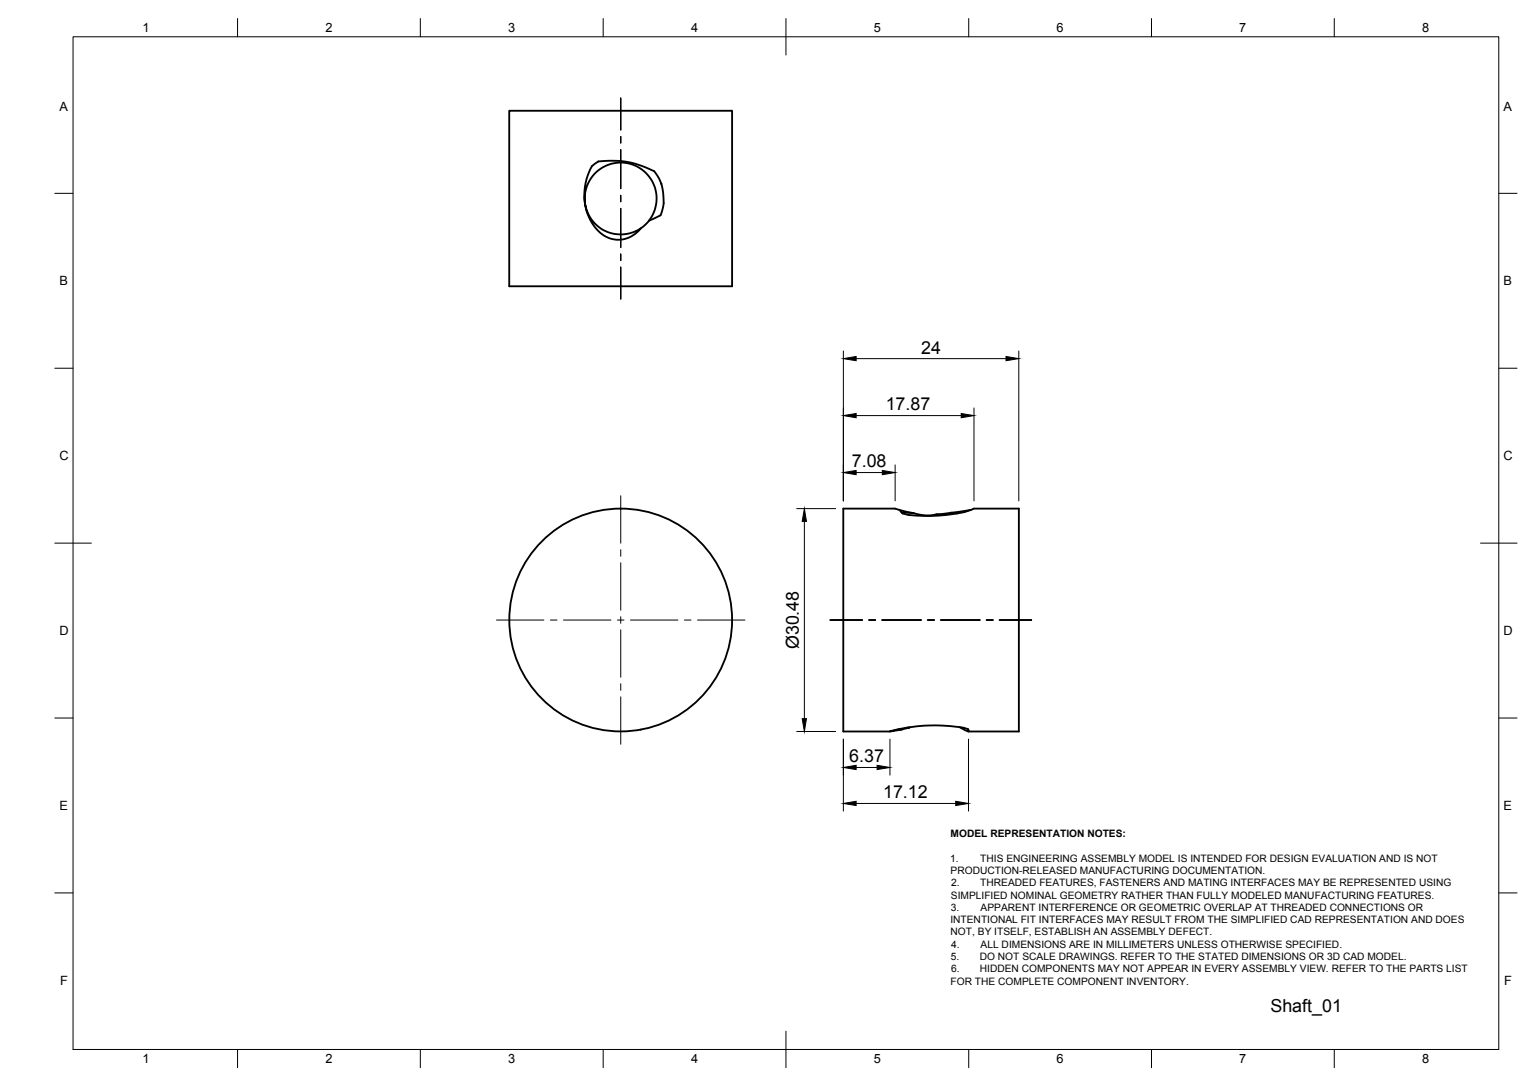
ISO-10303-21;
HEADER;
/* Generated by software containing ST-Developer
 * from STEP Tools, Inc. (www.steptools.com) 
 */

FILE_DESCRIPTION(
/* description */ (''),
/* implementation_level */ '2;1');

FILE_NAME(
/* name */ 'Shaft_01.step',
/* time_stamp */ '2026-10-06T13:41:14-07:00',
/* author */ (''),
/* organization */ (''),
/* preprocessor_version */ 'ST-DEVELOPER v20.2',
/* originating_system */ 'Autodesk Translation Framework v15.15.0.0',
/* authorisation */ '');

FILE_SCHEMA (('AUTOMOTIVE_DESIGN { 1 0 10303 214 3 1 1 }'));
ENDSEC;

DATA;
#10=MECHANICAL_DESIGN_GEOMETRIC_PRESENTATION_REPRESENTATION('',(#1963),#279266);
#49=B_SPLINE_SURFACE_WITH_KNOTS('',3,3,((#209501,#209502,#209503,#209504,
#209505,#209506,#209507,#209508,#209509,#209510,#209511,#209512,#209513,
#209514,#209515,#209516,#209517,#209518,#209519,#209520,#209521,#209522,
#209523,#209524,#209525,#209526,#209527,#209528,#209529,#209530,#209531,
#209532,#209533,#209534,#209535,#209536,#209537,#209538,#209539,#209540,
#209541,#209542,#209543,#209544,#209545,#209546,#209547,#209548,#209549,
#209550,#209551,#209552,#209553,#209554,#209555,#209556,#209557,#209558,
#209559,#209560,#209561,#209562,#209563,#209564,#209565,#209566,#209567,
#209568,#209569,#209570,#209571,#209572,#209573,#209574,#209575,#209576,
#209577,#209578,#209579,#209580,#209581,#209582,#209583,#209584,#209585,
#209586,#209587,#209588,#209589,#209590,#209591,#209592,#209593,#209594,
#209595,#209596,#209597,#209598,#209599,#209600,#209601,#209602,#209603,
#209604,#209605,#209606,#209607,#209608,#209609,#209610,#209611,#209612,
#209613,#209614,#209615,#209616,#209617,#209618,#209619,#209620,#209621,
#209622,#209623,#209624,#209625,#209626,#209627,#209628,#209629,#209630,
#209631,#209632,#209633,#209634,#209635,#209636,#209637,#209638,#209639,
#209640,#209641,#209642,#209643,#209644,#209645,#209646,#209647,#209648,
#209649,#209650,#209651,#209652,#209653,#209654,#209655,#209656,#209657,
#209658,#209659,#209660,#209661,#209662,#209663,#209664,#209665,#209666,
#209667,#209668,#209669,#209670,#209671,#209672,#209673,#209674,#209675,
#209676,#209677,#209678,#209679,#209680,#209681,#209682,#209683,#209684,
#209685,#209686,#209687,#209688,#209689,#209690,#209691,#209692,#209693,
#209694,#209695,#209696,#209697,#209698,#209699,#209700,#209701,#209702,
#209703,#209704,#209705,#209706,#209707,#209708,#209709,#209710,#209711,
#209712,#209713,#209714,#209715,#209716,#209717,#209718,#209719,#209720,
#209721,#209722,#209723,#209724,#209725,#209726,#209727,#209728,#209729,
#209730,#209731,#209732,#209733,#209734,#209735,#209736,#209737,#209738,
#209739,#209740,#209741,#209742,#209743,#209744,#209745,#209746,#209747,
#209748,#209749,#209750,#209751,#209752,#209753,#209754,#209755,#209756,
#209757,#209758,#209759,#209760,#209761,#209762,#209763,#209764,#209765,
#209766,#209767,#209768,#209769,#209770,#209771,#209772,#209773,#209774,
#209775,#209776,#209777,#209778,#209779,#209780,#209781,#209782,#209783,
#209784,#209785,#209786,#209787,#209788,#209789,#209790,#209791,#209792,
#209793,#209794,#209795,#209796,#209797,#209798,#209799,#209800,#209801,
#209802,#209803,#209804,#209805,#209806,#209807,#209808,#209809,#209810,
#209811,#209812,#209813,#209814,#209815,#209816,#209817,#209818,#209819,
#209820,#209821,#209822,#209823,#209824,#209825,#209826,#209827,#209828,
#209829,#209830,#209831,#209832,#209833,#209834,#209835,#209836,#209837,
#209838,#209839,#209840,#209841,#209842,#209843,#209844,#209845,#209846,
#209847,#209848,#209849,#209850,#209851,#209852,#209853,#209854,#209855,
#209856,#209857,#209858,#209859,#209860,#209861,#209862,#209863,#209864,
#209865,#209866,#209867,#209868,#209869,#209870,#209871,#209872,#209873,
#209874,#209875,#209876,#209877,#209878,#209879,#209880,#209881,#209882,
#209883,#209884,#209885,#209886,#209887,#209888,#209889,#209890,#209891,
#209892,#209893,#209894,#209895,#209896,#209897,#209898,#209899,#209900,
#209901,#209902,#209903,#209904,#209905,#209906,#209907,#209908,#209909,
#209910,#209911,#209912,#209913,#209914,#209915,#209916,#209917,#209918,
#209919,#209920,#209921,#209922,#209923,#209924,#209925,#209926,#209927,
#209928,#209929,#209930,#209931,#209932,#209933,#209934,#209935,#209936,
#209937,#209938,#209939,#209940,#209941,#209942,#209943,#209944,#209945,
#209946,#209947,#209948,#209949,#209950,#209951,#209952,#209953,#209954,
#209955,#209956,#209957,#209958,#209959,#209960,#209961,#209962,#209963,
#209964,#209965,#209966,#209967,#209968,#209969,#209970,#209971,#209972,
#209973,#209974,#209975,#209976,#209977,#209978,#209979,#209980,#209981,
#209982,#209983,#209984,#209985,#209986,#209987,#209988,#209989,#209990,
#209991,#209992,#209993,#209994,#209995,#209996,#209997,#209998,#209999,
#210000,#210001,#210002,#210003,#210004,#210005,#210006,#210007,#210008,
#210009,#210010,#210011,#210012,#210013,#210014,#210015,#210016,#210017,
#210018,#210019,#210020,#210021,#210022,#210023,#210024,#210025,#210026,
#210027,#210028,#210029,#210030,#210031,#210032,#210033,#210034,#210035,
#210036,#210037,#210038,#210039,#210040,#210041,#210042,#210043,#210044,
#210045,#210046,#210047,#210048,#210049,#210050,#210051,#210052,#210053,
#210054,#210055,#210056,#210057,#210058,#210059,#210060,#210061,#210062,
#210063,#210064,#210065,#210066,#210067,#210068,#210069,#210070,#210071,
#210072,#210073,#210074,#210075,#210076,#210077,#210078,#210079,#210080,
#210081,#210082,#210083,#210084,#210085,#210086,#210087,#210088,#210089,
#210090,#210091,#210092,#210093,#210094,#210095,#210096,#210097,#210098,
#210099,#210100,#210101,#210102,#210103,#210104,#210105,#210106,#210107,
#210108,#210109,#210110,#210111,#210112,#210113,#210114,#210115,#210116,
#210117,#210118,#210119,#210120,#210121,#210122,#210123,#210124,#210125,
#210126,#210127,#210128,#210129,#210130,#210131,#210132,#210133,#210134,
#210135,#210136,#210137,#210138,#210139,#210140,#210141,#210142,#210143,
#210144,#210145,#210146,#210147,#210148,#210149,#210150,#210151,#210152,
#210153,#210154,#210155,#210156,#210157,#210158,#210159,#210160,#210161,
#210162,#210163,#210164,#210165,#210166,#210167,#210168,#210169,#210170,
#210171,#210172,#210173,#210174,#210175,#210176,#210177,#210178,#210179,
#210180,#210181,#210182,#210183,#210184,#210185,#210186,#210187,#210188,
#210189,#210190,#210191,#210192,#210193,#210194,#210195,#210196,#210197,
#210198,#210199,#210200,#210201,#210202,#210203,#210204,#210205,#210206,
#210207,#210208,#210209,#210210,#210211,#210212,#210213,#210214,#210215,
#210216,#210217,#210218,#210219,#210220,#210221,#210222,#210223,#210224,
#210225,#210226,#210227,#210228,#210229,#210230,#210231,#210232,#210233,
#210234,#210235,#210236,#210237,#210238,#210239,#210240,#210241,#210242,
#210243,#210244,#210245,#210246,#210247,#210248,#210249,#210250,#210251,
#210252,#210253,#210254,#210255,#210256,#210257,#210258,#210259,#210260,
#210261,#210262,#210263,#210264,#210265,#210266,#210267,#210268,#210269,
#210270,#210271,#210272,#210273,#210274,#210275,#210276,#210277,#210278,
#210279,#210280,#210281,#210282,#210283,#210284,#210285,#210286,#210287,
#210288,#210289,#210290,#210291,#210292,#210293,#210294,#210295,#210296,
#210297,#210298,#210299,#210300,#210301,#210302,#210303,#210304,#210305,
#210306,#210307,#210308,#210309,#210310,#210311,#210312,#210313,#210314,
#210315,#210316,#210317,#210318,#210319,#210320,#210321,#210322,#210323,
#210324,#210325,#210326,#210327,#210328,#210329,#210330,#210331,#210332,
#210333,#210334,#210335,#210336,#210337,#210338,#210339,#210340,#210341,
#210342,#210343,#210344,#210345,#210346,#210347,#210348,#210349,#210350,
#210351,#210352,#210353,#210354,#210355,#210356,#210357,#210358,#210359,
#210360,#210361,#210362,#210363,#210364,#210365,#210366,#210367,#210368,
#210369,#210370,#210371,#210372,#210373,#210374,#210375,#210376,#210377,
#210378,#210379,#210380,#210381,#210382,#210383,#210384,#210385,#210386,
#210387,#210388,#210389,#210390,#210391,#210392,#210393,#210394,#210395,
#210396,#210397,#210398,#210399,#210400,#210401,#210402,#210403,#210404,
#210405,#210406,#210407,#210408,#210409,#210410,#210411,#210412,#210413,
#210414,#210415,#210416,#210417,#210418,#210419,#210420,#210421,#210422,
#210423,#210424,#210425,#210426,#210427,#210428,#210429,#210430,#210431,
#210432,#210433,#210434,#210435,#210436,#210437,#210438,#210439,#210440,
#210441,#210442,#210443,#210444,#210445,#210446,#210447,#210448,#210449,
#210450,#210451,#210452,#210453,#210454,#210455,#210456,#210457,#210458,
#210459,#210460,#210461,#210462,#210463,#210464,#210465,#210466,#210467,
#210468,#210469,#210470,#210471,#210472,#210473,#210474,#210475,#210476,
#210477,#210478,#210479,#210480,#210481,#210482,#210483,#210484,#210485,
#210486,#210487,#210488,#210489,#210490,#210491,#210492,#210493,#210494,
#210495,#210496,#210497,#210498,#210499,#210500,#210501,#210502,#210503,
#210504,#210505,#210506,#210507,#210508,#210509,#210510,#210511,#210512,
#210513,#210514,#210515,#210516,#210517,#210518,#210519,#210520,#210521,
#210522,#210523,#210524,#210525,#210526,#210527,#210528,#210529,#210530,
#210531,#210532,#210533,#210534,#210535,#210536,#210537,#210538,#210539,
#210540,#210541,#210542,#210543,#210544,#210545,#210546,#210547,#210548,
#210549,#210550,#210551,#210552,#210553,#210554,#210555,#210556,#210557,
#210558,#210559,#210560,#210561,#210562,#210563,#210564,#210565,#210566,
#210567,#210568,#210569,#210570,#210571,#210572,#210573,#210574,#210575,
#210576,#210577,#210578,#210579,#210580,#210581,#210582,#210583,#210584,
#210585,#210586,#210587,#210588,#210589,#210590,#210591,#210592,#210593,
#210594,#210595,#210596,#210597,#210598,#210599,#210600,#210601,#210602,
#210603,#210604,#210605,#210606,#210607,#210608,#210609,#210610,#210611,
#210612,#210613,#210614,#210615,#210616,#210617,#210618,#210619,#210620,
#210621,#210622,#210623,#210624,#210625,#210626,#210627,#210628,#210629,
#210630,#210631,#210632,#210633,#210634,#210635,#210636,#210637,#210638,
#210639,#210640,#210641,#210642,#210643,#210644,#210645,#210646,#210647,
#210648,#210649,#210650,#210651,#210652,#210653,#210654,#210655,#210656,
#210657,#210658,#210659,#210660,#210661,#210662,#210663,#210664,#210665,
#210666,#210667,#210668,#210669,#210670,#210671,#210672,#210673,#210674,
#210675,#210676,#210677,#210678,#210679,#210680,#210681,#210682,#210683,
#210684,#210685,#210686,#210687,#210688,#210689,#210690,#210691,#210692,
#210693,#210694,#210695,#210696,#210697,#210698,#210699,#210700,#210701,
#210702,#210703,#210704,#210705,#210706,#210707,#210708,#210709,#210710,
#210711,#210712,#210713,#210714,#210715,#210716,#210717,#210718,#210719,
#210720,#210721,#210722,#210723,#210724,#210725,#210726,#210727,#210728,
#210729,#210730,#210731,#210732,#210733,#210734,#210735,#210736,#210737,
#210738,#210739,#210740,#210741,#210742,#210743,#210744,#210745,#210746,
#210747,#210748,#210749,#210750,#210751,#210752,#210753,#210754,#210755,
#210756,#210757,#210758,#210759,#210760,#210761,#210762,#210763,#210764,
#210765,#210766,#210767,#210768,#210769,#210770,#210771,#210772,#210773,
#210774,#210775,#210776,#210777,#210778,#210779,#210780,#210781,#210782,
#210783,#210784,#210785,#210786,#210787,#210788,#210789,#210790,#210791,
#210792,#210793,#210794,#210795,#210796,#210797,#210798,#210799,#210800,
#210801,#210802,#210803,#210804,#210805,#210806,#210807,#210808,#210809,
#210810,#210811,#210812,#210813,#210814,#210815,#210816,#210817,#210818,
#210819,#210820,#210821,#210822,#210823,#210824,#210825,#210826,#210827,
#210828,#210829,#210830,#210831,#210832,#210833,#210834,#210835,#210836,
#210837,#210838,#210839,#210840,#210841,#210842,#210843,#210844,#210845,
#210846,#210847,#210848,#210849,#210850,#210851,#210852,#210853,#210854,
#210855,#210856,#210857,#210858,#210859,#210860,#210861,#210862,#210863,
#210864,#210865,#210866,#210867,#210868,#210869,#210870,#210871,#210872,
#210873,#210874,#210875,#210876,#210877,#210878,#210879,#210880,#210881,
#210882,#210883,#210884,#210885,#210886,#210887,#210888,#210889,#210890,
#210891,#210892,#210893,#210894,#210895,#210896,#210897,#210898,#210899,
#210900,#210901,#210902,#210903,#210904,#210905,#210906,#210907,#210908,
#210909,#210910,#210911,#210912,#210913,#210914,#210915,#210916,#210917,
#210918,#210919,#210920,#210921,#210922,#210923,#210924,#210925,#210926,
#210927,#210928,#210929,#210930,#210931,#210932,#210933,#210934,#210935,
#210936,#210937,#210938,#210939,#210940,#210941,#210942,#210943,#210944,
#210945,#210946,#210947,#210948,#210949,#210950,#210951,#210952,#210953,
#210954,#210955,#210956,#210957,#210958,#210959,#210960,#210961,#210962,
#210963,#210964,#210965,#210966,#210967,#210968,#210969,#210970,#210971,
#210972,#210973,#210974,#210975,#210976,#210977,#210978,#210979,#210980,
#210981,#210982,#210983,#210984,#210985,#210986,#210987,#210988,#210989,
#210990,#210991,#210992,#210993,#210994,#210995,#210996,#210997,#210998,
#210999,#211000,#211001,#211002,#211003,#211004,#211005,#211006,#211007,
#211008,#211009,#211010,#211011,#211012,#211013,#211014,#211015,#211016,
#211017,#211018,#211019,#211020,#211021,#211022,#211023,#211024,#211025,
#211026,#211027,#211028,#211029,#211030,#211031,#211032,#211033,#211034,
#211035,#211036,#211037,#211038,#211039,#211040,#211041,#211042,#211043,
#211044,#211045,#211046,#211047,#211048,#211049,#211050,#211051,#211052,
#211053,#211054,#211055,#211056,#211057,#211058,#211059,#211060,#211061,
#211062,#211063,#211064,#211065,#211066,#211067,#211068,#211069,#211070,
#211071,#211072,#211073,#211074,#211075,#211076,#211077,#211078,#211079,
#211080,#211081,#211082,#211083,#211084,#211085,#211086,#211087,#211088,
#211089,#211090,#211091,#211092,#211093,#211094,#211095,#211096,#211097,
#211098,#211099,#211100,#211101,#211102,#211103,#211104,#211105,#211106,
#211107,#211108,#211109,#211110,#211111,#211112,#211113,#211114,#211115,
#211116,#211117,#211118,#211119,#211120,#211121,#211122,#211123,#211124,
#211125,#211126,#211127,#211128,#211129,#211130,#211131,#211132,#211133,
#211134,#211135,#211136,#211137,#211138,#211139,#211140,#211141,#211142,
#211143,#211144,#211145,#211146,#211147,#211148,#211149,#211150,#211151,
#211152,#211153,#211154,#211155,#211156,#211157,#211158,#211159,#211160,
#211161,#211162,#211163,#211164,#211165,#211166,#211167,#211168,#211169,
#211170,#211171,#211172,#211173,#211174,#211175,#211176,#211177,#211178,
#211179,#211180,#211181,#211182,#211183,#211184,#211185,#211186,#211187,
#211188,#211189,#211190,#211191,#211192,#211193,#211194,#211195),(#211196,
#211197,#211198,#211199,#211200,#211201,#211202,#211203,#211204,#211205,
#211206,#211207,#211208,#211209,#211210,#211211,#211212,#211213,#211214,
#211215,#211216,#211217,#211218,#211219,#211220,#211221,#211222,#211223,
#211224,#211225,#211226,#211227,#211228,#211229,#211230,#211231,#211232,
#211233,#211234,#211235,#211236,#211237,#211238,#211239,#211240,#211241,
#211242,#211243,#211244,#211245,#211246,#211247,#211248,#211249,#211250,
#211251,#211252,#211253,#211254,#211255,#211256,#211257,#211258,#211259,
#211260,#211261,#211262,#211263,#211264,#211265,#211266,#211267,#211268,
#211269,#211270,#211271,#211272,#211273,#211274,#211275,#211276,#211277,
#211278,#211279,#211280,#211281,#211282,#211283,#211284,#211285,#211286,
#211287,#211288,#211289,#211290,#211291,#211292,#211293,#211294,#211295,
#211296,#211297,#211298,#211299,#211300,#211301,#211302,#211303,#211304,
#211305,#211306,#211307,#211308,#211309,#211310,#211311,#211312,#211313,
#211314,#211315,#211316,#211317,#211318,#211319,#211320,#211321,#211322,
#211323,#211324,#211325,#211326,#211327,#211328,#211329,#211330,#211331,
#211332,#211333,#211334,#211335,#211336,#211337,#211338,#211339,#211340,
#211341,#211342,#211343,#211344,#211345,#211346,#211347,#211348,#211349,
#211350,#211351,#211352,#211353,#211354,#211355,#211356,#211357,#211358,
#211359,#211360,#211361,#211362,#211363,#211364,#211365,#211366,#211367,
#211368,#211369,#211370,#211371,#211372,#211373,#211374,#211375,#211376,
#211377,#211378,#211379,#211380,#211381,#211382,#211383,#211384,#211385,
#211386,#211387,#211388,#211389,#211390,#211391,#211392,#211393,#211394,
#211395,#211396,#211397,#211398,#211399,#211400,#211401,#211402,#211403,
#211404,#211405,#211406,#211407,#211408,#211409,#211410,#211411,#211412,
#211413,#211414,#211415,#211416,#211417,#211418,#211419,#211420,#211421,
#211422,#211423,#211424,#211425,#211426,#211427,#211428,#211429,#211430,
#211431,#211432,#211433,#211434,#211435,#211436,#211437,#211438,#211439,
#211440,#211441,#211442,#211443,#211444,#211445,#211446,#211447,#211448,
#211449,#211450,#211451,#211452,#211453,#211454,#211455,#211456,#211457,
#211458,#211459,#211460,#211461,#211462,#211463,#211464,#211465,#211466,
#211467,#211468,#211469,#211470,#211471,#211472,#211473,#211474,#211475,
#211476,#211477,#211478,#211479,#211480,#211481,#211482,#211483,#211484,
#211485,#211486,#211487,#211488,#211489,#211490,#211491,#211492,#211493,
#211494,#211495,#211496,#211497,#211498,#211499,#211500,#211501,#211502,
#211503,#211504,#211505,#211506,#211507,#211508,#211509,#211510,#211511,
#211512,#211513,#211514,#211515,#211516,#211517,#211518,#211519,#211520,
#211521,#211522,#211523,#211524,#211525,#211526,#211527,#211528,#211529,
#211530,#211531,#211532,#211533,#211534,#211535,#211536,#211537,#211538,
#211539,#211540,#211541,#211542,#211543,#211544,#211545,#211546,#211547,
#211548,#211549,#211550,#211551,#211552,#211553,#211554,#211555,#211556,
#211557,#211558,#211559,#211560,#211561,#211562,#211563,#211564,#211565,
#211566,#211567,#211568,#211569,#211570,#211571,#211572,#211573,#211574,
#211575,#211576,#211577,#211578,#211579,#211580,#211581,#211582,#211583,
#211584,#211585,#211586,#211587,#211588,#211589,#211590,#211591,#211592,
#211593,#211594,#211595,#211596,#211597,#211598,#211599,#211600,#211601,
#211602,#211603,#211604,#211605,#211606,#211607,#211608,#211609,#211610,
#211611,#211612,#211613,#211614,#211615,#211616,#211617,#211618,#211619,
#211620,#211621,#211622,#211623,#211624,#211625,#211626,#211627,#211628,
#211629,#211630,#211631,#211632,#211633,#211634,#211635,#211636,#211637,
#211638,#211639,#211640,#211641,#211642,#211643,#211644,#211645,#211646,
#211647,#211648,#211649,#211650,#211651,#211652,#211653,#211654,#211655,
#211656,#211657,#211658,#211659,#211660,#211661,#211662,#211663,#211664,
#211665,#211666,#211667,#211668,#211669,#211670,#211671,#211672,#211673,
#211674,#211675,#211676,#211677,#211678,#211679,#211680,#211681,#211682,
#211683,#211684,#211685,#211686,#211687,#211688,#211689,#211690,#211691,
#211692,#211693,#211694,#211695,#211696,#211697,#211698,#211699,#211700,
#211701,#211702,#211703,#211704,#211705,#211706,#211707,#211708,#211709,
#211710,#211711,#211712,#211713,#211714,#211715,#211716,#211717,#211718,
#211719,#211720,#211721,#211722,#211723,#211724,#211725,#211726,#211727,
#211728,#211729,#211730,#211731,#211732,#211733,#211734,#211735,#211736,
#211737,#211738,#211739,#211740,#211741,#211742,#211743,#211744,#211745,
#211746,#211747,#211748,#211749,#211750,#211751,#211752,#211753,#211754,
#211755,#211756,#211757,#211758,#211759,#211760,#211761,#211762,#211763,
#211764,#211765,#211766,#211767,#211768,#211769,#211770,#211771,#211772,
#211773,#211774,#211775,#211776,#211777,#211778,#211779,#211780,#211781,
#211782,#211783,#211784,#211785,#211786,#211787,#211788,#211789,#211790,
#211791,#211792,#211793,#211794,#211795,#211796,#211797,#211798,#211799,
#211800,#211801,#211802,#211803,#211804,#211805,#211806,#211807,#211808,
#211809,#211810,#211811,#211812,#211813,#211814,#211815,#211816,#211817,
#211818,#211819,#211820,#211821,#211822,#211823,#211824,#211825,#211826,
#211827,#211828,#211829,#211830,#211831,#211832,#211833,#211834,#211835,
#211836,#211837,#211838,#211839,#211840,#211841,#211842,#211843,#211844,
#211845,#211846,#211847,#211848,#211849,#211850,#211851,#211852,#211853,
#211854,#211855,#211856,#211857,#211858,#211859,#211860,#211861,#211862,
#211863,#211864,#211865,#211866,#211867,#211868,#211869,#211870,#211871,
#211872,#211873,#211874,#211875,#211876,#211877,#211878,#211879,#211880,
#211881,#211882,#211883,#211884,#211885,#211886,#211887,#211888,#211889,
#211890,#211891,#211892,#211893,#211894,#211895,#211896,#211897,#211898,
#211899,#211900,#211901,#211902,#211903,#211904,#211905,#211906,#211907,
#211908,#211909,#211910,#211911,#211912,#211913,#211914,#211915,#211916,
#211917,#211918,#211919,#211920,#211921,#211922,#211923,#211924,#211925,
#211926,#211927,#211928,#211929,#211930,#211931,#211932,#211933,#211934,
#211935,#211936,#211937,#211938,#211939,#211940,#211941,#211942,#211943,
#211944,#211945,#211946,#211947,#211948,#211949,#211950,#211951,#211952,
#211953,#211954,#211955,#211956,#211957,#211958,#211959,#211960,#211961,
#211962,#211963,#211964,#211965,#211966,#211967,#211968,#211969,#211970,
#211971,#211972,#211973,#211974,#211975,#211976,#211977,#211978,#211979,
#211980,#211981,#211982,#211983,#211984,#211985,#211986,#211987,#211988,
#211989,#211990,#211991,#211992,#211993,#211994,#211995,#211996,#211997,
#211998,#211999,#212000,#212001,#212002,#212003,#212004,#212005,#212006,
#212007,#212008,#212009,#212010,#212011,#212012,#212013,#212014,#212015,
#212016,#212017,#212018,#212019,#212020,#212021,#212022,#212023,#212024,
#212025,#212026,#212027,#212028,#212029,#212030,#212031,#212032,#212033,
#212034,#212035,#212036,#212037,#212038,#212039,#212040,#212041,#212042,
#212043,#212044,#212045,#212046,#212047,#212048,#212049,#212050,#212051,
#212052,#212053,#212054,#212055,#212056,#212057,#212058,#212059,#212060,
#212061,#212062,#212063,#212064,#212065,#212066,#212067,#212068,#212069,
#212070,#212071,#212072,#212073,#212074,#212075,#212076,#212077,#212078,
#212079,#212080,#212081,#212082,#212083,#212084,#212085,#212086,#212087,
#212088,#212089,#212090,#212091,#212092,#212093,#212094,#212095,#212096,
#212097,#212098,#212099,#212100,#212101,#212102,#212103,#212104,#212105,
#212106,#212107,#212108,#212109,#212110,#212111,#212112,#212113,#212114,
#212115,#212116,#212117,#212118,#212119,#212120,#212121,#212122,#212123,
#212124,#212125,#212126,#212127,#212128,#212129,#212130,#212131,#212132,
#212133,#212134,#212135,#212136,#212137,#212138,#212139,#212140,#212141,
#212142,#212143,#212144,#212145,#212146,#212147,#212148,#212149,#212150,
#212151,#212152,#212153,#212154,#212155,#212156,#212157,#212158,#212159,
#212160,#212161,#212162,#212163,#212164,#212165,#212166,#212167,#212168,
#212169,#212170,#212171,#212172,#212173,#212174,#212175,#212176,#212177,
#212178,#212179,#212180,#212181,#212182,#212183,#212184,#212185,#212186,
#212187,#212188,#212189,#212190,#212191,#212192,#212193,#212194,#212195,
#212196,#212197,#212198,#212199,#212200,#212201,#212202,#212203,#212204,
#212205,#212206,#212207,#212208,#212209,#212210,#212211,#212212,#212213,
#212214,#212215,#212216,#212217,#212218,#212219,#212220,#212221,#212222,
#212223,#212224,#212225,#212226,#212227,#212228,#212229,#212230,#212231,
#212232,#212233,#212234,#212235,#212236,#212237,#212238,#212239,#212240,
#212241,#212242,#212243,#212244,#212245,#212246,#212247,#212248,#212249,
#212250,#212251,#212252,#212253,#212254,#212255,#212256,#212257,#212258,
#212259,#212260,#212261,#212262,#212263,#212264,#212265,#212266,#212267,
#212268,#212269,#212270,#212271,#212272,#212273,#212274,#212275,#212276,
#212277,#212278,#212279,#212280,#212281,#212282,#212283,#212284,#212285,
#212286,#212287,#212288,#212289,#212290,#212291,#212292,#212293,#212294,
#212295,#212296,#212297,#212298,#212299,#212300,#212301,#212302,#212303,
#212304,#212305,#212306,#212307,#212308,#212309,#212310,#212311,#212312,
#212313,#212314,#212315,#212316,#212317,#212318,#212319,#212320,#212321,
#212322,#212323,#212324,#212325,#212326,#212327,#212328,#212329,#212330,
#212331,#212332,#212333,#212334,#212335,#212336,#212337,#212338,#212339,
#212340,#212341,#212342,#212343,#212344,#212345,#212346,#212347,#212348,
#212349,#212350,#212351,#212352,#212353,#212354,#212355,#212356,#212357,
#212358,#212359,#212360,#212361,#212362,#212363,#212364,#212365,#212366,
#212367,#212368,#212369,#212370,#212371,#212372,#212373,#212374,#212375,
#212376,#212377,#212378,#212379,#212380,#212381,#212382,#212383,#212384,
#212385,#212386,#212387,#212388,#212389,#212390,#212391,#212392,#212393,
#212394,#212395,#212396,#212397,#212398,#212399,#212400,#212401,#212402,
#212403,#212404,#212405,#212406,#212407,#212408,#212409,#212410,#212411,
#212412,#212413,#212414,#212415,#212416,#212417,#212418,#212419,#212420,
#212421,#212422,#212423,#212424,#212425,#212426,#212427,#212428,#212429,
#212430,#212431,#212432,#212433,#212434,#212435,#212436,#212437,#212438,
#212439,#212440,#212441,#212442,#212443,#212444,#212445,#212446,#212447,
#212448,#212449,#212450,#212451,#212452,#212453,#212454,#212455,#212456,
#212457,#212458,#212459,#212460,#212461,#212462,#212463,#212464,#212465,
#212466,#212467,#212468,#212469,#212470,#212471,#212472,#212473,#212474,
#212475,#212476,#212477,#212478,#212479,#212480,#212481,#212482,#212483,
#212484,#212485,#212486,#212487,#212488,#212489,#212490,#212491,#212492,
#212493,#212494,#212495,#212496,#212497,#212498,#212499,#212500,#212501,
#212502,#212503,#212504,#212505,#212506,#212507,#212508,#212509,#212510,
#212511,#212512,#212513,#212514,#212515,#212516,#212517,#212518,#212519,
#212520,#212521,#212522,#212523,#212524,#212525,#212526,#212527,#212528,
#212529,#212530,#212531,#212532,#212533,#212534,#212535,#212536,#212537,
#212538,#212539,#212540,#212541,#212542,#212543,#212544,#212545,#212546,
#212547,#212548,#212549,#212550,#212551,#212552,#212553,#212554,#212555,
#212556,#212557,#212558,#212559,#212560,#212561,#212562,#212563,#212564,
#212565,#212566,#212567,#212568,#212569,#212570,#212571,#212572,#212573,
#212574,#212575,#212576,#212577,#212578,#212579,#212580,#212581,#212582,
#212583,#212584,#212585,#212586,#212587,#212588,#212589,#212590,#212591,
#212592,#212593,#212594,#212595,#212596,#212597,#212598,#212599,#212600,
#212601,#212602,#212603,#212604,#212605,#212606,#212607,#212608,#212609,
#212610,#212611,#212612,#212613,#212614,#212615,#212616,#212617,#212618,
#212619,#212620,#212621,#212622,#212623,#212624,#212625,#212626,#212627,
#212628,#212629,#212630,#212631,#212632,#212633,#212634,#212635,#212636,
#212637,#212638,#212639,#212640,#212641,#212642,#212643,#212644,#212645,
#212646,#212647,#212648,#212649,#212650,#212651,#212652,#212653,#212654,
#212655,#212656,#212657,#212658,#212659,#212660,#212661,#212662,#212663,
#212664,#212665,#212666,#212667,#212668,#212669,#212670,#212671,#212672,
#212673,#212674,#212675,#212676,#212677,#212678,#212679,#212680,#212681,
#212682,#212683,#212684,#212685,#212686,#212687,#212688,#212689,#212690,
#212691,#212692,#212693,#212694,#212695,#212696,#212697,#212698,#212699,
#212700,#212701,#212702,#212703,#212704,#212705,#212706,#212707,#212708,
#212709,#212710,#212711,#212712,#212713,#212714,#212715,#212716,#212717,
#212718,#212719,#212720,#212721,#212722,#212723,#212724,#212725,#212726,
#212727,#212728,#212729,#212730,#212731,#212732,#212733,#212734,#212735,
#212736,#212737,#212738,#212739,#212740,#212741,#212742,#212743,#212744,
#212745,#212746,#212747,#212748,#212749,#212750,#212751,#212752,#212753,
#212754,#212755,#212756,#212757,#212758,#212759,#212760,#212761,#212762,
#212763,#212764,#212765,#212766,#212767,#212768,#212769,#212770,#212771,
#212772,#212773,#212774,#212775,#212776,#212777,#212778,#212779,#212780,
#212781,#212782,#212783,#212784,#212785,#212786,#212787,#212788,#212789,
#212790,#212791,#212792,#212793,#212794,#212795,#212796,#212797,#212798,
#212799,#212800,#212801,#212802,#212803,#212804,#212805,#212806,#212807,
#212808,#212809,#212810,#212811,#212812,#212813,#212814,#212815,#212816,
#212817,#212818,#212819,#212820,#212821,#212822,#212823,#212824,#212825,
#212826,#212827,#212828,#212829,#212830,#212831,#212832,#212833,#212834,
#212835,#212836,#212837,#212838,#212839,#212840,#212841,#212842,#212843,
#212844,#212845,#212846,#212847,#212848,#212849,#212850,#212851,#212852,
#212853,#212854,#212855,#212856,#212857,#212858,#212859,#212860,#212861,
#212862,#212863,#212864,#212865,#212866,#212867,#212868,#212869,#212870,
#212871,#212872,#212873,#212874,#212875,#212876,#212877,#212878,#212879,
#212880,#212881,#212882,#212883,#212884,#212885,#212886,#212887,#212888,
#212889,#212890),(#212891,#212892,#212893,#212894,#212895,#212896,#212897,
#212898,#212899,#212900,#212901,#212902,#212903,#212904,#212905,#212906,
#212907,#212908,#212909,#212910,#212911,#212912,#212913,#212914,#212915,
#212916,#212917,#212918,#212919,#212920,#212921,#212922,#212923,#212924,
#212925,#212926,#212927,#212928,#212929,#212930,#212931,#212932,#212933,
#212934,#212935,#212936,#212937,#212938,#212939,#212940,#212941,#212942,
#212943,#212944,#212945,#212946,#212947,#212948,#212949,#212950,#212951,
#212952,#212953,#212954,#212955,#212956,#212957,#212958,#212959,#212960,
#212961,#212962,#212963,#212964,#212965,#212966,#212967,#212968,#212969,
#212970,#212971,#212972,#212973,#212974,#212975,#212976,#212977,#212978,
#212979,#212980,#212981,#212982,#212983,#212984,#212985,#212986,#212987,
#212988,#212989,#212990,#212991,#212992,#212993,#212994,#212995,#212996,
#212997,#212998,#212999,#213000,#213001,#213002,#213003,#213004,#213005,
#213006,#213007,#213008,#213009,#213010,#213011,#213012,#213013,#213014,
#213015,#213016,#213017,#213018,#213019,#213020,#213021,#213022,#213023,
#213024,#213025,#213026,#213027,#213028,#213029,#213030,#213031,#213032,
#213033,#213034,#213035,#213036,#213037,#213038,#213039,#213040,#213041,
#213042,#213043,#213044,#213045,#213046,#213047,#213048,#213049,#213050,
#213051,#213052,#213053,#213054,#213055,#213056,#213057,#213058,#213059,
#213060,#213061,#213062,#213063,#213064,#213065,#213066,#213067,#213068,
#213069,#213070,#213071,#213072,#213073,#213074,#213075,#213076,#213077,
#213078,#213079,#213080,#213081,#213082,#213083,#213084,#213085,#213086,
#213087,#213088,#213089,#213090,#213091,#213092,#213093,#213094,#213095,
#213096,#213097,#213098,#213099,#213100,#213101,#213102,#213103,#213104,
#213105,#213106,#213107,#213108,#213109,#213110,#213111,#213112,#213113,
#213114,#213115,#213116,#213117,#213118,#213119,#213120,#213121,#213122,
#213123,#213124,#213125,#213126,#213127,#213128,#213129,#213130,#213131,
#213132,#213133,#213134,#213135,#213136,#213137,#213138,#213139,#213140,
#213141,#213142,#213143,#213144,#213145,#213146,#213147,#213148,#213149,
#213150,#213151,#213152,#213153,#213154,#213155,#213156,#213157,#213158,
#213159,#213160,#213161,#213162,#213163,#213164,#213165,#213166,#213167,
#213168,#213169,#213170,#213171,#213172,#213173,#213174,#213175,#213176,
#213177,#213178,#213179,#213180,#213181,#213182,#213183,#213184,#213185,
#213186,#213187,#213188,#213189,#213190,#213191,#213192,#213193,#213194,
#213195,#213196,#213197,#213198,#213199,#213200,#213201,#213202,#213203,
#213204,#213205,#213206,#213207,#213208,#213209,#213210,#213211,#213212,
#213213,#213214,#213215,#213216,#213217,#213218,#213219,#213220,#213221,
#213222,#213223,#213224,#213225,#213226,#213227,#213228,#213229,#213230,
#213231,#213232,#213233,#213234,#213235,#213236,#213237,#213238,#213239,
#213240,#213241,#213242,#213243,#213244,#213245,#213246,#213247,#213248,
#213249,#213250,#213251,#213252,#213253,#213254,#213255,#213256,#213257,
#213258,#213259,#213260,#213261,#213262,#213263,#213264,#213265,#213266,
#213267,#213268,#213269,#213270,#213271,#213272,#213273,#213274,#213275,
#213276,#213277,#213278,#213279,#213280,#213281,#213282,#213283,#213284,
#213285,#213286,#213287,#213288,#213289,#213290,#213291,#213292,#213293,
#213294,#213295,#213296,#213297,#213298,#213299,#213300,#213301,#213302,
#213303,#213304,#213305,#213306,#213307,#213308,#213309,#213310,#213311,
#213312,#213313,#213314,#213315,#213316,#213317,#213318,#213319,#213320,
#213321,#213322,#213323,#213324,#213325,#213326,#213327,#213328,#213329,
#213330,#213331,#213332,#213333,#213334,#213335,#213336,#213337,#213338,
#213339,#213340,#213341,#213342,#213343,#213344,#213345,#213346,#213347,
#213348,#213349,#213350,#213351,#213352,#213353,#213354,#213355,#213356,
#213357,#213358,#213359,#213360,#213361,#213362,#213363,#213364,#213365,
#213366,#213367,#213368,#213369,#213370,#213371,#213372,#213373,#213374,
#213375,#213376,#213377,#213378,#213379,#213380,#213381,#213382,#213383,
#213384,#213385,#213386,#213387,#213388,#213389,#213390,#213391,#213392,
#213393,#213394,#213395,#213396,#213397,#213398,#213399,#213400,#213401,
#213402,#213403,#213404,#213405,#213406,#213407,#213408,#213409,#213410,
#213411,#213412,#213413,#213414,#213415,#213416,#213417,#213418,#213419,
#213420,#213421,#213422,#213423,#213424,#213425,#213426,#213427,#213428,
#213429,#213430,#213431,#213432,#213433,#213434,#213435,#213436,#213437,
#213438,#213439,#213440,#213441,#213442,#213443,#213444,#213445,#213446,
#213447,#213448,#213449,#213450,#213451,#213452,#213453,#213454,#213455,
#213456,#213457,#213458,#213459,#213460,#213461,#213462,#213463,#213464,
#213465,#213466,#213467,#213468,#213469,#213470,#213471,#213472,#213473,
#213474,#213475,#213476,#213477,#213478,#213479,#213480,#213481,#213482,
#213483,#213484,#213485,#213486,#213487,#213488,#213489,#213490,#213491,
#213492,#213493,#213494,#213495,#213496,#213497,#213498,#213499,#213500,
#213501,#213502,#213503,#213504,#213505,#213506,#213507,#213508,#213509,
#213510,#213511,#213512,#213513,#213514,#213515,#213516,#213517,#213518,
#213519,#213520,#213521,#213522,#213523,#213524,#213525,#213526,#213527,
#213528,#213529,#213530,#213531,#213532,#213533,#213534,#213535,#213536,
#213537,#213538,#213539,#213540,#213541,#213542,#213543,#213544,#213545,
#213546,#213547,#213548,#213549,#213550,#213551,#213552,#213553,#213554,
#213555,#213556,#213557,#213558,#213559,#213560,#213561,#213562,#213563,
#213564,#213565,#213566,#213567,#213568,#213569,#213570,#213571,#213572,
#213573,#213574,#213575,#213576,#213577,#213578,#213579,#213580,#213581,
#213582,#213583,#213584,#213585,#213586,#213587,#213588,#213589,#213590,
#213591,#213592,#213593,#213594,#213595,#213596,#213597,#213598,#213599,
#213600,#213601,#213602,#213603,#213604,#213605,#213606,#213607,#213608,
#213609,#213610,#213611,#213612,#213613,#213614,#213615,#213616,#213617,
#213618,#213619,#213620,#213621,#213622,#213623,#213624,#213625,#213626,
#213627,#213628,#213629,#213630,#213631,#213632,#213633,#213634,#213635,
#213636,#213637,#213638,#213639,#213640,#213641,#213642,#213643,#213644,
#213645,#213646,#213647,#213648,#213649,#213650,#213651,#213652,#213653,
#213654,#213655,#213656,#213657,#213658,#213659,#213660,#213661,#213662,
#213663,#213664,#213665,#213666,#213667,#213668,#213669,#213670,#213671,
#213672,#213673,#213674,#213675,#213676,#213677,#213678,#213679,#213680,
#213681,#213682,#213683,#213684,#213685,#213686,#213687,#213688,#213689,
#213690,#213691,#213692,#213693,#213694,#213695,#213696,#213697,#213698,
#213699,#213700,#213701,#213702,#213703,#213704,#213705,#213706,#213707,
#213708,#213709,#213710,#213711,#213712,#213713,#213714,#213715,#213716,
#213717,#213718,#213719,#213720,#213721,#213722,#213723,#213724,#213725,
#213726,#213727,#213728,#213729,#213730,#213731,#213732,#213733,#213734,
#213735,#213736,#213737,#213738,#213739,#213740,#213741,#213742,#213743,
#213744,#213745,#213746,#213747,#213748,#213749,#213750,#213751,#213752,
#213753,#213754,#213755,#213756,#213757,#213758,#213759,#213760,#213761,
#213762,#213763,#213764,#213765,#213766,#213767,#213768,#213769,#213770,
#213771,#213772,#213773,#213774,#213775,#213776,#213777,#213778,#213779,
#213780,#213781,#213782,#213783,#213784,#213785,#213786,#213787,#213788,
#213789,#213790,#213791,#213792,#213793,#213794,#213795,#213796,#213797,
#213798,#213799,#213800,#213801,#213802,#213803,#213804,#213805,#213806,
#213807,#213808,#213809,#213810,#213811,#213812,#213813,#213814,#213815,
#213816,#213817,#213818,#213819,#213820,#213821,#213822,#213823,#213824,
#213825,#213826,#213827,#213828,#213829,#213830,#213831,#213832,#213833,
#213834,#213835,#213836,#213837,#213838,#213839,#213840,#213841,#213842,
#213843,#213844,#213845,#213846,#213847,#213848,#213849,#213850,#213851,
#213852,#213853,#213854,#213855,#213856,#213857,#213858,#213859,#213860,
#213861,#213862,#213863,#213864,#213865,#213866,#213867,#213868,#213869,
#213870,#213871,#213872,#213873,#213874,#213875,#213876,#213877,#213878,
#213879,#213880,#213881,#213882,#213883,#213884,#213885,#213886,#213887,
#213888,#213889,#213890,#213891,#213892,#213893,#213894,#213895,#213896,
#213897,#213898,#213899,#213900,#213901,#213902,#213903,#213904,#213905,
#213906,#213907,#213908,#213909,#213910,#213911,#213912,#213913,#213914,
#213915,#213916,#213917,#213918,#213919,#213920,#213921,#213922,#213923,
#213924,#213925,#213926,#213927,#213928,#213929,#213930,#213931,#213932,
#213933,#213934,#213935,#213936,#213937,#213938,#213939,#213940,#213941,
#213942,#213943,#213944,#213945,#213946,#213947,#213948,#213949,#213950,
#213951,#213952,#213953,#213954,#213955,#213956,#213957,#213958,#213959,
#213960,#213961,#213962,#213963,#213964,#213965,#213966,#213967,#213968,
#213969,#213970,#213971,#213972,#213973,#213974,#213975,#213976,#213977,
#213978,#213979,#213980,#213981,#213982,#213983,#213984,#213985,#213986,
#213987,#213988,#213989,#213990,#213991,#213992,#213993,#213994,#213995,
#213996,#213997,#213998,#213999,#214000,#214001,#214002,#214003,#214004,
#214005,#214006,#214007,#214008,#214009,#214010,#214011,#214012,#214013,
#214014,#214015,#214016,#214017,#214018,#214019,#214020,#214021,#214022,
#214023,#214024,#214025,#214026,#214027,#214028,#214029,#214030,#214031,
#214032,#214033,#214034,#214035,#214036,#214037,#214038,#214039,#214040,
#214041,#214042,#214043,#214044,#214045,#214046,#214047,#214048,#214049,
#214050,#214051,#214052,#214053,#214054,#214055,#214056,#214057,#214058,
#214059,#214060,#214061,#214062,#214063,#214064,#214065,#214066,#214067,
#214068,#214069,#214070,#214071,#214072,#214073,#214074,#214075,#214076,
#214077,#214078,#214079,#214080,#214081,#214082,#214083,#214084,#214085,
#214086,#214087,#214088,#214089,#214090,#214091,#214092,#214093,#214094,
#214095,#214096,#214097,#214098,#214099,#214100,#214101,#214102,#214103,
#214104,#214105,#214106,#214107,#214108,#214109,#214110,#214111,#214112,
#214113,#214114,#214115,#214116,#214117,#214118,#214119,#214120,#214121,
#214122,#214123,#214124,#214125,#214126,#214127,#214128,#214129,#214130,
#214131,#214132,#214133,#214134,#214135,#214136,#214137,#214138,#214139,
#214140,#214141,#214142,#214143,#214144,#214145,#214146,#214147,#214148,
#214149,#214150,#214151,#214152,#214153,#214154,#214155,#214156,#214157,
#214158,#214159,#214160,#214161,#214162,#214163,#214164,#214165,#214166,
#214167,#214168,#214169,#214170,#214171,#214172,#214173,#214174,#214175,
#214176,#214177,#214178,#214179,#214180,#214181,#214182,#214183,#214184,
#214185,#214186,#214187,#214188,#214189,#214190,#214191,#214192,#214193,
#214194,#214195,#214196,#214197,#214198,#214199,#214200,#214201,#214202,
#214203,#214204,#214205,#214206,#214207,#214208,#214209,#214210,#214211,
#214212,#214213,#214214,#214215,#214216,#214217,#214218,#214219,#214220,
#214221,#214222,#214223,#214224,#214225,#214226,#214227,#214228,#214229,
#214230,#214231,#214232,#214233,#214234,#214235,#214236,#214237,#214238,
#214239,#214240,#214241,#214242,#214243,#214244,#214245,#214246,#214247,
#214248,#214249,#214250,#214251,#214252,#214253,#214254,#214255,#214256,
#214257,#214258,#214259,#214260,#214261,#214262,#214263,#214264,#214265,
#214266,#214267,#214268,#214269,#214270,#214271,#214272,#214273,#214274,
#214275,#214276,#214277,#214278,#214279,#214280,#214281,#214282,#214283,
#214284,#214285,#214286,#214287,#214288,#214289,#214290,#214291,#214292,
#214293,#214294,#214295,#214296,#214297,#214298,#214299,#214300,#214301,
#214302,#214303,#214304,#214305,#214306,#214307,#214308,#214309,#214310,
#214311,#214312,#214313,#214314,#214315,#214316,#214317,#214318,#214319,
#214320,#214321,#214322,#214323,#214324,#214325,#214326,#214327,#214328,
#214329,#214330,#214331,#214332,#214333,#214334,#214335,#214336,#214337,
#214338,#214339,#214340,#214341,#214342,#214343,#214344,#214345,#214346,
#214347,#214348,#214349,#214350,#214351,#214352,#214353,#214354,#214355,
#214356,#214357,#214358,#214359,#214360,#214361,#214362,#214363,#214364,
#214365,#214366,#214367,#214368,#214369,#214370,#214371,#214372,#214373,
#214374,#214375,#214376,#214377,#214378,#214379,#214380,#214381,#214382,
#214383,#214384,#214385,#214386,#214387,#214388,#214389,#214390,#214391,
#214392,#214393,#214394,#214395,#214396,#214397,#214398,#214399,#214400,
#214401,#214402,#214403,#214404,#214405,#214406,#214407,#214408,#214409,
#214410,#214411,#214412,#214413,#214414,#214415,#214416,#214417,#214418,
#214419,#214420,#214421,#214422,#214423,#214424,#214425,#214426,#214427,
#214428,#214429,#214430,#214431,#214432,#214433,#214434,#214435,#214436,
#214437,#214438,#214439,#214440,#214441,#214442,#214443,#214444,#214445,
#214446,#214447,#214448,#214449,#214450,#214451,#214452,#214453,#214454,
#214455,#214456,#214457,#214458,#214459,#214460,#214461,#214462,#214463,
#214464,#214465,#214466,#214467,#214468,#214469,#214470,#214471,#214472,
#214473,#214474,#214475,#214476,#214477,#214478,#214479,#214480,#214481,
#214482,#214483,#214484,#214485,#214486,#214487,#214488,#214489,#214490,
#214491,#214492,#214493,#214494,#214495,#214496,#214497,#214498,#214499,
#214500,#214501,#214502,#214503,#214504,#214505,#214506,#214507,#214508,
#214509,#214510,#214511,#214512,#214513,#214514,#214515,#214516,#214517,
#214518,#214519,#214520,#214521,#214522,#214523,#214524,#214525,#214526,
#214527,#214528,#214529,#214530,#214531,#214532,#214533,#214534,#214535,
#214536,#214537,#214538,#214539,#214540,#214541,#214542,#214543,#214544,
#214545,#214546,#214547,#214548,#214549,#214550,#214551,#214552,#214553,
#214554,#214555,#214556,#214557,#214558,#214559,#214560,#214561,#214562,
#214563,#214564,#214565,#214566,#214567,#214568,#214569,#214570,#214571,
#214572,#214573,#214574,#214575,#214576,#214577,#214578,#214579,#214580,
#214581,#214582,#214583,#214584,#214585),(#214586,#214587,#214588,#214589,
#214590,#214591,#214592,#214593,#214594,#214595,#214596,#214597,#214598,
#214599,#214600,#214601,#214602,#214603,#214604,#214605,#214606,#214607,
#214608,#214609,#214610,#214611,#214612,#214613,#214614,#214615,#214616,
#214617,#214618,#214619,#214620,#214621,#214622,#214623,#214624,#214625,
#214626,#214627,#214628,#214629,#214630,#214631,#214632,#214633,#214634,
#214635,#214636,#214637,#214638,#214639,#214640,#214641,#214642,#214643,
#214644,#214645,#214646,#214647,#214648,#214649,#214650,#214651,#214652,
#214653,#214654,#214655,#214656,#214657,#214658,#214659,#214660,#214661,
#214662,#214663,#214664,#214665,#214666,#214667,#214668,#214669,#214670,
#214671,#214672,#214673,#214674,#214675,#214676,#214677,#214678,#214679,
#214680,#214681,#214682,#214683,#214684,#214685,#214686,#214687,#214688,
#214689,#214690,#214691,#214692,#214693,#214694,#214695,#214696,#214697,
#214698,#214699,#214700,#214701,#214702,#214703,#214704,#214705,#214706,
#214707,#214708,#214709,#214710,#214711,#214712,#214713,#214714,#214715,
#214716,#214717,#214718,#214719,#214720,#214721,#214722,#214723,#214724,
#214725,#214726,#214727,#214728,#214729,#214730,#214731,#214732,#214733,
#214734,#214735,#214736,#214737,#214738,#214739,#214740,#214741,#214742,
#214743,#214744,#214745,#214746,#214747,#214748,#214749,#214750,#214751,
#214752,#214753,#214754,#214755,#214756,#214757,#214758,#214759,#214760,
#214761,#214762,#214763,#214764,#214765,#214766,#214767,#214768,#214769,
#214770,#214771,#214772,#214773,#214774,#214775,#214776,#214777,#214778,
#214779,#214780,#214781,#214782,#214783,#214784,#214785,#214786,#214787,
#214788,#214789,#214790,#214791,#214792,#214793,#214794,#214795,#214796,
#214797,#214798,#214799,#214800,#214801,#214802,#214803,#214804,#214805,
#214806,#214807,#214808,#214809,#214810,#214811,#214812,#214813,#214814,
#214815,#214816,#214817,#214818,#214819,#214820,#214821,#214822,#214823,
#214824,#214825,#214826,#214827,#214828,#214829,#214830,#214831,#214832,
#214833,#214834,#214835,#214836,#214837,#214838,#214839,#214840,#214841,
#214842,#214843,#214844,#214845,#214846,#214847,#214848,#214849,#214850,
#214851,#214852,#214853,#214854,#214855,#214856,#214857,#214858,#214859,
#214860,#214861,#214862,#214863,#214864,#214865,#214866,#214867,#214868,
#214869,#214870,#214871,#214872,#214873,#214874,#214875,#214876,#214877,
#214878,#214879,#214880,#214881,#214882,#214883,#214884,#214885,#214886,
#214887,#214888,#214889,#214890,#214891,#214892,#214893,#214894,#214895,
#214896,#214897,#214898,#214899,#214900,#214901,#214902,#214903,#214904,
#214905,#214906,#214907,#214908,#214909,#214910,#214911,#214912,#214913,
#214914,#214915,#214916,#214917,#214918,#214919,#214920,#214921,#214922,
#214923,#214924,#214925,#214926,#214927,#214928,#214929,#214930,#214931,
#214932,#214933,#214934,#214935,#214936,#214937,#214938,#214939,#214940,
#214941,#214942,#214943,#214944,#214945,#214946,#214947,#214948,#214949,
#214950,#214951,#214952,#214953,#214954,#214955,#214956,#214957,#214958,
#214959,#214960,#214961,#214962,#214963,#214964,#214965,#214966,#214967,
#214968,#214969,#214970,#214971,#214972,#214973,#214974,#214975,#214976,
#214977,#214978,#214979,#214980,#214981,#214982,#214983,#214984,#214985,
#214986,#214987,#214988,#214989,#214990,#214991,#214992,#214993,#214994,
#214995,#214996,#214997,#214998,#214999,#215000,#215001,#215002,#215003,
#215004,#215005,#215006,#215007,#215008,#215009,#215010,#215011,#215012,
#215013,#215014,#215015,#215016,#215017,#215018,#215019,#215020,#215021,
#215022,#215023,#215024,#215025,#215026,#215027,#215028,#215029,#215030,
#215031,#215032,#215033,#215034,#215035,#215036,#215037,#215038,#215039,
#215040,#215041,#215042,#215043,#215044,#215045,#215046,#215047,#215048,
#215049,#215050,#215051,#215052,#215053,#215054,#215055,#215056,#215057,
#215058,#215059,#215060,#215061,#215062,#215063,#215064,#215065,#215066,
#215067,#215068,#215069,#215070,#215071,#215072,#215073,#215074,#215075,
#215076,#215077,#215078,#215079,#215080,#215081,#215082,#215083,#215084,
#215085,#215086,#215087,#215088,#215089,#215090,#215091,#215092,#215093,
#215094,#215095,#215096,#215097,#215098,#215099,#215100,#215101,#215102,
#215103,#215104,#215105,#215106,#215107,#215108,#215109,#215110,#215111,
#215112,#215113,#215114,#215115,#215116,#215117,#215118,#215119,#215120,
#215121,#215122,#215123,#215124,#215125,#215126,#215127,#215128,#215129,
#215130,#215131,#215132,#215133,#215134,#215135,#215136,#215137,#215138,
#215139,#215140,#215141,#215142,#215143,#215144,#215145,#215146,#215147,
#215148,#215149,#215150,#215151,#215152,#215153,#215154,#215155,#215156,
#215157,#215158,#215159,#215160,#215161,#215162,#215163,#215164,#215165,
#215166,#215167,#215168,#215169,#215170,#215171,#215172,#215173,#215174,
#215175,#215176,#215177,#215178,#215179,#215180,#215181,#215182,#215183,
#215184,#215185,#215186,#215187,#215188,#215189,#215190,#215191,#215192,
#215193,#215194,#215195,#215196,#215197,#215198,#215199,#215200,#215201,
#215202,#215203,#215204,#215205,#215206,#215207,#215208,#215209,#215210,
#215211,#215212,#215213,#215214,#215215,#215216,#215217,#215218,#215219,
#215220,#215221,#215222,#215223,#215224,#215225,#215226,#215227,#215228,
#215229,#215230,#215231,#215232,#215233,#215234,#215235,#215236,#215237,
#215238,#215239,#215240,#215241,#215242,#215243,#215244,#215245,#215246,
#215247,#215248,#215249,#215250,#215251,#215252,#215253,#215254,#215255,
#215256,#215257,#215258,#215259,#215260,#215261,#215262,#215263,#215264,
#215265,#215266,#215267,#215268,#215269,#215270,#215271,#215272,#215273,
#215274,#215275,#215276,#215277,#215278,#215279,#215280,#215281,#215282,
#215283,#215284,#215285,#215286,#215287,#215288,#215289,#215290,#215291,
#215292,#215293,#215294,#215295,#215296,#215297,#215298,#215299,#215300,
#215301,#215302,#215303,#215304,#215305,#215306,#215307,#215308,#215309,
#215310,#215311,#215312,#215313,#215314,#215315,#215316,#215317,#215318,
#215319,#215320,#215321,#215322,#215323,#215324,#215325,#215326,#215327,
#215328,#215329,#215330,#215331,#215332,#215333,#215334,#215335,#215336,
#215337,#215338,#215339,#215340,#215341,#215342,#215343,#215344,#215345,
#215346,#215347,#215348,#215349,#215350,#215351,#215352,#215353,#215354,
#215355,#215356,#215357,#215358,#215359,#215360,#215361,#215362,#215363,
#215364,#215365,#215366,#215367,#215368,#215369,#215370,#215371,#215372,
#215373,#215374,#215375,#215376,#215377,#215378,#215379,#215380,#215381,
#215382,#215383,#215384,#215385,#215386,#215387,#215388,#215389,#215390,
#215391,#215392,#215393,#215394,#215395,#215396,#215397,#215398,#215399,
#215400,#215401,#215402,#215403,#215404,#215405,#215406,#215407,#215408,
#215409,#215410,#215411,#215412,#215413,#215414,#215415,#215416,#215417,
#215418,#215419,#215420,#215421,#215422,#215423,#215424,#215425,#215426,
#215427,#215428,#215429,#215430,#215431,#215432,#215433,#215434,#215435,
#215436,#215437,#215438,#215439,#215440,#215441,#215442,#215443,#215444,
#215445,#215446,#215447,#215448,#215449,#215450,#215451,#215452,#215453,
#215454,#215455,#215456,#215457,#215458,#215459,#215460,#215461,#215462,
#215463,#215464,#215465,#215466,#215467,#215468,#215469,#215470,#215471,
#215472,#215473,#215474,#215475,#215476,#215477,#215478,#215479,#215480,
#215481,#215482,#215483,#215484,#215485,#215486,#215487,#215488,#215489,
#215490,#215491,#215492,#215493,#215494,#215495,#215496,#215497,#215498,
#215499,#215500,#215501,#215502,#215503,#215504,#215505,#215506,#215507,
#215508,#215509,#215510,#215511,#215512,#215513,#215514,#215515,#215516,
#215517,#215518,#215519,#215520,#215521,#215522,#215523,#215524,#215525,
#215526,#215527,#215528,#215529,#215530,#215531,#215532,#215533,#215534,
#215535,#215536,#215537,#215538,#215539,#215540,#215541,#215542,#215543,
#215544,#215545,#215546,#215547,#215548,#215549,#215550,#215551,#215552,
#215553,#215554,#215555,#215556,#215557,#215558,#215559,#215560,#215561,
#215562,#215563,#215564,#215565,#215566,#215567,#215568,#215569,#215570,
#215571,#215572,#215573,#215574,#215575,#215576,#215577,#215578,#215579,
#215580,#215581,#215582,#215583,#215584,#215585,#215586,#215587,#215588,
#215589,#215590,#215591,#215592,#215593,#215594,#215595,#215596,#215597,
#215598,#215599,#215600,#215601,#215602,#215603,#215604,#215605,#215606,
#215607,#215608,#215609,#215610,#215611,#215612,#215613,#215614,#215615,
#215616,#215617,#215618,#215619,#215620,#215621,#215622,#215623,#215624,
#215625,#215626,#215627,#215628,#215629,#215630,#215631,#215632,#215633,
#215634,#215635,#215636,#215637,#215638,#215639,#215640,#215641,#215642,
#215643,#215644,#215645,#215646,#215647,#215648,#215649,#215650,#215651,
#215652,#215653,#215654,#215655,#215656,#215657,#215658,#215659,#215660,
#215661,#215662,#215663,#215664,#215665,#215666,#215667,#215668,#215669,
#215670,#215671,#215672,#215673,#215674,#215675,#215676,#215677,#215678,
#215679,#215680,#215681,#215682,#215683,#215684,#215685,#215686,#215687,
#215688,#215689,#215690,#215691,#215692,#215693,#215694,#215695,#215696,
#215697,#215698,#215699,#215700,#215701,#215702,#215703,#215704,#215705,
#215706,#215707,#215708,#215709,#215710,#215711,#215712,#215713,#215714,
#215715,#215716,#215717,#215718,#215719,#215720,#215721,#215722,#215723,
#215724,#215725,#215726,#215727,#215728,#215729,#215730,#215731,#215732,
#215733,#215734,#215735,#215736,#215737,#215738,#215739,#215740,#215741,
#215742,#215743,#215744,#215745,#215746,#215747,#215748,#215749,#215750,
#215751,#215752,#215753,#215754,#215755,#215756,#215757,#215758,#215759,
#215760,#215761,#215762,#215763,#215764,#215765,#215766,#215767,#215768,
#215769,#215770,#215771,#215772,#215773,#215774,#215775,#215776,#215777,
#215778,#215779,#215780,#215781,#215782,#215783,#215784,#215785,#215786,
#215787,#215788,#215789,#215790,#215791,#215792,#215793,#215794,#215795,
#215796,#215797,#215798,#215799,#215800,#215801,#215802,#215803,#215804,
#215805,#215806,#215807,#215808,#215809,#215810,#215811,#215812,#215813,
#215814,#215815,#215816,#215817,#215818,#215819,#215820,#215821,#215822,
#215823,#215824,#215825,#215826,#215827,#215828,#215829,#215830,#215831,
#215832,#215833,#215834,#215835,#215836,#215837,#215838,#215839,#215840,
#215841,#215842,#215843,#215844,#215845,#215846,#215847,#215848,#215849,
#215850,#215851,#215852,#215853,#215854,#215855,#215856,#215857,#215858,
#215859,#215860,#215861,#215862,#215863,#215864,#215865,#215866,#215867,
#215868,#215869,#215870,#215871,#215872,#215873,#215874,#215875,#215876,
#215877,#215878,#215879,#215880,#215881,#215882,#215883,#215884,#215885,
#215886,#215887,#215888,#215889,#215890,#215891,#215892,#215893,#215894,
#215895,#215896,#215897,#215898,#215899,#215900,#215901,#215902,#215903,
#215904,#215905,#215906,#215907,#215908,#215909,#215910,#215911,#215912,
#215913,#215914,#215915,#215916,#215917,#215918,#215919,#215920,#215921,
#215922,#215923,#215924,#215925,#215926,#215927,#215928,#215929,#215930,
#215931,#215932,#215933,#215934,#215935,#215936,#215937,#215938,#215939,
#215940,#215941,#215942,#215943,#215944,#215945,#215946,#215947,#215948,
#215949,#215950,#215951,#215952,#215953,#215954,#215955,#215956,#215957,
#215958,#215959,#215960,#215961,#215962,#215963,#215964,#215965,#215966,
#215967,#215968,#215969,#215970,#215971,#215972,#215973,#215974,#215975,
#215976,#215977,#215978,#215979,#215980,#215981,#215982,#215983,#215984,
#215985,#215986,#215987,#215988,#215989,#215990,#215991,#215992,#215993,
#215994,#215995,#215996,#215997,#215998,#215999,#216000,#216001,#216002,
#216003,#216004,#216005,#216006,#216007,#216008,#216009,#216010,#216011,
#216012,#216013,#216014,#216015,#216016,#216017,#216018,#216019,#216020,
#216021,#216022,#216023,#216024,#216025,#216026,#216027,#216028,#216029,
#216030,#216031,#216032,#216033,#216034,#216035,#216036,#216037,#216038,
#216039,#216040,#216041,#216042,#216043,#216044,#216045,#216046,#216047,
#216048,#216049,#216050,#216051,#216052,#216053,#216054,#216055,#216056,
#216057,#216058,#216059,#216060,#216061,#216062,#216063,#216064,#216065,
#216066,#216067,#216068,#216069,#216070,#216071,#216072,#216073,#216074,
#216075,#216076,#216077,#216078,#216079,#216080,#216081,#216082,#216083,
#216084,#216085,#216086,#216087,#216088,#216089,#216090,#216091,#216092,
#216093,#216094,#216095,#216096,#216097,#216098,#216099,#216100,#216101,
#216102,#216103,#216104,#216105,#216106,#216107,#216108,#216109,#216110,
#216111,#216112,#216113,#216114,#216115,#216116,#216117,#216118,#216119,
#216120,#216121,#216122,#216123,#216124,#216125,#216126,#216127,#216128,
#216129,#216130,#216131,#216132,#216133,#216134,#216135,#216136,#216137,
#216138,#216139,#216140,#216141,#216142,#216143,#216144,#216145,#216146,
#216147,#216148,#216149,#216150,#216151,#216152,#216153,#216154,#216155,
#216156,#216157,#216158,#216159,#216160,#216161,#216162,#216163,#216164,
#216165,#216166,#216167,#216168,#216169,#216170,#216171,#216172,#216173,
#216174,#216175,#216176,#216177,#216178,#216179,#216180,#216181,#216182,
#216183,#216184,#216185,#216186,#216187,#216188,#216189,#216190,#216191,
#216192,#216193,#216194,#216195,#216196,#216197,#216198,#216199,#216200,
#216201,#216202,#216203,#216204,#216205,#216206,#216207,#216208,#216209,
#216210,#216211,#216212,#216213,#216214,#216215,#216216,#216217,#216218,
#216219,#216220,#216221,#216222,#216223,#216224,#216225,#216226,#216227,
#216228,#216229,#216230,#216231,#216232,#216233,#216234,#216235,#216236,
#216237,#216238,#216239,#216240,#216241,#216242,#216243,#216244,#216245,
#216246,#216247,#216248,#216249,#216250,#216251,#216252,#216253,#216254,
#216255,#216256,#216257,#216258,#216259,#216260,#216261,#216262,#216263,
#216264,#216265,#216266,#216267,#216268,#216269,#216270,#216271,#216272,
#216273,#216274,#216275,#216276,#216277,#216278,#216279,#216280)),
 .UNSPECIFIED.,.F.,.F.,.F.,(4,4),(4,1,1,1,1,1,1,1,1,1,1,1,1,1,1,1,1,1,1,
1,1,1,1,1,1,1,1,1,1,1,1,1,1,1,1,1,1,1,1,1,1,1,1,1,1,1,1,1,1,1,1,1,1,1,1,
1,1,1,1,1,1,1,1,1,1,1,1,1,1,1,1,1,1,1,1,1,1,1,1,1,1,1,1,1,1,1,1,1,1,1,1,
1,1,1,1,1,1,1,1,1,1,1,1,1,1,1,1,1,1,1,1,1,1,1,1,1,1,1,1,1,1,1,1,1,1,1,1,
1,1,1,1,1,1,1,1,1,1,1,1,1,1,1,1,1,1,1,1,1,1,1,1,1,1,1,1,1,1,1,1,1,1,1,1,
1,1,1,1,1,1,1,1,1,1,1,1,1,1,1,1,1,1,1,1,1,1,1,1,1,1,1,1,1,1,1,1,1,1,1,1,
1,1,1,1,1,1,1,1,1,1,1,1,1,1,1,1,1,1,1,1,1,1,1,1,1,1,1,1,1,1,1,1,1,1,1,1,
1,1,1,1,1,1,1,1,1,1,1,1,1,1,1,1,1,1,1,1,1,1,1,1,1,1,1,1,1,1,1,1,1,1,1,1,
1,1,1,1,1,1,1,1,1,1,1,1,1,1,1,1,1,1,1,1,1,1,1,1,1,1,1,1,1,1,1,1,1,1,1,1,
1,1,1,1,1,1,1,1,1,1,1,1,1,1,1,1,1,1,1,1,1,1,1,1,1,1,1,1,1,1,1,1,1,1,1,1,
1,1,1,1,1,1,1,1,1,1,1,1,1,1,1,1,1,1,1,1,1,1,1,1,1,1,1,1,1,1,1,1,1,1,1,1,
1,1,1,1,1,1,1,1,1,1,1,1,1,1,1,1,1,1,1,1,1,1,1,1,1,1,1,1,1,1,1,1,1,1,1,1,
1,1,1,1,1,1,1,1,1,1,1,1,1,1,1,1,1,1,1,1,1,1,1,1,1,1,1,1,1,1,1,1,1,1,1,1,
1,1,1,1,1,1,1,1,1,1,1,1,1,1,1,1,1,1,1,1,1,1,1,1,1,1,1,1,1,1,1,1,1,1,1,1,
1,1,1,1,1,1,1,1,1,1,1,1,1,1,1,1,1,1,1,1,1,1,1,1,1,1,1,1,1,1,1,1,1,1,1,1,
1,1,1,1,1,1,1,1,1,1,1,1,1,1,1,1,1,1,1,1,1,1,1,1,1,1,1,1,1,1,1,1,1,1,1,1,
1,1,1,1,1,1,1,1,1,1,1,1,1,1,1,1,1,1,1,1,1,1,1,1,1,1,1,1,1,1,1,1,1,1,1,1,
1,1,1,1,1,1,1,1,1,1,1,1,1,1,1,1,1,1,1,1,1,1,1,1,1,1,1,1,1,1,1,1,1,1,1,1,
1,1,1,1,1,1,1,1,1,1,1,1,1,1,1,1,1,1,1,1,1,1,1,1,1,1,1,1,1,1,1,1,1,1,1,1,
1,1,1,1,1,1,1,1,1,1,1,1,1,1,1,1,1,1,1,1,1,1,1,1,1,1,1,1,1,1,1,1,1,1,1,1,
1,1,1,1,1,1,1,1,1,1,1,1,1,1,1,1,1,1,1,1,1,1,1,1,1,1,1,1,1,1,1,1,1,1,1,1,
1,1,1,1,1,1,1,1,1,1,1,1,1,1,1,1,1,1,1,1,1,1,1,1,1,1,1,1,1,1,1,1,1,1,1,1,
1,1,1,1,1,1,1,1,1,1,1,1,1,1,1,1,1,1,1,1,1,1,1,1,1,1,1,1,1,1,1,1,1,1,1,1,
1,1,1,1,1,1,1,1,1,1,1,1,1,1,1,1,1,1,1,1,1,1,1,1,1,1,1,1,1,1,1,1,1,1,1,1,
1,1,1,1,1,1,1,1,1,1,1,1,1,1,1,1,1,1,1,1,1,1,1,1,1,1,1,1,1,1,1,1,1,1,1,1,
1,1,1,1,1,1,1,1,1,1,1,1,1,1,1,1,1,1,1,1,1,1,1,1,1,1,1,1,1,1,1,1,1,1,1,1,
1,1,1,1,1,1,1,1,1,1,1,1,1,1,1,1,1,1,1,1,1,1,1,1,1,1,1,1,1,1,1,1,1,1,1,1,
1,1,1,1,1,1,1,1,1,1,1,1,1,1,1,1,1,1,1,1,1,1,1,1,1,1,1,1,1,1,1,1,1,1,1,1,
1,1,1,1,1,1,1,1,1,1,1,1,1,1,1,1,1,1,1,1,1,1,1,1,1,1,1,1,1,1,1,1,1,1,1,1,
1,1,1,1,1,1,1,1,1,1,1,1,1,1,1,1,1,1,1,1,1,1,1,1,1,1,1,1,1,1,1,1,1,1,1,1,
1,1,1,1,1,1,1,1,1,1,1,1,1,1,1,1,1,1,1,1,1,1,1,1,1,1,1,1,1,1,1,1,1,1,1,1,
1,1,1,1,1,1,1,1,1,1,1,1,1,1,1,1,1,1,1,1,1,1,1,1,1,1,1,1,1,1,1,1,1,1,1,1,
1,1,1,1,1,1,1,1,1,1,1,1,1,1,1,1,1,1,1,1,1,1,1,1,1,1,1,1,1,1,1,1,1,1,1,1,
1,1,1,1,1,1,1,1,1,1,1,1,1,1,1,1,1,1,1,1,1,1,1,1,1,1,1,1,1,1,1,1,1,1,1,1,
1,1,1,1,1,1,1,1,1,1,1,1,1,1,1,1,1,1,1,1,1,1,1,1,1,1,1,1,1,1,1,1,1,1,1,1,
1,1,1,1,1,1,1,1,1,1,1,1,1,1,1,1,1,1,1,1,1,1,1,1,1,1,1,1,1,1,1,1,1,1,1,1,
1,1,1,1,1,1,1,1,1,1,1,1,1,1,1,1,1,1,1,1,1,1,1,1,1,1,1,1,1,1,1,1,1,1,1,1,
1,1,1,1,1,1,1,1,1,1,1,1,1,1,1,1,1,1,1,1,1,1,1,1,1,1,1,1,1,1,1,1,1,1,1,1,
1,1,1,1,1,1,1,1,1,1,1,1,1,1,1,1,1,1,1,1,1,1,1,1,1,1,1,1,1,1,1,1,1,1,1,1,
1,1,1,1,1,1,1,1,1,1,1,1,1,1,1,1,1,1,1,1,1,1,1,1,1,1,1,1,1,1,1,1,1,1,1,1,
1,1,1,1,1,1,1,1,1,1,1,1,1,1,1,1,1,1,1,1,1,1,1,1,1,1,1,1,1,1,1,1,1,1,1,1,
1,1,1,1,1,1,1,1,1,1,1,1,1,1,1,1,1,1,1,1,1,1,1,1,1,1,1,1,1,1,1,1,1,1,1,1,
1,1,1,1,1,1,1,1,1,1,1,1,1,1,1,1,1,1,1,1,1,1,1,1,1,1,1,1,1,1,1,1,1,1,1,1,
1,1,1,1,1,1,1,1,1,1,1,1,1,1,1,1,1,1,1,1,1,1,1,1,1,1,1,1,1,1,1,1,1,1,1,1,
1,1,1,1,1,1,1,1,1,1,1,1,1,1,1,1,1,1,1,1,1,1,1,1,1,1,1,1,1,1,1,1,1,1,1,1,
1,1,1,1,1,1,1,1,1,1,1,1,1,1,1,1,1,1,1,1,1,1,1,1,1,1,1,1,1,1,1,1,1,1,1,1,
1,1,1,1,1,1,1,1,1,1,1,1,1,1,1,1,1,1,1,1,1,1,1,1,1,1,1,1,1,1,1,1,1,1,1,1,
1,1,1,1,1,1,1,1,1,1,1,1,1,1,1,1,1,4),(-0.000423095957202541,0.115881565465356),
(11.6153146011728,12.1152895244478,12.6151575298078,13.614893540528,14.6146295512481,
15.6143655619682,16.6141015726884,17.6138375834085,18.6135735941286,19.6133096048488,
20.6130456155689,21.612781626289,22.6125176370092,23.6122536477293,24.6119896584494,
25.6117256691696,26.6114616798897,27.6111976906098,28.6109337013299,29.6106697120501,
30.6104057227702,31.6101417334903,32.6098777442105,33.6096137549306,34.6093497656507,
35.6090857763709,36.608821787091,37.6085577978111,38.6082938085313,39.6080298192514,
40.6077658299715,41.6075018406916,42.6072378514118,43.6069738621319,44.606709872852,
45.6064458835722,46.6061818942923,47.6059179050124,48.6056539157326,49.6053899264527,
50.6051259371728,51.604861947893,52.6045979586131,53.6043339693332,54.6040699800534,
55.6038059907735,56.6035420014936,57.6032780122137,58.6030140229339,59.602750033654,
60.6024860443741,61.6022220550943,62.6019580658144,63.6016940765345,64.6014300872547,
65.6011660979748,66.6009021086949,67.6006381194151,68.6003741301352,69.6001101408553,
70.5998461515754,71.5995821622956,72.5993181730157,73.5990541837358,74.598790194456,
75.5985262051761,76.5982622158962,77.5979982266164,78.5977342373365,79.5974702480566,
80.5972062587768,81.5969422694969,82.596678280217,83.5964142909372,84.5961503016573,
85.5958863123774,86.5956223230975,87.5953583338177,88.5950943445378,89.5948303552579,
90.5945663659781,91.5943023766982,92.5940383874183,93.5937743981385,94.5935104088586,
95.5932464195787,96.5929824302989,97.592718441019,98.5924544517391,99.5921904624593,
100.591926473179,101.5916624839,102.59139849462,103.59113450534,104.59087051606,
105.59060652678,106.5903425375,107.59007854822,108.58981455894,109.589550569661,
110.589286580381,111.589022591101,112.588758601821,113.588494612541,114.588230623261,
115.587966633981,116.587702644701,117.587438655422,118.587174666142,119.586910676862,
120.586646687582,121.586382698302,122.586118709022,123.585854719742,124.585590730463,
125.585326741183,126.585062751903,127.584798762623,128.584534773343,129.584270784063,
130.584006794783,131.583742805503,132.583478816224,133.583214826944,134.582950837664,
135.582686848384,136.582422859104,137.582158869824,138.581894880544,139.581630891264,
140.581366901985,141.581102912705,142.580838923425,143.580574934145,144.580310944865,
145.580046955585,146.579782966305,147.579518977026,148.579254987746,149.578990998466,
150.578727009186,151.578463019906,152.578199030626,153.577935041346,154.577671052066,
155.577407062787,156.577143073507,157.576879084227,158.576615094947,159.576351105667,
160.576087116387,161.575823127107,162.575559137827,163.575295148548,164.575031159268,
165.574767169988,166.574503180708,167.574239191428,168.573975202148,169.573711212868,
170.573447223589,171.573183234309,172.572919245029,173.572655255749,174.572391266469,
175.572127277189,176.571863287909,177.571599298629,178.57133530935,179.57107132007,
180.57080733079,181.57054334151,182.57027935223,183.57001536295,184.56975137367,
185.56948738439,186.569223395111,187.568959405831,188.568695416551,189.568431427271,
190.568167437991,191.567903448711,192.567639459431,193.567375470152,194.567111480872,
195.566847491592,196.566583502312,197.566319513032,198.566055523752,199.565791534472,
200.565527545192,201.565263555913,202.564999566633,203.564735577353,204.564471588073,
205.564207598793,206.563943609513,207.563679620233,208.563415630954,209.563151641674,
210.562887652394,211.562623663114,212.562359673834,213.562095684554,214.561831695274,
215.561567705994,216.561303716715,217.561039727435,218.560775738155,219.560511748875,
220.560247759595,221.559983770315,222.559719781035,223.559455791755,224.559191802476,
225.558927813196,226.558663823916,227.558399834636,228.558135845356,229.557871856076,
230.557607866796,231.557343877517,232.557079888237,233.556815898957,234.556551909677,
235.556287920397,236.556023931117,237.555759941837,238.555495952557,239.555231963278,
240.554967973998,241.554703984718,242.554439995438,243.554176006158,244.553912016878,
245.553648027598,246.553384038319,247.553120049039,248.552856059759,249.552592070479,
250.552328081199,251.552064091919,252.551800102639,253.551536113359,254.55127212408,
255.5510081348,256.55074414552,257.55048015624,258.55021616696,259.54995217768,
260.5496881884,261.54942419912,262.549160209841,263.548896220561,264.548632231281,
265.548368242001,266.548104252721,267.547840263441,268.547576274161,269.547312284882,
270.547048295602,271.546784306322,272.546520317042,273.546256327762,274.545992338482,
275.545728349202,276.545464359922,277.545200370643,278.544936381363,279.544672392083,
280.544408402803,281.544144413523,282.543880424243,283.543616434963,284.543352445683,
285.543088456404,286.542824467124,287.542560477844,288.542296488564,289.542032499284,
290.541768510004,291.541504520724,292.541240531445,293.540976542165,294.540712552885,
295.540448563605,296.540184574325,297.539920585045,298.539656595765,299.539392606485,
300.539128617206,301.538864627926,302.538600638646,303.538336649366,304.538072660086,
305.537808670806,306.537544681526,307.537280692246,308.537016702967,309.536752713687,
310.536488724407,311.536224735127,312.535960745847,313.535696756567,314.535432767287,
315.535168778008,316.534904788728,317.534640799448,318.534376810168,319.534112820888,
320.533848831608,321.533584842328,322.533320853048,323.533056863769,324.532792874489,
325.532528885209,326.532264895929,327.532000906649,328.531736917369,329.531472928089,
330.53120893881,331.53094494953,332.53068096025,333.53041697097,334.53015298169,
335.52988899241,336.52962500313,337.52936101385,338.529097024571,339.528833035291,
340.528569046011,341.528305056731,342.528041067451,343.527777078171,344.527513088891,
345.527249099611,346.526985110332,347.526721121052,348.526457131772,349.526193142492,
350.525929153212,351.525665163932,352.525401174652,353.525137185373,354.524873196093,
355.524609206813,356.524345217533,357.524081228253,358.523817238973,359.523553249693,
360.523289260413,361.523025271134,362.522761281854,363.522497292574,364.522233303294,
365.521969314014,366.521705324734,367.521441335454,368.521177346175,369.520913356895,
370.520649367615,371.520385378335,372.520121389055,373.519857399775,374.519593410495,
375.519329421215,376.519065431936,377.518801442656,378.518537453376,379.518273464096,
380.518009474816,381.517745485536,382.517481496256,383.517217506976,384.516953517697,
385.516689528417,386.516425539137,387.516161549857,388.515897560577,389.515633571297,
390.515369582017,391.515105592737,392.514841603458,393.514577614178,394.514313624898,
395.514049635618,396.513785646338,397.513521657058,398.513257667778,399.512993678499,
400.512729689219,401.512465699939,402.512201710659,403.511937721379,404.511673732099,
405.511409742819,406.511145753539,407.51088176426,408.51061777498,409.5103537857,
410.51008979642,411.50982580714,412.50956181786,413.50929782858,414.509033839301,
415.508769850021,416.508505860741,417.508241871461,418.507977882181,419.507713892901,
420.507449903621,421.507185914341,422.506921925062,423.506657935782,424.506393946502,
425.506129957222,426.505865967942,427.505601978662,428.505337989382,429.505074000102,
430.504810010823,431.504546021543,432.504282032263,433.504018042983,434.503754053703,
435.503490064423,436.503226075143,437.502962085864,438.502698096584,439.502434107304,
440.502170118024,441.501906128744,442.501642139464,443.501378150184,444.501114160904,
445.500850171625,446.500586182345,447.500322193065,448.500058203785,449.499794214505,
450.499530225225,451.499266235945,452.499002246665,453.498738257386,454.498474268106,
455.498210278826,456.497946289546,457.497682300266,458.497418310986,459.497154321706,
460.496890332427,461.496626343147,462.496362353867,463.496098364587,464.495834375307,
465.495570386027,466.495306396747,467.495042407467,468.494778418188,469.494514428908,
470.494250439628,471.493986450348,472.493722461068,473.493458471788,474.493194482508,
475.492930493229,476.492666503949,477.492402514669,478.492138525389,479.491874536109,
480.491610546829,481.491346557549,482.491082568269,483.49081857899,484.49055458971,
485.49029060043,486.49002661115,487.48976262187,488.48949863259,489.48923464331,
490.48897065403,491.488706664751,492.488442675471,493.488178686191,494.487914696911,
495.487650707631,496.487386718351,497.487122729071,498.486858739792,499.486594750512,
500.486330761232,501.486066771952,502.485802782672,503.485538793392,504.485274804112,
505.485010814832,506.484746825553,507.484482836273,508.484218846993,509.483954857713,
510.483690868433,511.483426879153,512.483162889873,513.482898900594,514.482634911314,
515.482370922034,516.482106932754,517.481842943474,518.481578954194,519.481314964914,
520.481050975635,521.480786986355,522.480522997075,523.480259007795,524.479995018515,
525.479731029235,526.479467039955,527.479203050675,528.478939061396,529.478675072116,
530.478411082836,531.478147093556,532.477883104276,533.477619114996,534.477355125716,
535.477091136436,536.476827147157,537.476563157877,538.476299168597,539.476035179317,
540.475771190037,541.475507200757,542.475243211477,543.474979222197,544.474715232918,
545.474451243638,546.474187254358,547.473923265078,548.473659275798,549.473395286518,
550.473131297238,551.472867307958,552.472603318679,553.472339329399,554.472075340119,
555.471811350839,556.471547361559,557.471283372279,558.471019382999,559.47075539372,
560.47049140444,561.47022741516,562.46996342588,563.4696994366,564.46943544732,
565.46917145804,566.46890746876,567.468643479481,568.468379490201,569.468115500921,
570.467851511641,571.467587522361,572.467323533081,573.467059543801,574.466795554521,
575.466531565242,576.466267575962,577.466003586682,578.465739597402,579.465475608122,
580.465211618842,581.464947629562,582.464683640283,583.464419651003,584.464155661723,
585.463891672443,586.463627683163,587.463363693883,588.463099704603,589.462835715323,
590.462571726044,591.462307736764,592.462043747484,593.461779758204,594.461515768924,
595.461251779644,596.460987790364,597.460723801085,598.460459811805,599.460195822525,
600.459931833245,601.459667843965,602.459403854685,603.459139865405,604.458875876125,
605.458611886846,606.458347897566,607.458083908286,608.457819919006,609.457555929726,
610.457291940446,611.457027951166,612.456763961887,613.456499972607,614.456235983327,
615.455971994047,616.455708004767,617.455444015487,618.455180026207,619.454916036927,
620.454652047648,621.454388058368,622.454124069088,623.453860079808,624.453596090528,
625.453332101248,626.453068111968,627.452804122688,628.452540133409,629.452276144129,
630.452012154849,631.451748165569,632.451484176289,633.451220187009,634.450956197729,
635.450692208449,636.45042821917,637.45016422989,638.44990024061,639.44963625133,
640.44937226205,641.44910827277,642.44884428349,643.448580294211,644.448316304931,
645.448052315651,646.447788326371,647.447524337091,648.447260347811,649.446996358531,
650.446732369251,651.446468379972,652.446204390692,653.445940401412,654.445676412132,
655.445412422852,656.445148433572,657.444884444292,658.444620455012,659.444356465733,
660.444092476453,661.443828487173,662.443564497893,663.443300508613,664.443036519333,
665.442772530053,666.442508540774,667.442244551494,668.441980562214,669.441716572934,
670.441452583654,671.441188594374,672.440924605094,673.440660615815,674.440396626535,
675.440132637255,676.439868647975,677.439604658695,678.439340669415,679.439076680135,
680.438812690855,681.438548701576,682.438284712296,683.438020723016,684.437756733736,
685.437492744456,686.437228755176,687.436964765896,688.436700776616,689.436436787337,
690.436172798057,691.435908808777,692.435644819497,693.435380830217,694.435116840937,
695.434852851657,696.434588862377,697.434324873098,698.434060883818,699.433796894538,
700.433532905258,701.433268915978,702.433004926698,703.432740937418,704.432476948139,
705.432212958859,706.431948969579,707.431684980299,708.431420991019,709.431157001739,
710.430893012459,711.430629023179,712.4303650339,713.43010104462,714.42983705534,
715.42957306606,716.42930907678,717.4290450875,718.42878109822,719.42851710894,
720.428253119661,721.427989130381,722.427725141101,723.427461151821,724.427197162541,
725.426933173261,726.426669183981,727.426405194702,728.426141205422,729.425877216142,
730.425613226862,731.425349237582,732.425085248302,733.424821259022,734.424557269742,
735.424293280463,736.424029291183,737.423765301903,738.423501312623,739.423237323343,
740.422973334063,741.422709344783,742.422445355504,743.422181366224,744.421917376944,
745.421653387664,746.421389398384,747.421125409104,748.420861419824,749.420597430544,
750.420333441265,751.420069451985,752.419805462705,753.419541473425,754.419277484145,
755.419013494865,756.418749505585,757.418485516306,758.418221527026,759.417957537746,
760.417693548466,761.417429559186,762.417165569906,763.416901580626,764.416637591346,
765.416373602067,766.416109612787,767.415845623507,768.415581634227,769.415317644947,
770.415053655667,771.414789666387,772.414525677107,773.414261687828,774.413997698548,
775.413733709268,776.413469719988,777.413205730708,778.412941741428,779.412677752148,
780.412413762868,781.412149773589,782.411885784309,783.411621795029,784.411357805749,
785.411093816469,786.410829827189,787.410565837909,788.41030184863,789.41003785935,
790.40977387007,791.40950988079,792.40924589151,793.40898190223,794.40871791295,
795.40845392367,796.408189934391,797.407925945111,798.407661955831,799.407397966551,
800.407133977271,801.406869987991,802.406605998711,803.406342009432,804.406078020152,
805.405814030872,806.405550041592,807.405286052312,808.405022063032,809.404758073752,
810.404494084472,811.404230095193,812.403966105913,813.403702116633,814.403438127353,
815.403174138073,816.402910148793,817.402646159513,818.402382170234,819.402118180954,
820.401854191674,821.401590202394,822.401326213114,823.401062223834,824.400798234554,
825.400534245274,826.400270255995,827.400006266715,828.399742277435,829.399478288155,
830.399214298875,831.398950309595,832.398686320315,833.398422331035,834.398158341756,
835.397894352476,836.397630363196,837.397366373916,838.397102384636,839.396838395356,
840.396574406076,841.396310416796,842.396046427517,843.395782438237,844.395518448957,
845.395254459677,846.394990470397,847.394726481117,848.394462491837,849.394198502558,
850.393934513278,851.393670523998,852.393406534718,853.393142545438,854.392878556158,
855.392614566878,856.392350577598,857.392086588319,858.391822599039,859.391558609759,
860.391294620479,861.391030631199,862.390766641919,863.390502652639,864.390238663359,
865.38997467408,866.3897106848,867.38944669552,868.38918270624,869.38891871696,
870.38865472768,871.3883907384,872.388126749121,873.387862759841,874.387598770561,
875.387334781281,876.387070792001,877.386806802721,878.386542813441,879.386278824161,
880.386014834882,881.385750845602,882.385486856322,883.385222867042,884.384958877762,
885.384694888482,886.384430899202,887.384166909923,888.383902920643,889.383638931363,
890.383374942083,891.383110952803,892.382846963523,893.382582974243,894.382318984963,
895.382054995684,896.381791006404,897.381527017124,898.381263027844,899.380999038564,
900.380735049284,901.380471060004,902.380207070725,903.379943081445,904.379679092165,
905.379415102885,906.379151113605,907.378887124325,908.378623135045,909.378359145765,
910.378095156486,911.377831167206,912.377567177926,913.377303188646,914.377039199366,
915.376775210086,916.376511220806,917.376247231526,918.375983242247,919.375719252967,
920.375455263687,921.375191274407,922.374927285127,923.374663295847,924.374399306567,
925.374135317287,926.373871328008,927.373607338728,928.373343349448,929.373079360168,
930.372815370888,931.372551381608,932.372287392328,933.372023403049,934.371759413769,
935.371495424489,936.371231435209,937.370967445929,938.370703456649,939.370439467369,
940.370175478089,941.36991148881,942.36964749953,943.36938351025,944.36911952097,
945.36885553169,946.36859154241,947.36832755313,948.368063563851,949.367799574571,
950.367535585291,951.367271596011,952.367007606731,953.366743617451,954.366479628171,
955.366215638891,956.365951649612,957.365687660332,958.365423671052,959.365159681772,
960.364895692492,961.364631703212,962.364367713932,963.364103724653,964.363839735373,
965.363575746093,966.363311756813,967.363047767533,968.362783778253,969.362519788973,
970.362255799693,971.361991810414,972.361727821134,973.361463831854,974.361199842574,
975.360935853294,976.360671864014,977.360407874734,978.360143885454,979.359879896175,
980.359615906895,981.359351917615,982.359087928335,983.358823939055,984.358559949775,
985.358295960495,986.358031971215,987.357767981936,988.357503992656,989.357240003376,
990.356976014096,991.356712024816,992.356448035536,993.356184046256,994.355920056977,
995.355656067697,996.355392078417,997.355128089137,998.354864099857,999.354600110577,
1000.3543361213,1001.35407213202,1002.35380814274,1003.35354415346,1004.35328016418,
1005.3530161749,1006.35275218562,1007.35248819634,1008.35222420706,1009.35196021778,
1010.3516962285,1011.35143223922,1012.35116824994,1013.35090426066,1014.35064027138,
1015.3503762821,1016.35011229282,1017.34984830354,1018.34958431426,1019.34932032498,
1020.3490563357,1021.34879234642,1022.34852835714,1023.34826436786,1024.34800037858,
1025.3477363893,1026.34747240002,1027.34720841074,1028.34694442146,1029.34668043218,
1030.3464164429,1031.34615245362,1032.34588846434,1033.34562447506,1034.34536048578,
1035.3450964965,1036.34483250722,1037.34456851794,1038.34430452866,1039.34404053938,
1040.3437765501,1041.34351256082,1042.34324857154,1043.34298458226,1044.34272059298,
1045.3424566037,1046.34219261442,1047.34192862514,1048.34166463586,1049.34140064658,
1050.3411366573,1051.34087266802,1052.34060867874,1053.34034468946,1054.34008070018,
1055.3398167109,1056.33955272162,1057.33928873234,1058.33902474307,1059.33876075378,
1060.33849676451,1061.33823277523,1062.33796878595,1063.33770479667,1064.33744080739,
1065.33717681811,1066.33691282883,1067.33664883955,1068.33638485027,1069.33612086099,
1070.33585687171,1071.33559288243,1072.33532889315,1073.33506490387,1074.33480091459,
1075.33453692531,1076.33427293603,1077.33400894675,1078.33374495747,1079.33348096819,
1080.33321697891,1081.33295298963,1082.33268900035,1083.33242501107,1084.33216102179,
1085.33189703251,1086.33163304323,1087.33136905395,1088.33110506467,1089.33084107539,
1090.33057708611,1091.33031309683,1092.33004910755,1093.32978511827,1094.32952112899,
1095.32925713971,1096.32899315043,1097.32872916115,1098.32846517187,1099.32820118259,
1100.32793719331,1101.32767320403,1102.32740921475,1103.32714522547,1104.32688123619,
1105.32661724691,1106.32635325763,1107.32608926835,1108.32582527907,1109.32556128979,
1110.32529730051,1111.32503331123,1112.32476932195,1113.32450533267,1114.32424134339,
1115.32397735411,1116.32371336483,1117.32344937555,1118.32318538627,1119.32292139699,
1120.32265740771,1121.32239341843,1122.32212942915,1123.32186543987,1124.32160145059,
1125.32133746131,1126.32107347203,1127.32080948275,1128.32054549347,1129.32028150419,
1130.32001751491,1131.31975352563,1132.31948953635,1133.31922554707,1134.31896155779,
1135.31869756852,1136.31843357924,1137.31816958996,1138.31790560068,1139.3176416114,
1140.31737762212,1141.31711363284,1142.31684964356,1143.31658565428,1144.316321665,
1145.31605767572,1146.31579368644,1147.31552969716,1148.31526570788,1149.3150017186,
1150.31473772932,1151.31447374004,1152.31420975076,1153.31394576148,1154.3136817722,
1155.31341778292,1156.31315379364,1157.31288980436,1158.31262581508,1159.3123618258,
1160.31209783652,1161.31183384724,1162.31156985796,1163.31130586868,1164.3110418794,
1165.31077789012,1166.31051390084,1167.31024991156,1168.30998592228,1169.309721933,
1170.30945794372,1171.30919395444,1172.30892996516,1173.30866597588,1174.3084019866,
1175.30813799732,1176.30787400804,1177.30761001876,1178.30734602948,1179.3070820402,
1180.30681805092,1181.30655406164,1182.30629007236,1183.30602608308,1184.3057620938,
1185.30549810452,1186.30523411524,1187.30497012596,1188.30470613668,1189.3044421474,
1190.30417815812,1191.30391416884,1192.30365017956,1193.30338619028,1194.303122201,
1195.30285821172,1196.30259422244,1197.30233023316,1198.30206624388,1199.3018022546,
1200.30153826532,1201.30127427604,1202.30101028676,1203.30074629748,1204.3004823082,
1205.30021831892,1206.29995432964,1207.29969034036,1208.29942635108,1209.2991623618,
1210.29889837252,1211.29863438324,1212.29837039397,1213.29810640469,1214.29784241541,
1215.29757842613,1216.29731443685,1217.29705044757,1218.29678645829,1219.29652246901,
1220.29625847973,1221.29599449045,1222.29573050117,1223.29546651189,1224.29520252261,
1225.29493853333,1226.29467454405,1227.29441055477,1228.29414656549,1229.29388257621,
1230.29361858693,1231.29335459765,1232.29309060837,1233.29282661909,1234.29256262981,
1235.29229864053,1236.29203465125,1237.29177066197,1238.29150667269,1239.29124268341,
1240.29097869413,1241.29071470485,1242.29045071557,1243.29018672629,1244.28992273701,
1245.28965874773,1246.28939475845,1247.28913076917,1248.28886677989,1249.28860279061,
1250.28833880133,1251.28807481205,1252.28781082277,1253.28754683349,1254.28728284421,
1255.28701885493,1256.28675486565,1257.28649087637,1258.28622688709,1259.28596289781,
1260.28569890853,1261.28543491925,1262.28517092997,1263.28490694069,1264.28464295141,
1265.28437896213,1266.28411497285,1267.28385098357,1268.28358699429,1269.28332300501,
1270.28305901573,1271.28279502645,1272.28253103717,1273.28226704789,1274.28200305861,
1275.28173906933,1276.28147508005,1277.28121109077,1278.28094710149,1279.28068311221,
1280.28041912293,1281.28015513365,1282.27989114437,1283.27962715509,1284.27936316581,
1285.27909917653,1286.27883518725,1287.27857119797,1288.2783072087,1289.27804321942,
1290.27777923014,1291.27751524086,1292.27725125158,1293.2769872623,1294.27672327302,
1295.27645928374,1296.27619529446,1297.27593130518,1298.2756673159,1299.27540332662,
1300.27513933734,1301.27487534806,1302.27461135878,1303.2743473695,1304.27408338022,
1305.27381939094,1306.27355540166,1307.27329141238,1308.2730274231,1309.27276343382,
1310.27249944454,1311.27223545526,1312.27197146598,1313.2717074767,1314.27144348742,
1315.27117949814,1316.27091550886,1317.27065151958,1318.2703875303,1319.27012354102,
1320.26985955174,1321.26959556246,1322.26933157318,1323.2690675839,1324.26880359462,
1325.26853960534,1326.26827561606,1327.26801162678,1328.2677476375,1329.26748364822,
1330.26721965894,1331.26695566966,1332.26669168038,1333.2664276911,1334.26616370182,
1335.26589971254,1336.26563572326,1337.26537173398,1338.2651077447,1339.26484375542,
1340.26457976614,1341.26431577686,1342.26405178758,1343.2637877983,1344.26352380902,
1345.26325981974,1346.26299583046,1347.26273184118,1348.2624678519,1349.26220386262,
1350.26193987334,1351.26167588406,1352.26141189478,1353.2611479055,1354.26088391622,
1355.26061992694,1356.26035593766,1357.26009194838,1358.2598279591,1359.25956396982,
1360.25929998054,1361.25903599126,1362.25877200198,1363.2585080127,1364.25824402343,
1365.25798003415,1366.25771604487,1367.25745205559,1368.25718806631,1369.25692407703,
1370.25666008775,1371.25639609847,1372.25613210919,1373.25586811991,1374.25560413063,
1375.25534014135,1376.25507615207,1377.25481216279,1378.25454817351,1379.25428418423,
1380.25402019495,1381.25375620567,1382.25349221639,1383.25322822711,1384.25296423783,
1385.25270024855,1386.25243625927,1387.25217226999,1388.25190828071,1389.25164429143,
1390.25138030215,1391.25111631287,1392.25085232359,1393.25058833431,1394.25032434503,
1395.25006035575,1396.24979636647,1397.24953237719,1398.24926838791,1399.24900439863,
1400.24874040935,1401.24847642007,1402.24821243079,1403.24794844151,1404.24768445223,
1405.24742046295,1406.24715647367,1407.24689248439,1408.24662849511,1409.24636450583,
1410.24610051655,1411.24583652727,1412.24557253799,1413.24530854871,1414.24504455943,
1415.24478057015,1416.24451658087,1417.24425259159,1418.24398860231,1419.24372461303,
1420.24346062375,1421.24319663447,1422.24293264519,1423.24266865591,1424.24240466663,
1425.24214067735,1426.24187668807,1427.24161269879,1428.24134870951,1429.24108472023,
1430.24082073095,1431.24055674167,1432.24029275239,1433.24002876311,1434.23976477383,
1435.23950078455,1436.23923679527,1437.23897280599,1438.23870881671,1439.23844482743,
1440.23818083815,1441.23791684888,1442.2376528596,1443.23738887032,1444.23712488104,
1445.23686089176,1446.23659690248,1447.2363329132,1448.23606892392,1449.23580493464,
1450.23554094536,1451.23527695608,1452.2350129668,1453.23474897752,1454.23448498824,
1455.23422099896,1456.23395700968,1457.2336930204,1458.23342903112,1459.23316504184,
1460.23290105256,1461.23263706328,1462.232373074,1463.23210908472,1464.23184509544,
1465.23158110616,1466.23131711688,1467.2310531276,1468.23078913832,1469.23052514904,
1470.23026115976,1471.22999717048,1472.2297331812,1473.22946919192,1474.22920520264,
1475.22894121336,1476.22867722408,1477.2284132348,1478.22814924552,1479.22788525624,
1480.22762126696,1481.22735727768,1482.2270932884,1483.22682929912,1484.22656530984,
1485.22630132056,1486.22603733128,1487.225773342,1488.22550935272,1489.22524536344,
1490.22498137416,1491.22471738488,1492.2244533956,1493.22418940632,1494.22392541704,
1495.22366142776,1496.22339743848,1497.2231334492,1498.22286945992,1499.22260547064,
1500.22234148136,1501.22207749208,1502.2218135028,1503.22154951352,1504.22128552424,
1505.22102153496,1506.22075754568,1507.2204935564,1508.22022956712,1509.21996557784,
1510.21970158856,1511.21943759928,1512.21917361,1513.21890962072,1514.21864563144,
1515.21838164216,1516.21811765288,1517.21785366361,1518.21758967433,1519.21732568505,
1520.21706169577,1521.21679770649,1522.21653371721,1523.21626972793,1524.21600573865,
1525.21574174937,1526.21547776009,1527.21521377081,1528.21494978153,1529.21468579225,
1530.21442180297,1531.21415781369,1532.21389382441,1533.21362983513,1534.21336584585,
1535.21310185657,1536.21283786729,1537.21257387801,1538.21230988873,1539.21204589945,
1540.21178191017,1541.21151792089,1542.21125393161,1543.21098994233,1544.21072595305,
1545.21046196377,1546.21019797449,1547.20993398521,1548.20966999593,1549.20940600665,
1550.20914201737,1551.20887802809,1552.20861403881,1553.20835004953,1554.20808606025,
1555.20782207097,1556.20755808169,1557.20729409241,1558.20703010313,1559.20676611385,
1560.20650212457,1561.20623813529,1562.20597414601,1563.20571015673,1564.20544616745,
1565.20518217817,1566.20491818889,1567.20465419961,1568.20439021033,1569.20412622105,
1570.20386223177,1571.20359824249,1572.20333425321,1573.20307026393,1574.20280627465,
1575.20254228537,1576.20227829609,1577.20201430681,1578.20175031753,1579.20148632825,
1580.20122233897,1581.20095834969,1582.20069436041,1583.20043037113,1584.20016638185,
1585.19990239257,1586.19963840329,1587.19937441401,1588.19911042473,1589.19884643545,
1590.19858244617,1591.19831845689,1592.19805446761,1593.19779047834,1594.19752648906,
1595.19726249978,1596.1969985105,1597.19673452122,1598.19647053194,1599.19620654266,
1600.19594255338,1601.1956785641,1602.19541457482,1603.19515058554,1604.19488659626,
1605.19462260698,1606.1943586177,1607.19409462842,1608.19383063914,1609.19356664986,
1610.19330266058,1611.1930386713,1612.19277468202,1613.19251069274,1614.19224670346,
1615.19198271418,1616.1917187249,1617.19145473562,1618.19119074634,1619.19092675706,
1620.19066276778,1621.1903987785,1622.19013478922,1623.18987079994,1624.18960681066,
1625.18934282138,1626.1890788321,1627.18881484282,1628.18855085354,1629.18828686426,
1630.18802287498,1631.1877588857,1632.18749489642,1633.18723090714,1634.18696691786,
1635.18670292858,1636.1864389393,1637.18617495002,1638.18591096074,1639.18564697146,
1640.18538298218,1641.1851189929,1642.18485500362,1643.18459101434,1644.18432702506,
1645.18406303578,1646.1837990465,1647.18353505722,1648.18327106794,1649.18300707866,
1650.18274308938,1651.1824791001,1652.18221511082,1653.18195112154,1654.18168713226,
1655.18142314298,1656.1811591537,1657.18089516442,1658.18063117514,1659.18036718586,
1660.18010319658,1661.1798392073,1662.17957521802,1663.17931122874,1664.17904723946,
1665.17878325018,1666.1785192609,1667.17825527162,1668.17799128234,1669.17772729307,
1670.17746330379,1671.17719931451,1672.17693532523,1673.17667133595,1674.17640734667,
1675.17614335739,1676.17587936811,1677.17561537883,1678.17535138955,1679.17508740027,
1680.17482341099,1681.17455942171,1682.17429543243,1683.17403144315,1684.17376745387,
1685.17350346459,1686.17323947531,1687.17297548603,1688.17271149675,1689.17244750747,
1690.17218351819,1691.17191952891,1692.17165553963,1693.17139155035,1694.17112756107,
1695.17086357179,1696.17059958251,1697.17033559323,1698.17007160395,1699.16980761467,
1700.16954362539,1700.66941163075,1701.16959429301),.UNSPECIFIED.);
#50=B_SPLINE_SURFACE_WITH_KNOTS('',3,3,((#218357,#218358,#218359,#218360,
#218361,#218362,#218363,#218364,#218365,#218366,#218367,#218368,#218369,
#218370,#218371,#218372,#218373,#218374,#218375,#218376,#218377,#218378,
#218379,#218380,#218381,#218382,#218383,#218384,#218385,#218386,#218387,
#218388,#218389,#218390,#218391,#218392,#218393,#218394,#218395,#218396,
#218397,#218398,#218399,#218400,#218401,#218402,#218403,#218404,#218405,
#218406,#218407,#218408,#218409,#218410,#218411,#218412,#218413,#218414,
#218415,#218416,#218417,#218418,#218419,#218420,#218421,#218422,#218423,
#218424,#218425,#218426,#218427,#218428,#218429,#218430,#218431,#218432,
#218433,#218434,#218435,#218436,#218437,#218438,#218439,#218440,#218441,
#218442,#218443,#218444,#218445,#218446,#218447,#218448,#218449,#218450,
#218451,#218452,#218453,#218454,#218455,#218456,#218457,#218458,#218459,
#218460,#218461,#218462,#218463,#218464,#218465,#218466,#218467,#218468,
#218469,#218470,#218471,#218472,#218473,#218474,#218475,#218476,#218477,
#218478,#218479,#218480,#218481,#218482,#218483,#218484,#218485,#218486,
#218487,#218488,#218489,#218490,#218491,#218492,#218493,#218494,#218495,
#218496,#218497,#218498,#218499,#218500,#218501,#218502,#218503,#218504,
#218505,#218506,#218507,#218508,#218509,#218510,#218511,#218512,#218513,
#218514,#218515,#218516,#218517,#218518,#218519,#218520,#218521,#218522,
#218523,#218524,#218525,#218526,#218527,#218528,#218529,#218530,#218531,
#218532,#218533,#218534,#218535,#218536,#218537,#218538,#218539,#218540,
#218541,#218542,#218543,#218544,#218545,#218546,#218547,#218548,#218549,
#218550,#218551,#218552,#218553,#218554,#218555,#218556,#218557,#218558,
#218559,#218560,#218561,#218562,#218563,#218564,#218565,#218566,#218567,
#218568,#218569,#218570,#218571,#218572,#218573,#218574,#218575,#218576,
#218577,#218578,#218579,#218580,#218581,#218582,#218583,#218584,#218585,
#218586,#218587,#218588,#218589,#218590,#218591,#218592,#218593,#218594,
#218595,#218596,#218597,#218598,#218599,#218600,#218601,#218602,#218603,
#218604,#218605,#218606,#218607,#218608,#218609,#218610,#218611,#218612,
#218613,#218614,#218615,#218616,#218617,#218618,#218619,#218620,#218621,
#218622,#218623,#218624,#218625,#218626,#218627,#218628,#218629,#218630,
#218631,#218632,#218633,#218634,#218635,#218636,#218637,#218638,#218639,
#218640,#218641,#218642,#218643,#218644,#218645,#218646,#218647,#218648,
#218649,#218650,#218651,#218652,#218653,#218654,#218655,#218656,#218657,
#218658,#218659,#218660,#218661,#218662,#218663,#218664,#218665,#218666,
#218667,#218668,#218669,#218670,#218671,#218672,#218673,#218674,#218675,
#218676,#218677,#218678,#218679,#218680,#218681,#218682,#218683,#218684,
#218685,#218686,#218687,#218688,#218689,#218690,#218691,#218692,#218693,
#218694,#218695,#218696,#218697,#218698,#218699,#218700,#218701,#218702,
#218703,#218704,#218705,#218706,#218707,#218708,#218709,#218710,#218711,
#218712,#218713,#218714,#218715,#218716,#218717,#218718,#218719,#218720,
#218721,#218722,#218723,#218724,#218725,#218726,#218727,#218728,#218729,
#218730,#218731,#218732,#218733,#218734,#218735,#218736,#218737,#218738,
#218739,#218740,#218741,#218742,#218743,#218744,#218745,#218746,#218747,
#218748,#218749,#218750,#218751,#218752,#218753,#218754,#218755,#218756,
#218757,#218758,#218759,#218760,#218761,#218762,#218763,#218764,#218765,
#218766,#218767,#218768,#218769,#218770,#218771,#218772,#218773,#218774,
#218775,#218776,#218777,#218778,#218779,#218780,#218781,#218782,#218783,
#218784,#218785,#218786,#218787,#218788,#218789,#218790,#218791,#218792,
#218793,#218794,#218795,#218796,#218797,#218798,#218799,#218800,#218801,
#218802,#218803,#218804,#218805,#218806,#218807,#218808,#218809,#218810,
#218811,#218812,#218813,#218814,#218815,#218816,#218817,#218818,#218819,
#218820,#218821,#218822,#218823,#218824,#218825,#218826,#218827,#218828,
#218829,#218830,#218831,#218832,#218833,#218834,#218835,#218836,#218837,
#218838,#218839,#218840,#218841,#218842,#218843,#218844,#218845,#218846,
#218847,#218848,#218849,#218850,#218851,#218852,#218853,#218854,#218855,
#218856,#218857,#218858,#218859,#218860,#218861,#218862,#218863,#218864,
#218865,#218866,#218867,#218868,#218869,#218870,#218871,#218872,#218873,
#218874,#218875,#218876,#218877,#218878,#218879,#218880,#218881,#218882,
#218883,#218884,#218885,#218886,#218887,#218888,#218889,#218890,#218891,
#218892,#218893,#218894,#218895,#218896,#218897,#218898,#218899,#218900,
#218901,#218902,#218903,#218904,#218905,#218906,#218907,#218908,#218909,
#218910,#218911,#218912,#218913,#218914,#218915,#218916,#218917,#218918,
#218919,#218920,#218921,#218922,#218923,#218924,#218925,#218926,#218927,
#218928,#218929,#218930,#218931,#218932,#218933,#218934,#218935,#218936,
#218937,#218938,#218939,#218940,#218941,#218942,#218943,#218944,#218945,
#218946,#218947,#218948,#218949,#218950,#218951,#218952,#218953,#218954,
#218955,#218956,#218957,#218958,#218959,#218960,#218961,#218962,#218963,
#218964,#218965,#218966,#218967,#218968,#218969,#218970,#218971,#218972,
#218973,#218974,#218975,#218976,#218977,#218978,#218979,#218980,#218981,
#218982,#218983,#218984,#218985,#218986,#218987,#218988,#218989,#218990,
#218991,#218992,#218993,#218994,#218995,#218996,#218997,#218998,#218999,
#219000,#219001,#219002,#219003,#219004,#219005,#219006,#219007,#219008,
#219009,#219010,#219011,#219012,#219013,#219014,#219015,#219016,#219017,
#219018,#219019,#219020,#219021,#219022,#219023,#219024,#219025,#219026,
#219027,#219028,#219029,#219030,#219031,#219032,#219033,#219034,#219035,
#219036,#219037,#219038,#219039,#219040,#219041,#219042,#219043,#219044,
#219045,#219046,#219047,#219048,#219049,#219050,#219051,#219052,#219053,
#219054,#219055,#219056,#219057,#219058,#219059,#219060,#219061,#219062,
#219063,#219064,#219065,#219066,#219067,#219068,#219069,#219070,#219071,
#219072,#219073,#219074,#219075,#219076,#219077,#219078,#219079,#219080,
#219081,#219082,#219083,#219084,#219085,#219086,#219087,#219088,#219089,
#219090,#219091,#219092,#219093,#219094,#219095,#219096,#219097,#219098,
#219099,#219100,#219101,#219102,#219103,#219104,#219105,#219106,#219107,
#219108,#219109,#219110,#219111,#219112,#219113,#219114,#219115,#219116,
#219117,#219118,#219119,#219120,#219121,#219122,#219123,#219124,#219125,
#219126,#219127,#219128,#219129,#219130,#219131,#219132,#219133,#219134,
#219135,#219136,#219137,#219138,#219139,#219140,#219141,#219142,#219143,
#219144,#219145,#219146,#219147,#219148,#219149,#219150,#219151,#219152,
#219153,#219154,#219155,#219156,#219157,#219158,#219159,#219160,#219161,
#219162,#219163,#219164,#219165,#219166,#219167,#219168,#219169,#219170,
#219171,#219172,#219173,#219174,#219175,#219176,#219177,#219178,#219179,
#219180,#219181,#219182,#219183,#219184,#219185,#219186,#219187,#219188,
#219189,#219190,#219191,#219192,#219193,#219194,#219195,#219196,#219197,
#219198,#219199,#219200,#219201,#219202,#219203,#219204,#219205,#219206,
#219207,#219208,#219209,#219210,#219211,#219212,#219213,#219214,#219215,
#219216,#219217,#219218,#219219,#219220,#219221,#219222,#219223,#219224,
#219225,#219226,#219227,#219228,#219229,#219230,#219231,#219232,#219233,
#219234,#219235,#219236,#219237,#219238,#219239,#219240,#219241,#219242,
#219243,#219244,#219245,#219246,#219247,#219248,#219249,#219250,#219251,
#219252,#219253,#219254,#219255,#219256,#219257,#219258,#219259,#219260,
#219261,#219262,#219263,#219264,#219265,#219266,#219267,#219268,#219269,
#219270,#219271,#219272,#219273,#219274,#219275,#219276,#219277,#219278,
#219279,#219280,#219281,#219282,#219283,#219284,#219285,#219286,#219287,
#219288,#219289,#219290,#219291,#219292,#219293,#219294,#219295,#219296,
#219297,#219298,#219299,#219300,#219301,#219302,#219303,#219304,#219305,
#219306,#219307,#219308,#219309,#219310,#219311,#219312,#219313,#219314,
#219315,#219316,#219317,#219318,#219319,#219320,#219321,#219322,#219323,
#219324,#219325,#219326,#219327,#219328,#219329,#219330,#219331,#219332,
#219333,#219334,#219335,#219336,#219337,#219338,#219339,#219340,#219341,
#219342,#219343,#219344,#219345,#219346,#219347,#219348,#219349,#219350,
#219351,#219352,#219353,#219354,#219355,#219356,#219357,#219358,#219359,
#219360,#219361,#219362,#219363,#219364,#219365,#219366,#219367,#219368,
#219369,#219370,#219371,#219372,#219373,#219374,#219375,#219376,#219377,
#219378,#219379,#219380,#219381,#219382,#219383,#219384,#219385,#219386,
#219387,#219388,#219389,#219390,#219391,#219392,#219393,#219394,#219395,
#219396,#219397,#219398,#219399,#219400,#219401,#219402,#219403,#219404,
#219405,#219406,#219407,#219408,#219409,#219410,#219411,#219412,#219413,
#219414,#219415,#219416,#219417,#219418,#219419,#219420,#219421,#219422,
#219423,#219424,#219425,#219426,#219427,#219428,#219429,#219430,#219431,
#219432,#219433,#219434,#219435,#219436,#219437,#219438,#219439,#219440,
#219441,#219442,#219443,#219444,#219445,#219446,#219447,#219448,#219449,
#219450,#219451,#219452,#219453,#219454,#219455,#219456,#219457,#219458,
#219459,#219460,#219461,#219462,#219463,#219464,#219465,#219466,#219467,
#219468,#219469,#219470,#219471,#219472,#219473,#219474,#219475,#219476,
#219477,#219478,#219479,#219480,#219481,#219482,#219483,#219484,#219485,
#219486,#219487,#219488,#219489,#219490,#219491,#219492,#219493,#219494,
#219495,#219496,#219497,#219498,#219499,#219500,#219501,#219502,#219503,
#219504,#219505,#219506,#219507,#219508,#219509,#219510,#219511,#219512,
#219513,#219514,#219515,#219516,#219517,#219518,#219519,#219520,#219521,
#219522,#219523,#219524,#219525,#219526,#219527,#219528,#219529,#219530,
#219531,#219532,#219533,#219534,#219535,#219536,#219537,#219538,#219539,
#219540,#219541,#219542,#219543,#219544,#219545,#219546,#219547,#219548,
#219549,#219550,#219551,#219552,#219553,#219554,#219555,#219556,#219557,
#219558,#219559,#219560,#219561,#219562,#219563,#219564,#219565,#219566,
#219567,#219568,#219569,#219570,#219571,#219572,#219573,#219574,#219575,
#219576,#219577,#219578,#219579,#219580,#219581,#219582,#219583,#219584,
#219585,#219586,#219587,#219588,#219589,#219590,#219591,#219592,#219593,
#219594,#219595,#219596,#219597,#219598,#219599,#219600,#219601,#219602,
#219603,#219604,#219605,#219606,#219607,#219608,#219609,#219610,#219611,
#219612,#219613,#219614,#219615,#219616,#219617,#219618,#219619,#219620,
#219621,#219622,#219623,#219624,#219625,#219626,#219627,#219628,#219629,
#219630,#219631,#219632,#219633,#219634,#219635,#219636,#219637,#219638,
#219639,#219640,#219641,#219642,#219643,#219644,#219645,#219646,#219647,
#219648,#219649,#219650,#219651,#219652,#219653,#219654,#219655,#219656,
#219657,#219658,#219659,#219660,#219661,#219662,#219663,#219664,#219665,
#219666,#219667,#219668,#219669,#219670,#219671,#219672,#219673,#219674,
#219675,#219676,#219677,#219678,#219679,#219680,#219681,#219682,#219683,
#219684,#219685,#219686,#219687,#219688,#219689,#219690,#219691,#219692,
#219693,#219694,#219695,#219696,#219697,#219698,#219699,#219700,#219701,
#219702,#219703,#219704,#219705,#219706,#219707,#219708,#219709,#219710,
#219711,#219712,#219713,#219714,#219715,#219716,#219717,#219718,#219719,
#219720,#219721,#219722,#219723,#219724,#219725,#219726,#219727,#219728,
#219729,#219730,#219731,#219732,#219733,#219734,#219735,#219736,#219737,
#219738,#219739,#219740,#219741,#219742,#219743,#219744,#219745,#219746,
#219747,#219748,#219749,#219750,#219751,#219752,#219753,#219754,#219755,
#219756,#219757,#219758,#219759,#219760,#219761,#219762,#219763,#219764,
#219765,#219766,#219767,#219768,#219769,#219770,#219771,#219772,#219773,
#219774,#219775,#219776,#219777,#219778,#219779,#219780,#219781,#219782,
#219783,#219784,#219785,#219786,#219787,#219788,#219789,#219790,#219791,
#219792,#219793,#219794,#219795,#219796,#219797,#219798,#219799,#219800,
#219801,#219802,#219803,#219804,#219805,#219806,#219807,#219808,#219809,
#219810,#219811,#219812,#219813,#219814,#219815,#219816,#219817,#219818,
#219819,#219820,#219821,#219822,#219823,#219824,#219825,#219826,#219827,
#219828,#219829,#219830,#219831,#219832,#219833,#219834,#219835,#219836,
#219837,#219838,#219839,#219840,#219841,#219842,#219843,#219844,#219845,
#219846,#219847,#219848,#219849,#219850,#219851,#219852,#219853,#219854,
#219855,#219856,#219857,#219858,#219859,#219860,#219861,#219862,#219863,
#219864,#219865,#219866,#219867,#219868,#219869,#219870,#219871,#219872,
#219873,#219874,#219875,#219876,#219877,#219878,#219879,#219880,#219881,
#219882,#219883,#219884,#219885,#219886,#219887,#219888,#219889,#219890,
#219891,#219892,#219893,#219894,#219895,#219896,#219897,#219898,#219899,
#219900,#219901,#219902,#219903,#219904,#219905,#219906,#219907,#219908,
#219909,#219910,#219911,#219912,#219913,#219914,#219915,#219916,#219917,
#219918,#219919,#219920,#219921,#219922,#219923,#219924,#219925,#219926,
#219927,#219928,#219929,#219930,#219931,#219932,#219933,#219934,#219935,
#219936,#219937,#219938,#219939,#219940,#219941,#219942,#219943,#219944,
#219945,#219946,#219947,#219948,#219949,#219950,#219951,#219952,#219953,
#219954,#219955,#219956,#219957,#219958,#219959,#219960,#219961,#219962,
#219963,#219964,#219965,#219966,#219967,#219968,#219969,#219970,#219971,
#219972,#219973,#219974,#219975,#219976,#219977,#219978,#219979,#219980,
#219981,#219982,#219983,#219984,#219985,#219986,#219987,#219988,#219989,
#219990,#219991,#219992,#219993,#219994,#219995,#219996,#219997,#219998,
#219999,#220000,#220001,#220002,#220003,#220004,#220005,#220006,#220007,
#220008,#220009,#220010,#220011,#220012,#220013,#220014,#220015,#220016,
#220017,#220018,#220019,#220020,#220021,#220022,#220023,#220024,#220025,
#220026,#220027,#220028,#220029,#220030,#220031,#220032,#220033,#220034,
#220035,#220036,#220037,#220038,#220039,#220040,#220041,#220042,#220043,
#220044,#220045,#220046,#220047,#220048,#220049,#220050,#220051),(#220052,
#220053,#220054,#220055,#220056,#220057,#220058,#220059,#220060,#220061,
#220062,#220063,#220064,#220065,#220066,#220067,#220068,#220069,#220070,
#220071,#220072,#220073,#220074,#220075,#220076,#220077,#220078,#220079,
#220080,#220081,#220082,#220083,#220084,#220085,#220086,#220087,#220088,
#220089,#220090,#220091,#220092,#220093,#220094,#220095,#220096,#220097,
#220098,#220099,#220100,#220101,#220102,#220103,#220104,#220105,#220106,
#220107,#220108,#220109,#220110,#220111,#220112,#220113,#220114,#220115,
#220116,#220117,#220118,#220119,#220120,#220121,#220122,#220123,#220124,
#220125,#220126,#220127,#220128,#220129,#220130,#220131,#220132,#220133,
#220134,#220135,#220136,#220137,#220138,#220139,#220140,#220141,#220142,
#220143,#220144,#220145,#220146,#220147,#220148,#220149,#220150,#220151,
#220152,#220153,#220154,#220155,#220156,#220157,#220158,#220159,#220160,
#220161,#220162,#220163,#220164,#220165,#220166,#220167,#220168,#220169,
#220170,#220171,#220172,#220173,#220174,#220175,#220176,#220177,#220178,
#220179,#220180,#220181,#220182,#220183,#220184,#220185,#220186,#220187,
#220188,#220189,#220190,#220191,#220192,#220193,#220194,#220195,#220196,
#220197,#220198,#220199,#220200,#220201,#220202,#220203,#220204,#220205,
#220206,#220207,#220208,#220209,#220210,#220211,#220212,#220213,#220214,
#220215,#220216,#220217,#220218,#220219,#220220,#220221,#220222,#220223,
#220224,#220225,#220226,#220227,#220228,#220229,#220230,#220231,#220232,
#220233,#220234,#220235,#220236,#220237,#220238,#220239,#220240,#220241,
#220242,#220243,#220244,#220245,#220246,#220247,#220248,#220249,#220250,
#220251,#220252,#220253,#220254,#220255,#220256,#220257,#220258,#220259,
#220260,#220261,#220262,#220263,#220264,#220265,#220266,#220267,#220268,
#220269,#220270,#220271,#220272,#220273,#220274,#220275,#220276,#220277,
#220278,#220279,#220280,#220281,#220282,#220283,#220284,#220285,#220286,
#220287,#220288,#220289,#220290,#220291,#220292,#220293,#220294,#220295,
#220296,#220297,#220298,#220299,#220300,#220301,#220302,#220303,#220304,
#220305,#220306,#220307,#220308,#220309,#220310,#220311,#220312,#220313,
#220314,#220315,#220316,#220317,#220318,#220319,#220320,#220321,#220322,
#220323,#220324,#220325,#220326,#220327,#220328,#220329,#220330,#220331,
#220332,#220333,#220334,#220335,#220336,#220337,#220338,#220339,#220340,
#220341,#220342,#220343,#220344,#220345,#220346,#220347,#220348,#220349,
#220350,#220351,#220352,#220353,#220354,#220355,#220356,#220357,#220358,
#220359,#220360,#220361,#220362,#220363,#220364,#220365,#220366,#220367,
#220368,#220369,#220370,#220371,#220372,#220373,#220374,#220375,#220376,
#220377,#220378,#220379,#220380,#220381,#220382,#220383,#220384,#220385,
#220386,#220387,#220388,#220389,#220390,#220391,#220392,#220393,#220394,
#220395,#220396,#220397,#220398,#220399,#220400,#220401,#220402,#220403,
#220404,#220405,#220406,#220407,#220408,#220409,#220410,#220411,#220412,
#220413,#220414,#220415,#220416,#220417,#220418,#220419,#220420,#220421,
#220422,#220423,#220424,#220425,#220426,#220427,#220428,#220429,#220430,
#220431,#220432,#220433,#220434,#220435,#220436,#220437,#220438,#220439,
#220440,#220441,#220442,#220443,#220444,#220445,#220446,#220447,#220448,
#220449,#220450,#220451,#220452,#220453,#220454,#220455,#220456,#220457,
#220458,#220459,#220460,#220461,#220462,#220463,#220464,#220465,#220466,
#220467,#220468,#220469,#220470,#220471,#220472,#220473,#220474,#220475,
#220476,#220477,#220478,#220479,#220480,#220481,#220482,#220483,#220484,
#220485,#220486,#220487,#220488,#220489,#220490,#220491,#220492,#220493,
#220494,#220495,#220496,#220497,#220498,#220499,#220500,#220501,#220502,
#220503,#220504,#220505,#220506,#220507,#220508,#220509,#220510,#220511,
#220512,#220513,#220514,#220515,#220516,#220517,#220518,#220519,#220520,
#220521,#220522,#220523,#220524,#220525,#220526,#220527,#220528,#220529,
#220530,#220531,#220532,#220533,#220534,#220535,#220536,#220537,#220538,
#220539,#220540,#220541,#220542,#220543,#220544,#220545,#220546,#220547,
#220548,#220549,#220550,#220551,#220552,#220553,#220554,#220555,#220556,
#220557,#220558,#220559,#220560,#220561,#220562,#220563,#220564,#220565,
#220566,#220567,#220568,#220569,#220570,#220571,#220572,#220573,#220574,
#220575,#220576,#220577,#220578,#220579,#220580,#220581,#220582,#220583,
#220584,#220585,#220586,#220587,#220588,#220589,#220590,#220591,#220592,
#220593,#220594,#220595,#220596,#220597,#220598,#220599,#220600,#220601,
#220602,#220603,#220604,#220605,#220606,#220607,#220608,#220609,#220610,
#220611,#220612,#220613,#220614,#220615,#220616,#220617,#220618,#220619,
#220620,#220621,#220622,#220623,#220624,#220625,#220626,#220627,#220628,
#220629,#220630,#220631,#220632,#220633,#220634,#220635,#220636,#220637,
#220638,#220639,#220640,#220641,#220642,#220643,#220644,#220645,#220646,
#220647,#220648,#220649,#220650,#220651,#220652,#220653,#220654,#220655,
#220656,#220657,#220658,#220659,#220660,#220661,#220662,#220663,#220664,
#220665,#220666,#220667,#220668,#220669,#220670,#220671,#220672,#220673,
#220674,#220675,#220676,#220677,#220678,#220679,#220680,#220681,#220682,
#220683,#220684,#220685,#220686,#220687,#220688,#220689,#220690,#220691,
#220692,#220693,#220694,#220695,#220696,#220697,#220698,#220699,#220700,
#220701,#220702,#220703,#220704,#220705,#220706,#220707,#220708,#220709,
#220710,#220711,#220712,#220713,#220714,#220715,#220716,#220717,#220718,
#220719,#220720,#220721,#220722,#220723,#220724,#220725,#220726,#220727,
#220728,#220729,#220730,#220731,#220732,#220733,#220734,#220735,#220736,
#220737,#220738,#220739,#220740,#220741,#220742,#220743,#220744,#220745,
#220746,#220747,#220748,#220749,#220750,#220751,#220752,#220753,#220754,
#220755,#220756,#220757,#220758,#220759,#220760,#220761,#220762,#220763,
#220764,#220765,#220766,#220767,#220768,#220769,#220770,#220771,#220772,
#220773,#220774,#220775,#220776,#220777,#220778,#220779,#220780,#220781,
#220782,#220783,#220784,#220785,#220786,#220787,#220788,#220789,#220790,
#220791,#220792,#220793,#220794,#220795,#220796,#220797,#220798,#220799,
#220800,#220801,#220802,#220803,#220804,#220805,#220806,#220807,#220808,
#220809,#220810,#220811,#220812,#220813,#220814,#220815,#220816,#220817,
#220818,#220819,#220820,#220821,#220822,#220823,#220824,#220825,#220826,
#220827,#220828,#220829,#220830,#220831,#220832,#220833,#220834,#220835,
#220836,#220837,#220838,#220839,#220840,#220841,#220842,#220843,#220844,
#220845,#220846,#220847,#220848,#220849,#220850,#220851,#220852,#220853,
#220854,#220855,#220856,#220857,#220858,#220859,#220860,#220861,#220862,
#220863,#220864,#220865,#220866,#220867,#220868,#220869,#220870,#220871,
#220872,#220873,#220874,#220875,#220876,#220877,#220878,#220879,#220880,
#220881,#220882,#220883,#220884,#220885,#220886,#220887,#220888,#220889,
#220890,#220891,#220892,#220893,#220894,#220895,#220896,#220897,#220898,
#220899,#220900,#220901,#220902,#220903,#220904,#220905,#220906,#220907,
#220908,#220909,#220910,#220911,#220912,#220913,#220914,#220915,#220916,
#220917,#220918,#220919,#220920,#220921,#220922,#220923,#220924,#220925,
#220926,#220927,#220928,#220929,#220930,#220931,#220932,#220933,#220934,
#220935,#220936,#220937,#220938,#220939,#220940,#220941,#220942,#220943,
#220944,#220945,#220946,#220947,#220948,#220949,#220950,#220951,#220952,
#220953,#220954,#220955,#220956,#220957,#220958,#220959,#220960,#220961,
#220962,#220963,#220964,#220965,#220966,#220967,#220968,#220969,#220970,
#220971,#220972,#220973,#220974,#220975,#220976,#220977,#220978,#220979,
#220980,#220981,#220982,#220983,#220984,#220985,#220986,#220987,#220988,
#220989,#220990,#220991,#220992,#220993,#220994,#220995,#220996,#220997,
#220998,#220999,#221000,#221001,#221002,#221003,#221004,#221005,#221006,
#221007,#221008,#221009,#221010,#221011,#221012,#221013,#221014,#221015,
#221016,#221017,#221018,#221019,#221020,#221021,#221022,#221023,#221024,
#221025,#221026,#221027,#221028,#221029,#221030,#221031,#221032,#221033,
#221034,#221035,#221036,#221037,#221038,#221039,#221040,#221041,#221042,
#221043,#221044,#221045,#221046,#221047,#221048,#221049,#221050,#221051,
#221052,#221053,#221054,#221055,#221056,#221057,#221058,#221059,#221060,
#221061,#221062,#221063,#221064,#221065,#221066,#221067,#221068,#221069,
#221070,#221071,#221072,#221073,#221074,#221075,#221076,#221077,#221078,
#221079,#221080,#221081,#221082,#221083,#221084,#221085,#221086,#221087,
#221088,#221089,#221090,#221091,#221092,#221093,#221094,#221095,#221096,
#221097,#221098,#221099,#221100,#221101,#221102,#221103,#221104,#221105,
#221106,#221107,#221108,#221109,#221110,#221111,#221112,#221113,#221114,
#221115,#221116,#221117,#221118,#221119,#221120,#221121,#221122,#221123,
#221124,#221125,#221126,#221127,#221128,#221129,#221130,#221131,#221132,
#221133,#221134,#221135,#221136,#221137,#221138,#221139,#221140,#221141,
#221142,#221143,#221144,#221145,#221146,#221147,#221148,#221149,#221150,
#221151,#221152,#221153,#221154,#221155,#221156,#221157,#221158,#221159,
#221160,#221161,#221162,#221163,#221164,#221165,#221166,#221167,#221168,
#221169,#221170,#221171,#221172,#221173,#221174,#221175,#221176,#221177,
#221178,#221179,#221180,#221181,#221182,#221183,#221184,#221185,#221186,
#221187,#221188,#221189,#221190,#221191,#221192,#221193,#221194,#221195,
#221196,#221197,#221198,#221199,#221200,#221201,#221202,#221203,#221204,
#221205,#221206,#221207,#221208,#221209,#221210,#221211,#221212,#221213,
#221214,#221215,#221216,#221217,#221218,#221219,#221220,#221221,#221222,
#221223,#221224,#221225,#221226,#221227,#221228,#221229,#221230,#221231,
#221232,#221233,#221234,#221235,#221236,#221237,#221238,#221239,#221240,
#221241,#221242,#221243,#221244,#221245,#221246,#221247,#221248,#221249,
#221250,#221251,#221252,#221253,#221254,#221255,#221256,#221257,#221258,
#221259,#221260,#221261,#221262,#221263,#221264,#221265,#221266,#221267,
#221268,#221269,#221270,#221271,#221272,#221273,#221274,#221275,#221276,
#221277,#221278,#221279,#221280,#221281,#221282,#221283,#221284,#221285,
#221286,#221287,#221288,#221289,#221290,#221291,#221292,#221293,#221294,
#221295,#221296,#221297,#221298,#221299,#221300,#221301,#221302,#221303,
#221304,#221305,#221306,#221307,#221308,#221309,#221310,#221311,#221312,
#221313,#221314,#221315,#221316,#221317,#221318,#221319,#221320,#221321,
#221322,#221323,#221324,#221325,#221326,#221327,#221328,#221329,#221330,
#221331,#221332,#221333,#221334,#221335,#221336,#221337,#221338,#221339,
#221340,#221341,#221342,#221343,#221344,#221345,#221346,#221347,#221348,
#221349,#221350,#221351,#221352,#221353,#221354,#221355,#221356,#221357,
#221358,#221359,#221360,#221361,#221362,#221363,#221364,#221365,#221366,
#221367,#221368,#221369,#221370,#221371,#221372,#221373,#221374,#221375,
#221376,#221377,#221378,#221379,#221380,#221381,#221382,#221383,#221384,
#221385,#221386,#221387,#221388,#221389,#221390,#221391,#221392,#221393,
#221394,#221395,#221396,#221397,#221398,#221399,#221400,#221401,#221402,
#221403,#221404,#221405,#221406,#221407,#221408,#221409,#221410,#221411,
#221412,#221413,#221414,#221415,#221416,#221417,#221418,#221419,#221420,
#221421,#221422,#221423,#221424,#221425,#221426,#221427,#221428,#221429,
#221430,#221431,#221432,#221433,#221434,#221435,#221436,#221437,#221438,
#221439,#221440,#221441,#221442,#221443,#221444,#221445,#221446,#221447,
#221448,#221449,#221450,#221451,#221452,#221453,#221454,#221455,#221456,
#221457,#221458,#221459,#221460,#221461,#221462,#221463,#221464,#221465,
#221466,#221467,#221468,#221469,#221470,#221471,#221472,#221473,#221474,
#221475,#221476,#221477,#221478,#221479,#221480,#221481,#221482,#221483,
#221484,#221485,#221486,#221487,#221488,#221489,#221490,#221491,#221492,
#221493,#221494,#221495,#221496,#221497,#221498,#221499,#221500,#221501,
#221502,#221503,#221504,#221505,#221506,#221507,#221508,#221509,#221510,
#221511,#221512,#221513,#221514,#221515,#221516,#221517,#221518,#221519,
#221520,#221521,#221522,#221523,#221524,#221525,#221526,#221527,#221528,
#221529,#221530,#221531,#221532,#221533,#221534,#221535,#221536,#221537,
#221538,#221539,#221540,#221541,#221542,#221543,#221544,#221545,#221546,
#221547,#221548,#221549,#221550,#221551,#221552,#221553,#221554,#221555,
#221556,#221557,#221558,#221559,#221560,#221561,#221562,#221563,#221564,
#221565,#221566,#221567,#221568,#221569,#221570,#221571,#221572,#221573,
#221574,#221575,#221576,#221577,#221578,#221579,#221580,#221581,#221582,
#221583,#221584,#221585,#221586,#221587,#221588,#221589,#221590,#221591,
#221592,#221593,#221594,#221595,#221596,#221597,#221598,#221599,#221600,
#221601,#221602,#221603,#221604,#221605,#221606,#221607,#221608,#221609,
#221610,#221611,#221612,#221613,#221614,#221615,#221616,#221617,#221618,
#221619,#221620,#221621,#221622,#221623,#221624,#221625,#221626,#221627,
#221628,#221629,#221630,#221631,#221632,#221633,#221634,#221635,#221636,
#221637,#221638,#221639,#221640,#221641,#221642,#221643,#221644,#221645,
#221646,#221647,#221648,#221649,#221650,#221651,#221652,#221653,#221654,
#221655,#221656,#221657,#221658,#221659,#221660,#221661,#221662,#221663,
#221664,#221665,#221666,#221667,#221668,#221669,#221670,#221671,#221672,
#221673,#221674,#221675,#221676,#221677,#221678,#221679,#221680,#221681,
#221682,#221683,#221684,#221685,#221686,#221687,#221688,#221689,#221690,
#221691,#221692,#221693,#221694,#221695,#221696,#221697,#221698,#221699,
#221700,#221701,#221702,#221703,#221704,#221705,#221706,#221707,#221708,
#221709,#221710,#221711,#221712,#221713,#221714,#221715,#221716,#221717,
#221718,#221719,#221720,#221721,#221722,#221723,#221724,#221725,#221726,
#221727,#221728,#221729,#221730,#221731,#221732,#221733,#221734,#221735,
#221736,#221737,#221738,#221739,#221740,#221741,#221742,#221743,#221744,
#221745,#221746),(#221747,#221748,#221749,#221750,#221751,#221752,#221753,
#221754,#221755,#221756,#221757,#221758,#221759,#221760,#221761,#221762,
#221763,#221764,#221765,#221766,#221767,#221768,#221769,#221770,#221771,
#221772,#221773,#221774,#221775,#221776,#221777,#221778,#221779,#221780,
#221781,#221782,#221783,#221784,#221785,#221786,#221787,#221788,#221789,
#221790,#221791,#221792,#221793,#221794,#221795,#221796,#221797,#221798,
#221799,#221800,#221801,#221802,#221803,#221804,#221805,#221806,#221807,
#221808,#221809,#221810,#221811,#221812,#221813,#221814,#221815,#221816,
#221817,#221818,#221819,#221820,#221821,#221822,#221823,#221824,#221825,
#221826,#221827,#221828,#221829,#221830,#221831,#221832,#221833,#221834,
#221835,#221836,#221837,#221838,#221839,#221840,#221841,#221842,#221843,
#221844,#221845,#221846,#221847,#221848,#221849,#221850,#221851,#221852,
#221853,#221854,#221855,#221856,#221857,#221858,#221859,#221860,#221861,
#221862,#221863,#221864,#221865,#221866,#221867,#221868,#221869,#221870,
#221871,#221872,#221873,#221874,#221875,#221876,#221877,#221878,#221879,
#221880,#221881,#221882,#221883,#221884,#221885,#221886,#221887,#221888,
#221889,#221890,#221891,#221892,#221893,#221894,#221895,#221896,#221897,
#221898,#221899,#221900,#221901,#221902,#221903,#221904,#221905,#221906,
#221907,#221908,#221909,#221910,#221911,#221912,#221913,#221914,#221915,
#221916,#221917,#221918,#221919,#221920,#221921,#221922,#221923,#221924,
#221925,#221926,#221927,#221928,#221929,#221930,#221931,#221932,#221933,
#221934,#221935,#221936,#221937,#221938,#221939,#221940,#221941,#221942,
#221943,#221944,#221945,#221946,#221947,#221948,#221949,#221950,#221951,
#221952,#221953,#221954,#221955,#221956,#221957,#221958,#221959,#221960,
#221961,#221962,#221963,#221964,#221965,#221966,#221967,#221968,#221969,
#221970,#221971,#221972,#221973,#221974,#221975,#221976,#221977,#221978,
#221979,#221980,#221981,#221982,#221983,#221984,#221985,#221986,#221987,
#221988,#221989,#221990,#221991,#221992,#221993,#221994,#221995,#221996,
#221997,#221998,#221999,#222000,#222001,#222002,#222003,#222004,#222005,
#222006,#222007,#222008,#222009,#222010,#222011,#222012,#222013,#222014,
#222015,#222016,#222017,#222018,#222019,#222020,#222021,#222022,#222023,
#222024,#222025,#222026,#222027,#222028,#222029,#222030,#222031,#222032,
#222033,#222034,#222035,#222036,#222037,#222038,#222039,#222040,#222041,
#222042,#222043,#222044,#222045,#222046,#222047,#222048,#222049,#222050,
#222051,#222052,#222053,#222054,#222055,#222056,#222057,#222058,#222059,
#222060,#222061,#222062,#222063,#222064,#222065,#222066,#222067,#222068,
#222069,#222070,#222071,#222072,#222073,#222074,#222075,#222076,#222077,
#222078,#222079,#222080,#222081,#222082,#222083,#222084,#222085,#222086,
#222087,#222088,#222089,#222090,#222091,#222092,#222093,#222094,#222095,
#222096,#222097,#222098,#222099,#222100,#222101,#222102,#222103,#222104,
#222105,#222106,#222107,#222108,#222109,#222110,#222111,#222112,#222113,
#222114,#222115,#222116,#222117,#222118,#222119,#222120,#222121,#222122,
#222123,#222124,#222125,#222126,#222127,#222128,#222129,#222130,#222131,
#222132,#222133,#222134,#222135,#222136,#222137,#222138,#222139,#222140,
#222141,#222142,#222143,#222144,#222145,#222146,#222147,#222148,#222149,
#222150,#222151,#222152,#222153,#222154,#222155,#222156,#222157,#222158,
#222159,#222160,#222161,#222162,#222163,#222164,#222165,#222166,#222167,
#222168,#222169,#222170,#222171,#222172,#222173,#222174,#222175,#222176,
#222177,#222178,#222179,#222180,#222181,#222182,#222183,#222184,#222185,
#222186,#222187,#222188,#222189,#222190,#222191,#222192,#222193,#222194,
#222195,#222196,#222197,#222198,#222199,#222200,#222201,#222202,#222203,
#222204,#222205,#222206,#222207,#222208,#222209,#222210,#222211,#222212,
#222213,#222214,#222215,#222216,#222217,#222218,#222219,#222220,#222221,
#222222,#222223,#222224,#222225,#222226,#222227,#222228,#222229,#222230,
#222231,#222232,#222233,#222234,#222235,#222236,#222237,#222238,#222239,
#222240,#222241,#222242,#222243,#222244,#222245,#222246,#222247,#222248,
#222249,#222250,#222251,#222252,#222253,#222254,#222255,#222256,#222257,
#222258,#222259,#222260,#222261,#222262,#222263,#222264,#222265,#222266,
#222267,#222268,#222269,#222270,#222271,#222272,#222273,#222274,#222275,
#222276,#222277,#222278,#222279,#222280,#222281,#222282,#222283,#222284,
#222285,#222286,#222287,#222288,#222289,#222290,#222291,#222292,#222293,
#222294,#222295,#222296,#222297,#222298,#222299,#222300,#222301,#222302,
#222303,#222304,#222305,#222306,#222307,#222308,#222309,#222310,#222311,
#222312,#222313,#222314,#222315,#222316,#222317,#222318,#222319,#222320,
#222321,#222322,#222323,#222324,#222325,#222326,#222327,#222328,#222329,
#222330,#222331,#222332,#222333,#222334,#222335,#222336,#222337,#222338,
#222339,#222340,#222341,#222342,#222343,#222344,#222345,#222346,#222347,
#222348,#222349,#222350,#222351,#222352,#222353,#222354,#222355,#222356,
#222357,#222358,#222359,#222360,#222361,#222362,#222363,#222364,#222365,
#222366,#222367,#222368,#222369,#222370,#222371,#222372,#222373,#222374,
#222375,#222376,#222377,#222378,#222379,#222380,#222381,#222382,#222383,
#222384,#222385,#222386,#222387,#222388,#222389,#222390,#222391,#222392,
#222393,#222394,#222395,#222396,#222397,#222398,#222399,#222400,#222401,
#222402,#222403,#222404,#222405,#222406,#222407,#222408,#222409,#222410,
#222411,#222412,#222413,#222414,#222415,#222416,#222417,#222418,#222419,
#222420,#222421,#222422,#222423,#222424,#222425,#222426,#222427,#222428,
#222429,#222430,#222431,#222432,#222433,#222434,#222435,#222436,#222437,
#222438,#222439,#222440,#222441,#222442,#222443,#222444,#222445,#222446,
#222447,#222448,#222449,#222450,#222451,#222452,#222453,#222454,#222455,
#222456,#222457,#222458,#222459,#222460,#222461,#222462,#222463,#222464,
#222465,#222466,#222467,#222468,#222469,#222470,#222471,#222472,#222473,
#222474,#222475,#222476,#222477,#222478,#222479,#222480,#222481,#222482,
#222483,#222484,#222485,#222486,#222487,#222488,#222489,#222490,#222491,
#222492,#222493,#222494,#222495,#222496,#222497,#222498,#222499,#222500,
#222501,#222502,#222503,#222504,#222505,#222506,#222507,#222508,#222509,
#222510,#222511,#222512,#222513,#222514,#222515,#222516,#222517,#222518,
#222519,#222520,#222521,#222522,#222523,#222524,#222525,#222526,#222527,
#222528,#222529,#222530,#222531,#222532,#222533,#222534,#222535,#222536,
#222537,#222538,#222539,#222540,#222541,#222542,#222543,#222544,#222545,
#222546,#222547,#222548,#222549,#222550,#222551,#222552,#222553,#222554,
#222555,#222556,#222557,#222558,#222559,#222560,#222561,#222562,#222563,
#222564,#222565,#222566,#222567,#222568,#222569,#222570,#222571,#222572,
#222573,#222574,#222575,#222576,#222577,#222578,#222579,#222580,#222581,
#222582,#222583,#222584,#222585,#222586,#222587,#222588,#222589,#222590,
#222591,#222592,#222593,#222594,#222595,#222596,#222597,#222598,#222599,
#222600,#222601,#222602,#222603,#222604,#222605,#222606,#222607,#222608,
#222609,#222610,#222611,#222612,#222613,#222614,#222615,#222616,#222617,
#222618,#222619,#222620,#222621,#222622,#222623,#222624,#222625,#222626,
#222627,#222628,#222629,#222630,#222631,#222632,#222633,#222634,#222635,
#222636,#222637,#222638,#222639,#222640,#222641,#222642,#222643,#222644,
#222645,#222646,#222647,#222648,#222649,#222650,#222651,#222652,#222653,
#222654,#222655,#222656,#222657,#222658,#222659,#222660,#222661,#222662,
#222663,#222664,#222665,#222666,#222667,#222668,#222669,#222670,#222671,
#222672,#222673,#222674,#222675,#222676,#222677,#222678,#222679,#222680,
#222681,#222682,#222683,#222684,#222685,#222686,#222687,#222688,#222689,
#222690,#222691,#222692,#222693,#222694,#222695,#222696,#222697,#222698,
#222699,#222700,#222701,#222702,#222703,#222704,#222705,#222706,#222707,
#222708,#222709,#222710,#222711,#222712,#222713,#222714,#222715,#222716,
#222717,#222718,#222719,#222720,#222721,#222722,#222723,#222724,#222725,
#222726,#222727,#222728,#222729,#222730,#222731,#222732,#222733,#222734,
#222735,#222736,#222737,#222738,#222739,#222740,#222741,#222742,#222743,
#222744,#222745,#222746,#222747,#222748,#222749,#222750,#222751,#222752,
#222753,#222754,#222755,#222756,#222757,#222758,#222759,#222760,#222761,
#222762,#222763,#222764,#222765,#222766,#222767,#222768,#222769,#222770,
#222771,#222772,#222773,#222774,#222775,#222776,#222777,#222778,#222779,
#222780,#222781,#222782,#222783,#222784,#222785,#222786,#222787,#222788,
#222789,#222790,#222791,#222792,#222793,#222794,#222795,#222796,#222797,
#222798,#222799,#222800,#222801,#222802,#222803,#222804,#222805,#222806,
#222807,#222808,#222809,#222810,#222811,#222812,#222813,#222814,#222815,
#222816,#222817,#222818,#222819,#222820,#222821,#222822,#222823,#222824,
#222825,#222826,#222827,#222828,#222829,#222830,#222831,#222832,#222833,
#222834,#222835,#222836,#222837,#222838,#222839,#222840,#222841,#222842,
#222843,#222844,#222845,#222846,#222847,#222848,#222849,#222850,#222851,
#222852,#222853,#222854,#222855,#222856,#222857,#222858,#222859,#222860,
#222861,#222862,#222863,#222864,#222865,#222866,#222867,#222868,#222869,
#222870,#222871,#222872,#222873,#222874,#222875,#222876,#222877,#222878,
#222879,#222880,#222881,#222882,#222883,#222884,#222885,#222886,#222887,
#222888,#222889,#222890,#222891,#222892,#222893,#222894,#222895,#222896,
#222897,#222898,#222899,#222900,#222901,#222902,#222903,#222904,#222905,
#222906,#222907,#222908,#222909,#222910,#222911,#222912,#222913,#222914,
#222915,#222916,#222917,#222918,#222919,#222920,#222921,#222922,#222923,
#222924,#222925,#222926,#222927,#222928,#222929,#222930,#222931,#222932,
#222933,#222934,#222935,#222936,#222937,#222938,#222939,#222940,#222941,
#222942,#222943,#222944,#222945,#222946,#222947,#222948,#222949,#222950,
#222951,#222952,#222953,#222954,#222955,#222956,#222957,#222958,#222959,
#222960,#222961,#222962,#222963,#222964,#222965,#222966,#222967,#222968,
#222969,#222970,#222971,#222972,#222973,#222974,#222975,#222976,#222977,
#222978,#222979,#222980,#222981,#222982,#222983,#222984,#222985,#222986,
#222987,#222988,#222989,#222990,#222991,#222992,#222993,#222994,#222995,
#222996,#222997,#222998,#222999,#223000,#223001,#223002,#223003,#223004,
#223005,#223006,#223007,#223008,#223009,#223010,#223011,#223012,#223013,
#223014,#223015,#223016,#223017,#223018,#223019,#223020,#223021,#223022,
#223023,#223024,#223025,#223026,#223027,#223028,#223029,#223030,#223031,
#223032,#223033,#223034,#223035,#223036,#223037,#223038,#223039,#223040,
#223041,#223042,#223043,#223044,#223045,#223046,#223047,#223048,#223049,
#223050,#223051,#223052,#223053,#223054,#223055,#223056,#223057,#223058,
#223059,#223060,#223061,#223062,#223063,#223064,#223065,#223066,#223067,
#223068,#223069,#223070,#223071,#223072,#223073,#223074,#223075,#223076,
#223077,#223078,#223079,#223080,#223081,#223082,#223083,#223084,#223085,
#223086,#223087,#223088,#223089,#223090,#223091,#223092,#223093,#223094,
#223095,#223096,#223097,#223098,#223099,#223100,#223101,#223102,#223103,
#223104,#223105,#223106,#223107,#223108,#223109,#223110,#223111,#223112,
#223113,#223114,#223115,#223116,#223117,#223118,#223119,#223120,#223121,
#223122,#223123,#223124,#223125,#223126,#223127,#223128,#223129,#223130,
#223131,#223132,#223133,#223134,#223135,#223136,#223137,#223138,#223139,
#223140,#223141,#223142,#223143,#223144,#223145,#223146,#223147,#223148,
#223149,#223150,#223151,#223152,#223153,#223154,#223155,#223156,#223157,
#223158,#223159,#223160,#223161,#223162,#223163,#223164,#223165,#223166,
#223167,#223168,#223169,#223170,#223171,#223172,#223173,#223174,#223175,
#223176,#223177,#223178,#223179,#223180,#223181,#223182,#223183,#223184,
#223185,#223186,#223187,#223188,#223189,#223190,#223191,#223192,#223193,
#223194,#223195,#223196,#223197,#223198,#223199,#223200,#223201,#223202,
#223203,#223204,#223205,#223206,#223207,#223208,#223209,#223210,#223211,
#223212,#223213,#223214,#223215,#223216,#223217,#223218,#223219,#223220,
#223221,#223222,#223223,#223224,#223225,#223226,#223227,#223228,#223229,
#223230,#223231,#223232,#223233,#223234,#223235,#223236,#223237,#223238,
#223239,#223240,#223241,#223242,#223243,#223244,#223245,#223246,#223247,
#223248,#223249,#223250,#223251,#223252,#223253,#223254,#223255,#223256,
#223257,#223258,#223259,#223260,#223261,#223262,#223263,#223264,#223265,
#223266,#223267,#223268,#223269,#223270,#223271,#223272,#223273,#223274,
#223275,#223276,#223277,#223278,#223279,#223280,#223281,#223282,#223283,
#223284,#223285,#223286,#223287,#223288,#223289,#223290,#223291,#223292,
#223293,#223294,#223295,#223296,#223297,#223298,#223299,#223300,#223301,
#223302,#223303,#223304,#223305,#223306,#223307,#223308,#223309,#223310,
#223311,#223312,#223313,#223314,#223315,#223316,#223317,#223318,#223319,
#223320,#223321,#223322,#223323,#223324,#223325,#223326,#223327,#223328,
#223329,#223330,#223331,#223332,#223333,#223334,#223335,#223336,#223337,
#223338,#223339,#223340,#223341,#223342,#223343,#223344,#223345,#223346,
#223347,#223348,#223349,#223350,#223351,#223352,#223353,#223354,#223355,
#223356,#223357,#223358,#223359,#223360,#223361,#223362,#223363,#223364,
#223365,#223366,#223367,#223368,#223369,#223370,#223371,#223372,#223373,
#223374,#223375,#223376,#223377,#223378,#223379,#223380,#223381,#223382,
#223383,#223384,#223385,#223386,#223387,#223388,#223389,#223390,#223391,
#223392,#223393,#223394,#223395,#223396,#223397,#223398,#223399,#223400,
#223401,#223402,#223403,#223404,#223405,#223406,#223407,#223408,#223409,
#223410,#223411,#223412,#223413,#223414,#223415,#223416,#223417,#223418,
#223419,#223420,#223421,#223422,#223423,#223424,#223425,#223426,#223427,
#223428,#223429,#223430,#223431,#223432,#223433,#223434,#223435,#223436,
#223437,#223438,#223439,#223440,#223441),(#223442,#223443,#223444,#223445,
#223446,#223447,#223448,#223449,#223450,#223451,#223452,#223453,#223454,
#223455,#223456,#223457,#223458,#223459,#223460,#223461,#223462,#223463,
#223464,#223465,#223466,#223467,#223468,#223469,#223470,#223471,#223472,
#223473,#223474,#223475,#223476,#223477,#223478,#223479,#223480,#223481,
#223482,#223483,#223484,#223485,#223486,#223487,#223488,#223489,#223490,
#223491,#223492,#223493,#223494,#223495,#223496,#223497,#223498,#223499,
#223500,#223501,#223502,#223503,#223504,#223505,#223506,#223507,#223508,
#223509,#223510,#223511,#223512,#223513,#223514,#223515,#223516,#223517,
#223518,#223519,#223520,#223521,#223522,#223523,#223524,#223525,#223526,
#223527,#223528,#223529,#223530,#223531,#223532,#223533,#223534,#223535,
#223536,#223537,#223538,#223539,#223540,#223541,#223542,#223543,#223544,
#223545,#223546,#223547,#223548,#223549,#223550,#223551,#223552,#223553,
#223554,#223555,#223556,#223557,#223558,#223559,#223560,#223561,#223562,
#223563,#223564,#223565,#223566,#223567,#223568,#223569,#223570,#223571,
#223572,#223573,#223574,#223575,#223576,#223577,#223578,#223579,#223580,
#223581,#223582,#223583,#223584,#223585,#223586,#223587,#223588,#223589,
#223590,#223591,#223592,#223593,#223594,#223595,#223596,#223597,#223598,
#223599,#223600,#223601,#223602,#223603,#223604,#223605,#223606,#223607,
#223608,#223609,#223610,#223611,#223612,#223613,#223614,#223615,#223616,
#223617,#223618,#223619,#223620,#223621,#223622,#223623,#223624,#223625,
#223626,#223627,#223628,#223629,#223630,#223631,#223632,#223633,#223634,
#223635,#223636,#223637,#223638,#223639,#223640,#223641,#223642,#223643,
#223644,#223645,#223646,#223647,#223648,#223649,#223650,#223651,#223652,
#223653,#223654,#223655,#223656,#223657,#223658,#223659,#223660,#223661,
#223662,#223663,#223664,#223665,#223666,#223667,#223668,#223669,#223670,
#223671,#223672,#223673,#223674,#223675,#223676,#223677,#223678,#223679,
#223680,#223681,#223682,#223683,#223684,#223685,#223686,#223687,#223688,
#223689,#223690,#223691,#223692,#223693,#223694,#223695,#223696,#223697,
#223698,#223699,#223700,#223701,#223702,#223703,#223704,#223705,#223706,
#223707,#223708,#223709,#223710,#223711,#223712,#223713,#223714,#223715,
#223716,#223717,#223718,#223719,#223720,#223721,#223722,#223723,#223724,
#223725,#223726,#223727,#223728,#223729,#223730,#223731,#223732,#223733,
#223734,#223735,#223736,#223737,#223738,#223739,#223740,#223741,#223742,
#223743,#223744,#223745,#223746,#223747,#223748,#223749,#223750,#223751,
#223752,#223753,#223754,#223755,#223756,#223757,#223758,#223759,#223760,
#223761,#223762,#223763,#223764,#223765,#223766,#223767,#223768,#223769,
#223770,#223771,#223772,#223773,#223774,#223775,#223776,#223777,#223778,
#223779,#223780,#223781,#223782,#223783,#223784,#223785,#223786,#223787,
#223788,#223789,#223790,#223791,#223792,#223793,#223794,#223795,#223796,
#223797,#223798,#223799,#223800,#223801,#223802,#223803,#223804,#223805,
#223806,#223807,#223808,#223809,#223810,#223811,#223812,#223813,#223814,
#223815,#223816,#223817,#223818,#223819,#223820,#223821,#223822,#223823,
#223824,#223825,#223826,#223827,#223828,#223829,#223830,#223831,#223832,
#223833,#223834,#223835,#223836,#223837,#223838,#223839,#223840,#223841,
#223842,#223843,#223844,#223845,#223846,#223847,#223848,#223849,#223850,
#223851,#223852,#223853,#223854,#223855,#223856,#223857,#223858,#223859,
#223860,#223861,#223862,#223863,#223864,#223865,#223866,#223867,#223868,
#223869,#223870,#223871,#223872,#223873,#223874,#223875,#223876,#223877,
#223878,#223879,#223880,#223881,#223882,#223883,#223884,#223885,#223886,
#223887,#223888,#223889,#223890,#223891,#223892,#223893,#223894,#223895,
#223896,#223897,#223898,#223899,#223900,#223901,#223902,#223903,#223904,
#223905,#223906,#223907,#223908,#223909,#223910,#223911,#223912,#223913,
#223914,#223915,#223916,#223917,#223918,#223919,#223920,#223921,#223922,
#223923,#223924,#223925,#223926,#223927,#223928,#223929,#223930,#223931,
#223932,#223933,#223934,#223935,#223936,#223937,#223938,#223939,#223940,
#223941,#223942,#223943,#223944,#223945,#223946,#223947,#223948,#223949,
#223950,#223951,#223952,#223953,#223954,#223955,#223956,#223957,#223958,
#223959,#223960,#223961,#223962,#223963,#223964,#223965,#223966,#223967,
#223968,#223969,#223970,#223971,#223972,#223973,#223974,#223975,#223976,
#223977,#223978,#223979,#223980,#223981,#223982,#223983,#223984,#223985,
#223986,#223987,#223988,#223989,#223990,#223991,#223992,#223993,#223994,
#223995,#223996,#223997,#223998,#223999,#224000,#224001,#224002,#224003,
#224004,#224005,#224006,#224007,#224008,#224009,#224010,#224011,#224012,
#224013,#224014,#224015,#224016,#224017,#224018,#224019,#224020,#224021,
#224022,#224023,#224024,#224025,#224026,#224027,#224028,#224029,#224030,
#224031,#224032,#224033,#224034,#224035,#224036,#224037,#224038,#224039,
#224040,#224041,#224042,#224043,#224044,#224045,#224046,#224047,#224048,
#224049,#224050,#224051,#224052,#224053,#224054,#224055,#224056,#224057,
#224058,#224059,#224060,#224061,#224062,#224063,#224064,#224065,#224066,
#224067,#224068,#224069,#224070,#224071,#224072,#224073,#224074,#224075,
#224076,#224077,#224078,#224079,#224080,#224081,#224082,#224083,#224084,
#224085,#224086,#224087,#224088,#224089,#224090,#224091,#224092,#224093,
#224094,#224095,#224096,#224097,#224098,#224099,#224100,#224101,#224102,
#224103,#224104,#224105,#224106,#224107,#224108,#224109,#224110,#224111,
#224112,#224113,#224114,#224115,#224116,#224117,#224118,#224119,#224120,
#224121,#224122,#224123,#224124,#224125,#224126,#224127,#224128,#224129,
#224130,#224131,#224132,#224133,#224134,#224135,#224136,#224137,#224138,
#224139,#224140,#224141,#224142,#224143,#224144,#224145,#224146,#224147,
#224148,#224149,#224150,#224151,#224152,#224153,#224154,#224155,#224156,
#224157,#224158,#224159,#224160,#224161,#224162,#224163,#224164,#224165,
#224166,#224167,#224168,#224169,#224170,#224171,#224172,#224173,#224174,
#224175,#224176,#224177,#224178,#224179,#224180,#224181,#224182,#224183,
#224184,#224185,#224186,#224187,#224188,#224189,#224190,#224191,#224192,
#224193,#224194,#224195,#224196,#224197,#224198,#224199,#224200,#224201,
#224202,#224203,#224204,#224205,#224206,#224207,#224208,#224209,#224210,
#224211,#224212,#224213,#224214,#224215,#224216,#224217,#224218,#224219,
#224220,#224221,#224222,#224223,#224224,#224225,#224226,#224227,#224228,
#224229,#224230,#224231,#224232,#224233,#224234,#224235,#224236,#224237,
#224238,#224239,#224240,#224241,#224242,#224243,#224244,#224245,#224246,
#224247,#224248,#224249,#224250,#224251,#224252,#224253,#224254,#224255,
#224256,#224257,#224258,#224259,#224260,#224261,#224262,#224263,#224264,
#224265,#224266,#224267,#224268,#224269,#224270,#224271,#224272,#224273,
#224274,#224275,#224276,#224277,#224278,#224279,#224280,#224281,#224282,
#224283,#224284,#224285,#224286,#224287,#224288,#224289,#224290,#224291,
#224292,#224293,#224294,#224295,#224296,#224297,#224298,#224299,#224300,
#224301,#224302,#224303,#224304,#224305,#224306,#224307,#224308,#224309,
#224310,#224311,#224312,#224313,#224314,#224315,#224316,#224317,#224318,
#224319,#224320,#224321,#224322,#224323,#224324,#224325,#224326,#224327,
#224328,#224329,#224330,#224331,#224332,#224333,#224334,#224335,#224336,
#224337,#224338,#224339,#224340,#224341,#224342,#224343,#224344,#224345,
#224346,#224347,#224348,#224349,#224350,#224351,#224352,#224353,#224354,
#224355,#224356,#224357,#224358,#224359,#224360,#224361,#224362,#224363,
#224364,#224365,#224366,#224367,#224368,#224369,#224370,#224371,#224372,
#224373,#224374,#224375,#224376,#224377,#224378,#224379,#224380,#224381,
#224382,#224383,#224384,#224385,#224386,#224387,#224388,#224389,#224390,
#224391,#224392,#224393,#224394,#224395,#224396,#224397,#224398,#224399,
#224400,#224401,#224402,#224403,#224404,#224405,#224406,#224407,#224408,
#224409,#224410,#224411,#224412,#224413,#224414,#224415,#224416,#224417,
#224418,#224419,#224420,#224421,#224422,#224423,#224424,#224425,#224426,
#224427,#224428,#224429,#224430,#224431,#224432,#224433,#224434,#224435,
#224436,#224437,#224438,#224439,#224440,#224441,#224442,#224443,#224444,
#224445,#224446,#224447,#224448,#224449,#224450,#224451,#224452,#224453,
#224454,#224455,#224456,#224457,#224458,#224459,#224460,#224461,#224462,
#224463,#224464,#224465,#224466,#224467,#224468,#224469,#224470,#224471,
#224472,#224473,#224474,#224475,#224476,#224477,#224478,#224479,#224480,
#224481,#224482,#224483,#224484,#224485,#224486,#224487,#224488,#224489,
#224490,#224491,#224492,#224493,#224494,#224495,#224496,#224497,#224498,
#224499,#224500,#224501,#224502,#224503,#224504,#224505,#224506,#224507,
#224508,#224509,#224510,#224511,#224512,#224513,#224514,#224515,#224516,
#224517,#224518,#224519,#224520,#224521,#224522,#224523,#224524,#224525,
#224526,#224527,#224528,#224529,#224530,#224531,#224532,#224533,#224534,
#224535,#224536,#224537,#224538,#224539,#224540,#224541,#224542,#224543,
#224544,#224545,#224546,#224547,#224548,#224549,#224550,#224551,#224552,
#224553,#224554,#224555,#224556,#224557,#224558,#224559,#224560,#224561,
#224562,#224563,#224564,#224565,#224566,#224567,#224568,#224569,#224570,
#224571,#224572,#224573,#224574,#224575,#224576,#224577,#224578,#224579,
#224580,#224581,#224582,#224583,#224584,#224585,#224586,#224587,#224588,
#224589,#224590,#224591,#224592,#224593,#224594,#224595,#224596,#224597,
#224598,#224599,#224600,#224601,#224602,#224603,#224604,#224605,#224606,
#224607,#224608,#224609,#224610,#224611,#224612,#224613,#224614,#224615,
#224616,#224617,#224618,#224619,#224620,#224621,#224622,#224623,#224624,
#224625,#224626,#224627,#224628,#224629,#224630,#224631,#224632,#224633,
#224634,#224635,#224636,#224637,#224638,#224639,#224640,#224641,#224642,
#224643,#224644,#224645,#224646,#224647,#224648,#224649,#224650,#224651,
#224652,#224653,#224654,#224655,#224656,#224657,#224658,#224659,#224660,
#224661,#224662,#224663,#224664,#224665,#224666,#224667,#224668,#224669,
#224670,#224671,#224672,#224673,#224674,#224675,#224676,#224677,#224678,
#224679,#224680,#224681,#224682,#224683,#224684,#224685,#224686,#224687,
#224688,#224689,#224690,#224691,#224692,#224693,#224694,#224695,#224696,
#224697,#224698,#224699,#224700,#224701,#224702,#224703,#224704,#224705,
#224706,#224707,#224708,#224709,#224710,#224711,#224712,#224713,#224714,
#224715,#224716,#224717,#224718,#224719,#224720,#224721,#224722,#224723,
#224724,#224725,#224726,#224727,#224728,#224729,#224730,#224731,#224732,
#224733,#224734,#224735,#224736,#224737,#224738,#224739,#224740,#224741,
#224742,#224743,#224744,#224745,#224746,#224747,#224748,#224749,#224750,
#224751,#224752,#224753,#224754,#224755,#224756,#224757,#224758,#224759,
#224760,#224761,#224762,#224763,#224764,#224765,#224766,#224767,#224768,
#224769,#224770,#224771,#224772,#224773,#224774,#224775,#224776,#224777,
#224778,#224779,#224780,#224781,#224782,#224783,#224784,#224785,#224786,
#224787,#224788,#224789,#224790,#224791,#224792,#224793,#224794,#224795,
#224796,#224797,#224798,#224799,#224800,#224801,#224802,#224803,#224804,
#224805,#224806,#224807,#224808,#224809,#224810,#224811,#224812,#224813,
#224814,#224815,#224816,#224817,#224818,#224819,#224820,#224821,#224822,
#224823,#224824,#224825,#224826,#224827,#224828,#224829,#224830,#224831,
#224832,#224833,#224834,#224835,#224836,#224837,#224838,#224839,#224840,
#224841,#224842,#224843,#224844,#224845,#224846,#224847,#224848,#224849,
#224850,#224851,#224852,#224853,#224854,#224855,#224856,#224857,#224858,
#224859,#224860,#224861,#224862,#224863,#224864,#224865,#224866,#224867,
#224868,#224869,#224870,#224871,#224872,#224873,#224874,#224875,#224876,
#224877,#224878,#224879,#224880,#224881,#224882,#224883,#224884,#224885,
#224886,#224887,#224888,#224889,#224890,#224891,#224892,#224893,#224894,
#224895,#224896,#224897,#224898,#224899,#224900,#224901,#224902,#224903,
#224904,#224905,#224906,#224907,#224908,#224909,#224910,#224911,#224912,
#224913,#224914,#224915,#224916,#224917,#224918,#224919,#224920,#224921,
#224922,#224923,#224924,#224925,#224926,#224927,#224928,#224929,#224930,
#224931,#224932,#224933,#224934,#224935,#224936,#224937,#224938,#224939,
#224940,#224941,#224942,#224943,#224944,#224945,#224946,#224947,#224948,
#224949,#224950,#224951,#224952,#224953,#224954,#224955,#224956,#224957,
#224958,#224959,#224960,#224961,#224962,#224963,#224964,#224965,#224966,
#224967,#224968,#224969,#224970,#224971,#224972,#224973,#224974,#224975,
#224976,#224977,#224978,#224979,#224980,#224981,#224982,#224983,#224984,
#224985,#224986,#224987,#224988,#224989,#224990,#224991,#224992,#224993,
#224994,#224995,#224996,#224997,#224998,#224999,#225000,#225001,#225002,
#225003,#225004,#225005,#225006,#225007,#225008,#225009,#225010,#225011,
#225012,#225013,#225014,#225015,#225016,#225017,#225018,#225019,#225020,
#225021,#225022,#225023,#225024,#225025,#225026,#225027,#225028,#225029,
#225030,#225031,#225032,#225033,#225034,#225035,#225036,#225037,#225038,
#225039,#225040,#225041,#225042,#225043,#225044,#225045,#225046,#225047,
#225048,#225049,#225050,#225051,#225052,#225053,#225054,#225055,#225056,
#225057,#225058,#225059,#225060,#225061,#225062,#225063,#225064,#225065,
#225066,#225067,#225068,#225069,#225070,#225071,#225072,#225073,#225074,
#225075,#225076,#225077,#225078,#225079,#225080,#225081,#225082,#225083,
#225084,#225085,#225086,#225087,#225088,#225089,#225090,#225091,#225092,
#225093,#225094,#225095,#225096,#225097,#225098,#225099,#225100,#225101,
#225102,#225103,#225104,#225105,#225106,#225107,#225108,#225109,#225110,
#225111,#225112,#225113,#225114,#225115,#225116,#225117,#225118,#225119,
#225120,#225121,#225122,#225123,#225124,#225125,#225126,#225127,#225128,
#225129,#225130,#225131,#225132,#225133,#225134,#225135,#225136)),
 .UNSPECIFIED.,.F.,.F.,.F.,(4,4),(4,1,1,1,1,1,1,1,1,1,1,1,1,1,1,1,1,1,1,
1,1,1,1,1,1,1,1,1,1,1,1,1,1,1,1,1,1,1,1,1,1,1,1,1,1,1,1,1,1,1,1,1,1,1,1,
1,1,1,1,1,1,1,1,1,1,1,1,1,1,1,1,1,1,1,1,1,1,1,1,1,1,1,1,1,1,1,1,1,1,1,1,
1,1,1,1,1,1,1,1,1,1,1,1,1,1,1,1,1,1,1,1,1,1,1,1,1,1,1,1,1,1,1,1,1,1,1,1,
1,1,1,1,1,1,1,1,1,1,1,1,1,1,1,1,1,1,1,1,1,1,1,1,1,1,1,1,1,1,1,1,1,1,1,1,
1,1,1,1,1,1,1,1,1,1,1,1,1,1,1,1,1,1,1,1,1,1,1,1,1,1,1,1,1,1,1,1,1,1,1,1,
1,1,1,1,1,1,1,1,1,1,1,1,1,1,1,1,1,1,1,1,1,1,1,1,1,1,1,1,1,1,1,1,1,1,1,1,
1,1,1,1,1,1,1,1,1,1,1,1,1,1,1,1,1,1,1,1,1,1,1,1,1,1,1,1,1,1,1,1,1,1,1,1,
1,1,1,1,1,1,1,1,1,1,1,1,1,1,1,1,1,1,1,1,1,1,1,1,1,1,1,1,1,1,1,1,1,1,1,1,
1,1,1,1,1,1,1,1,1,1,1,1,1,1,1,1,1,1,1,1,1,1,1,1,1,1,1,1,1,1,1,1,1,1,1,1,
1,1,1,1,1,1,1,1,1,1,1,1,1,1,1,1,1,1,1,1,1,1,1,1,1,1,1,1,1,1,1,1,1,1,1,1,
1,1,1,1,1,1,1,1,1,1,1,1,1,1,1,1,1,1,1,1,1,1,1,1,1,1,1,1,1,1,1,1,1,1,1,1,
1,1,1,1,1,1,1,1,1,1,1,1,1,1,1,1,1,1,1,1,1,1,1,1,1,1,1,1,1,1,1,1,1,1,1,1,
1,1,1,1,1,1,1,1,1,1,1,1,1,1,1,1,1,1,1,1,1,1,1,1,1,1,1,1,1,1,1,1,1,1,1,1,
1,1,1,1,1,1,1,1,1,1,1,1,1,1,1,1,1,1,1,1,1,1,1,1,1,1,1,1,1,1,1,1,1,1,1,1,
1,1,1,1,1,1,1,1,1,1,1,1,1,1,1,1,1,1,1,1,1,1,1,1,1,1,1,1,1,1,1,1,1,1,1,1,
1,1,1,1,1,1,1,1,1,1,1,1,1,1,1,1,1,1,1,1,1,1,1,1,1,1,1,1,1,1,1,1,1,1,1,1,
1,1,1,1,1,1,1,1,1,1,1,1,1,1,1,1,1,1,1,1,1,1,1,1,1,1,1,1,1,1,1,1,1,1,1,1,
1,1,1,1,1,1,1,1,1,1,1,1,1,1,1,1,1,1,1,1,1,1,1,1,1,1,1,1,1,1,1,1,1,1,1,1,
1,1,1,1,1,1,1,1,1,1,1,1,1,1,1,1,1,1,1,1,1,1,1,1,1,1,1,1,1,1,1,1,1,1,1,1,
1,1,1,1,1,1,1,1,1,1,1,1,1,1,1,1,1,1,1,1,1,1,1,1,1,1,1,1,1,1,1,1,1,1,1,1,
1,1,1,1,1,1,1,1,1,1,1,1,1,1,1,1,1,1,1,1,1,1,1,1,1,1,1,1,1,1,1,1,1,1,1,1,
1,1,1,1,1,1,1,1,1,1,1,1,1,1,1,1,1,1,1,1,1,1,1,1,1,1,1,1,1,1,1,1,1,1,1,1,
1,1,1,1,1,1,1,1,1,1,1,1,1,1,1,1,1,1,1,1,1,1,1,1,1,1,1,1,1,1,1,1,1,1,1,1,
1,1,1,1,1,1,1,1,1,1,1,1,1,1,1,1,1,1,1,1,1,1,1,1,1,1,1,1,1,1,1,1,1,1,1,1,
1,1,1,1,1,1,1,1,1,1,1,1,1,1,1,1,1,1,1,1,1,1,1,1,1,1,1,1,1,1,1,1,1,1,1,1,
1,1,1,1,1,1,1,1,1,1,1,1,1,1,1,1,1,1,1,1,1,1,1,1,1,1,1,1,1,1,1,1,1,1,1,1,
1,1,1,1,1,1,1,1,1,1,1,1,1,1,1,1,1,1,1,1,1,1,1,1,1,1,1,1,1,1,1,1,1,1,1,1,
1,1,1,1,1,1,1,1,1,1,1,1,1,1,1,1,1,1,1,1,1,1,1,1,1,1,1,1,1,1,1,1,1,1,1,1,
1,1,1,1,1,1,1,1,1,1,1,1,1,1,1,1,1,1,1,1,1,1,1,1,1,1,1,1,1,1,1,1,1,1,1,1,
1,1,1,1,1,1,1,1,1,1,1,1,1,1,1,1,1,1,1,1,1,1,1,1,1,1,1,1,1,1,1,1,1,1,1,1,
1,1,1,1,1,1,1,1,1,1,1,1,1,1,1,1,1,1,1,1,1,1,1,1,1,1,1,1,1,1,1,1,1,1,1,1,
1,1,1,1,1,1,1,1,1,1,1,1,1,1,1,1,1,1,1,1,1,1,1,1,1,1,1,1,1,1,1,1,1,1,1,1,
1,1,1,1,1,1,1,1,1,1,1,1,1,1,1,1,1,1,1,1,1,1,1,1,1,1,1,1,1,1,1,1,1,1,1,1,
1,1,1,1,1,1,1,1,1,1,1,1,1,1,1,1,1,1,1,1,1,1,1,1,1,1,1,1,1,1,1,1,1,1,1,1,
1,1,1,1,1,1,1,1,1,1,1,1,1,1,1,1,1,1,1,1,1,1,1,1,1,1,1,1,1,1,1,1,1,1,1,1,
1,1,1,1,1,1,1,1,1,1,1,1,1,1,1,1,1,1,1,1,1,1,1,1,1,1,1,1,1,1,1,1,1,1,1,1,
1,1,1,1,1,1,1,1,1,1,1,1,1,1,1,1,1,1,1,1,1,1,1,1,1,1,1,1,1,1,1,1,1,1,1,1,
1,1,1,1,1,1,1,1,1,1,1,1,1,1,1,1,1,1,1,1,1,1,1,1,1,1,1,1,1,1,1,1,1,1,1,1,
1,1,1,1,1,1,1,1,1,1,1,1,1,1,1,1,1,1,1,1,1,1,1,1,1,1,1,1,1,1,1,1,1,1,1,1,
1,1,1,1,1,1,1,1,1,1,1,1,1,1,1,1,1,1,1,1,1,1,1,1,1,1,1,1,1,1,1,1,1,1,1,1,
1,1,1,1,1,1,1,1,1,1,1,1,1,1,1,1,1,1,1,1,1,1,1,1,1,1,1,1,1,1,1,1,1,1,1,1,
1,1,1,1,1,1,1,1,1,1,1,1,1,1,1,1,1,1,1,1,1,1,1,1,1,1,1,1,1,1,1,1,1,1,1,1,
1,1,1,1,1,1,1,1,1,1,1,1,1,1,1,1,1,1,1,1,1,1,1,1,1,1,1,1,1,1,1,1,1,1,1,1,
1,1,1,1,1,1,1,1,1,1,1,1,1,1,1,1,1,1,1,1,1,1,1,1,1,1,1,1,1,1,1,1,1,1,1,1,
1,1,1,1,1,1,1,1,1,1,1,1,1,1,1,1,1,1,1,1,1,1,1,1,1,1,1,1,1,1,1,1,1,1,1,1,
1,1,1,1,1,1,1,1,1,1,1,1,1,1,1,1,1,1,1,1,1,1,1,1,1,1,1,1,1,1,1,1,1,1,1,1,
1,1,1,1,1,1,1,1,1,1,1,1,1,1,1,1,1,4),(-0.000423095957202541,0.115881565465356),
(11.6153146011728,12.1152895244478,12.6151575298078,13.614893540528,14.6146295512481,
15.6143655619682,16.6141015726884,17.6138375834085,18.6135735941286,19.6133096048488,
20.6130456155689,21.612781626289,22.6125176370092,23.6122536477293,24.6119896584494,
25.6117256691696,26.6114616798897,27.6111976906098,28.6109337013299,29.6106697120501,
30.6104057227702,31.6101417334903,32.6098777442105,33.6096137549306,34.6093497656507,
35.6090857763709,36.608821787091,37.6085577978111,38.6082938085313,39.6080298192514,
40.6077658299715,41.6075018406916,42.6072378514118,43.6069738621319,44.606709872852,
45.6064458835722,46.6061818942923,47.6059179050124,48.6056539157326,49.6053899264527,
50.6051259371728,51.604861947893,52.6045979586131,53.6043339693332,54.6040699800534,
55.6038059907735,56.6035420014936,57.6032780122137,58.6030140229339,59.602750033654,
60.6024860443741,61.6022220550943,62.6019580658144,63.6016940765345,64.6014300872547,
65.6011660979748,66.6009021086949,67.6006381194151,68.6003741301352,69.6001101408553,
70.5998461515754,71.5995821622956,72.5993181730157,73.5990541837358,74.598790194456,
75.5985262051761,76.5982622158962,77.5979982266164,78.5977342373365,79.5974702480566,
80.5972062587768,81.5969422694969,82.596678280217,83.5964142909372,84.5961503016573,
85.5958863123774,86.5956223230975,87.5953583338177,88.5950943445378,89.5948303552579,
90.5945663659781,91.5943023766982,92.5940383874183,93.5937743981385,94.5935104088586,
95.5932464195787,96.5929824302989,97.592718441019,98.5924544517391,99.5921904624593,
100.591926473179,101.5916624839,102.59139849462,103.59113450534,104.59087051606,
105.59060652678,106.5903425375,107.59007854822,108.58981455894,109.589550569661,
110.589286580381,111.589022591101,112.588758601821,113.588494612541,114.588230623261,
115.587966633981,116.587702644701,117.587438655422,118.587174666142,119.586910676862,
120.586646687582,121.586382698302,122.586118709022,123.585854719742,124.585590730463,
125.585326741183,126.585062751903,127.584798762623,128.584534773343,129.584270784063,
130.584006794783,131.583742805503,132.583478816224,133.583214826944,134.582950837664,
135.582686848384,136.582422859104,137.582158869824,138.581894880544,139.581630891264,
140.581366901985,141.581102912705,142.580838923425,143.580574934145,144.580310944865,
145.580046955585,146.579782966305,147.579518977026,148.579254987746,149.578990998466,
150.578727009186,151.578463019906,152.578199030626,153.577935041346,154.577671052066,
155.577407062787,156.577143073507,157.576879084227,158.576615094947,159.576351105667,
160.576087116387,161.575823127107,162.575559137827,163.575295148548,164.575031159268,
165.574767169988,166.574503180708,167.574239191428,168.573975202148,169.573711212868,
170.573447223589,171.573183234309,172.572919245029,173.572655255749,174.572391266469,
175.572127277189,176.571863287909,177.571599298629,178.57133530935,179.57107132007,
180.57080733079,181.57054334151,182.57027935223,183.57001536295,184.56975137367,
185.56948738439,186.569223395111,187.568959405831,188.568695416551,189.568431427271,
190.568167437991,191.567903448711,192.567639459431,193.567375470152,194.567111480872,
195.566847491592,196.566583502312,197.566319513032,198.566055523752,199.565791534472,
200.565527545192,201.565263555913,202.564999566633,203.564735577353,204.564471588073,
205.564207598793,206.563943609513,207.563679620233,208.563415630954,209.563151641674,
210.562887652394,211.562623663114,212.562359673834,213.562095684554,214.561831695274,
215.561567705994,216.561303716715,217.561039727435,218.560775738155,219.560511748875,
220.560247759595,221.559983770315,222.559719781035,223.559455791755,224.559191802476,
225.558927813196,226.558663823916,227.558399834636,228.558135845356,229.557871856076,
230.557607866796,231.557343877517,232.557079888237,233.556815898957,234.556551909677,
235.556287920397,236.556023931117,237.555759941837,238.555495952557,239.555231963278,
240.554967973998,241.554703984718,242.554439995438,243.554176006158,244.553912016878,
245.553648027598,246.553384038319,247.553120049039,248.552856059759,249.552592070479,
250.552328081199,251.552064091919,252.551800102639,253.551536113359,254.55127212408,
255.5510081348,256.55074414552,257.55048015624,258.55021616696,259.54995217768,
260.5496881884,261.54942419912,262.549160209841,263.548896220561,264.548632231281,
265.548368242001,266.548104252721,267.547840263441,268.547576274161,269.547312284882,
270.547048295602,271.546784306322,272.546520317042,273.546256327762,274.545992338482,
275.545728349202,276.545464359922,277.545200370643,278.544936381363,279.544672392083,
280.544408402803,281.544144413523,282.543880424243,283.543616434963,284.543352445683,
285.543088456404,286.542824467124,287.542560477844,288.542296488564,289.542032499284,
290.541768510004,291.541504520724,292.541240531445,293.540976542165,294.540712552885,
295.540448563605,296.540184574325,297.539920585045,298.539656595765,299.539392606485,
300.539128617206,301.538864627926,302.538600638646,303.538336649366,304.538072660086,
305.537808670806,306.537544681526,307.537280692246,308.537016702967,309.536752713687,
310.536488724407,311.536224735127,312.535960745847,313.535696756567,314.535432767287,
315.535168778008,316.534904788728,317.534640799448,318.534376810168,319.534112820888,
320.533848831608,321.533584842328,322.533320853048,323.533056863769,324.532792874489,
325.532528885209,326.532264895929,327.532000906649,328.531736917369,329.531472928089,
330.53120893881,331.53094494953,332.53068096025,333.53041697097,334.53015298169,
335.52988899241,336.52962500313,337.52936101385,338.529097024571,339.528833035291,
340.528569046011,341.528305056731,342.528041067451,343.527777078171,344.527513088891,
345.527249099611,346.526985110332,347.526721121052,348.526457131772,349.526193142492,
350.525929153212,351.525665163932,352.525401174652,353.525137185373,354.524873196093,
355.524609206813,356.524345217533,357.524081228253,358.523817238973,359.523553249693,
360.523289260413,361.523025271134,362.522761281854,363.522497292574,364.522233303294,
365.521969314014,366.521705324734,367.521441335454,368.521177346175,369.520913356895,
370.520649367615,371.520385378335,372.520121389055,373.519857399775,374.519593410495,
375.519329421215,376.519065431936,377.518801442656,378.518537453376,379.518273464096,
380.518009474816,381.517745485536,382.517481496256,383.517217506976,384.516953517697,
385.516689528417,386.516425539137,387.516161549857,388.515897560577,389.515633571297,
390.515369582017,391.515105592737,392.514841603458,393.514577614178,394.514313624898,
395.514049635618,396.513785646338,397.513521657058,398.513257667778,399.512993678499,
400.512729689219,401.512465699939,402.512201710659,403.511937721379,404.511673732099,
405.511409742819,406.511145753539,407.51088176426,408.51061777498,409.5103537857,
410.51008979642,411.50982580714,412.50956181786,413.50929782858,414.509033839301,
415.508769850021,416.508505860741,417.508241871461,418.507977882181,419.507713892901,
420.507449903621,421.507185914341,422.506921925062,423.506657935782,424.506393946502,
425.506129957222,426.505865967942,427.505601978662,428.505337989382,429.505074000102,
430.504810010823,431.504546021543,432.504282032263,433.504018042983,434.503754053703,
435.503490064423,436.503226075143,437.502962085864,438.502698096584,439.502434107304,
440.502170118024,441.501906128744,442.501642139464,443.501378150184,444.501114160904,
445.500850171625,446.500586182345,447.500322193065,448.500058203785,449.499794214505,
450.499530225225,451.499266235945,452.499002246665,453.498738257386,454.498474268106,
455.498210278826,456.497946289546,457.497682300266,458.497418310986,459.497154321706,
460.496890332427,461.496626343147,462.496362353867,463.496098364587,464.495834375307,
465.495570386027,466.495306396747,467.495042407467,468.494778418188,469.494514428908,
470.494250439628,471.493986450348,472.493722461068,473.493458471788,474.493194482508,
475.492930493229,476.492666503949,477.492402514669,478.492138525389,479.491874536109,
480.491610546829,481.491346557549,482.491082568269,483.49081857899,484.49055458971,
485.49029060043,486.49002661115,487.48976262187,488.48949863259,489.48923464331,
490.48897065403,491.488706664751,492.488442675471,493.488178686191,494.487914696911,
495.487650707631,496.487386718351,497.487122729071,498.486858739792,499.486594750512,
500.486330761232,501.486066771952,502.485802782672,503.485538793392,504.485274804112,
505.485010814832,506.484746825553,507.484482836273,508.484218846993,509.483954857713,
510.483690868433,511.483426879153,512.483162889873,513.482898900594,514.482634911314,
515.482370922034,516.482106932754,517.481842943474,518.481578954194,519.481314964914,
520.481050975635,521.480786986355,522.480522997075,523.480259007795,524.479995018515,
525.479731029235,526.479467039955,527.479203050675,528.478939061396,529.478675072116,
530.478411082836,531.478147093556,532.477883104276,533.477619114996,534.477355125716,
535.477091136436,536.476827147157,537.476563157877,538.476299168597,539.476035179317,
540.475771190037,541.475507200757,542.475243211477,543.474979222197,544.474715232918,
545.474451243638,546.474187254358,547.473923265078,548.473659275798,549.473395286518,
550.473131297238,551.472867307958,552.472603318679,553.472339329399,554.472075340119,
555.471811350839,556.471547361559,557.471283372279,558.471019382999,559.47075539372,
560.47049140444,561.47022741516,562.46996342588,563.4696994366,564.46943544732,
565.46917145804,566.46890746876,567.468643479481,568.468379490201,569.468115500921,
570.467851511641,571.467587522361,572.467323533081,573.467059543801,574.466795554521,
575.466531565242,576.466267575962,577.466003586682,578.465739597402,579.465475608122,
580.465211618842,581.464947629562,582.464683640283,583.464419651003,584.464155661723,
585.463891672443,586.463627683163,587.463363693883,588.463099704603,589.462835715323,
590.462571726044,591.462307736764,592.462043747484,593.461779758204,594.461515768924,
595.461251779644,596.460987790364,597.460723801085,598.460459811805,599.460195822525,
600.459931833245,601.459667843965,602.459403854685,603.459139865405,604.458875876125,
605.458611886846,606.458347897566,607.458083908286,608.457819919006,609.457555929726,
610.457291940446,611.457027951166,612.456763961887,613.456499972607,614.456235983327,
615.455971994047,616.455708004767,617.455444015487,618.455180026207,619.454916036927,
620.454652047648,621.454388058368,622.454124069088,623.453860079808,624.453596090528,
625.453332101248,626.453068111968,627.452804122688,628.452540133409,629.452276144129,
630.452012154849,631.451748165569,632.451484176289,633.451220187009,634.450956197729,
635.450692208449,636.45042821917,637.45016422989,638.44990024061,639.44963625133,
640.44937226205,641.44910827277,642.44884428349,643.448580294211,644.448316304931,
645.448052315651,646.447788326371,647.447524337091,648.447260347811,649.446996358531,
650.446732369251,651.446468379972,652.446204390692,653.445940401412,654.445676412132,
655.445412422852,656.445148433572,657.444884444292,658.444620455012,659.444356465733,
660.444092476453,661.443828487173,662.443564497893,663.443300508613,664.443036519333,
665.442772530053,666.442508540774,667.442244551494,668.441980562214,669.441716572934,
670.441452583654,671.441188594374,672.440924605094,673.440660615815,674.440396626535,
675.440132637255,676.439868647975,677.439604658695,678.439340669415,679.439076680135,
680.438812690855,681.438548701576,682.438284712296,683.438020723016,684.437756733736,
685.437492744456,686.437228755176,687.436964765896,688.436700776616,689.436436787337,
690.436172798057,691.435908808777,692.435644819497,693.435380830217,694.435116840937,
695.434852851657,696.434588862377,697.434324873098,698.434060883818,699.433796894538,
700.433532905258,701.433268915978,702.433004926698,703.432740937418,704.432476948139,
705.432212958859,706.431948969579,707.431684980299,708.431420991019,709.431157001739,
710.430893012459,711.430629023179,712.4303650339,713.43010104462,714.42983705534,
715.42957306606,716.42930907678,717.4290450875,718.42878109822,719.42851710894,
720.428253119661,721.427989130381,722.427725141101,723.427461151821,724.427197162541,
725.426933173261,726.426669183981,727.426405194702,728.426141205422,729.425877216142,
730.425613226862,731.425349237582,732.425085248302,733.424821259022,734.424557269742,
735.424293280463,736.424029291183,737.423765301903,738.423501312623,739.423237323343,
740.422973334063,741.422709344783,742.422445355504,743.422181366224,744.421917376944,
745.421653387664,746.421389398384,747.421125409104,748.420861419824,749.420597430544,
750.420333441265,751.420069451985,752.419805462705,753.419541473425,754.419277484145,
755.419013494865,756.418749505585,757.418485516306,758.418221527026,759.417957537746,
760.417693548466,761.417429559186,762.417165569906,763.416901580626,764.416637591346,
765.416373602067,766.416109612787,767.415845623507,768.415581634227,769.415317644947,
770.415053655667,771.414789666387,772.414525677107,773.414261687828,774.413997698548,
775.413733709268,776.413469719988,777.413205730708,778.412941741428,779.412677752148,
780.412413762868,781.412149773589,782.411885784309,783.411621795029,784.411357805749,
785.411093816469,786.410829827189,787.410565837909,788.41030184863,789.41003785935,
790.40977387007,791.40950988079,792.40924589151,793.40898190223,794.40871791295,
795.40845392367,796.408189934391,797.407925945111,798.407661955831,799.407397966551,
800.407133977271,801.406869987991,802.406605998711,803.406342009432,804.406078020152,
805.405814030872,806.405550041592,807.405286052312,808.405022063032,809.404758073752,
810.404494084472,811.404230095193,812.403966105913,813.403702116633,814.403438127353,
815.403174138073,816.402910148793,817.402646159513,818.402382170234,819.402118180954,
820.401854191674,821.401590202394,822.401326213114,823.401062223834,824.400798234554,
825.400534245274,826.400270255995,827.400006266715,828.399742277435,829.399478288155,
830.399214298875,831.398950309595,832.398686320315,833.398422331035,834.398158341756,
835.397894352476,836.397630363196,837.397366373916,838.397102384636,839.396838395356,
840.396574406076,841.396310416796,842.396046427517,843.395782438237,844.395518448957,
845.395254459677,846.394990470397,847.394726481117,848.394462491837,849.394198502558,
850.393934513278,851.393670523998,852.393406534718,853.393142545438,854.392878556158,
855.392614566878,856.392350577598,857.392086588319,858.391822599039,859.391558609759,
860.391294620479,861.391030631199,862.390766641919,863.390502652639,864.390238663359,
865.38997467408,866.3897106848,867.38944669552,868.38918270624,869.38891871696,
870.38865472768,871.3883907384,872.388126749121,873.387862759841,874.387598770561,
875.387334781281,876.387070792001,877.386806802721,878.386542813441,879.386278824161,
880.386014834882,881.385750845602,882.385486856322,883.385222867042,884.384958877762,
885.384694888482,886.384430899202,887.384166909923,888.383902920643,889.383638931363,
890.383374942083,891.383110952803,892.382846963523,893.382582974243,894.382318984963,
895.382054995684,896.381791006404,897.381527017124,898.381263027844,899.380999038564,
900.380735049284,901.380471060004,902.380207070725,903.379943081445,904.379679092165,
905.379415102885,906.379151113605,907.378887124325,908.378623135045,909.378359145765,
910.378095156486,911.377831167206,912.377567177926,913.377303188646,914.377039199366,
915.376775210086,916.376511220806,917.376247231526,918.375983242247,919.375719252967,
920.375455263687,921.375191274407,922.374927285127,923.374663295847,924.374399306567,
925.374135317287,926.373871328008,927.373607338728,928.373343349448,929.373079360168,
930.372815370888,931.372551381608,932.372287392328,933.372023403049,934.371759413769,
935.371495424489,936.371231435209,937.370967445929,938.370703456649,939.370439467369,
940.370175478089,941.36991148881,942.36964749953,943.36938351025,944.36911952097,
945.36885553169,946.36859154241,947.36832755313,948.368063563851,949.367799574571,
950.367535585291,951.367271596011,952.367007606731,953.366743617451,954.366479628171,
955.366215638891,956.365951649612,957.365687660332,958.365423671052,959.365159681772,
960.364895692492,961.364631703212,962.364367713932,963.364103724653,964.363839735373,
965.363575746093,966.363311756813,967.363047767533,968.362783778253,969.362519788973,
970.362255799693,971.361991810414,972.361727821134,973.361463831854,974.361199842574,
975.360935853294,976.360671864014,977.360407874734,978.360143885454,979.359879896175,
980.359615906895,981.359351917615,982.359087928335,983.358823939055,984.358559949775,
985.358295960495,986.358031971215,987.357767981936,988.357503992656,989.357240003376,
990.356976014096,991.356712024816,992.356448035536,993.356184046256,994.355920056977,
995.355656067697,996.355392078417,997.355128089137,998.354864099857,999.354600110577,
1000.3543361213,1001.35407213202,1002.35380814274,1003.35354415346,1004.35328016418,
1005.3530161749,1006.35275218562,1007.35248819634,1008.35222420706,1009.35196021778,
1010.3516962285,1011.35143223922,1012.35116824994,1013.35090426066,1014.35064027138,
1015.3503762821,1016.35011229282,1017.34984830354,1018.34958431426,1019.34932032498,
1020.3490563357,1021.34879234642,1022.34852835714,1023.34826436786,1024.34800037858,
1025.3477363893,1026.34747240002,1027.34720841074,1028.34694442146,1029.34668043218,
1030.3464164429,1031.34615245362,1032.34588846434,1033.34562447506,1034.34536048578,
1035.3450964965,1036.34483250722,1037.34456851794,1038.34430452866,1039.34404053938,
1040.3437765501,1041.34351256082,1042.34324857154,1043.34298458226,1044.34272059298,
1045.3424566037,1046.34219261442,1047.34192862514,1048.34166463586,1049.34140064658,
1050.3411366573,1051.34087266802,1052.34060867874,1053.34034468946,1054.34008070018,
1055.3398167109,1056.33955272162,1057.33928873234,1058.33902474307,1059.33876075378,
1060.33849676451,1061.33823277523,1062.33796878595,1063.33770479667,1064.33744080739,
1065.33717681811,1066.33691282883,1067.33664883955,1068.33638485027,1069.33612086099,
1070.33585687171,1071.33559288243,1072.33532889315,1073.33506490387,1074.33480091459,
1075.33453692531,1076.33427293603,1077.33400894675,1078.33374495747,1079.33348096819,
1080.33321697891,1081.33295298963,1082.33268900035,1083.33242501107,1084.33216102179,
1085.33189703251,1086.33163304323,1087.33136905395,1088.33110506467,1089.33084107539,
1090.33057708611,1091.33031309683,1092.33004910755,1093.32978511827,1094.32952112899,
1095.32925713971,1096.32899315043,1097.32872916115,1098.32846517187,1099.32820118259,
1100.32793719331,1101.32767320403,1102.32740921475,1103.32714522547,1104.32688123619,
1105.32661724691,1106.32635325763,1107.32608926835,1108.32582527907,1109.32556128979,
1110.32529730051,1111.32503331123,1112.32476932195,1113.32450533267,1114.32424134339,
1115.32397735411,1116.32371336483,1117.32344937555,1118.32318538627,1119.32292139699,
1120.32265740771,1121.32239341843,1122.32212942915,1123.32186543987,1124.32160145059,
1125.32133746131,1126.32107347203,1127.32080948275,1128.32054549347,1129.32028150419,
1130.32001751491,1131.31975352563,1132.31948953635,1133.31922554707,1134.31896155779,
1135.31869756852,1136.31843357924,1137.31816958996,1138.31790560068,1139.3176416114,
1140.31737762212,1141.31711363284,1142.31684964356,1143.31658565428,1144.316321665,
1145.31605767572,1146.31579368644,1147.31552969716,1148.31526570788,1149.3150017186,
1150.31473772932,1151.31447374004,1152.31420975076,1153.31394576148,1154.3136817722,
1155.31341778292,1156.31315379364,1157.31288980436,1158.31262581508,1159.3123618258,
1160.31209783652,1161.31183384724,1162.31156985796,1163.31130586868,1164.3110418794,
1165.31077789012,1166.31051390084,1167.31024991156,1168.30998592228,1169.309721933,
1170.30945794372,1171.30919395444,1172.30892996516,1173.30866597588,1174.3084019866,
1175.30813799732,1176.30787400804,1177.30761001876,1178.30734602948,1179.3070820402,
1180.30681805092,1181.30655406164,1182.30629007236,1183.30602608308,1184.3057620938,
1185.30549810452,1186.30523411524,1187.30497012596,1188.30470613668,1189.3044421474,
1190.30417815812,1191.30391416884,1192.30365017956,1193.30338619028,1194.303122201,
1195.30285821172,1196.30259422244,1197.30233023316,1198.30206624388,1199.3018022546,
1200.30153826532,1201.30127427604,1202.30101028676,1203.30074629748,1204.3004823082,
1205.30021831892,1206.29995432964,1207.29969034036,1208.29942635108,1209.2991623618,
1210.29889837252,1211.29863438324,1212.29837039397,1213.29810640469,1214.29784241541,
1215.29757842613,1216.29731443685,1217.29705044757,1218.29678645829,1219.29652246901,
1220.29625847973,1221.29599449045,1222.29573050117,1223.29546651189,1224.29520252261,
1225.29493853333,1226.29467454405,1227.29441055477,1228.29414656549,1229.29388257621,
1230.29361858693,1231.29335459765,1232.29309060837,1233.29282661909,1234.29256262981,
1235.29229864053,1236.29203465125,1237.29177066197,1238.29150667269,1239.29124268341,
1240.29097869413,1241.29071470485,1242.29045071557,1243.29018672629,1244.28992273701,
1245.28965874773,1246.28939475845,1247.28913076917,1248.28886677989,1249.28860279061,
1250.28833880133,1251.28807481205,1252.28781082277,1253.28754683349,1254.28728284421,
1255.28701885493,1256.28675486565,1257.28649087637,1258.28622688709,1259.28596289781,
1260.28569890853,1261.28543491925,1262.28517092997,1263.28490694069,1264.28464295141,
1265.28437896213,1266.28411497285,1267.28385098357,1268.28358699429,1269.28332300501,
1270.28305901573,1271.28279502645,1272.28253103717,1273.28226704789,1274.28200305861,
1275.28173906933,1276.28147508005,1277.28121109077,1278.28094710149,1279.28068311221,
1280.28041912293,1281.28015513365,1282.27989114437,1283.27962715509,1284.27936316581,
1285.27909917653,1286.27883518725,1287.27857119797,1288.2783072087,1289.27804321942,
1290.27777923014,1291.27751524086,1292.27725125158,1293.2769872623,1294.27672327302,
1295.27645928374,1296.27619529446,1297.27593130518,1298.2756673159,1299.27540332662,
1300.27513933734,1301.27487534806,1302.27461135878,1303.2743473695,1304.27408338022,
1305.27381939094,1306.27355540166,1307.27329141238,1308.2730274231,1309.27276343382,
1310.27249944454,1311.27223545526,1312.27197146598,1313.2717074767,1314.27144348742,
1315.27117949814,1316.27091550886,1317.27065151958,1318.2703875303,1319.27012354102,
1320.26985955174,1321.26959556246,1322.26933157318,1323.2690675839,1324.26880359462,
1325.26853960534,1326.26827561606,1327.26801162678,1328.2677476375,1329.26748364822,
1330.26721965894,1331.26695566966,1332.26669168038,1333.2664276911,1334.26616370182,
1335.26589971254,1336.26563572326,1337.26537173398,1338.2651077447,1339.26484375542,
1340.26457976614,1341.26431577686,1342.26405178758,1343.2637877983,1344.26352380902,
1345.26325981974,1346.26299583046,1347.26273184118,1348.2624678519,1349.26220386262,
1350.26193987334,1351.26167588406,1352.26141189478,1353.2611479055,1354.26088391622,
1355.26061992694,1356.26035593766,1357.26009194838,1358.2598279591,1359.25956396982,
1360.25929998054,1361.25903599126,1362.25877200198,1363.2585080127,1364.25824402343,
1365.25798003415,1366.25771604487,1367.25745205559,1368.25718806631,1369.25692407703,
1370.25666008775,1371.25639609847,1372.25613210919,1373.25586811991,1374.25560413063,
1375.25534014135,1376.25507615207,1377.25481216279,1378.25454817351,1379.25428418423,
1380.25402019495,1381.25375620567,1382.25349221639,1383.25322822711,1384.25296423783,
1385.25270024855,1386.25243625927,1387.25217226999,1388.25190828071,1389.25164429143,
1390.25138030215,1391.25111631287,1392.25085232359,1393.25058833431,1394.25032434503,
1395.25006035575,1396.24979636647,1397.24953237719,1398.24926838791,1399.24900439863,
1400.24874040935,1401.24847642007,1402.24821243079,1403.24794844151,1404.24768445223,
1405.24742046295,1406.24715647367,1407.24689248439,1408.24662849511,1409.24636450583,
1410.24610051655,1411.24583652727,1412.24557253799,1413.24530854871,1414.24504455943,
1415.24478057015,1416.24451658087,1417.24425259159,1418.24398860231,1419.24372461303,
1420.24346062375,1421.24319663447,1422.24293264519,1423.24266865591,1424.24240466663,
1425.24214067735,1426.24187668807,1427.24161269879,1428.24134870951,1429.24108472023,
1430.24082073095,1431.24055674167,1432.24029275239,1433.24002876311,1434.23976477383,
1435.23950078455,1436.23923679527,1437.23897280599,1438.23870881671,1439.23844482743,
1440.23818083815,1441.23791684888,1442.2376528596,1443.23738887032,1444.23712488104,
1445.23686089176,1446.23659690248,1447.2363329132,1448.23606892392,1449.23580493464,
1450.23554094536,1451.23527695608,1452.2350129668,1453.23474897752,1454.23448498824,
1455.23422099896,1456.23395700968,1457.2336930204,1458.23342903112,1459.23316504184,
1460.23290105256,1461.23263706328,1462.232373074,1463.23210908472,1464.23184509544,
1465.23158110616,1466.23131711688,1467.2310531276,1468.23078913832,1469.23052514904,
1470.23026115976,1471.22999717048,1472.2297331812,1473.22946919192,1474.22920520264,
1475.22894121336,1476.22867722408,1477.2284132348,1478.22814924552,1479.22788525624,
1480.22762126696,1481.22735727768,1482.2270932884,1483.22682929912,1484.22656530984,
1485.22630132056,1486.22603733128,1487.225773342,1488.22550935272,1489.22524536344,
1490.22498137416,1491.22471738488,1492.2244533956,1493.22418940632,1494.22392541704,
1495.22366142776,1496.22339743848,1497.2231334492,1498.22286945992,1499.22260547064,
1500.22234148136,1501.22207749208,1502.2218135028,1503.22154951352,1504.22128552424,
1505.22102153496,1506.22075754568,1507.2204935564,1508.22022956712,1509.21996557784,
1510.21970158856,1511.21943759928,1512.21917361,1513.21890962072,1514.21864563144,
1515.21838164216,1516.21811765288,1517.21785366361,1518.21758967433,1519.21732568505,
1520.21706169577,1521.21679770649,1522.21653371721,1523.21626972793,1524.21600573865,
1525.21574174937,1526.21547776009,1527.21521377081,1528.21494978153,1529.21468579225,
1530.21442180297,1531.21415781369,1532.21389382441,1533.21362983513,1534.21336584585,
1535.21310185657,1536.21283786729,1537.21257387801,1538.21230988873,1539.21204589945,
1540.21178191017,1541.21151792089,1542.21125393161,1543.21098994233,1544.21072595305,
1545.21046196377,1546.21019797449,1547.20993398521,1548.20966999593,1549.20940600665,
1550.20914201737,1551.20887802809,1552.20861403881,1553.20835004953,1554.20808606025,
1555.20782207097,1556.20755808169,1557.20729409241,1558.20703010313,1559.20676611385,
1560.20650212457,1561.20623813529,1562.20597414601,1563.20571015673,1564.20544616745,
1565.20518217817,1566.20491818889,1567.20465419961,1568.20439021033,1569.20412622105,
1570.20386223177,1571.20359824249,1572.20333425321,1573.20307026393,1574.20280627465,
1575.20254228537,1576.20227829609,1577.20201430681,1578.20175031753,1579.20148632825,
1580.20122233897,1581.20095834969,1582.20069436041,1583.20043037113,1584.20016638185,
1585.19990239257,1586.19963840329,1587.19937441401,1588.19911042473,1589.19884643545,
1590.19858244617,1591.19831845689,1592.19805446761,1593.19779047834,1594.19752648906,
1595.19726249978,1596.1969985105,1597.19673452122,1598.19647053194,1599.19620654266,
1600.19594255338,1601.1956785641,1602.19541457482,1603.19515058554,1604.19488659626,
1605.19462260698,1606.1943586177,1607.19409462842,1608.19383063914,1609.19356664986,
1610.19330266058,1611.1930386713,1612.19277468202,1613.19251069274,1614.19224670346,
1615.19198271418,1616.1917187249,1617.19145473562,1618.19119074634,1619.19092675706,
1620.19066276778,1621.1903987785,1622.19013478922,1623.18987079994,1624.18960681066,
1625.18934282138,1626.1890788321,1627.18881484282,1628.18855085354,1629.18828686426,
1630.18802287498,1631.1877588857,1632.18749489642,1633.18723090714,1634.18696691786,
1635.18670292858,1636.1864389393,1637.18617495002,1638.18591096074,1639.18564697146,
1640.18538298218,1641.1851189929,1642.18485500362,1643.18459101434,1644.18432702506,
1645.18406303578,1646.1837990465,1647.18353505722,1648.18327106794,1649.18300707866,
1650.18274308938,1651.1824791001,1652.18221511082,1653.18195112154,1654.18168713226,
1655.18142314298,1656.1811591537,1657.18089516442,1658.18063117514,1659.18036718586,
1660.18010319658,1661.1798392073,1662.17957521802,1663.17931122874,1664.17904723946,
1665.17878325018,1666.1785192609,1667.17825527162,1668.17799128234,1669.17772729307,
1670.17746330379,1671.17719931451,1672.17693532523,1673.17667133595,1674.17640734667,
1675.17614335739,1676.17587936811,1677.17561537883,1678.17535138955,1679.17508740027,
1680.17482341099,1681.17455942171,1682.17429543243,1683.17403144315,1684.17376745387,
1685.17350346459,1686.17323947531,1687.17297548603,1688.17271149675,1689.17244750747,
1690.17218351819,1691.17191952891,1692.17165553963,1693.17139155035,1694.17112756107,
1695.17086357179,1696.17059958251,1697.17033559323,1698.17007160395,1699.16980761467,
1700.16954362539,1700.66941163075,1701.16959429301),.UNSPECIFIED.);
#51=B_SPLINE_SURFACE_WITH_KNOTS('',3,3,((#226317,#226318,#226319,#226320,
#226321,#226322,#226323,#226324,#226325,#226326,#226327,#226328,#226329,
#226330,#226331,#226332,#226333,#226334,#226335,#226336,#226337,#226338,
#226339,#226340,#226341,#226342,#226343,#226344,#226345,#226346,#226347,
#226348,#226349,#226350,#226351,#226352,#226353,#226354,#226355,#226356,
#226357,#226358,#226359,#226360,#226361,#226362,#226363,#226364,#226365,
#226366,#226367,#226368,#226369,#226370,#226371,#226372,#226373,#226374,
#226375,#226376,#226377,#226378,#226379,#226380,#226381,#226382,#226383,
#226384,#226385,#226386,#226387,#226388,#226389,#226390,#226391,#226392,
#226393,#226394,#226395,#226396,#226397,#226398,#226399,#226400,#226401,
#226402,#226403,#226404,#226405,#226406,#226407,#226408,#226409,#226410,
#226411,#226412,#226413,#226414,#226415,#226416,#226417,#226418,#226419,
#226420,#226421,#226422,#226423,#226424,#226425,#226426,#226427,#226428,
#226429,#226430,#226431,#226432,#226433,#226434,#226435,#226436,#226437,
#226438,#226439,#226440,#226441,#226442,#226443,#226444,#226445,#226446,
#226447,#226448,#226449,#226450,#226451,#226452,#226453,#226454,#226455,
#226456,#226457,#226458,#226459,#226460,#226461,#226462,#226463,#226464,
#226465,#226466,#226467,#226468,#226469,#226470,#226471,#226472,#226473,
#226474,#226475,#226476,#226477,#226478,#226479,#226480,#226481,#226482,
#226483,#226484,#226485,#226486,#226487,#226488,#226489,#226490,#226491,
#226492,#226493,#226494,#226495,#226496,#226497,#226498,#226499,#226500,
#226501,#226502,#226503,#226504,#226505,#226506,#226507,#226508,#226509,
#226510,#226511,#226512,#226513,#226514,#226515,#226516,#226517,#226518,
#226519,#226520,#226521,#226522,#226523,#226524,#226525,#226526,#226527,
#226528,#226529,#226530,#226531,#226532,#226533,#226534,#226535,#226536,
#226537,#226538,#226539,#226540,#226541,#226542,#226543,#226544,#226545,
#226546,#226547,#226548,#226549,#226550,#226551,#226552,#226553,#226554,
#226555,#226556,#226557,#226558,#226559,#226560,#226561,#226562,#226563,
#226564,#226565,#226566,#226567,#226568,#226569,#226570,#226571,#226572,
#226573,#226574,#226575,#226576,#226577,#226578,#226579,#226580,#226581,
#226582,#226583,#226584,#226585,#226586,#226587,#226588,#226589,#226590,
#226591,#226592,#226593,#226594,#226595,#226596,#226597,#226598,#226599,
#226600,#226601,#226602,#226603,#226604,#226605,#226606,#226607,#226608,
#226609,#226610,#226611,#226612,#226613,#226614,#226615,#226616,#226617,
#226618,#226619,#226620,#226621,#226622,#226623,#226624,#226625,#226626,
#226627,#226628,#226629,#226630,#226631,#226632,#226633,#226634,#226635,
#226636,#226637,#226638,#226639,#226640,#226641,#226642,#226643,#226644,
#226645,#226646,#226647,#226648,#226649,#226650,#226651,#226652,#226653,
#226654,#226655,#226656,#226657,#226658,#226659,#226660,#226661,#226662,
#226663,#226664,#226665,#226666,#226667,#226668,#226669,#226670,#226671,
#226672,#226673,#226674,#226675,#226676,#226677,#226678,#226679,#226680,
#226681,#226682,#226683,#226684,#226685,#226686,#226687,#226688,#226689,
#226690,#226691,#226692,#226693,#226694,#226695,#226696,#226697,#226698,
#226699,#226700,#226701,#226702,#226703,#226704,#226705,#226706,#226707,
#226708,#226709,#226710,#226711,#226712,#226713,#226714,#226715,#226716,
#226717,#226718,#226719,#226720,#226721,#226722,#226723,#226724,#226725,
#226726,#226727,#226728,#226729,#226730,#226731,#226732,#226733,#226734,
#226735,#226736,#226737,#226738,#226739,#226740,#226741,#226742,#226743,
#226744,#226745,#226746,#226747,#226748,#226749,#226750,#226751,#226752,
#226753,#226754,#226755,#226756,#226757,#226758,#226759,#226760,#226761,
#226762,#226763,#226764,#226765,#226766,#226767,#226768,#226769,#226770,
#226771,#226772,#226773,#226774,#226775,#226776,#226777,#226778,#226779,
#226780,#226781,#226782,#226783,#226784,#226785,#226786,#226787,#226788,
#226789,#226790,#226791,#226792,#226793,#226794,#226795,#226796,#226797,
#226798,#226799,#226800,#226801,#226802,#226803,#226804,#226805,#226806,
#226807,#226808,#226809,#226810,#226811,#226812,#226813,#226814,#226815,
#226816,#226817,#226818,#226819,#226820,#226821,#226822,#226823,#226824,
#226825,#226826,#226827,#226828,#226829,#226830,#226831,#226832,#226833,
#226834,#226835,#226836,#226837,#226838,#226839,#226840,#226841,#226842,
#226843,#226844,#226845,#226846,#226847,#226848,#226849,#226850,#226851,
#226852,#226853,#226854,#226855,#226856,#226857,#226858,#226859,#226860,
#226861,#226862,#226863,#226864,#226865,#226866,#226867,#226868,#226869,
#226870,#226871,#226872,#226873,#226874,#226875,#226876,#226877,#226878,
#226879,#226880,#226881,#226882,#226883,#226884,#226885,#226886,#226887,
#226888,#226889,#226890,#226891,#226892,#226893,#226894,#226895,#226896,
#226897,#226898,#226899,#226900,#226901,#226902,#226903,#226904,#226905,
#226906,#226907,#226908,#226909,#226910,#226911,#226912,#226913,#226914,
#226915,#226916,#226917,#226918,#226919,#226920,#226921,#226922,#226923,
#226924,#226925,#226926,#226927,#226928,#226929,#226930,#226931,#226932,
#226933,#226934,#226935,#226936,#226937,#226938,#226939,#226940,#226941,
#226942,#226943,#226944,#226945,#226946,#226947,#226948,#226949,#226950,
#226951,#226952,#226953,#226954,#226955,#226956,#226957,#226958,#226959,
#226960,#226961,#226962,#226963,#226964,#226965,#226966,#226967,#226968,
#226969,#226970,#226971,#226972,#226973,#226974,#226975,#226976,#226977,
#226978,#226979,#226980,#226981,#226982,#226983,#226984,#226985,#226986,
#226987,#226988,#226989,#226990,#226991,#226992,#226993,#226994,#226995,
#226996,#226997,#226998,#226999,#227000,#227001,#227002,#227003,#227004,
#227005,#227006,#227007,#227008,#227009,#227010,#227011,#227012,#227013,
#227014,#227015,#227016,#227017,#227018,#227019,#227020,#227021,#227022,
#227023,#227024,#227025,#227026,#227027,#227028,#227029,#227030,#227031,
#227032,#227033,#227034,#227035,#227036,#227037,#227038,#227039,#227040,
#227041,#227042,#227043,#227044,#227045,#227046,#227047,#227048,#227049,
#227050,#227051,#227052,#227053,#227054,#227055,#227056,#227057,#227058,
#227059,#227060,#227061,#227062,#227063,#227064,#227065,#227066,#227067,
#227068,#227069,#227070,#227071,#227072,#227073,#227074,#227075,#227076,
#227077,#227078,#227079,#227080,#227081,#227082,#227083,#227084,#227085,
#227086,#227087,#227088,#227089,#227090,#227091,#227092,#227093,#227094,
#227095,#227096,#227097,#227098,#227099,#227100,#227101,#227102,#227103,
#227104,#227105,#227106,#227107,#227108,#227109,#227110,#227111,#227112,
#227113,#227114,#227115,#227116,#227117,#227118,#227119,#227120,#227121,
#227122,#227123,#227124,#227125,#227126,#227127,#227128,#227129,#227130,
#227131,#227132,#227133,#227134,#227135,#227136,#227137,#227138,#227139,
#227140,#227141,#227142,#227143,#227144,#227145,#227146,#227147,#227148,
#227149,#227150,#227151,#227152,#227153,#227154,#227155,#227156,#227157,
#227158,#227159,#227160,#227161,#227162,#227163,#227164,#227165,#227166,
#227167,#227168,#227169,#227170,#227171,#227172,#227173,#227174,#227175,
#227176,#227177,#227178,#227179,#227180,#227181,#227182,#227183,#227184,
#227185,#227186,#227187,#227188,#227189,#227190,#227191,#227192,#227193,
#227194,#227195,#227196,#227197,#227198,#227199,#227200,#227201,#227202,
#227203,#227204,#227205,#227206,#227207,#227208,#227209,#227210,#227211,
#227212,#227213,#227214,#227215,#227216,#227217,#227218,#227219,#227220,
#227221,#227222,#227223,#227224,#227225,#227226,#227227,#227228,#227229,
#227230,#227231,#227232,#227233,#227234,#227235,#227236,#227237,#227238,
#227239,#227240,#227241,#227242,#227243,#227244,#227245,#227246,#227247,
#227248,#227249,#227250,#227251,#227252,#227253,#227254,#227255,#227256,
#227257,#227258,#227259,#227260,#227261,#227262,#227263,#227264,#227265,
#227266,#227267,#227268,#227269,#227270,#227271,#227272,#227273,#227274,
#227275,#227276,#227277,#227278,#227279,#227280,#227281,#227282,#227283,
#227284,#227285,#227286,#227287,#227288,#227289,#227290,#227291,#227292,
#227293,#227294,#227295,#227296,#227297,#227298,#227299,#227300,#227301,
#227302,#227303,#227304,#227305,#227306,#227307,#227308,#227309,#227310,
#227311,#227312,#227313,#227314,#227315,#227316,#227317,#227318,#227319,
#227320,#227321,#227322,#227323,#227324,#227325,#227326,#227327,#227328,
#227329,#227330,#227331,#227332,#227333,#227334,#227335,#227336,#227337,
#227338,#227339,#227340,#227341,#227342,#227343,#227344,#227345,#227346,
#227347,#227348,#227349,#227350,#227351,#227352,#227353,#227354,#227355,
#227356,#227357,#227358,#227359,#227360,#227361,#227362,#227363,#227364,
#227365,#227366,#227367,#227368,#227369,#227370,#227371,#227372,#227373,
#227374,#227375,#227376,#227377,#227378,#227379,#227380,#227381,#227382,
#227383,#227384,#227385,#227386,#227387,#227388,#227389,#227390,#227391,
#227392,#227393,#227394,#227395,#227396,#227397,#227398,#227399,#227400,
#227401,#227402,#227403,#227404,#227405,#227406,#227407,#227408,#227409,
#227410,#227411,#227412,#227413,#227414,#227415,#227416,#227417,#227418,
#227419,#227420,#227421,#227422,#227423,#227424,#227425,#227426,#227427,
#227428,#227429,#227430,#227431,#227432,#227433,#227434,#227435,#227436,
#227437,#227438,#227439,#227440,#227441,#227442,#227443,#227444,#227445,
#227446,#227447,#227448,#227449,#227450,#227451,#227452,#227453,#227454,
#227455,#227456,#227457,#227458,#227459,#227460,#227461,#227462,#227463,
#227464,#227465,#227466,#227467,#227468,#227469,#227470,#227471,#227472,
#227473,#227474,#227475,#227476,#227477,#227478,#227479,#227480,#227481,
#227482,#227483,#227484,#227485,#227486,#227487,#227488,#227489,#227490,
#227491,#227492,#227493,#227494,#227495,#227496,#227497,#227498,#227499,
#227500,#227501,#227502,#227503,#227504,#227505,#227506,#227507,#227508,
#227509,#227510,#227511,#227512,#227513,#227514,#227515,#227516,#227517,
#227518,#227519,#227520,#227521,#227522,#227523,#227524,#227525,#227526,
#227527,#227528,#227529,#227530,#227531,#227532,#227533,#227534,#227535,
#227536,#227537,#227538,#227539,#227540,#227541,#227542,#227543,#227544,
#227545,#227546,#227547,#227548,#227549,#227550,#227551,#227552,#227553,
#227554,#227555,#227556,#227557,#227558,#227559,#227560,#227561,#227562,
#227563,#227564,#227565,#227566,#227567,#227568,#227569,#227570,#227571,
#227572,#227573,#227574,#227575,#227576,#227577,#227578,#227579,#227580,
#227581,#227582,#227583,#227584,#227585,#227586,#227587,#227588,#227589,
#227590,#227591,#227592,#227593,#227594,#227595,#227596,#227597,#227598,
#227599,#227600,#227601,#227602,#227603,#227604,#227605,#227606,#227607,
#227608,#227609,#227610,#227611,#227612,#227613,#227614,#227615,#227616,
#227617,#227618,#227619,#227620,#227621,#227622,#227623,#227624,#227625,
#227626,#227627,#227628,#227629,#227630,#227631,#227632,#227633,#227634,
#227635,#227636,#227637,#227638,#227639,#227640,#227641,#227642,#227643,
#227644,#227645,#227646,#227647,#227648,#227649,#227650,#227651,#227652,
#227653,#227654,#227655,#227656,#227657,#227658,#227659,#227660,#227661,
#227662,#227663,#227664,#227665,#227666,#227667,#227668,#227669,#227670,
#227671,#227672,#227673,#227674,#227675,#227676,#227677,#227678,#227679,
#227680,#227681,#227682,#227683,#227684,#227685,#227686,#227687,#227688,
#227689,#227690,#227691,#227692,#227693,#227694,#227695,#227696,#227697,
#227698,#227699,#227700,#227701,#227702,#227703,#227704,#227705,#227706,
#227707,#227708,#227709,#227710,#227711,#227712,#227713,#227714,#227715,
#227716,#227717,#227718,#227719,#227720,#227721,#227722,#227723,#227724,
#227725,#227726,#227727,#227728,#227729,#227730,#227731,#227732,#227733,
#227734,#227735,#227736,#227737,#227738,#227739,#227740,#227741,#227742,
#227743,#227744,#227745,#227746,#227747,#227748,#227749,#227750,#227751,
#227752,#227753,#227754,#227755,#227756,#227757,#227758,#227759,#227760,
#227761,#227762,#227763,#227764,#227765,#227766,#227767,#227768,#227769,
#227770,#227771,#227772,#227773,#227774,#227775,#227776,#227777,#227778,
#227779,#227780,#227781,#227782,#227783,#227784,#227785,#227786,#227787,
#227788,#227789,#227790,#227791,#227792,#227793,#227794,#227795,#227796,
#227797,#227798,#227799,#227800,#227801,#227802,#227803,#227804,#227805,
#227806,#227807,#227808,#227809,#227810,#227811,#227812,#227813,#227814,
#227815,#227816,#227817,#227818,#227819,#227820,#227821,#227822,#227823,
#227824,#227825,#227826,#227827,#227828,#227829,#227830,#227831,#227832,
#227833,#227834,#227835,#227836,#227837,#227838,#227839,#227840,#227841,
#227842,#227843,#227844,#227845,#227846,#227847,#227848,#227849,#227850,
#227851,#227852,#227853,#227854,#227855,#227856,#227857,#227858,#227859,
#227860,#227861,#227862,#227863,#227864,#227865,#227866,#227867,#227868,
#227869,#227870,#227871,#227872,#227873,#227874,#227875,#227876,#227877,
#227878,#227879,#227880,#227881,#227882,#227883,#227884,#227885,#227886,
#227887,#227888,#227889,#227890,#227891,#227892,#227893,#227894,#227895,
#227896,#227897,#227898,#227899,#227900,#227901,#227902,#227903,#227904,
#227905,#227906,#227907,#227908,#227909,#227910,#227911,#227912,#227913,
#227914,#227915,#227916,#227917,#227918,#227919,#227920,#227921,#227922,
#227923,#227924,#227925,#227926,#227927,#227928,#227929,#227930,#227931,
#227932,#227933,#227934,#227935,#227936,#227937,#227938,#227939,#227940,
#227941,#227942,#227943,#227944,#227945,#227946,#227947,#227948,#227949,
#227950,#227951,#227952,#227953,#227954,#227955,#227956,#227957,#227958,
#227959,#227960,#227961,#227962,#227963,#227964,#227965,#227966,#227967,
#227968,#227969,#227970,#227971,#227972,#227973,#227974,#227975,#227976,
#227977,#227978,#227979,#227980,#227981,#227982,#227983,#227984,#227985,
#227986,#227987,#227988,#227989,#227990,#227991,#227992,#227993,#227994,
#227995,#227996,#227997,#227998,#227999,#228000,#228001,#228002,#228003,
#228004,#228005,#228006,#228007,#228008,#228009,#228010,#228011),(#228012,
#228013,#228014,#228015,#228016,#228017,#228018,#228019,#228020,#228021,
#228022,#228023,#228024,#228025,#228026,#228027,#228028,#228029,#228030,
#228031,#228032,#228033,#228034,#228035,#228036,#228037,#228038,#228039,
#228040,#228041,#228042,#228043,#228044,#228045,#228046,#228047,#228048,
#228049,#228050,#228051,#228052,#228053,#228054,#228055,#228056,#228057,
#228058,#228059,#228060,#228061,#228062,#228063,#228064,#228065,#228066,
#228067,#228068,#228069,#228070,#228071,#228072,#228073,#228074,#228075,
#228076,#228077,#228078,#228079,#228080,#228081,#228082,#228083,#228084,
#228085,#228086,#228087,#228088,#228089,#228090,#228091,#228092,#228093,
#228094,#228095,#228096,#228097,#228098,#228099,#228100,#228101,#228102,
#228103,#228104,#228105,#228106,#228107,#228108,#228109,#228110,#228111,
#228112,#228113,#228114,#228115,#228116,#228117,#228118,#228119,#228120,
#228121,#228122,#228123,#228124,#228125,#228126,#228127,#228128,#228129,
#228130,#228131,#228132,#228133,#228134,#228135,#228136,#228137,#228138,
#228139,#228140,#228141,#228142,#228143,#228144,#228145,#228146,#228147,
#228148,#228149,#228150,#228151,#228152,#228153,#228154,#228155,#228156,
#228157,#228158,#228159,#228160,#228161,#228162,#228163,#228164,#228165,
#228166,#228167,#228168,#228169,#228170,#228171,#228172,#228173,#228174,
#228175,#228176,#228177,#228178,#228179,#228180,#228181,#228182,#228183,
#228184,#228185,#228186,#228187,#228188,#228189,#228190,#228191,#228192,
#228193,#228194,#228195,#228196,#228197,#228198,#228199,#228200,#228201,
#228202,#228203,#228204,#228205,#228206,#228207,#228208,#228209,#228210,
#228211,#228212,#228213,#228214,#228215,#228216,#228217,#228218,#228219,
#228220,#228221,#228222,#228223,#228224,#228225,#228226,#228227,#228228,
#228229,#228230,#228231,#228232,#228233,#228234,#228235,#228236,#228237,
#228238,#228239,#228240,#228241,#228242,#228243,#228244,#228245,#228246,
#228247,#228248,#228249,#228250,#228251,#228252,#228253,#228254,#228255,
#228256,#228257,#228258,#228259,#228260,#228261,#228262,#228263,#228264,
#228265,#228266,#228267,#228268,#228269,#228270,#228271,#228272,#228273,
#228274,#228275,#228276,#228277,#228278,#228279,#228280,#228281,#228282,
#228283,#228284,#228285,#228286,#228287,#228288,#228289,#228290,#228291,
#228292,#228293,#228294,#228295,#228296,#228297,#228298,#228299,#228300,
#228301,#228302,#228303,#228304,#228305,#228306,#228307,#228308,#228309,
#228310,#228311,#228312,#228313,#228314,#228315,#228316,#228317,#228318,
#228319,#228320,#228321,#228322,#228323,#228324,#228325,#228326,#228327,
#228328,#228329,#228330,#228331,#228332,#228333,#228334,#228335,#228336,
#228337,#228338,#228339,#228340,#228341,#228342,#228343,#228344,#228345,
#228346,#228347,#228348,#228349,#228350,#228351,#228352,#228353,#228354,
#228355,#228356,#228357,#228358,#228359,#228360,#228361,#228362,#228363,
#228364,#228365,#228366,#228367,#228368,#228369,#228370,#228371,#228372,
#228373,#228374,#228375,#228376,#228377,#228378,#228379,#228380,#228381,
#228382,#228383,#228384,#228385,#228386,#228387,#228388,#228389,#228390,
#228391,#228392,#228393,#228394,#228395,#228396,#228397,#228398,#228399,
#228400,#228401,#228402,#228403,#228404,#228405,#228406,#228407,#228408,
#228409,#228410,#228411,#228412,#228413,#228414,#228415,#228416,#228417,
#228418,#228419,#228420,#228421,#228422,#228423,#228424,#228425,#228426,
#228427,#228428,#228429,#228430,#228431,#228432,#228433,#228434,#228435,
#228436,#228437,#228438,#228439,#228440,#228441,#228442,#228443,#228444,
#228445,#228446,#228447,#228448,#228449,#228450,#228451,#228452,#228453,
#228454,#228455,#228456,#228457,#228458,#228459,#228460,#228461,#228462,
#228463,#228464,#228465,#228466,#228467,#228468,#228469,#228470,#228471,
#228472,#228473,#228474,#228475,#228476,#228477,#228478,#228479,#228480,
#228481,#228482,#228483,#228484,#228485,#228486,#228487,#228488,#228489,
#228490,#228491,#228492,#228493,#228494,#228495,#228496,#228497,#228498,
#228499,#228500,#228501,#228502,#228503,#228504,#228505,#228506,#228507,
#228508,#228509,#228510,#228511,#228512,#228513,#228514,#228515,#228516,
#228517,#228518,#228519,#228520,#228521,#228522,#228523,#228524,#228525,
#228526,#228527,#228528,#228529,#228530,#228531,#228532,#228533,#228534,
#228535,#228536,#228537,#228538,#228539,#228540,#228541,#228542,#228543,
#228544,#228545,#228546,#228547,#228548,#228549,#228550,#228551,#228552,
#228553,#228554,#228555,#228556,#228557,#228558,#228559,#228560,#228561,
#228562,#228563,#228564,#228565,#228566,#228567,#228568,#228569,#228570,
#228571,#228572,#228573,#228574,#228575,#228576,#228577,#228578,#228579,
#228580,#228581,#228582,#228583,#228584,#228585,#228586,#228587,#228588,
#228589,#228590,#228591,#228592,#228593,#228594,#228595,#228596,#228597,
#228598,#228599,#228600,#228601,#228602,#228603,#228604,#228605,#228606,
#228607,#228608,#228609,#228610,#228611,#228612,#228613,#228614,#228615,
#228616,#228617,#228618,#228619,#228620,#228621,#228622,#228623,#228624,
#228625,#228626,#228627,#228628,#228629,#228630,#228631,#228632,#228633,
#228634,#228635,#228636,#228637,#228638,#228639,#228640,#228641,#228642,
#228643,#228644,#228645,#228646,#228647,#228648,#228649,#228650,#228651,
#228652,#228653,#228654,#228655,#228656,#228657,#228658,#228659,#228660,
#228661,#228662,#228663,#228664,#228665,#228666,#228667,#228668,#228669,
#228670,#228671,#228672,#228673,#228674,#228675,#228676,#228677,#228678,
#228679,#228680,#228681,#228682,#228683,#228684,#228685,#228686,#228687,
#228688,#228689,#228690,#228691,#228692,#228693,#228694,#228695,#228696,
#228697,#228698,#228699,#228700,#228701,#228702,#228703,#228704,#228705,
#228706,#228707,#228708,#228709,#228710,#228711,#228712,#228713,#228714,
#228715,#228716,#228717,#228718,#228719,#228720,#228721,#228722,#228723,
#228724,#228725,#228726,#228727,#228728,#228729,#228730,#228731,#228732,
#228733,#228734,#228735,#228736,#228737,#228738,#228739,#228740,#228741,
#228742,#228743,#228744,#228745,#228746,#228747,#228748,#228749,#228750,
#228751,#228752,#228753,#228754,#228755,#228756,#228757,#228758,#228759,
#228760,#228761,#228762,#228763,#228764,#228765,#228766,#228767,#228768,
#228769,#228770,#228771,#228772,#228773,#228774,#228775,#228776,#228777,
#228778,#228779,#228780,#228781,#228782,#228783,#228784,#228785,#228786,
#228787,#228788,#228789,#228790,#228791,#228792,#228793,#228794,#228795,
#228796,#228797,#228798,#228799,#228800,#228801,#228802,#228803,#228804,
#228805,#228806,#228807,#228808,#228809,#228810,#228811,#228812,#228813,
#228814,#228815,#228816,#228817,#228818,#228819,#228820,#228821,#228822,
#228823,#228824,#228825,#228826,#228827,#228828,#228829,#228830,#228831,
#228832,#228833,#228834,#228835,#228836,#228837,#228838,#228839,#228840,
#228841,#228842,#228843,#228844,#228845,#228846,#228847,#228848,#228849,
#228850,#228851,#228852,#228853,#228854,#228855,#228856,#228857,#228858,
#228859,#228860,#228861,#228862,#228863,#228864,#228865,#228866,#228867,
#228868,#228869,#228870,#228871,#228872,#228873,#228874,#228875,#228876,
#228877,#228878,#228879,#228880,#228881,#228882,#228883,#228884,#228885,
#228886,#228887,#228888,#228889,#228890,#228891,#228892,#228893,#228894,
#228895,#228896,#228897,#228898,#228899,#228900,#228901,#228902,#228903,
#228904,#228905,#228906,#228907,#228908,#228909,#228910,#228911,#228912,
#228913,#228914,#228915,#228916,#228917,#228918,#228919,#228920,#228921,
#228922,#228923,#228924,#228925,#228926,#228927,#228928,#228929,#228930,
#228931,#228932,#228933,#228934,#228935,#228936,#228937,#228938,#228939,
#228940,#228941,#228942,#228943,#228944,#228945,#228946,#228947,#228948,
#228949,#228950,#228951,#228952,#228953,#228954,#228955,#228956,#228957,
#228958,#228959,#228960,#228961,#228962,#228963,#228964,#228965,#228966,
#228967,#228968,#228969,#228970,#228971,#228972,#228973,#228974,#228975,
#228976,#228977,#228978,#228979,#228980,#228981,#228982,#228983,#228984,
#228985,#228986,#228987,#228988,#228989,#228990,#228991,#228992,#228993,
#228994,#228995,#228996,#228997,#228998,#228999,#229000,#229001,#229002,
#229003,#229004,#229005,#229006,#229007,#229008,#229009,#229010,#229011,
#229012,#229013,#229014,#229015,#229016,#229017,#229018,#229019,#229020,
#229021,#229022,#229023,#229024,#229025,#229026,#229027,#229028,#229029,
#229030,#229031,#229032,#229033,#229034,#229035,#229036,#229037,#229038,
#229039,#229040,#229041,#229042,#229043,#229044,#229045,#229046,#229047,
#229048,#229049,#229050,#229051,#229052,#229053,#229054,#229055,#229056,
#229057,#229058,#229059,#229060,#229061,#229062,#229063,#229064,#229065,
#229066,#229067,#229068,#229069,#229070,#229071,#229072,#229073,#229074,
#229075,#229076,#229077,#229078,#229079,#229080,#229081,#229082,#229083,
#229084,#229085,#229086,#229087,#229088,#229089,#229090,#229091,#229092,
#229093,#229094,#229095,#229096,#229097,#229098,#229099,#229100,#229101,
#229102,#229103,#229104,#229105,#229106,#229107,#229108,#229109,#229110,
#229111,#229112,#229113,#229114,#229115,#229116,#229117,#229118,#229119,
#229120,#229121,#229122,#229123,#229124,#229125,#229126,#229127,#229128,
#229129,#229130,#229131,#229132,#229133,#229134,#229135,#229136,#229137,
#229138,#229139,#229140,#229141,#229142,#229143,#229144,#229145,#229146,
#229147,#229148,#229149,#229150,#229151,#229152,#229153,#229154,#229155,
#229156,#229157,#229158,#229159,#229160,#229161,#229162,#229163,#229164,
#229165,#229166,#229167,#229168,#229169,#229170,#229171,#229172,#229173,
#229174,#229175,#229176,#229177,#229178,#229179,#229180,#229181,#229182,
#229183,#229184,#229185,#229186,#229187,#229188,#229189,#229190,#229191,
#229192,#229193,#229194,#229195,#229196,#229197,#229198,#229199,#229200,
#229201,#229202,#229203,#229204,#229205,#229206,#229207,#229208,#229209,
#229210,#229211,#229212,#229213,#229214,#229215,#229216,#229217,#229218,
#229219,#229220,#229221,#229222,#229223,#229224,#229225,#229226,#229227,
#229228,#229229,#229230,#229231,#229232,#229233,#229234,#229235,#229236,
#229237,#229238,#229239,#229240,#229241,#229242,#229243,#229244,#229245,
#229246,#229247,#229248,#229249,#229250,#229251,#229252,#229253,#229254,
#229255,#229256,#229257,#229258,#229259,#229260,#229261,#229262,#229263,
#229264,#229265,#229266,#229267,#229268,#229269,#229270,#229271,#229272,
#229273,#229274,#229275,#229276,#229277,#229278,#229279,#229280,#229281,
#229282,#229283,#229284,#229285,#229286,#229287,#229288,#229289,#229290,
#229291,#229292,#229293,#229294,#229295,#229296,#229297,#229298,#229299,
#229300,#229301,#229302,#229303,#229304,#229305,#229306,#229307,#229308,
#229309,#229310,#229311,#229312,#229313,#229314,#229315,#229316,#229317,
#229318,#229319,#229320,#229321,#229322,#229323,#229324,#229325,#229326,
#229327,#229328,#229329,#229330,#229331,#229332,#229333,#229334,#229335,
#229336,#229337,#229338,#229339,#229340,#229341,#229342,#229343,#229344,
#229345,#229346,#229347,#229348,#229349,#229350,#229351,#229352,#229353,
#229354,#229355,#229356,#229357,#229358,#229359,#229360,#229361,#229362,
#229363,#229364,#229365,#229366,#229367,#229368,#229369,#229370,#229371,
#229372,#229373,#229374,#229375,#229376,#229377,#229378,#229379,#229380,
#229381,#229382,#229383,#229384,#229385,#229386,#229387,#229388,#229389,
#229390,#229391,#229392,#229393,#229394,#229395,#229396,#229397,#229398,
#229399,#229400,#229401,#229402,#229403,#229404,#229405,#229406,#229407,
#229408,#229409,#229410,#229411,#229412,#229413,#229414,#229415,#229416,
#229417,#229418,#229419,#229420,#229421,#229422,#229423,#229424,#229425,
#229426,#229427,#229428,#229429,#229430,#229431,#229432,#229433,#229434,
#229435,#229436,#229437,#229438,#229439,#229440,#229441,#229442,#229443,
#229444,#229445,#229446,#229447,#229448,#229449,#229450,#229451,#229452,
#229453,#229454,#229455,#229456,#229457,#229458,#229459,#229460,#229461,
#229462,#229463,#229464,#229465,#229466,#229467,#229468,#229469,#229470,
#229471,#229472,#229473,#229474,#229475,#229476,#229477,#229478,#229479,
#229480,#229481,#229482,#229483,#229484,#229485,#229486,#229487,#229488,
#229489,#229490,#229491,#229492,#229493,#229494,#229495,#229496,#229497,
#229498,#229499,#229500,#229501,#229502,#229503,#229504,#229505,#229506,
#229507,#229508,#229509,#229510,#229511,#229512,#229513,#229514,#229515,
#229516,#229517,#229518,#229519,#229520,#229521,#229522,#229523,#229524,
#229525,#229526,#229527,#229528,#229529,#229530,#229531,#229532,#229533,
#229534,#229535,#229536,#229537,#229538,#229539,#229540,#229541,#229542,
#229543,#229544,#229545,#229546,#229547,#229548,#229549,#229550,#229551,
#229552,#229553,#229554,#229555,#229556,#229557,#229558,#229559,#229560,
#229561,#229562,#229563,#229564,#229565,#229566,#229567,#229568,#229569,
#229570,#229571,#229572,#229573,#229574,#229575,#229576,#229577,#229578,
#229579,#229580,#229581,#229582,#229583,#229584,#229585,#229586,#229587,
#229588,#229589,#229590,#229591,#229592,#229593,#229594,#229595,#229596,
#229597,#229598,#229599,#229600,#229601,#229602,#229603,#229604,#229605,
#229606,#229607,#229608,#229609,#229610,#229611,#229612,#229613,#229614,
#229615,#229616,#229617,#229618,#229619,#229620,#229621,#229622,#229623,
#229624,#229625,#229626,#229627,#229628,#229629,#229630,#229631,#229632,
#229633,#229634,#229635,#229636,#229637,#229638,#229639,#229640,#229641,
#229642,#229643,#229644,#229645,#229646,#229647,#229648,#229649,#229650,
#229651,#229652,#229653,#229654,#229655,#229656,#229657,#229658,#229659,
#229660,#229661,#229662,#229663,#229664,#229665,#229666,#229667,#229668,
#229669,#229670,#229671,#229672,#229673,#229674,#229675,#229676,#229677,
#229678,#229679,#229680,#229681,#229682,#229683,#229684,#229685,#229686,
#229687,#229688,#229689,#229690,#229691,#229692,#229693,#229694,#229695,
#229696,#229697,#229698,#229699,#229700,#229701,#229702,#229703,#229704,
#229705,#229706),(#229707,#229708,#229709,#229710,#229711,#229712,#229713,
#229714,#229715,#229716,#229717,#229718,#229719,#229720,#229721,#229722,
#229723,#229724,#229725,#229726,#229727,#229728,#229729,#229730,#229731,
#229732,#229733,#229734,#229735,#229736,#229737,#229738,#229739,#229740,
#229741,#229742,#229743,#229744,#229745,#229746,#229747,#229748,#229749,
#229750,#229751,#229752,#229753,#229754,#229755,#229756,#229757,#229758,
#229759,#229760,#229761,#229762,#229763,#229764,#229765,#229766,#229767,
#229768,#229769,#229770,#229771,#229772,#229773,#229774,#229775,#229776,
#229777,#229778,#229779,#229780,#229781,#229782,#229783,#229784,#229785,
#229786,#229787,#229788,#229789,#229790,#229791,#229792,#229793,#229794,
#229795,#229796,#229797,#229798,#229799,#229800,#229801,#229802,#229803,
#229804,#229805,#229806,#229807,#229808,#229809,#229810,#229811,#229812,
#229813,#229814,#229815,#229816,#229817,#229818,#229819,#229820,#229821,
#229822,#229823,#229824,#229825,#229826,#229827,#229828,#229829,#229830,
#229831,#229832,#229833,#229834,#229835,#229836,#229837,#229838,#229839,
#229840,#229841,#229842,#229843,#229844,#229845,#229846,#229847,#229848,
#229849,#229850,#229851,#229852,#229853,#229854,#229855,#229856,#229857,
#229858,#229859,#229860,#229861,#229862,#229863,#229864,#229865,#229866,
#229867,#229868,#229869,#229870,#229871,#229872,#229873,#229874,#229875,
#229876,#229877,#229878,#229879,#229880,#229881,#229882,#229883,#229884,
#229885,#229886,#229887,#229888,#229889,#229890,#229891,#229892,#229893,
#229894,#229895,#229896,#229897,#229898,#229899,#229900,#229901,#229902,
#229903,#229904,#229905,#229906,#229907,#229908,#229909,#229910,#229911,
#229912,#229913,#229914,#229915,#229916,#229917,#229918,#229919,#229920,
#229921,#229922,#229923,#229924,#229925,#229926,#229927,#229928,#229929,
#229930,#229931,#229932,#229933,#229934,#229935,#229936,#229937,#229938,
#229939,#229940,#229941,#229942,#229943,#229944,#229945,#229946,#229947,
#229948,#229949,#229950,#229951,#229952,#229953,#229954,#229955,#229956,
#229957,#229958,#229959,#229960,#229961,#229962,#229963,#229964,#229965,
#229966,#229967,#229968,#229969,#229970,#229971,#229972,#229973,#229974,
#229975,#229976,#229977,#229978,#229979,#229980,#229981,#229982,#229983,
#229984,#229985,#229986,#229987,#229988,#229989,#229990,#229991,#229992,
#229993,#229994,#229995,#229996,#229997,#229998,#229999,#230000,#230001,
#230002,#230003,#230004,#230005,#230006,#230007,#230008,#230009,#230010,
#230011,#230012,#230013,#230014,#230015,#230016,#230017,#230018,#230019,
#230020,#230021,#230022,#230023,#230024,#230025,#230026,#230027,#230028,
#230029,#230030,#230031,#230032,#230033,#230034,#230035,#230036,#230037,
#230038,#230039,#230040,#230041,#230042,#230043,#230044,#230045,#230046,
#230047,#230048,#230049,#230050,#230051,#230052,#230053,#230054,#230055,
#230056,#230057,#230058,#230059,#230060,#230061,#230062,#230063,#230064,
#230065,#230066,#230067,#230068,#230069,#230070,#230071,#230072,#230073,
#230074,#230075,#230076,#230077,#230078,#230079,#230080,#230081,#230082,
#230083,#230084,#230085,#230086,#230087,#230088,#230089,#230090,#230091,
#230092,#230093,#230094,#230095,#230096,#230097,#230098,#230099,#230100,
#230101,#230102,#230103,#230104,#230105,#230106,#230107,#230108,#230109,
#230110,#230111,#230112,#230113,#230114,#230115,#230116,#230117,#230118,
#230119,#230120,#230121,#230122,#230123,#230124,#230125,#230126,#230127,
#230128,#230129,#230130,#230131,#230132,#230133,#230134,#230135,#230136,
#230137,#230138,#230139,#230140,#230141,#230142,#230143,#230144,#230145,
#230146,#230147,#230148,#230149,#230150,#230151,#230152,#230153,#230154,
#230155,#230156,#230157,#230158,#230159,#230160,#230161,#230162,#230163,
#230164,#230165,#230166,#230167,#230168,#230169,#230170,#230171,#230172,
#230173,#230174,#230175,#230176,#230177,#230178,#230179,#230180,#230181,
#230182,#230183,#230184,#230185,#230186,#230187,#230188,#230189,#230190,
#230191,#230192,#230193,#230194,#230195,#230196,#230197,#230198,#230199,
#230200,#230201,#230202,#230203,#230204,#230205,#230206,#230207,#230208,
#230209,#230210,#230211,#230212,#230213,#230214,#230215,#230216,#230217,
#230218,#230219,#230220,#230221,#230222,#230223,#230224,#230225,#230226,
#230227,#230228,#230229,#230230,#230231,#230232,#230233,#230234,#230235,
#230236,#230237,#230238,#230239,#230240,#230241,#230242,#230243,#230244,
#230245,#230246,#230247,#230248,#230249,#230250,#230251,#230252,#230253,
#230254,#230255,#230256,#230257,#230258,#230259,#230260,#230261,#230262,
#230263,#230264,#230265,#230266,#230267,#230268,#230269,#230270,#230271,
#230272,#230273,#230274,#230275,#230276,#230277,#230278,#230279,#230280,
#230281,#230282,#230283,#230284,#230285,#230286,#230287,#230288,#230289,
#230290,#230291,#230292,#230293,#230294,#230295,#230296,#230297,#230298,
#230299,#230300,#230301,#230302,#230303,#230304,#230305,#230306,#230307,
#230308,#230309,#230310,#230311,#230312,#230313,#230314,#230315,#230316,
#230317,#230318,#230319,#230320,#230321,#230322,#230323,#230324,#230325,
#230326,#230327,#230328,#230329,#230330,#230331,#230332,#230333,#230334,
#230335,#230336,#230337,#230338,#230339,#230340,#230341,#230342,#230343,
#230344,#230345,#230346,#230347,#230348,#230349,#230350,#230351,#230352,
#230353,#230354,#230355,#230356,#230357,#230358,#230359,#230360,#230361,
#230362,#230363,#230364,#230365,#230366,#230367,#230368,#230369,#230370,
#230371,#230372,#230373,#230374,#230375,#230376,#230377,#230378,#230379,
#230380,#230381,#230382,#230383,#230384,#230385,#230386,#230387,#230388,
#230389,#230390,#230391,#230392,#230393,#230394,#230395,#230396,#230397,
#230398,#230399,#230400,#230401,#230402,#230403,#230404,#230405,#230406,
#230407,#230408,#230409,#230410,#230411,#230412,#230413,#230414,#230415,
#230416,#230417,#230418,#230419,#230420,#230421,#230422,#230423,#230424,
#230425,#230426,#230427,#230428,#230429,#230430,#230431,#230432,#230433,
#230434,#230435,#230436,#230437,#230438,#230439,#230440,#230441,#230442,
#230443,#230444,#230445,#230446,#230447,#230448,#230449,#230450,#230451,
#230452,#230453,#230454,#230455,#230456,#230457,#230458,#230459,#230460,
#230461,#230462,#230463,#230464,#230465,#230466,#230467,#230468,#230469,
#230470,#230471,#230472,#230473,#230474,#230475,#230476,#230477,#230478,
#230479,#230480,#230481,#230482,#230483,#230484,#230485,#230486,#230487,
#230488,#230489,#230490,#230491,#230492,#230493,#230494,#230495,#230496,
#230497,#230498,#230499,#230500,#230501,#230502,#230503,#230504,#230505,
#230506,#230507,#230508,#230509,#230510,#230511,#230512,#230513,#230514,
#230515,#230516,#230517,#230518,#230519,#230520,#230521,#230522,#230523,
#230524,#230525,#230526,#230527,#230528,#230529,#230530,#230531,#230532,
#230533,#230534,#230535,#230536,#230537,#230538,#230539,#230540,#230541,
#230542,#230543,#230544,#230545,#230546,#230547,#230548,#230549,#230550,
#230551,#230552,#230553,#230554,#230555,#230556,#230557,#230558,#230559,
#230560,#230561,#230562,#230563,#230564,#230565,#230566,#230567,#230568,
#230569,#230570,#230571,#230572,#230573,#230574,#230575,#230576,#230577,
#230578,#230579,#230580,#230581,#230582,#230583,#230584,#230585,#230586,
#230587,#230588,#230589,#230590,#230591,#230592,#230593,#230594,#230595,
#230596,#230597,#230598,#230599,#230600,#230601,#230602,#230603,#230604,
#230605,#230606,#230607,#230608,#230609,#230610,#230611,#230612,#230613,
#230614,#230615,#230616,#230617,#230618,#230619,#230620,#230621,#230622,
#230623,#230624,#230625,#230626,#230627,#230628,#230629,#230630,#230631,
#230632,#230633,#230634,#230635,#230636,#230637,#230638,#230639,#230640,
#230641,#230642,#230643,#230644,#230645,#230646,#230647,#230648,#230649,
#230650,#230651,#230652,#230653,#230654,#230655,#230656,#230657,#230658,
#230659,#230660,#230661,#230662,#230663,#230664,#230665,#230666,#230667,
#230668,#230669,#230670,#230671,#230672,#230673,#230674,#230675,#230676,
#230677,#230678,#230679,#230680,#230681,#230682,#230683,#230684,#230685,
#230686,#230687,#230688,#230689,#230690,#230691,#230692,#230693,#230694,
#230695,#230696,#230697,#230698,#230699,#230700,#230701,#230702,#230703,
#230704,#230705,#230706,#230707,#230708,#230709,#230710,#230711,#230712,
#230713,#230714,#230715,#230716,#230717,#230718,#230719,#230720,#230721,
#230722,#230723,#230724,#230725,#230726,#230727,#230728,#230729,#230730,
#230731,#230732,#230733,#230734,#230735,#230736,#230737,#230738,#230739,
#230740,#230741,#230742,#230743,#230744,#230745,#230746,#230747,#230748,
#230749,#230750,#230751,#230752,#230753,#230754,#230755,#230756,#230757,
#230758,#230759,#230760,#230761,#230762,#230763,#230764,#230765,#230766,
#230767,#230768,#230769,#230770,#230771,#230772,#230773,#230774,#230775,
#230776,#230777,#230778,#230779,#230780,#230781,#230782,#230783,#230784,
#230785,#230786,#230787,#230788,#230789,#230790,#230791,#230792,#230793,
#230794,#230795,#230796,#230797,#230798,#230799,#230800,#230801,#230802,
#230803,#230804,#230805,#230806,#230807,#230808,#230809,#230810,#230811,
#230812,#230813,#230814,#230815,#230816,#230817,#230818,#230819,#230820,
#230821,#230822,#230823,#230824,#230825,#230826,#230827,#230828,#230829,
#230830,#230831,#230832,#230833,#230834,#230835,#230836,#230837,#230838,
#230839,#230840,#230841,#230842,#230843,#230844,#230845,#230846,#230847,
#230848,#230849,#230850,#230851,#230852,#230853,#230854,#230855,#230856,
#230857,#230858,#230859,#230860,#230861,#230862,#230863,#230864,#230865,
#230866,#230867,#230868,#230869,#230870,#230871,#230872,#230873,#230874,
#230875,#230876,#230877,#230878,#230879,#230880,#230881,#230882,#230883,
#230884,#230885,#230886,#230887,#230888,#230889,#230890,#230891,#230892,
#230893,#230894,#230895,#230896,#230897,#230898,#230899,#230900,#230901,
#230902,#230903,#230904,#230905,#230906,#230907,#230908,#230909,#230910,
#230911,#230912,#230913,#230914,#230915,#230916,#230917,#230918,#230919,
#230920,#230921,#230922,#230923,#230924,#230925,#230926,#230927,#230928,
#230929,#230930,#230931,#230932,#230933,#230934,#230935,#230936,#230937,
#230938,#230939,#230940,#230941,#230942,#230943,#230944,#230945,#230946,
#230947,#230948,#230949,#230950,#230951,#230952,#230953,#230954,#230955,
#230956,#230957,#230958,#230959,#230960,#230961,#230962,#230963,#230964,
#230965,#230966,#230967,#230968,#230969,#230970,#230971,#230972,#230973,
#230974,#230975,#230976,#230977,#230978,#230979,#230980,#230981,#230982,
#230983,#230984,#230985,#230986,#230987,#230988,#230989,#230990,#230991,
#230992,#230993,#230994,#230995,#230996,#230997,#230998,#230999,#231000,
#231001,#231002,#231003,#231004,#231005,#231006,#231007,#231008,#231009,
#231010,#231011,#231012,#231013,#231014,#231015,#231016,#231017,#231018,
#231019,#231020,#231021,#231022,#231023,#231024,#231025,#231026,#231027,
#231028,#231029,#231030,#231031,#231032,#231033,#231034,#231035,#231036,
#231037,#231038,#231039,#231040,#231041,#231042,#231043,#231044,#231045,
#231046,#231047,#231048,#231049,#231050,#231051,#231052,#231053,#231054,
#231055,#231056,#231057,#231058,#231059,#231060,#231061,#231062,#231063,
#231064,#231065,#231066,#231067,#231068,#231069,#231070,#231071,#231072,
#231073,#231074,#231075,#231076,#231077,#231078,#231079,#231080,#231081,
#231082,#231083,#231084,#231085,#231086,#231087,#231088,#231089,#231090,
#231091,#231092,#231093,#231094,#231095,#231096,#231097,#231098,#231099,
#231100,#231101,#231102,#231103,#231104,#231105,#231106,#231107,#231108,
#231109,#231110,#231111,#231112,#231113,#231114,#231115,#231116,#231117,
#231118,#231119,#231120,#231121,#231122,#231123,#231124,#231125,#231126,
#231127,#231128,#231129,#231130,#231131,#231132,#231133,#231134,#231135,
#231136,#231137,#231138,#231139,#231140,#231141,#231142,#231143,#231144,
#231145,#231146,#231147,#231148,#231149,#231150,#231151,#231152,#231153,
#231154,#231155,#231156,#231157,#231158,#231159,#231160,#231161,#231162,
#231163,#231164,#231165,#231166,#231167,#231168,#231169,#231170,#231171,
#231172,#231173,#231174,#231175,#231176,#231177,#231178,#231179,#231180,
#231181,#231182,#231183,#231184,#231185,#231186,#231187,#231188,#231189,
#231190,#231191,#231192,#231193,#231194,#231195,#231196,#231197,#231198,
#231199,#231200,#231201,#231202,#231203,#231204,#231205,#231206,#231207,
#231208,#231209,#231210,#231211,#231212,#231213,#231214,#231215,#231216,
#231217,#231218,#231219,#231220,#231221,#231222,#231223,#231224,#231225,
#231226,#231227,#231228,#231229,#231230,#231231,#231232,#231233,#231234,
#231235,#231236,#231237,#231238,#231239,#231240,#231241,#231242,#231243,
#231244,#231245,#231246,#231247,#231248,#231249,#231250,#231251,#231252,
#231253,#231254,#231255,#231256,#231257,#231258,#231259,#231260,#231261,
#231262,#231263,#231264,#231265,#231266,#231267,#231268,#231269,#231270,
#231271,#231272,#231273,#231274,#231275,#231276,#231277,#231278,#231279,
#231280,#231281,#231282,#231283,#231284,#231285,#231286,#231287,#231288,
#231289,#231290,#231291,#231292,#231293,#231294,#231295,#231296,#231297,
#231298,#231299,#231300,#231301,#231302,#231303,#231304,#231305,#231306,
#231307,#231308,#231309,#231310,#231311,#231312,#231313,#231314,#231315,
#231316,#231317,#231318,#231319,#231320,#231321,#231322,#231323,#231324,
#231325,#231326,#231327,#231328,#231329,#231330,#231331,#231332,#231333,
#231334,#231335,#231336,#231337,#231338,#231339,#231340,#231341,#231342,
#231343,#231344,#231345,#231346,#231347,#231348,#231349,#231350,#231351,
#231352,#231353,#231354,#231355,#231356,#231357,#231358,#231359,#231360,
#231361,#231362,#231363,#231364,#231365,#231366,#231367,#231368,#231369,
#231370,#231371,#231372,#231373,#231374,#231375,#231376,#231377,#231378,
#231379,#231380,#231381,#231382,#231383,#231384,#231385,#231386,#231387,
#231388,#231389,#231390,#231391,#231392,#231393,#231394,#231395,#231396,
#231397,#231398,#231399,#231400,#231401),(#231402,#231403,#231404,#231405,
#231406,#231407,#231408,#231409,#231410,#231411,#231412,#231413,#231414,
#231415,#231416,#231417,#231418,#231419,#231420,#231421,#231422,#231423,
#231424,#231425,#231426,#231427,#231428,#231429,#231430,#231431,#231432,
#231433,#231434,#231435,#231436,#231437,#231438,#231439,#231440,#231441,
#231442,#231443,#231444,#231445,#231446,#231447,#231448,#231449,#231450,
#231451,#231452,#231453,#231454,#231455,#231456,#231457,#231458,#231459,
#231460,#231461,#231462,#231463,#231464,#231465,#231466,#231467,#231468,
#231469,#231470,#231471,#231472,#231473,#231474,#231475,#231476,#231477,
#231478,#231479,#231480,#231481,#231482,#231483,#231484,#231485,#231486,
#231487,#231488,#231489,#231490,#231491,#231492,#231493,#231494,#231495,
#231496,#231497,#231498,#231499,#231500,#231501,#231502,#231503,#231504,
#231505,#231506,#231507,#231508,#231509,#231510,#231511,#231512,#231513,
#231514,#231515,#231516,#231517,#231518,#231519,#231520,#231521,#231522,
#231523,#231524,#231525,#231526,#231527,#231528,#231529,#231530,#231531,
#231532,#231533,#231534,#231535,#231536,#231537,#231538,#231539,#231540,
#231541,#231542,#231543,#231544,#231545,#231546,#231547,#231548,#231549,
#231550,#231551,#231552,#231553,#231554,#231555,#231556,#231557,#231558,
#231559,#231560,#231561,#231562,#231563,#231564,#231565,#231566,#231567,
#231568,#231569,#231570,#231571,#231572,#231573,#231574,#231575,#231576,
#231577,#231578,#231579,#231580,#231581,#231582,#231583,#231584,#231585,
#231586,#231587,#231588,#231589,#231590,#231591,#231592,#231593,#231594,
#231595,#231596,#231597,#231598,#231599,#231600,#231601,#231602,#231603,
#231604,#231605,#231606,#231607,#231608,#231609,#231610,#231611,#231612,
#231613,#231614,#231615,#231616,#231617,#231618,#231619,#231620,#231621,
#231622,#231623,#231624,#231625,#231626,#231627,#231628,#231629,#231630,
#231631,#231632,#231633,#231634,#231635,#231636,#231637,#231638,#231639,
#231640,#231641,#231642,#231643,#231644,#231645,#231646,#231647,#231648,
#231649,#231650,#231651,#231652,#231653,#231654,#231655,#231656,#231657,
#231658,#231659,#231660,#231661,#231662,#231663,#231664,#231665,#231666,
#231667,#231668,#231669,#231670,#231671,#231672,#231673,#231674,#231675,
#231676,#231677,#231678,#231679,#231680,#231681,#231682,#231683,#231684,
#231685,#231686,#231687,#231688,#231689,#231690,#231691,#231692,#231693,
#231694,#231695,#231696,#231697,#231698,#231699,#231700,#231701,#231702,
#231703,#231704,#231705,#231706,#231707,#231708,#231709,#231710,#231711,
#231712,#231713,#231714,#231715,#231716,#231717,#231718,#231719,#231720,
#231721,#231722,#231723,#231724,#231725,#231726,#231727,#231728,#231729,
#231730,#231731,#231732,#231733,#231734,#231735,#231736,#231737,#231738,
#231739,#231740,#231741,#231742,#231743,#231744,#231745,#231746,#231747,
#231748,#231749,#231750,#231751,#231752,#231753,#231754,#231755,#231756,
#231757,#231758,#231759,#231760,#231761,#231762,#231763,#231764,#231765,
#231766,#231767,#231768,#231769,#231770,#231771,#231772,#231773,#231774,
#231775,#231776,#231777,#231778,#231779,#231780,#231781,#231782,#231783,
#231784,#231785,#231786,#231787,#231788,#231789,#231790,#231791,#231792,
#231793,#231794,#231795,#231796,#231797,#231798,#231799,#231800,#231801,
#231802,#231803,#231804,#231805,#231806,#231807,#231808,#231809,#231810,
#231811,#231812,#231813,#231814,#231815,#231816,#231817,#231818,#231819,
#231820,#231821,#231822,#231823,#231824,#231825,#231826,#231827,#231828,
#231829,#231830,#231831,#231832,#231833,#231834,#231835,#231836,#231837,
#231838,#231839,#231840,#231841,#231842,#231843,#231844,#231845,#231846,
#231847,#231848,#231849,#231850,#231851,#231852,#231853,#231854,#231855,
#231856,#231857,#231858,#231859,#231860,#231861,#231862,#231863,#231864,
#231865,#231866,#231867,#231868,#231869,#231870,#231871,#231872,#231873,
#231874,#231875,#231876,#231877,#231878,#231879,#231880,#231881,#231882,
#231883,#231884,#231885,#231886,#231887,#231888,#231889,#231890,#231891,
#231892,#231893,#231894,#231895,#231896,#231897,#231898,#231899,#231900,
#231901,#231902,#231903,#231904,#231905,#231906,#231907,#231908,#231909,
#231910,#231911,#231912,#231913,#231914,#231915,#231916,#231917,#231918,
#231919,#231920,#231921,#231922,#231923,#231924,#231925,#231926,#231927,
#231928,#231929,#231930,#231931,#231932,#231933,#231934,#231935,#231936,
#231937,#231938,#231939,#231940,#231941,#231942,#231943,#231944,#231945,
#231946,#231947,#231948,#231949,#231950,#231951,#231952,#231953,#231954,
#231955,#231956,#231957,#231958,#231959,#231960,#231961,#231962,#231963,
#231964,#231965,#231966,#231967,#231968,#231969,#231970,#231971,#231972,
#231973,#231974,#231975,#231976,#231977,#231978,#231979,#231980,#231981,
#231982,#231983,#231984,#231985,#231986,#231987,#231988,#231989,#231990,
#231991,#231992,#231993,#231994,#231995,#231996,#231997,#231998,#231999,
#232000,#232001,#232002,#232003,#232004,#232005,#232006,#232007,#232008,
#232009,#232010,#232011,#232012,#232013,#232014,#232015,#232016,#232017,
#232018,#232019,#232020,#232021,#232022,#232023,#232024,#232025,#232026,
#232027,#232028,#232029,#232030,#232031,#232032,#232033,#232034,#232035,
#232036,#232037,#232038,#232039,#232040,#232041,#232042,#232043,#232044,
#232045,#232046,#232047,#232048,#232049,#232050,#232051,#232052,#232053,
#232054,#232055,#232056,#232057,#232058,#232059,#232060,#232061,#232062,
#232063,#232064,#232065,#232066,#232067,#232068,#232069,#232070,#232071,
#232072,#232073,#232074,#232075,#232076,#232077,#232078,#232079,#232080,
#232081,#232082,#232083,#232084,#232085,#232086,#232087,#232088,#232089,
#232090,#232091,#232092,#232093,#232094,#232095,#232096,#232097,#232098,
#232099,#232100,#232101,#232102,#232103,#232104,#232105,#232106,#232107,
#232108,#232109,#232110,#232111,#232112,#232113,#232114,#232115,#232116,
#232117,#232118,#232119,#232120,#232121,#232122,#232123,#232124,#232125,
#232126,#232127,#232128,#232129,#232130,#232131,#232132,#232133,#232134,
#232135,#232136,#232137,#232138,#232139,#232140,#232141,#232142,#232143,
#232144,#232145,#232146,#232147,#232148,#232149,#232150,#232151,#232152,
#232153,#232154,#232155,#232156,#232157,#232158,#232159,#232160,#232161,
#232162,#232163,#232164,#232165,#232166,#232167,#232168,#232169,#232170,
#232171,#232172,#232173,#232174,#232175,#232176,#232177,#232178,#232179,
#232180,#232181,#232182,#232183,#232184,#232185,#232186,#232187,#232188,
#232189,#232190,#232191,#232192,#232193,#232194,#232195,#232196,#232197,
#232198,#232199,#232200,#232201,#232202,#232203,#232204,#232205,#232206,
#232207,#232208,#232209,#232210,#232211,#232212,#232213,#232214,#232215,
#232216,#232217,#232218,#232219,#232220,#232221,#232222,#232223,#232224,
#232225,#232226,#232227,#232228,#232229,#232230,#232231,#232232,#232233,
#232234,#232235,#232236,#232237,#232238,#232239,#232240,#232241,#232242,
#232243,#232244,#232245,#232246,#232247,#232248,#232249,#232250,#232251,
#232252,#232253,#232254,#232255,#232256,#232257,#232258,#232259,#232260,
#232261,#232262,#232263,#232264,#232265,#232266,#232267,#232268,#232269,
#232270,#232271,#232272,#232273,#232274,#232275,#232276,#232277,#232278,
#232279,#232280,#232281,#232282,#232283,#232284,#232285,#232286,#232287,
#232288,#232289,#232290,#232291,#232292,#232293,#232294,#232295,#232296,
#232297,#232298,#232299,#232300,#232301,#232302,#232303,#232304,#232305,
#232306,#232307,#232308,#232309,#232310,#232311,#232312,#232313,#232314,
#232315,#232316,#232317,#232318,#232319,#232320,#232321,#232322,#232323,
#232324,#232325,#232326,#232327,#232328,#232329,#232330,#232331,#232332,
#232333,#232334,#232335,#232336,#232337,#232338,#232339,#232340,#232341,
#232342,#232343,#232344,#232345,#232346,#232347,#232348,#232349,#232350,
#232351,#232352,#232353,#232354,#232355,#232356,#232357,#232358,#232359,
#232360,#232361,#232362,#232363,#232364,#232365,#232366,#232367,#232368,
#232369,#232370,#232371,#232372,#232373,#232374,#232375,#232376,#232377,
#232378,#232379,#232380,#232381,#232382,#232383,#232384,#232385,#232386,
#232387,#232388,#232389,#232390,#232391,#232392,#232393,#232394,#232395,
#232396,#232397,#232398,#232399,#232400,#232401,#232402,#232403,#232404,
#232405,#232406,#232407,#232408,#232409,#232410,#232411,#232412,#232413,
#232414,#232415,#232416,#232417,#232418,#232419,#232420,#232421,#232422,
#232423,#232424,#232425,#232426,#232427,#232428,#232429,#232430,#232431,
#232432,#232433,#232434,#232435,#232436,#232437,#232438,#232439,#232440,
#232441,#232442,#232443,#232444,#232445,#232446,#232447,#232448,#232449,
#232450,#232451,#232452,#232453,#232454,#232455,#232456,#232457,#232458,
#232459,#232460,#232461,#232462,#232463,#232464,#232465,#232466,#232467,
#232468,#232469,#232470,#232471,#232472,#232473,#232474,#232475,#232476,
#232477,#232478,#232479,#232480,#232481,#232482,#232483,#232484,#232485,
#232486,#232487,#232488,#232489,#232490,#232491,#232492,#232493,#232494,
#232495,#232496,#232497,#232498,#232499,#232500,#232501,#232502,#232503,
#232504,#232505,#232506,#232507,#232508,#232509,#232510,#232511,#232512,
#232513,#232514,#232515,#232516,#232517,#232518,#232519,#232520,#232521,
#232522,#232523,#232524,#232525,#232526,#232527,#232528,#232529,#232530,
#232531,#232532,#232533,#232534,#232535,#232536,#232537,#232538,#232539,
#232540,#232541,#232542,#232543,#232544,#232545,#232546,#232547,#232548,
#232549,#232550,#232551,#232552,#232553,#232554,#232555,#232556,#232557,
#232558,#232559,#232560,#232561,#232562,#232563,#232564,#232565,#232566,
#232567,#232568,#232569,#232570,#232571,#232572,#232573,#232574,#232575,
#232576,#232577,#232578,#232579,#232580,#232581,#232582,#232583,#232584,
#232585,#232586,#232587,#232588,#232589,#232590,#232591,#232592,#232593,
#232594,#232595,#232596,#232597,#232598,#232599,#232600,#232601,#232602,
#232603,#232604,#232605,#232606,#232607,#232608,#232609,#232610,#232611,
#232612,#232613,#232614,#232615,#232616,#232617,#232618,#232619,#232620,
#232621,#232622,#232623,#232624,#232625,#232626,#232627,#232628,#232629,
#232630,#232631,#232632,#232633,#232634,#232635,#232636,#232637,#232638,
#232639,#232640,#232641,#232642,#232643,#232644,#232645,#232646,#232647,
#232648,#232649,#232650,#232651,#232652,#232653,#232654,#232655,#232656,
#232657,#232658,#232659,#232660,#232661,#232662,#232663,#232664,#232665,
#232666,#232667,#232668,#232669,#232670,#232671,#232672,#232673,#232674,
#232675,#232676,#232677,#232678,#232679,#232680,#232681,#232682,#232683,
#232684,#232685,#232686,#232687,#232688,#232689,#232690,#232691,#232692,
#232693,#232694,#232695,#232696,#232697,#232698,#232699,#232700,#232701,
#232702,#232703,#232704,#232705,#232706,#232707,#232708,#232709,#232710,
#232711,#232712,#232713,#232714,#232715,#232716,#232717,#232718,#232719,
#232720,#232721,#232722,#232723,#232724,#232725,#232726,#232727,#232728,
#232729,#232730,#232731,#232732,#232733,#232734,#232735,#232736,#232737,
#232738,#232739,#232740,#232741,#232742,#232743,#232744,#232745,#232746,
#232747,#232748,#232749,#232750,#232751,#232752,#232753,#232754,#232755,
#232756,#232757,#232758,#232759,#232760,#232761,#232762,#232763,#232764,
#232765,#232766,#232767,#232768,#232769,#232770,#232771,#232772,#232773,
#232774,#232775,#232776,#232777,#232778,#232779,#232780,#232781,#232782,
#232783,#232784,#232785,#232786,#232787,#232788,#232789,#232790,#232791,
#232792,#232793,#232794,#232795,#232796,#232797,#232798,#232799,#232800,
#232801,#232802,#232803,#232804,#232805,#232806,#232807,#232808,#232809,
#232810,#232811,#232812,#232813,#232814,#232815,#232816,#232817,#232818,
#232819,#232820,#232821,#232822,#232823,#232824,#232825,#232826,#232827,
#232828,#232829,#232830,#232831,#232832,#232833,#232834,#232835,#232836,
#232837,#232838,#232839,#232840,#232841,#232842,#232843,#232844,#232845,
#232846,#232847,#232848,#232849,#232850,#232851,#232852,#232853,#232854,
#232855,#232856,#232857,#232858,#232859,#232860,#232861,#232862,#232863,
#232864,#232865,#232866,#232867,#232868,#232869,#232870,#232871,#232872,
#232873,#232874,#232875,#232876,#232877,#232878,#232879,#232880,#232881,
#232882,#232883,#232884,#232885,#232886,#232887,#232888,#232889,#232890,
#232891,#232892,#232893,#232894,#232895,#232896,#232897,#232898,#232899,
#232900,#232901,#232902,#232903,#232904,#232905,#232906,#232907,#232908,
#232909,#232910,#232911,#232912,#232913,#232914,#232915,#232916,#232917,
#232918,#232919,#232920,#232921,#232922,#232923,#232924,#232925,#232926,
#232927,#232928,#232929,#232930,#232931,#232932,#232933,#232934,#232935,
#232936,#232937,#232938,#232939,#232940,#232941,#232942,#232943,#232944,
#232945,#232946,#232947,#232948,#232949,#232950,#232951,#232952,#232953,
#232954,#232955,#232956,#232957,#232958,#232959,#232960,#232961,#232962,
#232963,#232964,#232965,#232966,#232967,#232968,#232969,#232970,#232971,
#232972,#232973,#232974,#232975,#232976,#232977,#232978,#232979,#232980,
#232981,#232982,#232983,#232984,#232985,#232986,#232987,#232988,#232989,
#232990,#232991,#232992,#232993,#232994,#232995,#232996,#232997,#232998,
#232999,#233000,#233001,#233002,#233003,#233004,#233005,#233006,#233007,
#233008,#233009,#233010,#233011,#233012,#233013,#233014,#233015,#233016,
#233017,#233018,#233019,#233020,#233021,#233022,#233023,#233024,#233025,
#233026,#233027,#233028,#233029,#233030,#233031,#233032,#233033,#233034,
#233035,#233036,#233037,#233038,#233039,#233040,#233041,#233042,#233043,
#233044,#233045,#233046,#233047,#233048,#233049,#233050,#233051,#233052,
#233053,#233054,#233055,#233056,#233057,#233058,#233059,#233060,#233061,
#233062,#233063,#233064,#233065,#233066,#233067,#233068,#233069,#233070,
#233071,#233072,#233073,#233074,#233075,#233076,#233077,#233078,#233079,
#233080,#233081,#233082,#233083,#233084,#233085,#233086,#233087,#233088,
#233089,#233090,#233091,#233092,#233093,#233094,#233095,#233096)),
 .UNSPECIFIED.,.F.,.F.,.F.,(4,4),(4,1,1,1,1,1,1,1,1,1,1,1,1,1,1,1,1,1,1,
1,1,1,1,1,1,1,1,1,1,1,1,1,1,1,1,1,1,1,1,1,1,1,1,1,1,1,1,1,1,1,1,1,1,1,1,
1,1,1,1,1,1,1,1,1,1,1,1,1,1,1,1,1,1,1,1,1,1,1,1,1,1,1,1,1,1,1,1,1,1,1,1,
1,1,1,1,1,1,1,1,1,1,1,1,1,1,1,1,1,1,1,1,1,1,1,1,1,1,1,1,1,1,1,1,1,1,1,1,
1,1,1,1,1,1,1,1,1,1,1,1,1,1,1,1,1,1,1,1,1,1,1,1,1,1,1,1,1,1,1,1,1,1,1,1,
1,1,1,1,1,1,1,1,1,1,1,1,1,1,1,1,1,1,1,1,1,1,1,1,1,1,1,1,1,1,1,1,1,1,1,1,
1,1,1,1,1,1,1,1,1,1,1,1,1,1,1,1,1,1,1,1,1,1,1,1,1,1,1,1,1,1,1,1,1,1,1,1,
1,1,1,1,1,1,1,1,1,1,1,1,1,1,1,1,1,1,1,1,1,1,1,1,1,1,1,1,1,1,1,1,1,1,1,1,
1,1,1,1,1,1,1,1,1,1,1,1,1,1,1,1,1,1,1,1,1,1,1,1,1,1,1,1,1,1,1,1,1,1,1,1,
1,1,1,1,1,1,1,1,1,1,1,1,1,1,1,1,1,1,1,1,1,1,1,1,1,1,1,1,1,1,1,1,1,1,1,1,
1,1,1,1,1,1,1,1,1,1,1,1,1,1,1,1,1,1,1,1,1,1,1,1,1,1,1,1,1,1,1,1,1,1,1,1,
1,1,1,1,1,1,1,1,1,1,1,1,1,1,1,1,1,1,1,1,1,1,1,1,1,1,1,1,1,1,1,1,1,1,1,1,
1,1,1,1,1,1,1,1,1,1,1,1,1,1,1,1,1,1,1,1,1,1,1,1,1,1,1,1,1,1,1,1,1,1,1,1,
1,1,1,1,1,1,1,1,1,1,1,1,1,1,1,1,1,1,1,1,1,1,1,1,1,1,1,1,1,1,1,1,1,1,1,1,
1,1,1,1,1,1,1,1,1,1,1,1,1,1,1,1,1,1,1,1,1,1,1,1,1,1,1,1,1,1,1,1,1,1,1,1,
1,1,1,1,1,1,1,1,1,1,1,1,1,1,1,1,1,1,1,1,1,1,1,1,1,1,1,1,1,1,1,1,1,1,1,1,
1,1,1,1,1,1,1,1,1,1,1,1,1,1,1,1,1,1,1,1,1,1,1,1,1,1,1,1,1,1,1,1,1,1,1,1,
1,1,1,1,1,1,1,1,1,1,1,1,1,1,1,1,1,1,1,1,1,1,1,1,1,1,1,1,1,1,1,1,1,1,1,1,
1,1,1,1,1,1,1,1,1,1,1,1,1,1,1,1,1,1,1,1,1,1,1,1,1,1,1,1,1,1,1,1,1,1,1,1,
1,1,1,1,1,1,1,1,1,1,1,1,1,1,1,1,1,1,1,1,1,1,1,1,1,1,1,1,1,1,1,1,1,1,1,1,
1,1,1,1,1,1,1,1,1,1,1,1,1,1,1,1,1,1,1,1,1,1,1,1,1,1,1,1,1,1,1,1,1,1,1,1,
1,1,1,1,1,1,1,1,1,1,1,1,1,1,1,1,1,1,1,1,1,1,1,1,1,1,1,1,1,1,1,1,1,1,1,1,
1,1,1,1,1,1,1,1,1,1,1,1,1,1,1,1,1,1,1,1,1,1,1,1,1,1,1,1,1,1,1,1,1,1,1,1,
1,1,1,1,1,1,1,1,1,1,1,1,1,1,1,1,1,1,1,1,1,1,1,1,1,1,1,1,1,1,1,1,1,1,1,1,
1,1,1,1,1,1,1,1,1,1,1,1,1,1,1,1,1,1,1,1,1,1,1,1,1,1,1,1,1,1,1,1,1,1,1,1,
1,1,1,1,1,1,1,1,1,1,1,1,1,1,1,1,1,1,1,1,1,1,1,1,1,1,1,1,1,1,1,1,1,1,1,1,
1,1,1,1,1,1,1,1,1,1,1,1,1,1,1,1,1,1,1,1,1,1,1,1,1,1,1,1,1,1,1,1,1,1,1,1,
1,1,1,1,1,1,1,1,1,1,1,1,1,1,1,1,1,1,1,1,1,1,1,1,1,1,1,1,1,1,1,1,1,1,1,1,
1,1,1,1,1,1,1,1,1,1,1,1,1,1,1,1,1,1,1,1,1,1,1,1,1,1,1,1,1,1,1,1,1,1,1,1,
1,1,1,1,1,1,1,1,1,1,1,1,1,1,1,1,1,1,1,1,1,1,1,1,1,1,1,1,1,1,1,1,1,1,1,1,
1,1,1,1,1,1,1,1,1,1,1,1,1,1,1,1,1,1,1,1,1,1,1,1,1,1,1,1,1,1,1,1,1,1,1,1,
1,1,1,1,1,1,1,1,1,1,1,1,1,1,1,1,1,1,1,1,1,1,1,1,1,1,1,1,1,1,1,1,1,1,1,1,
1,1,1,1,1,1,1,1,1,1,1,1,1,1,1,1,1,1,1,1,1,1,1,1,1,1,1,1,1,1,1,1,1,1,1,1,
1,1,1,1,1,1,1,1,1,1,1,1,1,1,1,1,1,1,1,1,1,1,1,1,1,1,1,1,1,1,1,1,1,1,1,1,
1,1,1,1,1,1,1,1,1,1,1,1,1,1,1,1,1,1,1,1,1,1,1,1,1,1,1,1,1,1,1,1,1,1,1,1,
1,1,1,1,1,1,1,1,1,1,1,1,1,1,1,1,1,1,1,1,1,1,1,1,1,1,1,1,1,1,1,1,1,1,1,1,
1,1,1,1,1,1,1,1,1,1,1,1,1,1,1,1,1,1,1,1,1,1,1,1,1,1,1,1,1,1,1,1,1,1,1,1,
1,1,1,1,1,1,1,1,1,1,1,1,1,1,1,1,1,1,1,1,1,1,1,1,1,1,1,1,1,1,1,1,1,1,1,1,
1,1,1,1,1,1,1,1,1,1,1,1,1,1,1,1,1,1,1,1,1,1,1,1,1,1,1,1,1,1,1,1,1,1,1,1,
1,1,1,1,1,1,1,1,1,1,1,1,1,1,1,1,1,1,1,1,1,1,1,1,1,1,1,1,1,1,1,1,1,1,1,1,
1,1,1,1,1,1,1,1,1,1,1,1,1,1,1,1,1,1,1,1,1,1,1,1,1,1,1,1,1,1,1,1,1,1,1,1,
1,1,1,1,1,1,1,1,1,1,1,1,1,1,1,1,1,1,1,1,1,1,1,1,1,1,1,1,1,1,1,1,1,1,1,1,
1,1,1,1,1,1,1,1,1,1,1,1,1,1,1,1,1,1,1,1,1,1,1,1,1,1,1,1,1,1,1,1,1,1,1,1,
1,1,1,1,1,1,1,1,1,1,1,1,1,1,1,1,1,1,1,1,1,1,1,1,1,1,1,1,1,1,1,1,1,1,1,1,
1,1,1,1,1,1,1,1,1,1,1,1,1,1,1,1,1,1,1,1,1,1,1,1,1,1,1,1,1,1,1,1,1,1,1,1,
1,1,1,1,1,1,1,1,1,1,1,1,1,1,1,1,1,1,1,1,1,1,1,1,1,1,1,1,1,1,1,1,1,1,1,1,
1,1,1,1,1,1,1,1,1,1,1,1,1,1,1,1,1,1,1,1,1,1,1,1,1,1,1,1,1,1,1,1,1,1,1,1,
1,1,1,1,1,1,1,1,1,1,1,1,1,1,1,1,1,4),(-0.000587328099657093,0.1157205948422),
(8.30590413559005,8.80579087257276,9.30565887793282,10.305394888653,11.3051308993731,
12.3048669100932,13.3046029208133,14.3043389315335,15.3040749422536,16.3038109529737,
17.3035469636939,18.303282974414,19.3030189851341,20.3027549958542,21.3024910065744,
22.3022270172945,23.3019630280146,24.3016990387348,25.3014350494549,26.301171060175,
27.3009070708951,28.3006430816153,29.3003790923354,30.3001151030555,31.2998511137757,
32.2995871244958,33.2993231352159,34.299059145936,35.2987951566562,36.2985311673763,
37.2982671780964,38.2980031888166,39.2977391995367,40.2974752102568,41.2972112209769,
42.2969472316971,43.2966832424172,44.2964192531373,45.2961552638575,46.2958912745776,
47.2956272852977,48.2953632960178,49.295099306738,50.2948353174581,51.2945713281782,
52.2943073388984,53.2940433496185,54.2937793603386,55.2935153710587,56.2932513817789,
57.292987392499,58.2927234032191,59.2924594139393,60.2921954246594,61.2919314353795,
62.2916674460996,63.2914034568198,64.2911394675399,65.29087547826,66.2906114889802,
67.2903474997003,68.2900835104204,69.2898195211405,70.2895555318607,71.2892915425808,
72.2890275533009,73.2887635640211,74.2884995747412,75.2882355854613,76.2879715961814,
77.2877076069016,78.2874436176217,79.2871796283418,80.286915639062,81.2866516497821,
82.2863876605022,83.2861236712224,84.2858596819425,85.2855956926626,86.2853317033827,
87.2850677141029,88.284803724823,89.2845397355431,90.2842757462633,91.2840117569834,
92.2837477677035,93.2834837784236,94.2832197891438,95.2829557998639,96.282691810584,
97.2824278213041,98.2821638320243,99.2818998427444,100.281635853465,101.281371864185,
102.281107874905,103.280843885625,104.280579896345,105.280315907065,106.280051917785,
107.279787928505,108.279523939226,109.279259949946,110.278995960666,111.278731971386,
112.278467982106,113.278203992826,114.277940003546,115.277676014266,116.277412024987,
117.277148035707,118.276884046427,119.276620057147,120.276356067867,121.276092078587,
122.275828089307,123.275564100028,124.275300110748,125.275036121468,126.274772132188,
127.274508142908,128.274244153628,129.273980164348,130.273716175068,131.273452185789,
132.273188196509,133.272924207229,134.272660217949,135.272396228669,136.272132239389,
137.271868250109,138.271604260829,139.27134027155,140.27107628227,141.27081229299,
142.27054830371,143.27028431443,144.27002032515,145.26975633587,146.26949234659,
147.269228357311,148.268964368031,149.268700378751,150.268436389471,151.268172400191,
152.267908410911,153.267644421631,154.267380432352,155.267116443072,156.266852453792,
157.266588464512,158.266324475232,159.266060485952,160.265796496672,161.265532507392,
162.265268518113,163.265004528833,164.264740539553,165.264476550273,166.264212560993,
167.263948571713,168.263684582433,169.263420593153,170.263156603874,171.262892614594,
172.262628625314,173.262364636034,174.262100646754,175.261836657474,176.261572668194,
177.261308678914,178.261044689635,179.260780700355,180.260516711075,181.260252721795,
182.259988732515,183.259724743235,184.259460753955,185.259196764675,186.258932775396,
187.258668786116,188.258404796836,189.258140807556,190.257876818276,191.257612828996,
192.257348839716,193.257084850437,194.256820861157,195.256556871877,196.256292882597,
197.256028893317,198.255764904037,199.255500914757,200.255236925477,201.254972936198,
202.254708946918,203.254444957638,204.254180968358,205.253916979078,206.253652989798,
207.253389000518,208.253125011238,209.252861021959,210.252597032679,211.252333043399,
212.252069054119,213.251805064839,214.251541075559,215.251277086279,216.251013096999,
217.25074910772,218.25048511844,219.25022112916,220.24995713988,221.2496931506,
222.24942916132,223.24916517204,224.248901182761,225.248637193481,226.248373204201,
227.248109214921,228.247845225641,229.247581236361,230.247317247081,231.247053257801,
232.246789268522,233.246525279242,234.246261289962,235.245997300682,236.245733311402,
237.245469322122,238.245205332842,239.244941343562,240.244677354283,241.244413365003,
242.244149375723,243.243885386443,244.243621397163,245.243357407883,246.243093418603,
247.242829429323,248.242565440044,249.242301450764,250.242037461484,251.241773472204,
252.241509482924,253.241245493644,254.240981504364,255.240717515084,256.240453525805,
257.240189536525,258.239925547245,259.239661557965,260.239397568685,261.239133579405,
262.238869590125,263.238605600846,264.238341611566,265.238077622286,266.237813633006,
267.237549643726,268.237285654446,269.237021665166,270.236757675886,271.236493686607,
272.236229697327,273.235965708047,274.235701718767,275.235437729487,276.235173740207,
277.234909750927,278.234645761647,279.234381772368,280.234117783088,281.233853793808,
282.233589804528,283.233325815248,284.233061825968,285.232797836688,286.232533847408,
287.232269858129,288.232005868849,289.231741879569,290.231477890289,291.231213901009,
292.230949911729,293.230685922449,294.23042193317,295.23015794389,296.22989395461,
297.22962996533,298.22936597605,299.22910198677,300.22883799749,301.22857400821,
302.228310018931,303.228046029651,304.227782040371,305.227518051091,306.227254061811,
307.226990072531,308.226726083251,309.226462093971,310.226198104692,311.225934115412,
312.225670126132,313.225406136852,314.225142147572,315.224878158292,316.224614169012,
317.224350179732,318.224086190453,319.223822201173,320.223558211893,321.223294222613,
322.223030233333,323.222766244053,324.222502254773,325.222238265494,326.221974276214,
327.221710286934,328.221446297654,329.221182308374,330.220918319094,331.220654329814,
332.220390340534,333.220126351255,334.219862361975,335.219598372695,336.219334383415,
337.219070394135,338.218806404855,339.218542415575,340.218278426295,341.218014437016,
342.217750447736,343.217486458456,344.217222469176,345.216958479896,346.216694490616,
347.216430501336,348.216166512056,349.215902522777,350.215638533497,351.215374544217,
352.215110554937,353.214846565657,354.214582576377,355.214318587097,356.214054597817,
357.213790608538,358.213526619258,359.213262629978,360.212998640698,361.212734651418,
362.212470662138,363.212206672858,364.211942683579,365.211678694299,366.211414705019,
367.211150715739,368.210886726459,369.210622737179,370.210358747899,371.210094758619,
372.20983076934,373.20956678006,374.20930279078,375.2090388015,376.20877481222,
377.20851082294,378.20824683366,379.20798284438,380.207718855101,381.207454865821,
382.207190876541,383.206926887261,384.206662897981,385.206398908701,386.206134919421,
387.205870930141,388.205606940862,389.205342951582,390.205078962302,391.204814973022,
392.204550983742,393.204286994462,394.204023005182,395.203759015903,396.203495026623,
397.203231037343,398.202967048063,399.202703058783,400.202439069503,401.202175080223,
402.201911090943,403.201647101664,404.201383112384,405.201119123104,406.200855133824,
407.200591144544,408.200327155264,409.200063165984,410.199799176704,411.199535187425,
412.199271198145,413.199007208865,414.198743219585,415.198479230305,416.198215241025,
417.197951251745,418.197687262465,419.197423273186,420.197159283906,421.196895294626,
422.196631305346,423.196367316066,424.196103326786,425.195839337506,426.195575348226,
427.195311358947,428.195047369667,429.194783380387,430.194519391107,431.194255401827,
432.193991412547,433.193727423267,434.193463433988,435.193199444708,436.192935455428,
437.192671466148,438.192407476868,439.192143487588,440.191879498308,441.191615509028,
442.191351519749,443.191087530469,444.190823541189,445.190559551909,446.190295562629,
447.190031573349,448.189767584069,449.189503594789,450.18923960551,451.18897561623,
452.18871162695,453.18844763767,454.18818364839,455.18791965911,456.18765566983,
457.18739168055,458.187127691271,459.186863701991,460.186599712711,461.186335723431,
462.186071734151,463.185807744871,464.185543755591,465.185279766312,466.185015777032,
467.184751787752,468.184487798472,469.184223809192,470.183959819912,471.183695830632,
472.183431841352,473.183167852073,474.182903862793,475.182639873513,476.182375884233,
477.182111894953,478.181847905673,479.181583916393,480.181319927113,481.181055937834,
482.180791948554,483.180527959274,484.180263969994,485.179999980714,486.179735991434,
487.179472002154,488.179208012874,489.178944023595,490.178680034315,491.178416045035,
492.178152055755,493.177888066475,494.177624077195,495.177360087915,496.177096098636,
497.176832109356,498.176568120076,499.176304130796,500.176040141516,501.175776152236,
502.175512162956,503.175248173676,504.174984184397,505.174720195117,506.174456205837,
507.174192216557,508.173928227277,509.173664237997,510.173400248717,511.173136259437,
512.172872270158,513.172608280878,514.172344291598,515.172080302318,516.171816313038,
517.171552323758,518.171288334478,519.171024345198,520.170760355919,521.170496366639,
522.170232377359,523.169968388079,524.169704398799,525.169440409519,526.169176420239,
527.168912430959,528.16864844168,529.1683844524,530.16812046312,531.16785647384,
532.16759248456,533.16732849528,534.167064506,535.166800516721,536.166536527441,
537.166272538161,538.166008548881,539.165744559601,540.165480570321,541.165216581041,
542.164952591761,543.164688602482,544.164424613202,545.164160623922,546.163896634642,
547.163632645362,548.163368656082,549.163104666802,550.162840677522,551.162576688243,
552.162312698963,553.162048709683,554.161784720403,555.161520731123,556.161256741843,
557.160992752563,558.160728763283,559.160464774004,560.160200784724,561.159936795444,
562.159672806164,563.159408816884,564.159144827604,565.158880838324,566.158616849045,
567.158352859765,568.158088870485,569.157824881205,570.157560891925,571.157296902645,
572.157032913365,573.156768924085,574.156504934806,575.156240945526,576.155976956246,
577.155712966966,578.155448977686,579.155184988406,580.154920999126,581.154657009846,
582.154393020567,583.154129031287,584.153865042007,585.153601052727,586.153337063447,
587.153073074167,588.152809084887,589.152545095607,590.152281106328,591.152017117048,
592.151753127768,593.151489138488,594.151225149208,595.150961159928,596.150697170648,
597.150433181368,598.150169192089,599.149905202809,600.149641213529,601.149377224249,
602.149113234969,603.148849245689,604.148585256409,605.14832126713,606.14805727785,
607.14779328857,608.14752929929,609.14726531001,610.14700132073,611.14673733145,
612.14647334217,613.146209352891,614.145945363611,615.145681374331,616.145417385051,
617.145153395771,618.144889406491,619.144625417211,620.144361427931,621.144097438652,
622.143833449372,623.143569460092,624.143305470812,625.143041481532,626.142777492252,
627.142513502972,628.142249513692,629.141985524413,630.141721535133,631.141457545853,
632.141193556573,633.140929567293,634.140665578013,635.140401588733,636.140137599454,
637.139873610174,638.139609620894,639.139345631614,640.139081642334,641.138817653054,
642.138553663774,643.138289674494,644.138025685215,645.137761695935,646.137497706655,
647.137233717375,648.136969728095,649.136705738815,650.136441749535,651.136177760255,
652.135913770976,653.135649781696,654.135385792416,655.135121803136,656.134857813856,
657.134593824576,658.134329835296,659.134065846016,660.133801856737,661.133537867457,
662.133273878177,663.133009888897,664.132745899617,665.132481910337,666.132217921057,
667.131953931778,668.131689942498,669.131425953218,670.131161963938,671.130897974658,
672.130633985378,673.130369996098,674.130106006818,675.129842017539,676.129578028259,
677.129314038979,678.129050049699,679.128786060419,680.128522071139,681.128258081859,
682.127994092579,683.1277301033,684.12746611402,685.12720212474,686.12693813546,
687.12667414618,688.1264101569,689.12614616762,690.12588217834,691.125618189061,
692.125354199781,693.125090210501,694.124826221221,695.124562231941,696.124298242661,
697.124034253381,698.123770264101,699.123506274822,700.123242285542,701.122978296262,
702.122714306982,703.122450317702,704.122186328422,705.121922339142,706.121658349863,
707.121394360583,708.121130371303,709.120866382023,710.120602392743,711.120338403463,
712.120074414183,713.119810424903,714.119546435624,715.119282446344,716.119018457064,
717.118754467784,718.118490478504,719.118226489224,720.117962499944,721.117698510664,
722.117434521385,723.117170532105,724.116906542825,725.116642553545,726.116378564265,
727.116114574985,728.115850585705,729.115586596425,730.115322607146,731.115058617866,
732.114794628586,733.114530639306,734.114266650026,735.114002660746,736.113738671466,
737.113474682187,738.113210692907,739.112946703627,740.112682714347,741.112418725067,
742.112154735787,743.111890746507,744.111626757227,745.111362767948,746.111098778668,
747.110834789388,748.110570800108,749.110306810828,750.110042821548,751.109778832268,
752.109514842988,753.109250853709,754.108986864429,755.108722875149,756.108458885869,
757.108194896589,758.107930907309,759.107666918029,760.107402928749,761.10713893947,
762.10687495019,763.10661096091,764.10634697163,765.10608298235,766.10581899307,
767.10555500379,768.10529101451,769.105027025231,770.104763035951,771.104499046671,
772.104235057391,773.103971068111,774.103707078831,775.103443089551,776.103179100272,
777.102915110992,778.102651121712,779.102387132432,780.102123143152,781.101859153872,
782.101595164592,783.101331175312,784.101067186033,785.100803196753,786.100539207473,
787.100275218193,788.100011228913,789.099747239633,790.099483250353,791.099219261073,
792.098955271794,793.098691282514,794.098427293234,795.098163303954,796.097899314674,
797.097635325394,798.097371336114,799.097107346834,800.096843357555,801.096579368275,
802.096315378995,803.096051389715,804.095787400435,805.095523411155,806.095259421875,
807.094995432596,808.094731443316,809.094467454036,810.094203464756,811.093939475476,
812.093675486196,813.093411496916,814.093147507636,815.092883518357,816.092619529077,
817.092355539797,818.092091550517,819.091827561237,820.091563571957,821.091299582677,
822.091035593397,823.090771604118,824.090507614838,825.090243625558,826.089979636278,
827.089715646998,828.089451657718,829.089187668438,830.088923679158,831.088659689879,
832.088395700599,833.088131711319,834.087867722039,835.087603732759,836.087339743479,
837.087075754199,838.08681176492,839.08654777564,840.08628378636,841.08601979708,
842.0857558078,843.08549181852,844.08522782924,845.08496383996,846.084699850681,
847.084435861401,848.084171872121,849.083907882841,850.083643893561,851.083379904281,
852.083115915001,853.082851925721,854.082587936442,855.082323947162,856.082059957882,
857.081795968602,858.081531979322,859.081267990042,860.081004000762,861.080740011482,
862.080476022203,863.080212032923,864.079948043643,865.079684054363,866.079420065083,
867.079156075803,868.078892086523,869.078628097243,870.078364107964,871.078100118684,
872.077836129404,873.077572140124,874.077308150844,875.077044161564,876.076780172284,
877.076516183005,878.076252193725,879.075988204445,880.075724215165,881.075460225885,
882.075196236605,883.074932247325,884.074668258045,885.074404268766,886.074140279486,
887.073876290206,888.073612300926,889.073348311646,890.073084322366,891.072820333086,
892.072556343806,893.072292354527,894.072028365247,895.071764375967,896.071500386687,
897.071236397407,898.070972408127,899.070708418847,900.070444429567,901.070180440288,
902.069916451008,903.069652461728,904.069388472448,905.069124483168,906.068860493888,
907.068596504608,908.068332515329,909.068068526049,910.067804536769,911.067540547489,
912.067276558209,913.067012568929,914.066748579649,915.066484590369,916.06622060109,
917.06595661181,918.06569262253,919.06542863325,920.06516464397,921.06490065469,
922.06463666541,923.06437267613,924.064108686851,925.063844697571,926.063580708291,
927.063316719011,928.063052729731,929.062788740451,930.062524751171,931.062260761891,
932.061996772612,933.061732783332,934.061468794052,935.061204804772,936.060940815492,
937.060676826212,938.060412836932,939.060148847652,940.059884858373,941.059620869093,
942.059356879813,943.059092890533,944.058828901253,945.058564911973,946.058300922693,
947.058036933414,948.057772944134,949.057508954854,950.057244965574,951.056980976294,
952.056716987014,953.056452997734,954.056189008454,955.055925019175,956.055661029895,
957.055397040615,958.055133051335,959.054869062055,960.054605072775,961.054341083495,
962.054077094215,963.053813104936,964.053549115656,965.053285126376,966.053021137096,
967.052757147816,968.052493158536,969.052229169256,970.051965179976,971.051701190697,
972.051437201417,973.051173212137,974.050909222857,975.050645233577,976.050381244297,
977.050117255017,978.049853265738,979.049589276458,980.049325287178,981.049061297898,
982.048797308618,983.048533319338,984.048269330058,985.048005340778,986.047741351499,
987.047477362219,988.047213372939,989.046949383659,990.046685394379,991.046421405099,
992.046157415819,993.045893426539,994.04562943726,995.04536544798,996.0451014587,
997.04483746942,998.04457348014,999.04430949086,1000.04404550158,1001.0437815123,
1002.04351752302,1003.04325353374,1004.04298954446,1005.04272555518,1006.0424615659,
1007.04219757662,1008.04193358734,1009.04166959806,1010.04140560878,1011.0411416195,
1012.04087763022,1013.04061364094,1014.04034965166,1015.04008566238,1016.0398216731,
1017.03955768382,1018.03929369454,1019.03902970526,1020.03876571598,1021.0385017267,
1022.03823773742,1023.03797374814,1024.03770975886,1025.03744576958,1026.0371817803,
1027.03691779102,1028.03665380174,1029.03638981246,1030.03612582318,1031.0358618339,
1032.03559784462,1033.03533385534,1034.03506986606,1035.03480587678,1036.03454188751,
1037.03427789823,1038.03401390895,1039.03374991967,1040.03348593039,1041.03322194111,
1042.03295795183,1043.03269396255,1044.03242997327,1045.03216598399,1046.03190199471,
1047.03163800543,1048.03137401615,1049.03111002687,1050.03084603759,1051.03058204831,
1052.03031805903,1053.03005406975,1054.02979008047,1055.02952609119,1056.02926210191,
1057.02899811263,1058.02873412335,1059.02847013407,1060.02820614479,1061.02794215551,
1062.02767816623,1063.02741417695,1064.02715018767,1065.02688619839,1066.02662220911,
1067.02635821983,1068.02609423055,1069.02583024127,1070.02556625199,1071.02530226271,
1072.02503827343,1073.02477428415,1074.02451029487,1075.02424630559,1076.02398231631,
1077.02371832703,1078.02345433775,1079.02319034847,1080.02292635919,1081.02266236991,
1082.02239838063,1083.02213439135,1084.02187040207,1085.02160641279,1086.02134242351,
1087.02107843423,1088.02081444495,1089.02055045567,1090.02028646639,1091.02002247711,
1092.01975848783,1093.01949449855,1094.01923050927,1095.01896651999,1096.01870253071,
1097.01843854143,1098.01817455215,1099.01791056287,1100.01764657359,1101.01738258431,
1102.01711859503,1103.01685460575,1104.01659061647,1105.01632662719,1106.01606263791,
1107.01579864863,1108.01553465935,1109.01527067007,1110.01500668079,1111.01474269151,
1112.01447870223,1113.01421471295,1114.01395072368,1115.0136867344,1116.01342274512,
1117.01315875584,1118.01289476656,1119.01263077728,1120.012366788,1121.01210279872,
1122.01183880944,1123.01157482016,1124.01131083088,1125.0110468416,1126.01078285232,
1127.01051886304,1128.01025487376,1129.00999088448,1130.0097268952,1131.00946290592,
1132.00919891664,1133.00893492736,1134.00867093808,1135.0084069488,1136.00814295952,
1137.00787897024,1138.00761498096,1139.00735099168,1140.0070870024,1141.00682301312,
1142.00655902384,1143.00629503456,1144.00603104528,1145.005767056,1146.00550306672,
1147.00523907744,1148.00497508816,1149.00471109888,1150.0044471096,1151.00418312032,
1152.00391913104,1153.00365514176,1154.00339115248,1155.0031271632,1156.00286317392,
1157.00259918464,1158.00233519536,1159.00207120608,1160.0018072168,1161.00154322752,
1162.00127923824,1163.00101524896,1164.00075125968,1165.0004872704,1166.00022328112,
1166.99995929184,1167.99969530256,1168.99943131328,1169.999167324,1170.99890333472,
1171.99863934544,1172.99837535616,1173.99811136688,1174.9978473776,1175.99758338832,
1176.99731939904,1177.99705540976,1178.99679142048,1179.9965274312,1180.99626344192,
1181.99599945264,1182.99573546336,1183.99547147408,1184.9952074848,1185.99494349552,
1186.99467950624,1187.99441551696,1188.99415152768,1189.99388753841,1190.99362354913,
1191.99335955985,1192.99309557057,1193.99283158129,1194.99256759201,1195.99230360273,
1196.99203961345,1197.99177562417,1198.99151163489,1199.99124764561,1200.99098365633,
1201.99071966705,1202.99045567777,1203.99019168849,1204.98992769921,1205.98966370993,
1206.98939972065,1207.98913573137,1208.98887174209,1209.98860775281,1210.98834376353,
1211.98807977425,1212.98781578497,1213.98755179569,1214.98728780641,1215.98702381713,
1216.98675982785,1217.98649583857,1218.98623184929,1219.98596786001,1220.98570387073,
1221.98543988145,1222.98517589217,1223.98491190289,1224.98464791361,1225.98438392433,
1226.98411993505,1227.98385594577,1228.98359195649,1229.98332796721,1230.98306397793,
1231.98279998865,1232.98253599937,1233.98227201009,1234.98200802081,1235.98174403153,
1236.98148004225,1237.98121605297,1238.98095206369,1239.98068807441,1240.98042408513,
1241.98016009585,1242.97989610657,1243.97963211729,1244.97936812801,1245.97910413873,
1246.97884014945,1247.97857616017,1248.97831217089,1249.97804818161,1250.97778419233,
1251.97752020305,1252.97725621377,1253.97699222449,1254.97672823521,1255.97646424593,
1256.97620025665,1257.97593626737,1258.97567227809,1259.97540828881,1260.97514429953,
1261.97488031025,1262.97461632097,1263.97435233169,1264.97408834241,1265.97382435313,
1266.97356036385,1267.97329637458,1268.9730323853,1269.97276839602,1270.97250440674,
1271.97224041746,1272.97197642818,1273.9717124389,1274.97144844962,1275.97118446034,
1276.97092047106,1277.97065648178,1278.9703924925,1279.97012850322,1280.96986451394,
1281.96960052466,1282.96933653538,1283.9690725461,1284.96880855682,1285.96854456754,
1286.96828057826,1287.96801658898,1288.9677525997,1289.96748861042,1290.96722462114,
1291.96696063186,1292.96669664258,1293.9664326533,1294.96616866402,1295.96590467474,
1296.96564068546,1297.96537669618,1298.9651127069,1299.96484871762,1300.96458472834,
1301.96432073906,1302.96405674978,1303.9637927605,1304.96352877122,1305.96326478194,
1306.96300079266,1307.96273680338,1308.9624728141,1309.96220882482,1310.96194483554,
1311.96168084626,1312.96141685698,1313.9611528677,1314.96088887842,1315.96062488914,
1316.96036089986,1317.96009691058,1318.9598329213,1319.95956893202,1320.95930494274,
1321.95904095346,1322.95877696418,1323.9585129749,1324.95824898562,1325.95798499634,
1326.95772100706,1327.95745701778,1328.9571930285,1329.95692903922,1330.95666504994,
1331.95640106066,1332.95613707138,1333.9558730821,1334.95560909282,1335.95534510354,
1336.95508111426,1337.95481712498,1338.9545531357,1339.95428914642,1340.95402515714,
1341.95376116786,1342.95349717858,1343.9532331893,1344.95296920002,1345.95270521075,
1346.95244122147,1347.95217723219,1348.95191324291,1349.95164925363,1350.95138526435,
1351.95112127507,1352.95085728579,1353.95059329651,1354.95032930723,1355.95006531795,
1356.94980132867,1357.94953733939,1358.94927335011,1359.94900936083,1360.94874537155,
1361.94848138227,1362.94821739299,1363.94795340371,1364.94768941443,1365.94742542515,
1366.94716143587,1367.94689744659,1368.94663345731,1369.94636946803,1370.94610547875,
1371.94584148947,1372.94557750019,1373.94531351091,1374.94504952163,1375.94478553235,
1376.94452154307,1377.94425755379,1378.94399356451,1379.94372957523,1380.94346558595,
1381.94320159667,1382.94293760739,1383.94267361811,1384.94240962883,1385.94214563955,
1386.94188165027,1387.94161766099,1388.94135367171,1389.94108968243,1390.94082569315,
1391.94056170387,1392.94029771459,1393.94003372531,1394.93976973603,1395.93950574675,
1396.93924175747,1397.93897776819,1398.93871377891,1399.93844978963,1400.93818580035,
1401.93792181107,1402.93765782179,1403.93739383251,1404.93712984323,1405.93686585395,
1406.93660186467,1407.93633787539,1408.93607388611,1409.93580989683,1410.93554590755,
1411.93528191827,1412.93501792899,1413.93475393971,1414.93448995043,1415.93422596115,
1416.93396197187,1417.93369798259,1418.93343399331,1419.93317000403,1420.93290601475,
1421.93264202547,1422.93237803619,1423.93211404692,1424.93185005764,1425.93158606836,
1426.93132207908,1427.9310580898,1428.93079410052,1429.93053011124,1430.93026612196,
1431.93000213268,1432.9297381434,1433.92947415412,1434.92921016484,1435.92894617556,
1436.92868218628,1437.928418197,1438.92815420772,1439.92789021844,1440.92762622916,
1441.92736223988,1442.9270982506,1443.92683426132,1444.92657027204,1445.92630628276,
1446.92604229348,1447.9257783042,1448.92551431492,1449.92525032564,1450.92498633636,
1451.92472234708,1452.9244583578,1453.92419436852,1454.92393037924,1455.92366638996,
1456.92340240068,1457.9231384114,1458.92287442212,1459.92261043284,1460.92234644356,
1461.92208245428,1462.921818465,1463.92155447572,1464.92129048644,1465.92102649716,
1466.92076250788,1467.9204985186,1468.92023452932,1469.91997054004,1470.91970655076,
1471.91944256148,1472.9191785722,1473.91891458292,1474.91865059364,1475.91838660436,
1476.91812261508,1477.9178586258,1478.91759463652,1479.91733064724,1480.91706665796,
1481.91680266868,1482.9165386794,1483.91627469012,1484.91601070084,1485.91574671156,
1486.91548272228,1487.915218733,1488.91495474372,1489.91469075444,1490.91442676516,
1491.91416277588,1492.9138987866,1493.91363479732,1494.91337080804,1495.91310681876,
1496.91284282948,1497.9125788402,1498.91231485092,1499.91205086164,1500.91178687236,
1501.91152288309,1502.91125889381,1503.91099490453,1504.91073091525,1505.91046692597,
1506.91020293669,1507.90993894741,1508.90967495813,1509.90941096885,1510.90914697957,
1511.90888299029,1512.90861900101,1513.90835501173,1514.90809102245,1515.90782703317,
1516.90756304389,1517.90729905461,1518.90703506533,1519.90677107605,1520.90650708677,
1521.90624309749,1522.90597910821,1523.90571511893,1524.90545112965,1525.90518714037,
1526.90492315109,1527.90465916181,1528.90439517253,1529.90413118325,1530.90386719397,
1531.90360320469,1532.90333921541,1533.90307522613,1534.90281123685,1535.90254724757,
1536.90228325829,1537.90201926901,1538.90175527973,1539.90149129045,1540.90122730117,
1541.90096331189,1542.90069932261,1543.90043533333,1544.90017134405,1545.89990735477,
1546.89964336549,1547.89937937621,1548.89911538693,1549.89885139765,1550.89858740837,
1551.89832341909,1552.89805942981,1553.89779544053,1554.89753145125,1555.89726746197,
1556.89700347269,1557.89673948341,1558.89647549413,1559.89621150485,1560.89594751557,
1561.89568352629,1562.89541953701,1563.89515554773,1564.89489155845,1565.89462756917,
1566.89436357989,1567.89409959061,1568.89383560133,1569.89357161205,1570.89330762277,
1571.89304363349,1572.89277964421,1573.89251565493,1574.89225166565,1575.89198767637,
1576.89172368709,1577.89145969781,1578.89119570853,1579.89093171926,1580.89066772998,
1581.8904037407,1582.89013975142,1583.88987576214,1584.88961177286,1585.88934778358,
1586.8890837943,1587.88881980502,1588.88855581574,1589.88829182646,1590.88802783718,
1591.8877638479,1592.88749985862,1593.88723586934,1594.88697188006,1595.88670789078,
1596.8864439015,1597.88617991222,1598.88591592294,1599.88565193366,1600.88538794438,
1601.8851239551,1602.88485996582,1603.88459597654,1604.88433198726,1605.88406799798,
1606.8838040087,1607.88354001942,1608.88327603014,1609.88301204086,1610.88274805158,
1611.8824840623,1612.88222007302,1613.88195608374,1614.88169209446,1615.88142810518,
1616.8811641159,1617.88090012662,1618.88063613734,1619.88037214806,1620.88010815878,
1621.8798441695,1622.87958018022,1623.87931619094,1624.87905220166,1625.87878821238,
1626.8785242231,1627.87826023382,1628.87799624454,1629.87773225526,1630.87746826598,
1631.8772042767,1632.87694028742,1633.87667629814,1634.87641230886,1635.87614831958,
1636.8758843303,1637.87562034102,1638.87535635174,1639.87509236246,1640.87482837318,
1641.8745643839,1642.87430039462,1643.87403640534,1644.87377241606,1645.87350842678,
1646.8732444375,1647.87298044822,1648.87271645894,1649.87245246966,1650.87218848038,
1651.8719244911,1652.87166050182,1653.87139651254,1654.87113252326,1655.87086853399,
1656.8706045447,1657.87034055543,1658.87007656615,1659.86981257687,1660.86954858759,
1661.86928459831,1662.86902060903,1663.86875661975,1664.86849263047,1665.86822864119,
1666.86796465191,1667.86770066263,1668.86743667335,1669.86717268407,1670.86690869479,
1671.86664470551,1672.86638071623,1673.86611672695,1674.86585273767,1675.86558874839,
1676.86532475911,1677.86506076983,1678.86479678055,1679.86453279127,1680.86426880199,
1681.86400481271,1682.86374082343,1683.86347683415,1684.86321284487,1685.86294885559,
1686.86268486631,1687.86242087703,1688.86215688775,1689.86189289847,1690.86162890919,
1691.86136491991,1692.86110093063,1693.86083694135,1694.86057295207,1695.86030896279,
1696.86004497351,1697.35991297887,1697.85988790214),.UNSPECIFIED.);
#52=B_SPLINE_SURFACE_WITH_KNOTS('',3,3,((#233503,#233504,#233505,#233506,
#233507,#233508,#233509,#233510,#233511,#233512,#233513,#233514,#233515,
#233516,#233517,#233518,#233519,#233520,#233521,#233522,#233523,#233524,
#233525,#233526,#233527,#233528,#233529,#233530,#233531,#233532,#233533,
#233534,#233535,#233536,#233537,#233538,#233539,#233540,#233541,#233542,
#233543,#233544,#233545,#233546,#233547,#233548,#233549,#233550,#233551,
#233552,#233553,#233554,#233555,#233556,#233557,#233558,#233559,#233560,
#233561,#233562,#233563,#233564,#233565,#233566,#233567,#233568,#233569,
#233570,#233571,#233572,#233573,#233574,#233575,#233576,#233577,#233578,
#233579,#233580,#233581,#233582,#233583,#233584,#233585,#233586,#233587,
#233588,#233589,#233590,#233591,#233592,#233593,#233594,#233595,#233596,
#233597,#233598,#233599,#233600,#233601,#233602,#233603,#233604,#233605,
#233606,#233607,#233608,#233609,#233610,#233611,#233612,#233613,#233614,
#233615,#233616,#233617,#233618,#233619,#233620,#233621,#233622,#233623,
#233624,#233625,#233626,#233627,#233628,#233629,#233630,#233631,#233632,
#233633,#233634,#233635,#233636,#233637,#233638,#233639,#233640,#233641,
#233642,#233643,#233644,#233645,#233646,#233647,#233648,#233649,#233650,
#233651,#233652,#233653,#233654,#233655,#233656,#233657,#233658,#233659,
#233660,#233661,#233662,#233663,#233664,#233665,#233666,#233667,#233668,
#233669,#233670,#233671,#233672,#233673,#233674,#233675,#233676,#233677,
#233678,#233679,#233680,#233681,#233682,#233683,#233684,#233685,#233686,
#233687,#233688,#233689,#233690,#233691,#233692,#233693,#233694,#233695,
#233696,#233697,#233698,#233699,#233700,#233701,#233702,#233703,#233704,
#233705,#233706,#233707,#233708,#233709,#233710,#233711,#233712,#233713,
#233714,#233715,#233716,#233717,#233718,#233719,#233720,#233721,#233722,
#233723,#233724,#233725,#233726,#233727,#233728,#233729,#233730,#233731,
#233732,#233733,#233734,#233735,#233736,#233737,#233738,#233739,#233740,
#233741,#233742,#233743,#233744,#233745,#233746,#233747,#233748,#233749,
#233750,#233751,#233752,#233753,#233754,#233755,#233756,#233757,#233758,
#233759,#233760,#233761,#233762,#233763,#233764,#233765,#233766,#233767,
#233768,#233769,#233770,#233771,#233772,#233773,#233774,#233775,#233776,
#233777,#233778,#233779,#233780,#233781,#233782,#233783,#233784,#233785,
#233786,#233787,#233788,#233789,#233790,#233791,#233792,#233793,#233794,
#233795,#233796,#233797,#233798,#233799,#233800,#233801,#233802,#233803,
#233804,#233805,#233806,#233807,#233808,#233809,#233810,#233811,#233812,
#233813,#233814,#233815,#233816,#233817,#233818,#233819,#233820,#233821,
#233822,#233823,#233824,#233825,#233826,#233827,#233828,#233829,#233830,
#233831,#233832,#233833,#233834,#233835,#233836,#233837,#233838,#233839,
#233840,#233841,#233842,#233843,#233844,#233845,#233846,#233847,#233848,
#233849,#233850,#233851,#233852,#233853,#233854,#233855,#233856,#233857,
#233858,#233859,#233860,#233861,#233862,#233863,#233864,#233865,#233866,
#233867,#233868,#233869,#233870,#233871,#233872,#233873,#233874,#233875,
#233876,#233877,#233878,#233879,#233880,#233881,#233882,#233883,#233884,
#233885,#233886,#233887,#233888,#233889,#233890,#233891,#233892,#233893,
#233894,#233895,#233896,#233897,#233898,#233899,#233900,#233901,#233902,
#233903,#233904,#233905,#233906,#233907,#233908,#233909,#233910,#233911,
#233912,#233913,#233914,#233915,#233916,#233917,#233918,#233919,#233920,
#233921,#233922,#233923,#233924,#233925,#233926,#233927,#233928,#233929,
#233930,#233931,#233932,#233933,#233934,#233935,#233936,#233937,#233938,
#233939,#233940,#233941,#233942,#233943,#233944,#233945,#233946,#233947,
#233948,#233949,#233950,#233951,#233952,#233953,#233954,#233955,#233956,
#233957,#233958,#233959,#233960,#233961,#233962,#233963,#233964,#233965,
#233966,#233967,#233968,#233969,#233970,#233971,#233972,#233973,#233974,
#233975,#233976,#233977,#233978,#233979,#233980,#233981,#233982,#233983,
#233984,#233985,#233986,#233987,#233988,#233989,#233990,#233991,#233992,
#233993,#233994,#233995,#233996,#233997,#233998,#233999,#234000,#234001,
#234002,#234003,#234004,#234005,#234006,#234007,#234008,#234009,#234010,
#234011,#234012,#234013,#234014,#234015,#234016,#234017,#234018,#234019,
#234020,#234021,#234022,#234023,#234024,#234025,#234026,#234027,#234028,
#234029,#234030,#234031,#234032,#234033,#234034,#234035,#234036,#234037,
#234038,#234039,#234040,#234041,#234042,#234043,#234044,#234045,#234046,
#234047,#234048,#234049,#234050,#234051,#234052,#234053,#234054,#234055,
#234056,#234057,#234058,#234059,#234060,#234061,#234062,#234063,#234064,
#234065,#234066,#234067,#234068,#234069,#234070,#234071,#234072,#234073,
#234074,#234075,#234076,#234077,#234078,#234079,#234080,#234081,#234082,
#234083,#234084,#234085,#234086,#234087,#234088,#234089,#234090,#234091,
#234092,#234093,#234094,#234095,#234096,#234097,#234098,#234099,#234100,
#234101,#234102,#234103,#234104,#234105,#234106,#234107,#234108,#234109,
#234110,#234111,#234112,#234113,#234114,#234115,#234116,#234117,#234118,
#234119,#234120,#234121,#234122,#234123,#234124,#234125,#234126,#234127,
#234128,#234129,#234130,#234131,#234132,#234133,#234134,#234135,#234136,
#234137,#234138,#234139,#234140,#234141,#234142,#234143,#234144,#234145,
#234146,#234147,#234148,#234149,#234150,#234151,#234152,#234153,#234154,
#234155,#234156,#234157,#234158,#234159,#234160,#234161,#234162,#234163,
#234164,#234165,#234166,#234167,#234168,#234169,#234170,#234171,#234172,
#234173,#234174,#234175,#234176,#234177,#234178,#234179,#234180,#234181,
#234182,#234183,#234184,#234185,#234186,#234187,#234188,#234189,#234190,
#234191,#234192,#234193,#234194,#234195,#234196,#234197,#234198,#234199,
#234200,#234201,#234202,#234203,#234204,#234205,#234206,#234207,#234208,
#234209,#234210,#234211,#234212,#234213,#234214,#234215,#234216,#234217,
#234218,#234219,#234220,#234221,#234222,#234223,#234224,#234225,#234226,
#234227,#234228,#234229,#234230,#234231,#234232,#234233,#234234,#234235,
#234236,#234237,#234238,#234239,#234240,#234241,#234242,#234243,#234244,
#234245,#234246,#234247,#234248,#234249,#234250,#234251,#234252,#234253,
#234254,#234255,#234256,#234257,#234258,#234259,#234260,#234261,#234262,
#234263,#234264,#234265,#234266,#234267,#234268,#234269,#234270,#234271,
#234272,#234273,#234274,#234275,#234276,#234277,#234278,#234279,#234280,
#234281,#234282,#234283,#234284,#234285,#234286,#234287,#234288,#234289,
#234290,#234291,#234292,#234293,#234294,#234295,#234296,#234297,#234298,
#234299,#234300,#234301,#234302,#234303,#234304,#234305,#234306,#234307,
#234308,#234309,#234310,#234311,#234312,#234313,#234314,#234315,#234316,
#234317,#234318,#234319,#234320,#234321,#234322,#234323,#234324,#234325,
#234326,#234327,#234328,#234329,#234330,#234331,#234332,#234333,#234334,
#234335,#234336,#234337,#234338,#234339,#234340,#234341,#234342,#234343,
#234344,#234345,#234346,#234347,#234348,#234349,#234350,#234351,#234352,
#234353,#234354,#234355,#234356,#234357,#234358,#234359,#234360,#234361,
#234362,#234363,#234364,#234365,#234366,#234367,#234368,#234369,#234370,
#234371,#234372,#234373,#234374,#234375,#234376,#234377,#234378,#234379,
#234380,#234381,#234382,#234383,#234384,#234385,#234386,#234387,#234388,
#234389,#234390,#234391,#234392,#234393,#234394,#234395,#234396,#234397,
#234398,#234399,#234400,#234401,#234402,#234403,#234404,#234405,#234406,
#234407,#234408,#234409,#234410,#234411,#234412,#234413,#234414,#234415,
#234416,#234417,#234418,#234419,#234420,#234421,#234422,#234423,#234424,
#234425,#234426,#234427,#234428,#234429,#234430,#234431,#234432,#234433,
#234434,#234435,#234436,#234437,#234438,#234439,#234440,#234441,#234442,
#234443,#234444,#234445,#234446,#234447,#234448,#234449,#234450,#234451,
#234452,#234453,#234454,#234455,#234456,#234457,#234458,#234459,#234460,
#234461,#234462,#234463,#234464,#234465,#234466,#234467,#234468,#234469,
#234470,#234471,#234472,#234473,#234474,#234475,#234476,#234477,#234478,
#234479,#234480,#234481,#234482,#234483,#234484,#234485,#234486,#234487,
#234488,#234489,#234490,#234491,#234492,#234493,#234494,#234495,#234496,
#234497,#234498,#234499,#234500,#234501,#234502,#234503,#234504,#234505,
#234506,#234507,#234508,#234509,#234510,#234511,#234512,#234513,#234514,
#234515,#234516,#234517,#234518,#234519,#234520,#234521,#234522,#234523,
#234524,#234525,#234526,#234527,#234528,#234529,#234530,#234531,#234532,
#234533,#234534,#234535,#234536,#234537,#234538,#234539,#234540,#234541,
#234542,#234543,#234544,#234545,#234546,#234547,#234548,#234549,#234550,
#234551,#234552,#234553,#234554,#234555,#234556,#234557,#234558,#234559,
#234560,#234561,#234562,#234563,#234564,#234565,#234566,#234567,#234568,
#234569,#234570,#234571,#234572,#234573,#234574,#234575,#234576,#234577,
#234578,#234579,#234580,#234581,#234582,#234583,#234584,#234585,#234586,
#234587,#234588,#234589,#234590,#234591,#234592,#234593,#234594,#234595,
#234596,#234597,#234598,#234599,#234600,#234601,#234602,#234603,#234604,
#234605,#234606,#234607,#234608,#234609,#234610,#234611,#234612,#234613,
#234614,#234615,#234616,#234617,#234618,#234619,#234620,#234621,#234622,
#234623,#234624,#234625,#234626,#234627,#234628,#234629,#234630,#234631,
#234632,#234633,#234634,#234635,#234636,#234637,#234638,#234639,#234640,
#234641,#234642,#234643,#234644,#234645,#234646,#234647,#234648,#234649,
#234650,#234651,#234652,#234653,#234654,#234655,#234656,#234657,#234658,
#234659,#234660,#234661,#234662,#234663,#234664,#234665,#234666,#234667,
#234668,#234669,#234670,#234671,#234672,#234673,#234674,#234675,#234676,
#234677,#234678,#234679,#234680,#234681,#234682,#234683,#234684,#234685,
#234686,#234687,#234688,#234689,#234690,#234691,#234692,#234693,#234694,
#234695,#234696,#234697,#234698,#234699,#234700,#234701,#234702,#234703,
#234704,#234705,#234706,#234707,#234708,#234709,#234710,#234711,#234712,
#234713,#234714,#234715,#234716,#234717,#234718,#234719,#234720,#234721,
#234722,#234723,#234724,#234725,#234726,#234727,#234728,#234729,#234730,
#234731,#234732,#234733,#234734,#234735,#234736,#234737,#234738,#234739,
#234740,#234741,#234742,#234743,#234744,#234745,#234746,#234747,#234748,
#234749,#234750,#234751,#234752,#234753,#234754,#234755,#234756,#234757,
#234758,#234759,#234760,#234761,#234762,#234763,#234764,#234765,#234766,
#234767,#234768,#234769,#234770,#234771,#234772,#234773,#234774,#234775,
#234776,#234777,#234778,#234779,#234780,#234781,#234782,#234783,#234784,
#234785,#234786,#234787,#234788,#234789,#234790,#234791,#234792,#234793,
#234794,#234795,#234796,#234797,#234798,#234799,#234800,#234801,#234802,
#234803,#234804,#234805,#234806,#234807,#234808,#234809,#234810,#234811,
#234812,#234813,#234814,#234815,#234816,#234817,#234818,#234819,#234820,
#234821,#234822,#234823,#234824,#234825,#234826,#234827,#234828,#234829,
#234830,#234831,#234832,#234833,#234834,#234835,#234836,#234837,#234838,
#234839,#234840,#234841,#234842,#234843,#234844,#234845,#234846,#234847,
#234848,#234849,#234850,#234851,#234852,#234853,#234854,#234855,#234856,
#234857,#234858,#234859,#234860,#234861,#234862,#234863,#234864,#234865,
#234866,#234867,#234868,#234869,#234870,#234871,#234872,#234873,#234874,
#234875,#234876,#234877,#234878,#234879,#234880,#234881,#234882,#234883,
#234884,#234885,#234886,#234887,#234888,#234889,#234890,#234891,#234892,
#234893,#234894,#234895,#234896,#234897,#234898,#234899,#234900,#234901,
#234902,#234903,#234904,#234905,#234906,#234907,#234908,#234909,#234910,
#234911,#234912,#234913,#234914,#234915,#234916,#234917,#234918,#234919,
#234920,#234921,#234922,#234923,#234924,#234925,#234926,#234927,#234928,
#234929,#234930,#234931,#234932,#234933,#234934,#234935,#234936,#234937,
#234938,#234939,#234940,#234941,#234942,#234943,#234944,#234945,#234946,
#234947,#234948,#234949,#234950,#234951,#234952,#234953,#234954,#234955,
#234956,#234957,#234958,#234959,#234960,#234961,#234962,#234963,#234964,
#234965,#234966,#234967,#234968,#234969,#234970,#234971,#234972,#234973,
#234974,#234975,#234976,#234977,#234978,#234979,#234980,#234981,#234982,
#234983,#234984,#234985,#234986,#234987,#234988,#234989,#234990,#234991,
#234992,#234993,#234994,#234995,#234996,#234997,#234998,#234999,#235000,
#235001,#235002,#235003,#235004,#235005,#235006,#235007,#235008,#235009,
#235010,#235011,#235012,#235013,#235014,#235015,#235016,#235017,#235018,
#235019,#235020,#235021,#235022,#235023,#235024,#235025,#235026,#235027,
#235028,#235029,#235030,#235031,#235032,#235033,#235034,#235035,#235036,
#235037,#235038,#235039,#235040,#235041,#235042,#235043,#235044,#235045,
#235046,#235047,#235048,#235049,#235050,#235051,#235052,#235053,#235054,
#235055,#235056,#235057,#235058,#235059,#235060,#235061,#235062,#235063,
#235064,#235065,#235066,#235067,#235068,#235069,#235070,#235071,#235072,
#235073,#235074,#235075,#235076,#235077,#235078,#235079,#235080,#235081,
#235082,#235083,#235084,#235085,#235086,#235087,#235088,#235089,#235090,
#235091,#235092,#235093,#235094,#235095,#235096,#235097,#235098,#235099,
#235100,#235101,#235102,#235103,#235104,#235105,#235106,#235107,#235108,
#235109,#235110,#235111,#235112,#235113,#235114,#235115,#235116,#235117,
#235118,#235119,#235120,#235121,#235122,#235123,#235124,#235125,#235126,
#235127,#235128,#235129,#235130,#235131,#235132,#235133,#235134,#235135,
#235136,#235137,#235138,#235139,#235140,#235141,#235142,#235143,#235144,
#235145,#235146,#235147,#235148,#235149,#235150,#235151,#235152,#235153,
#235154,#235155,#235156,#235157,#235158,#235159,#235160,#235161,#235162,
#235163,#235164,#235165,#235166,#235167,#235168,#235169,#235170,#235171,
#235172,#235173,#235174,#235175,#235176,#235177,#235178,#235179,#235180,
#235181,#235182,#235183,#235184,#235185,#235186,#235187,#235188,#235189,
#235190,#235191,#235192,#235193,#235194,#235195,#235196,#235197),(#235198,
#235199,#235200,#235201,#235202,#235203,#235204,#235205,#235206,#235207,
#235208,#235209,#235210,#235211,#235212,#235213,#235214,#235215,#235216,
#235217,#235218,#235219,#235220,#235221,#235222,#235223,#235224,#235225,
#235226,#235227,#235228,#235229,#235230,#235231,#235232,#235233,#235234,
#235235,#235236,#235237,#235238,#235239,#235240,#235241,#235242,#235243,
#235244,#235245,#235246,#235247,#235248,#235249,#235250,#235251,#235252,
#235253,#235254,#235255,#235256,#235257,#235258,#235259,#235260,#235261,
#235262,#235263,#235264,#235265,#235266,#235267,#235268,#235269,#235270,
#235271,#235272,#235273,#235274,#235275,#235276,#235277,#235278,#235279,
#235280,#235281,#235282,#235283,#235284,#235285,#235286,#235287,#235288,
#235289,#235290,#235291,#235292,#235293,#235294,#235295,#235296,#235297,
#235298,#235299,#235300,#235301,#235302,#235303,#235304,#235305,#235306,
#235307,#235308,#235309,#235310,#235311,#235312,#235313,#235314,#235315,
#235316,#235317,#235318,#235319,#235320,#235321,#235322,#235323,#235324,
#235325,#235326,#235327,#235328,#235329,#235330,#235331,#235332,#235333,
#235334,#235335,#235336,#235337,#235338,#235339,#235340,#235341,#235342,
#235343,#235344,#235345,#235346,#235347,#235348,#235349,#235350,#235351,
#235352,#235353,#235354,#235355,#235356,#235357,#235358,#235359,#235360,
#235361,#235362,#235363,#235364,#235365,#235366,#235367,#235368,#235369,
#235370,#235371,#235372,#235373,#235374,#235375,#235376,#235377,#235378,
#235379,#235380,#235381,#235382,#235383,#235384,#235385,#235386,#235387,
#235388,#235389,#235390,#235391,#235392,#235393,#235394,#235395,#235396,
#235397,#235398,#235399,#235400,#235401,#235402,#235403,#235404,#235405,
#235406,#235407,#235408,#235409,#235410,#235411,#235412,#235413,#235414,
#235415,#235416,#235417,#235418,#235419,#235420,#235421,#235422,#235423,
#235424,#235425,#235426,#235427,#235428,#235429,#235430,#235431,#235432,
#235433,#235434,#235435,#235436,#235437,#235438,#235439,#235440,#235441,
#235442,#235443,#235444,#235445,#235446,#235447,#235448,#235449,#235450,
#235451,#235452,#235453,#235454,#235455,#235456,#235457,#235458,#235459,
#235460,#235461,#235462,#235463,#235464,#235465,#235466,#235467,#235468,
#235469,#235470,#235471,#235472,#235473,#235474,#235475,#235476,#235477,
#235478,#235479,#235480,#235481,#235482,#235483,#235484,#235485,#235486,
#235487,#235488,#235489,#235490,#235491,#235492,#235493,#235494,#235495,
#235496,#235497,#235498,#235499,#235500,#235501,#235502,#235503,#235504,
#235505,#235506,#235507,#235508,#235509,#235510,#235511,#235512,#235513,
#235514,#235515,#235516,#235517,#235518,#235519,#235520,#235521,#235522,
#235523,#235524,#235525,#235526,#235527,#235528,#235529,#235530,#235531,
#235532,#235533,#235534,#235535,#235536,#235537,#235538,#235539,#235540,
#235541,#235542,#235543,#235544,#235545,#235546,#235547,#235548,#235549,
#235550,#235551,#235552,#235553,#235554,#235555,#235556,#235557,#235558,
#235559,#235560,#235561,#235562,#235563,#235564,#235565,#235566,#235567,
#235568,#235569,#235570,#235571,#235572,#235573,#235574,#235575,#235576,
#235577,#235578,#235579,#235580,#235581,#235582,#235583,#235584,#235585,
#235586,#235587,#235588,#235589,#235590,#235591,#235592,#235593,#235594,
#235595,#235596,#235597,#235598,#235599,#235600,#235601,#235602,#235603,
#235604,#235605,#235606,#235607,#235608,#235609,#235610,#235611,#235612,
#235613,#235614,#235615,#235616,#235617,#235618,#235619,#235620,#235621,
#235622,#235623,#235624,#235625,#235626,#235627,#235628,#235629,#235630,
#235631,#235632,#235633,#235634,#235635,#235636,#235637,#235638,#235639,
#235640,#235641,#235642,#235643,#235644,#235645,#235646,#235647,#235648,
#235649,#235650,#235651,#235652,#235653,#235654,#235655,#235656,#235657,
#235658,#235659,#235660,#235661,#235662,#235663,#235664,#235665,#235666,
#235667,#235668,#235669,#235670,#235671,#235672,#235673,#235674,#235675,
#235676,#235677,#235678,#235679,#235680,#235681,#235682,#235683,#235684,
#235685,#235686,#235687,#235688,#235689,#235690,#235691,#235692,#235693,
#235694,#235695,#235696,#235697,#235698,#235699,#235700,#235701,#235702,
#235703,#235704,#235705,#235706,#235707,#235708,#235709,#235710,#235711,
#235712,#235713,#235714,#235715,#235716,#235717,#235718,#235719,#235720,
#235721,#235722,#235723,#235724,#235725,#235726,#235727,#235728,#235729,
#235730,#235731,#235732,#235733,#235734,#235735,#235736,#235737,#235738,
#235739,#235740,#235741,#235742,#235743,#235744,#235745,#235746,#235747,
#235748,#235749,#235750,#235751,#235752,#235753,#235754,#235755,#235756,
#235757,#235758,#235759,#235760,#235761,#235762,#235763,#235764,#235765,
#235766,#235767,#235768,#235769,#235770,#235771,#235772,#235773,#235774,
#235775,#235776,#235777,#235778,#235779,#235780,#235781,#235782,#235783,
#235784,#235785,#235786,#235787,#235788,#235789,#235790,#235791,#235792,
#235793,#235794,#235795,#235796,#235797,#235798,#235799,#235800,#235801,
#235802,#235803,#235804,#235805,#235806,#235807,#235808,#235809,#235810,
#235811,#235812,#235813,#235814,#235815,#235816,#235817,#235818,#235819,
#235820,#235821,#235822,#235823,#235824,#235825,#235826,#235827,#235828,
#235829,#235830,#235831,#235832,#235833,#235834,#235835,#235836,#235837,
#235838,#235839,#235840,#235841,#235842,#235843,#235844,#235845,#235846,
#235847,#235848,#235849,#235850,#235851,#235852,#235853,#235854,#235855,
#235856,#235857,#235858,#235859,#235860,#235861,#235862,#235863,#235864,
#235865,#235866,#235867,#235868,#235869,#235870,#235871,#235872,#235873,
#235874,#235875,#235876,#235877,#235878,#235879,#235880,#235881,#235882,
#235883,#235884,#235885,#235886,#235887,#235888,#235889,#235890,#235891,
#235892,#235893,#235894,#235895,#235896,#235897,#235898,#235899,#235900,
#235901,#235902,#235903,#235904,#235905,#235906,#235907,#235908,#235909,
#235910,#235911,#235912,#235913,#235914,#235915,#235916,#235917,#235918,
#235919,#235920,#235921,#235922,#235923,#235924,#235925,#235926,#235927,
#235928,#235929,#235930,#235931,#235932,#235933,#235934,#235935,#235936,
#235937,#235938,#235939,#235940,#235941,#235942,#235943,#235944,#235945,
#235946,#235947,#235948,#235949,#235950,#235951,#235952,#235953,#235954,
#235955,#235956,#235957,#235958,#235959,#235960,#235961,#235962,#235963,
#235964,#235965,#235966,#235967,#235968,#235969,#235970,#235971,#235972,
#235973,#235974,#235975,#235976,#235977,#235978,#235979,#235980,#235981,
#235982,#235983,#235984,#235985,#235986,#235987,#235988,#235989,#235990,
#235991,#235992,#235993,#235994,#235995,#235996,#235997,#235998,#235999,
#236000,#236001,#236002,#236003,#236004,#236005,#236006,#236007,#236008,
#236009,#236010,#236011,#236012,#236013,#236014,#236015,#236016,#236017,
#236018,#236019,#236020,#236021,#236022,#236023,#236024,#236025,#236026,
#236027,#236028,#236029,#236030,#236031,#236032,#236033,#236034,#236035,
#236036,#236037,#236038,#236039,#236040,#236041,#236042,#236043,#236044,
#236045,#236046,#236047,#236048,#236049,#236050,#236051,#236052,#236053,
#236054,#236055,#236056,#236057,#236058,#236059,#236060,#236061,#236062,
#236063,#236064,#236065,#236066,#236067,#236068,#236069,#236070,#236071,
#236072,#236073,#236074,#236075,#236076,#236077,#236078,#236079,#236080,
#236081,#236082,#236083,#236084,#236085,#236086,#236087,#236088,#236089,
#236090,#236091,#236092,#236093,#236094,#236095,#236096,#236097,#236098,
#236099,#236100,#236101,#236102,#236103,#236104,#236105,#236106,#236107,
#236108,#236109,#236110,#236111,#236112,#236113,#236114,#236115,#236116,
#236117,#236118,#236119,#236120,#236121,#236122,#236123,#236124,#236125,
#236126,#236127,#236128,#236129,#236130,#236131,#236132,#236133,#236134,
#236135,#236136,#236137,#236138,#236139,#236140,#236141,#236142,#236143,
#236144,#236145,#236146,#236147,#236148,#236149,#236150,#236151,#236152,
#236153,#236154,#236155,#236156,#236157,#236158,#236159,#236160,#236161,
#236162,#236163,#236164,#236165,#236166,#236167,#236168,#236169,#236170,
#236171,#236172,#236173,#236174,#236175,#236176,#236177,#236178,#236179,
#236180,#236181,#236182,#236183,#236184,#236185,#236186,#236187,#236188,
#236189,#236190,#236191,#236192,#236193,#236194,#236195,#236196,#236197,
#236198,#236199,#236200,#236201,#236202,#236203,#236204,#236205,#236206,
#236207,#236208,#236209,#236210,#236211,#236212,#236213,#236214,#236215,
#236216,#236217,#236218,#236219,#236220,#236221,#236222,#236223,#236224,
#236225,#236226,#236227,#236228,#236229,#236230,#236231,#236232,#236233,
#236234,#236235,#236236,#236237,#236238,#236239,#236240,#236241,#236242,
#236243,#236244,#236245,#236246,#236247,#236248,#236249,#236250,#236251,
#236252,#236253,#236254,#236255,#236256,#236257,#236258,#236259,#236260,
#236261,#236262,#236263,#236264,#236265,#236266,#236267,#236268,#236269,
#236270,#236271,#236272,#236273,#236274,#236275,#236276,#236277,#236278,
#236279,#236280,#236281,#236282,#236283,#236284,#236285,#236286,#236287,
#236288,#236289,#236290,#236291,#236292,#236293,#236294,#236295,#236296,
#236297,#236298,#236299,#236300,#236301,#236302,#236303,#236304,#236305,
#236306,#236307,#236308,#236309,#236310,#236311,#236312,#236313,#236314,
#236315,#236316,#236317,#236318,#236319,#236320,#236321,#236322,#236323,
#236324,#236325,#236326,#236327,#236328,#236329,#236330,#236331,#236332,
#236333,#236334,#236335,#236336,#236337,#236338,#236339,#236340,#236341,
#236342,#236343,#236344,#236345,#236346,#236347,#236348,#236349,#236350,
#236351,#236352,#236353,#236354,#236355,#236356,#236357,#236358,#236359,
#236360,#236361,#236362,#236363,#236364,#236365,#236366,#236367,#236368,
#236369,#236370,#236371,#236372,#236373,#236374,#236375,#236376,#236377,
#236378,#236379,#236380,#236381,#236382,#236383,#236384,#236385,#236386,
#236387,#236388,#236389,#236390,#236391,#236392,#236393,#236394,#236395,
#236396,#236397,#236398,#236399,#236400,#236401,#236402,#236403,#236404,
#236405,#236406,#236407,#236408,#236409,#236410,#236411,#236412,#236413,
#236414,#236415,#236416,#236417,#236418,#236419,#236420,#236421,#236422,
#236423,#236424,#236425,#236426,#236427,#236428,#236429,#236430,#236431,
#236432,#236433,#236434,#236435,#236436,#236437,#236438,#236439,#236440,
#236441,#236442,#236443,#236444,#236445,#236446,#236447,#236448,#236449,
#236450,#236451,#236452,#236453,#236454,#236455,#236456,#236457,#236458,
#236459,#236460,#236461,#236462,#236463,#236464,#236465,#236466,#236467,
#236468,#236469,#236470,#236471,#236472,#236473,#236474,#236475,#236476,
#236477,#236478,#236479,#236480,#236481,#236482,#236483,#236484,#236485,
#236486,#236487,#236488,#236489,#236490,#236491,#236492,#236493,#236494,
#236495,#236496,#236497,#236498,#236499,#236500,#236501,#236502,#236503,
#236504,#236505,#236506,#236507,#236508,#236509,#236510,#236511,#236512,
#236513,#236514,#236515,#236516,#236517,#236518,#236519,#236520,#236521,
#236522,#236523,#236524,#236525,#236526,#236527,#236528,#236529,#236530,
#236531,#236532,#236533,#236534,#236535,#236536,#236537,#236538,#236539,
#236540,#236541,#236542,#236543,#236544,#236545,#236546,#236547,#236548,
#236549,#236550,#236551,#236552,#236553,#236554,#236555,#236556,#236557,
#236558,#236559,#236560,#236561,#236562,#236563,#236564,#236565,#236566,
#236567,#236568,#236569,#236570,#236571,#236572,#236573,#236574,#236575,
#236576,#236577,#236578,#236579,#236580,#236581,#236582,#236583,#236584,
#236585,#236586,#236587,#236588,#236589,#236590,#236591,#236592,#236593,
#236594,#236595,#236596,#236597,#236598,#236599,#236600,#236601,#236602,
#236603,#236604,#236605,#236606,#236607,#236608,#236609,#236610,#236611,
#236612,#236613,#236614,#236615,#236616,#236617,#236618,#236619,#236620,
#236621,#236622,#236623,#236624,#236625,#236626,#236627,#236628,#236629,
#236630,#236631,#236632,#236633,#236634,#236635,#236636,#236637,#236638,
#236639,#236640,#236641,#236642,#236643,#236644,#236645,#236646,#236647,
#236648,#236649,#236650,#236651,#236652,#236653,#236654,#236655,#236656,
#236657,#236658,#236659,#236660,#236661,#236662,#236663,#236664,#236665,
#236666,#236667,#236668,#236669,#236670,#236671,#236672,#236673,#236674,
#236675,#236676,#236677,#236678,#236679,#236680,#236681,#236682,#236683,
#236684,#236685,#236686,#236687,#236688,#236689,#236690,#236691,#236692,
#236693,#236694,#236695,#236696,#236697,#236698,#236699,#236700,#236701,
#236702,#236703,#236704,#236705,#236706,#236707,#236708,#236709,#236710,
#236711,#236712,#236713,#236714,#236715,#236716,#236717,#236718,#236719,
#236720,#236721,#236722,#236723,#236724,#236725,#236726,#236727,#236728,
#236729,#236730,#236731,#236732,#236733,#236734,#236735,#236736,#236737,
#236738,#236739,#236740,#236741,#236742,#236743,#236744,#236745,#236746,
#236747,#236748,#236749,#236750,#236751,#236752,#236753,#236754,#236755,
#236756,#236757,#236758,#236759,#236760,#236761,#236762,#236763,#236764,
#236765,#236766,#236767,#236768,#236769,#236770,#236771,#236772,#236773,
#236774,#236775,#236776,#236777,#236778,#236779,#236780,#236781,#236782,
#236783,#236784,#236785,#236786,#236787,#236788,#236789,#236790,#236791,
#236792,#236793,#236794,#236795,#236796,#236797,#236798,#236799,#236800,
#236801,#236802,#236803,#236804,#236805,#236806,#236807,#236808,#236809,
#236810,#236811,#236812,#236813,#236814,#236815,#236816,#236817,#236818,
#236819,#236820,#236821,#236822,#236823,#236824,#236825,#236826,#236827,
#236828,#236829,#236830,#236831,#236832,#236833,#236834,#236835,#236836,
#236837,#236838,#236839,#236840,#236841,#236842,#236843,#236844,#236845,
#236846,#236847,#236848,#236849,#236850,#236851,#236852,#236853,#236854,
#236855,#236856,#236857,#236858,#236859,#236860,#236861,#236862,#236863,
#236864,#236865,#236866,#236867,#236868,#236869,#236870,#236871,#236872,
#236873,#236874,#236875,#236876,#236877,#236878,#236879,#236880,#236881,
#236882,#236883,#236884,#236885,#236886,#236887,#236888,#236889,#236890,
#236891,#236892),(#236893,#236894,#236895,#236896,#236897,#236898,#236899,
#236900,#236901,#236902,#236903,#236904,#236905,#236906,#236907,#236908,
#236909,#236910,#236911,#236912,#236913,#236914,#236915,#236916,#236917,
#236918,#236919,#236920,#236921,#236922,#236923,#236924,#236925,#236926,
#236927,#236928,#236929,#236930,#236931,#236932,#236933,#236934,#236935,
#236936,#236937,#236938,#236939,#236940,#236941,#236942,#236943,#236944,
#236945,#236946,#236947,#236948,#236949,#236950,#236951,#236952,#236953,
#236954,#236955,#236956,#236957,#236958,#236959,#236960,#236961,#236962,
#236963,#236964,#236965,#236966,#236967,#236968,#236969,#236970,#236971,
#236972,#236973,#236974,#236975,#236976,#236977,#236978,#236979,#236980,
#236981,#236982,#236983,#236984,#236985,#236986,#236987,#236988,#236989,
#236990,#236991,#236992,#236993,#236994,#236995,#236996,#236997,#236998,
#236999,#237000,#237001,#237002,#237003,#237004,#237005,#237006,#237007,
#237008,#237009,#237010,#237011,#237012,#237013,#237014,#237015,#237016,
#237017,#237018,#237019,#237020,#237021,#237022,#237023,#237024,#237025,
#237026,#237027,#237028,#237029,#237030,#237031,#237032,#237033,#237034,
#237035,#237036,#237037,#237038,#237039,#237040,#237041,#237042,#237043,
#237044,#237045,#237046,#237047,#237048,#237049,#237050,#237051,#237052,
#237053,#237054,#237055,#237056,#237057,#237058,#237059,#237060,#237061,
#237062,#237063,#237064,#237065,#237066,#237067,#237068,#237069,#237070,
#237071,#237072,#237073,#237074,#237075,#237076,#237077,#237078,#237079,
#237080,#237081,#237082,#237083,#237084,#237085,#237086,#237087,#237088,
#237089,#237090,#237091,#237092,#237093,#237094,#237095,#237096,#237097,
#237098,#237099,#237100,#237101,#237102,#237103,#237104,#237105,#237106,
#237107,#237108,#237109,#237110,#237111,#237112,#237113,#237114,#237115,
#237116,#237117,#237118,#237119,#237120,#237121,#237122,#237123,#237124,
#237125,#237126,#237127,#237128,#237129,#237130,#237131,#237132,#237133,
#237134,#237135,#237136,#237137,#237138,#237139,#237140,#237141,#237142,
#237143,#237144,#237145,#237146,#237147,#237148,#237149,#237150,#237151,
#237152,#237153,#237154,#237155,#237156,#237157,#237158,#237159,#237160,
#237161,#237162,#237163,#237164,#237165,#237166,#237167,#237168,#237169,
#237170,#237171,#237172,#237173,#237174,#237175,#237176,#237177,#237178,
#237179,#237180,#237181,#237182,#237183,#237184,#237185,#237186,#237187,
#237188,#237189,#237190,#237191,#237192,#237193,#237194,#237195,#237196,
#237197,#237198,#237199,#237200,#237201,#237202,#237203,#237204,#237205,
#237206,#237207,#237208,#237209,#237210,#237211,#237212,#237213,#237214,
#237215,#237216,#237217,#237218,#237219,#237220,#237221,#237222,#237223,
#237224,#237225,#237226,#237227,#237228,#237229,#237230,#237231,#237232,
#237233,#237234,#237235,#237236,#237237,#237238,#237239,#237240,#237241,
#237242,#237243,#237244,#237245,#237246,#237247,#237248,#237249,#237250,
#237251,#237252,#237253,#237254,#237255,#237256,#237257,#237258,#237259,
#237260,#237261,#237262,#237263,#237264,#237265,#237266,#237267,#237268,
#237269,#237270,#237271,#237272,#237273,#237274,#237275,#237276,#237277,
#237278,#237279,#237280,#237281,#237282,#237283,#237284,#237285,#237286,
#237287,#237288,#237289,#237290,#237291,#237292,#237293,#237294,#237295,
#237296,#237297,#237298,#237299,#237300,#237301,#237302,#237303,#237304,
#237305,#237306,#237307,#237308,#237309,#237310,#237311,#237312,#237313,
#237314,#237315,#237316,#237317,#237318,#237319,#237320,#237321,#237322,
#237323,#237324,#237325,#237326,#237327,#237328,#237329,#237330,#237331,
#237332,#237333,#237334,#237335,#237336,#237337,#237338,#237339,#237340,
#237341,#237342,#237343,#237344,#237345,#237346,#237347,#237348,#237349,
#237350,#237351,#237352,#237353,#237354,#237355,#237356,#237357,#237358,
#237359,#237360,#237361,#237362,#237363,#237364,#237365,#237366,#237367,
#237368,#237369,#237370,#237371,#237372,#237373,#237374,#237375,#237376,
#237377,#237378,#237379,#237380,#237381,#237382,#237383,#237384,#237385,
#237386,#237387,#237388,#237389,#237390,#237391,#237392,#237393,#237394,
#237395,#237396,#237397,#237398,#237399,#237400,#237401,#237402,#237403,
#237404,#237405,#237406,#237407,#237408,#237409,#237410,#237411,#237412,
#237413,#237414,#237415,#237416,#237417,#237418,#237419,#237420,#237421,
#237422,#237423,#237424,#237425,#237426,#237427,#237428,#237429,#237430,
#237431,#237432,#237433,#237434,#237435,#237436,#237437,#237438,#237439,
#237440,#237441,#237442,#237443,#237444,#237445,#237446,#237447,#237448,
#237449,#237450,#237451,#237452,#237453,#237454,#237455,#237456,#237457,
#237458,#237459,#237460,#237461,#237462,#237463,#237464,#237465,#237466,
#237467,#237468,#237469,#237470,#237471,#237472,#237473,#237474,#237475,
#237476,#237477,#237478,#237479,#237480,#237481,#237482,#237483,#237484,
#237485,#237486,#237487,#237488,#237489,#237490,#237491,#237492,#237493,
#237494,#237495,#237496,#237497,#237498,#237499,#237500,#237501,#237502,
#237503,#237504,#237505,#237506,#237507,#237508,#237509,#237510,#237511,
#237512,#237513,#237514,#237515,#237516,#237517,#237518,#237519,#237520,
#237521,#237522,#237523,#237524,#237525,#237526,#237527,#237528,#237529,
#237530,#237531,#237532,#237533,#237534,#237535,#237536,#237537,#237538,
#237539,#237540,#237541,#237542,#237543,#237544,#237545,#237546,#237547,
#237548,#237549,#237550,#237551,#237552,#237553,#237554,#237555,#237556,
#237557,#237558,#237559,#237560,#237561,#237562,#237563,#237564,#237565,
#237566,#237567,#237568,#237569,#237570,#237571,#237572,#237573,#237574,
#237575,#237576,#237577,#237578,#237579,#237580,#237581,#237582,#237583,
#237584,#237585,#237586,#237587,#237588,#237589,#237590,#237591,#237592,
#237593,#237594,#237595,#237596,#237597,#237598,#237599,#237600,#237601,
#237602,#237603,#237604,#237605,#237606,#237607,#237608,#237609,#237610,
#237611,#237612,#237613,#237614,#237615,#237616,#237617,#237618,#237619,
#237620,#237621,#237622,#237623,#237624,#237625,#237626,#237627,#237628,
#237629,#237630,#237631,#237632,#237633,#237634,#237635,#237636,#237637,
#237638,#237639,#237640,#237641,#237642,#237643,#237644,#237645,#237646,
#237647,#237648,#237649,#237650,#237651,#237652,#237653,#237654,#237655,
#237656,#237657,#237658,#237659,#237660,#237661,#237662,#237663,#237664,
#237665,#237666,#237667,#237668,#237669,#237670,#237671,#237672,#237673,
#237674,#237675,#237676,#237677,#237678,#237679,#237680,#237681,#237682,
#237683,#237684,#237685,#237686,#237687,#237688,#237689,#237690,#237691,
#237692,#237693,#237694,#237695,#237696,#237697,#237698,#237699,#237700,
#237701,#237702,#237703,#237704,#237705,#237706,#237707,#237708,#237709,
#237710,#237711,#237712,#237713,#237714,#237715,#237716,#237717,#237718,
#237719,#237720,#237721,#237722,#237723,#237724,#237725,#237726,#237727,
#237728,#237729,#237730,#237731,#237732,#237733,#237734,#237735,#237736,
#237737,#237738,#237739,#237740,#237741,#237742,#237743,#237744,#237745,
#237746,#237747,#237748,#237749,#237750,#237751,#237752,#237753,#237754,
#237755,#237756,#237757,#237758,#237759,#237760,#237761,#237762,#237763,
#237764,#237765,#237766,#237767,#237768,#237769,#237770,#237771,#237772,
#237773,#237774,#237775,#237776,#237777,#237778,#237779,#237780,#237781,
#237782,#237783,#237784,#237785,#237786,#237787,#237788,#237789,#237790,
#237791,#237792,#237793,#237794,#237795,#237796,#237797,#237798,#237799,
#237800,#237801,#237802,#237803,#237804,#237805,#237806,#237807,#237808,
#237809,#237810,#237811,#237812,#237813,#237814,#237815,#237816,#237817,
#237818,#237819,#237820,#237821,#237822,#237823,#237824,#237825,#237826,
#237827,#237828,#237829,#237830,#237831,#237832,#237833,#237834,#237835,
#237836,#237837,#237838,#237839,#237840,#237841,#237842,#237843,#237844,
#237845,#237846,#237847,#237848,#237849,#237850,#237851,#237852,#237853,
#237854,#237855,#237856,#237857,#237858,#237859,#237860,#237861,#237862,
#237863,#237864,#237865,#237866,#237867,#237868,#237869,#237870,#237871,
#237872,#237873,#237874,#237875,#237876,#237877,#237878,#237879,#237880,
#237881,#237882,#237883,#237884,#237885,#237886,#237887,#237888,#237889,
#237890,#237891,#237892,#237893,#237894,#237895,#237896,#237897,#237898,
#237899,#237900,#237901,#237902,#237903,#237904,#237905,#237906,#237907,
#237908,#237909,#237910,#237911,#237912,#237913,#237914,#237915,#237916,
#237917,#237918,#237919,#237920,#237921,#237922,#237923,#237924,#237925,
#237926,#237927,#237928,#237929,#237930,#237931,#237932,#237933,#237934,
#237935,#237936,#237937,#237938,#237939,#237940,#237941,#237942,#237943,
#237944,#237945,#237946,#237947,#237948,#237949,#237950,#237951,#237952,
#237953,#237954,#237955,#237956,#237957,#237958,#237959,#237960,#237961,
#237962,#237963,#237964,#237965,#237966,#237967,#237968,#237969,#237970,
#237971,#237972,#237973,#237974,#237975,#237976,#237977,#237978,#237979,
#237980,#237981,#237982,#237983,#237984,#237985,#237986,#237987,#237988,
#237989,#237990,#237991,#237992,#237993,#237994,#237995,#237996,#237997,
#237998,#237999,#238000,#238001,#238002,#238003,#238004,#238005,#238006,
#238007,#238008,#238009,#238010,#238011,#238012,#238013,#238014,#238015,
#238016,#238017,#238018,#238019,#238020,#238021,#238022,#238023,#238024,
#238025,#238026,#238027,#238028,#238029,#238030,#238031,#238032,#238033,
#238034,#238035,#238036,#238037,#238038,#238039,#238040,#238041,#238042,
#238043,#238044,#238045,#238046,#238047,#238048,#238049,#238050,#238051,
#238052,#238053,#238054,#238055,#238056,#238057,#238058,#238059,#238060,
#238061,#238062,#238063,#238064,#238065,#238066,#238067,#238068,#238069,
#238070,#238071,#238072,#238073,#238074,#238075,#238076,#238077,#238078,
#238079,#238080,#238081,#238082,#238083,#238084,#238085,#238086,#238087,
#238088,#238089,#238090,#238091,#238092,#238093,#238094,#238095,#238096,
#238097,#238098,#238099,#238100,#238101,#238102,#238103,#238104,#238105,
#238106,#238107,#238108,#238109,#238110,#238111,#238112,#238113,#238114,
#238115,#238116,#238117,#238118,#238119,#238120,#238121,#238122,#238123,
#238124,#238125,#238126,#238127,#238128,#238129,#238130,#238131,#238132,
#238133,#238134,#238135,#238136,#238137,#238138,#238139,#238140,#238141,
#238142,#238143,#238144,#238145,#238146,#238147,#238148,#238149,#238150,
#238151,#238152,#238153,#238154,#238155,#238156,#238157,#238158,#238159,
#238160,#238161,#238162,#238163,#238164,#238165,#238166,#238167,#238168,
#238169,#238170,#238171,#238172,#238173,#238174,#238175,#238176,#238177,
#238178,#238179,#238180,#238181,#238182,#238183,#238184,#238185,#238186,
#238187,#238188,#238189,#238190,#238191,#238192,#238193,#238194,#238195,
#238196,#238197,#238198,#238199,#238200,#238201,#238202,#238203,#238204,
#238205,#238206,#238207,#238208,#238209,#238210,#238211,#238212,#238213,
#238214,#238215,#238216,#238217,#238218,#238219,#238220,#238221,#238222,
#238223,#238224,#238225,#238226,#238227,#238228,#238229,#238230,#238231,
#238232,#238233,#238234,#238235,#238236,#238237,#238238,#238239,#238240,
#238241,#238242,#238243,#238244,#238245,#238246,#238247,#238248,#238249,
#238250,#238251,#238252,#238253,#238254,#238255,#238256,#238257,#238258,
#238259,#238260,#238261,#238262,#238263,#238264,#238265,#238266,#238267,
#238268,#238269,#238270,#238271,#238272,#238273,#238274,#238275,#238276,
#238277,#238278,#238279,#238280,#238281,#238282,#238283,#238284,#238285,
#238286,#238287,#238288,#238289,#238290,#238291,#238292,#238293,#238294,
#238295,#238296,#238297,#238298,#238299,#238300,#238301,#238302,#238303,
#238304,#238305,#238306,#238307,#238308,#238309,#238310,#238311,#238312,
#238313,#238314,#238315,#238316,#238317,#238318,#238319,#238320,#238321,
#238322,#238323,#238324,#238325,#238326,#238327,#238328,#238329,#238330,
#238331,#238332,#238333,#238334,#238335,#238336,#238337,#238338,#238339,
#238340,#238341,#238342,#238343,#238344,#238345,#238346,#238347,#238348,
#238349,#238350,#238351,#238352,#238353,#238354,#238355,#238356,#238357,
#238358,#238359,#238360,#238361,#238362,#238363,#238364,#238365,#238366,
#238367,#238368,#238369,#238370,#238371,#238372,#238373,#238374,#238375,
#238376,#238377,#238378,#238379,#238380,#238381,#238382,#238383,#238384,
#238385,#238386,#238387,#238388,#238389,#238390,#238391,#238392,#238393,
#238394,#238395,#238396,#238397,#238398,#238399,#238400,#238401,#238402,
#238403,#238404,#238405,#238406,#238407,#238408,#238409,#238410,#238411,
#238412,#238413,#238414,#238415,#238416,#238417,#238418,#238419,#238420,
#238421,#238422,#238423,#238424,#238425,#238426,#238427,#238428,#238429,
#238430,#238431,#238432,#238433,#238434,#238435,#238436,#238437,#238438,
#238439,#238440,#238441,#238442,#238443,#238444,#238445,#238446,#238447,
#238448,#238449,#238450,#238451,#238452,#238453,#238454,#238455,#238456,
#238457,#238458,#238459,#238460,#238461,#238462,#238463,#238464,#238465,
#238466,#238467,#238468,#238469,#238470,#238471,#238472,#238473,#238474,
#238475,#238476,#238477,#238478,#238479,#238480,#238481,#238482,#238483,
#238484,#238485,#238486,#238487,#238488,#238489,#238490,#238491,#238492,
#238493,#238494,#238495,#238496,#238497,#238498,#238499,#238500,#238501,
#238502,#238503,#238504,#238505,#238506,#238507,#238508,#238509,#238510,
#238511,#238512,#238513,#238514,#238515,#238516,#238517,#238518,#238519,
#238520,#238521,#238522,#238523,#238524,#238525,#238526,#238527,#238528,
#238529,#238530,#238531,#238532,#238533,#238534,#238535,#238536,#238537,
#238538,#238539,#238540,#238541,#238542,#238543,#238544,#238545,#238546,
#238547,#238548,#238549,#238550,#238551,#238552,#238553,#238554,#238555,
#238556,#238557,#238558,#238559,#238560,#238561,#238562,#238563,#238564,
#238565,#238566,#238567,#238568,#238569,#238570,#238571,#238572,#238573,
#238574,#238575,#238576,#238577,#238578,#238579,#238580,#238581,#238582,
#238583,#238584,#238585,#238586,#238587),(#238588,#238589,#238590,#238591,
#238592,#238593,#238594,#238595,#238596,#238597,#238598,#238599,#238600,
#238601,#238602,#238603,#238604,#238605,#238606,#238607,#238608,#238609,
#238610,#238611,#238612,#238613,#238614,#238615,#238616,#238617,#238618,
#238619,#238620,#238621,#238622,#238623,#238624,#238625,#238626,#238627,
#238628,#238629,#238630,#238631,#238632,#238633,#238634,#238635,#238636,
#238637,#238638,#238639,#238640,#238641,#238642,#238643,#238644,#238645,
#238646,#238647,#238648,#238649,#238650,#238651,#238652,#238653,#238654,
#238655,#238656,#238657,#238658,#238659,#238660,#238661,#238662,#238663,
#238664,#238665,#238666,#238667,#238668,#238669,#238670,#238671,#238672,
#238673,#238674,#238675,#238676,#238677,#238678,#238679,#238680,#238681,
#238682,#238683,#238684,#238685,#238686,#238687,#238688,#238689,#238690,
#238691,#238692,#238693,#238694,#238695,#238696,#238697,#238698,#238699,
#238700,#238701,#238702,#238703,#238704,#238705,#238706,#238707,#238708,
#238709,#238710,#238711,#238712,#238713,#238714,#238715,#238716,#238717,
#238718,#238719,#238720,#238721,#238722,#238723,#238724,#238725,#238726,
#238727,#238728,#238729,#238730,#238731,#238732,#238733,#238734,#238735,
#238736,#238737,#238738,#238739,#238740,#238741,#238742,#238743,#238744,
#238745,#238746,#238747,#238748,#238749,#238750,#238751,#238752,#238753,
#238754,#238755,#238756,#238757,#238758,#238759,#238760,#238761,#238762,
#238763,#238764,#238765,#238766,#238767,#238768,#238769,#238770,#238771,
#238772,#238773,#238774,#238775,#238776,#238777,#238778,#238779,#238780,
#238781,#238782,#238783,#238784,#238785,#238786,#238787,#238788,#238789,
#238790,#238791,#238792,#238793,#238794,#238795,#238796,#238797,#238798,
#238799,#238800,#238801,#238802,#238803,#238804,#238805,#238806,#238807,
#238808,#238809,#238810,#238811,#238812,#238813,#238814,#238815,#238816,
#238817,#238818,#238819,#238820,#238821,#238822,#238823,#238824,#238825,
#238826,#238827,#238828,#238829,#238830,#238831,#238832,#238833,#238834,
#238835,#238836,#238837,#238838,#238839,#238840,#238841,#238842,#238843,
#238844,#238845,#238846,#238847,#238848,#238849,#238850,#238851,#238852,
#238853,#238854,#238855,#238856,#238857,#238858,#238859,#238860,#238861,
#238862,#238863,#238864,#238865,#238866,#238867,#238868,#238869,#238870,
#238871,#238872,#238873,#238874,#238875,#238876,#238877,#238878,#238879,
#238880,#238881,#238882,#238883,#238884,#238885,#238886,#238887,#238888,
#238889,#238890,#238891,#238892,#238893,#238894,#238895,#238896,#238897,
#238898,#238899,#238900,#238901,#238902,#238903,#238904,#238905,#238906,
#238907,#238908,#238909,#238910,#238911,#238912,#238913,#238914,#238915,
#238916,#238917,#238918,#238919,#238920,#238921,#238922,#238923,#238924,
#238925,#238926,#238927,#238928,#238929,#238930,#238931,#238932,#238933,
#238934,#238935,#238936,#238937,#238938,#238939,#238940,#238941,#238942,
#238943,#238944,#238945,#238946,#238947,#238948,#238949,#238950,#238951,
#238952,#238953,#238954,#238955,#238956,#238957,#238958,#238959,#238960,
#238961,#238962,#238963,#238964,#238965,#238966,#238967,#238968,#238969,
#238970,#238971,#238972,#238973,#238974,#238975,#238976,#238977,#238978,
#238979,#238980,#238981,#238982,#238983,#238984,#238985,#238986,#238987,
#238988,#238989,#238990,#238991,#238992,#238993,#238994,#238995,#238996,
#238997,#238998,#238999,#239000,#239001,#239002,#239003,#239004,#239005,
#239006,#239007,#239008,#239009,#239010,#239011,#239012,#239013,#239014,
#239015,#239016,#239017,#239018,#239019,#239020,#239021,#239022,#239023,
#239024,#239025,#239026,#239027,#239028,#239029,#239030,#239031,#239032,
#239033,#239034,#239035,#239036,#239037,#239038,#239039,#239040,#239041,
#239042,#239043,#239044,#239045,#239046,#239047,#239048,#239049,#239050,
#239051,#239052,#239053,#239054,#239055,#239056,#239057,#239058,#239059,
#239060,#239061,#239062,#239063,#239064,#239065,#239066,#239067,#239068,
#239069,#239070,#239071,#239072,#239073,#239074,#239075,#239076,#239077,
#239078,#239079,#239080,#239081,#239082,#239083,#239084,#239085,#239086,
#239087,#239088,#239089,#239090,#239091,#239092,#239093,#239094,#239095,
#239096,#239097,#239098,#239099,#239100,#239101,#239102,#239103,#239104,
#239105,#239106,#239107,#239108,#239109,#239110,#239111,#239112,#239113,
#239114,#239115,#239116,#239117,#239118,#239119,#239120,#239121,#239122,
#239123,#239124,#239125,#239126,#239127,#239128,#239129,#239130,#239131,
#239132,#239133,#239134,#239135,#239136,#239137,#239138,#239139,#239140,
#239141,#239142,#239143,#239144,#239145,#239146,#239147,#239148,#239149,
#239150,#239151,#239152,#239153,#239154,#239155,#239156,#239157,#239158,
#239159,#239160,#239161,#239162,#239163,#239164,#239165,#239166,#239167,
#239168,#239169,#239170,#239171,#239172,#239173,#239174,#239175,#239176,
#239177,#239178,#239179,#239180,#239181,#239182,#239183,#239184,#239185,
#239186,#239187,#239188,#239189,#239190,#239191,#239192,#239193,#239194,
#239195,#239196,#239197,#239198,#239199,#239200,#239201,#239202,#239203,
#239204,#239205,#239206,#239207,#239208,#239209,#239210,#239211,#239212,
#239213,#239214,#239215,#239216,#239217,#239218,#239219,#239220,#239221,
#239222,#239223,#239224,#239225,#239226,#239227,#239228,#239229,#239230,
#239231,#239232,#239233,#239234,#239235,#239236,#239237,#239238,#239239,
#239240,#239241,#239242,#239243,#239244,#239245,#239246,#239247,#239248,
#239249,#239250,#239251,#239252,#239253,#239254,#239255,#239256,#239257,
#239258,#239259,#239260,#239261,#239262,#239263,#239264,#239265,#239266,
#239267,#239268,#239269,#239270,#239271,#239272,#239273,#239274,#239275,
#239276,#239277,#239278,#239279,#239280,#239281,#239282,#239283,#239284,
#239285,#239286,#239287,#239288,#239289,#239290,#239291,#239292,#239293,
#239294,#239295,#239296,#239297,#239298,#239299,#239300,#239301,#239302,
#239303,#239304,#239305,#239306,#239307,#239308,#239309,#239310,#239311,
#239312,#239313,#239314,#239315,#239316,#239317,#239318,#239319,#239320,
#239321,#239322,#239323,#239324,#239325,#239326,#239327,#239328,#239329,
#239330,#239331,#239332,#239333,#239334,#239335,#239336,#239337,#239338,
#239339,#239340,#239341,#239342,#239343,#239344,#239345,#239346,#239347,
#239348,#239349,#239350,#239351,#239352,#239353,#239354,#239355,#239356,
#239357,#239358,#239359,#239360,#239361,#239362,#239363,#239364,#239365,
#239366,#239367,#239368,#239369,#239370,#239371,#239372,#239373,#239374,
#239375,#239376,#239377,#239378,#239379,#239380,#239381,#239382,#239383,
#239384,#239385,#239386,#239387,#239388,#239389,#239390,#239391,#239392,
#239393,#239394,#239395,#239396,#239397,#239398,#239399,#239400,#239401,
#239402,#239403,#239404,#239405,#239406,#239407,#239408,#239409,#239410,
#239411,#239412,#239413,#239414,#239415,#239416,#239417,#239418,#239419,
#239420,#239421,#239422,#239423,#239424,#239425,#239426,#239427,#239428,
#239429,#239430,#239431,#239432,#239433,#239434,#239435,#239436,#239437,
#239438,#239439,#239440,#239441,#239442,#239443,#239444,#239445,#239446,
#239447,#239448,#239449,#239450,#239451,#239452,#239453,#239454,#239455,
#239456,#239457,#239458,#239459,#239460,#239461,#239462,#239463,#239464,
#239465,#239466,#239467,#239468,#239469,#239470,#239471,#239472,#239473,
#239474,#239475,#239476,#239477,#239478,#239479,#239480,#239481,#239482,
#239483,#239484,#239485,#239486,#239487,#239488,#239489,#239490,#239491,
#239492,#239493,#239494,#239495,#239496,#239497,#239498,#239499,#239500,
#239501,#239502,#239503,#239504,#239505,#239506,#239507,#239508,#239509,
#239510,#239511,#239512,#239513,#239514,#239515,#239516,#239517,#239518,
#239519,#239520,#239521,#239522,#239523,#239524,#239525,#239526,#239527,
#239528,#239529,#239530,#239531,#239532,#239533,#239534,#239535,#239536,
#239537,#239538,#239539,#239540,#239541,#239542,#239543,#239544,#239545,
#239546,#239547,#239548,#239549,#239550,#239551,#239552,#239553,#239554,
#239555,#239556,#239557,#239558,#239559,#239560,#239561,#239562,#239563,
#239564,#239565,#239566,#239567,#239568,#239569,#239570,#239571,#239572,
#239573,#239574,#239575,#239576,#239577,#239578,#239579,#239580,#239581,
#239582,#239583,#239584,#239585,#239586,#239587,#239588,#239589,#239590,
#239591,#239592,#239593,#239594,#239595,#239596,#239597,#239598,#239599,
#239600,#239601,#239602,#239603,#239604,#239605,#239606,#239607,#239608,
#239609,#239610,#239611,#239612,#239613,#239614,#239615,#239616,#239617,
#239618,#239619,#239620,#239621,#239622,#239623,#239624,#239625,#239626,
#239627,#239628,#239629,#239630,#239631,#239632,#239633,#239634,#239635,
#239636,#239637,#239638,#239639,#239640,#239641,#239642,#239643,#239644,
#239645,#239646,#239647,#239648,#239649,#239650,#239651,#239652,#239653,
#239654,#239655,#239656,#239657,#239658,#239659,#239660,#239661,#239662,
#239663,#239664,#239665,#239666,#239667,#239668,#239669,#239670,#239671,
#239672,#239673,#239674,#239675,#239676,#239677,#239678,#239679,#239680,
#239681,#239682,#239683,#239684,#239685,#239686,#239687,#239688,#239689,
#239690,#239691,#239692,#239693,#239694,#239695,#239696,#239697,#239698,
#239699,#239700,#239701,#239702,#239703,#239704,#239705,#239706,#239707,
#239708,#239709,#239710,#239711,#239712,#239713,#239714,#239715,#239716,
#239717,#239718,#239719,#239720,#239721,#239722,#239723,#239724,#239725,
#239726,#239727,#239728,#239729,#239730,#239731,#239732,#239733,#239734,
#239735,#239736,#239737,#239738,#239739,#239740,#239741,#239742,#239743,
#239744,#239745,#239746,#239747,#239748,#239749,#239750,#239751,#239752,
#239753,#239754,#239755,#239756,#239757,#239758,#239759,#239760,#239761,
#239762,#239763,#239764,#239765,#239766,#239767,#239768,#239769,#239770,
#239771,#239772,#239773,#239774,#239775,#239776,#239777,#239778,#239779,
#239780,#239781,#239782,#239783,#239784,#239785,#239786,#239787,#239788,
#239789,#239790,#239791,#239792,#239793,#239794,#239795,#239796,#239797,
#239798,#239799,#239800,#239801,#239802,#239803,#239804,#239805,#239806,
#239807,#239808,#239809,#239810,#239811,#239812,#239813,#239814,#239815,
#239816,#239817,#239818,#239819,#239820,#239821,#239822,#239823,#239824,
#239825,#239826,#239827,#239828,#239829,#239830,#239831,#239832,#239833,
#239834,#239835,#239836,#239837,#239838,#239839,#239840,#239841,#239842,
#239843,#239844,#239845,#239846,#239847,#239848,#239849,#239850,#239851,
#239852,#239853,#239854,#239855,#239856,#239857,#239858,#239859,#239860,
#239861,#239862,#239863,#239864,#239865,#239866,#239867,#239868,#239869,
#239870,#239871,#239872,#239873,#239874,#239875,#239876,#239877,#239878,
#239879,#239880,#239881,#239882,#239883,#239884,#239885,#239886,#239887,
#239888,#239889,#239890,#239891,#239892,#239893,#239894,#239895,#239896,
#239897,#239898,#239899,#239900,#239901,#239902,#239903,#239904,#239905,
#239906,#239907,#239908,#239909,#239910,#239911,#239912,#239913,#239914,
#239915,#239916,#239917,#239918,#239919,#239920,#239921,#239922,#239923,
#239924,#239925,#239926,#239927,#239928,#239929,#239930,#239931,#239932,
#239933,#239934,#239935,#239936,#239937,#239938,#239939,#239940,#239941,
#239942,#239943,#239944,#239945,#239946,#239947,#239948,#239949,#239950,
#239951,#239952,#239953,#239954,#239955,#239956,#239957,#239958,#239959,
#239960,#239961,#239962,#239963,#239964,#239965,#239966,#239967,#239968,
#239969,#239970,#239971,#239972,#239973,#239974,#239975,#239976,#239977,
#239978,#239979,#239980,#239981,#239982,#239983,#239984,#239985,#239986,
#239987,#239988,#239989,#239990,#239991,#239992,#239993,#239994,#239995,
#239996,#239997,#239998,#239999,#240000,#240001,#240002,#240003,#240004,
#240005,#240006,#240007,#240008,#240009,#240010,#240011,#240012,#240013,
#240014,#240015,#240016,#240017,#240018,#240019,#240020,#240021,#240022,
#240023,#240024,#240025,#240026,#240027,#240028,#240029,#240030,#240031,
#240032,#240033,#240034,#240035,#240036,#240037,#240038,#240039,#240040,
#240041,#240042,#240043,#240044,#240045,#240046,#240047,#240048,#240049,
#240050,#240051,#240052,#240053,#240054,#240055,#240056,#240057,#240058,
#240059,#240060,#240061,#240062,#240063,#240064,#240065,#240066,#240067,
#240068,#240069,#240070,#240071,#240072,#240073,#240074,#240075,#240076,
#240077,#240078,#240079,#240080,#240081,#240082,#240083,#240084,#240085,
#240086,#240087,#240088,#240089,#240090,#240091,#240092,#240093,#240094,
#240095,#240096,#240097,#240098,#240099,#240100,#240101,#240102,#240103,
#240104,#240105,#240106,#240107,#240108,#240109,#240110,#240111,#240112,
#240113,#240114,#240115,#240116,#240117,#240118,#240119,#240120,#240121,
#240122,#240123,#240124,#240125,#240126,#240127,#240128,#240129,#240130,
#240131,#240132,#240133,#240134,#240135,#240136,#240137,#240138,#240139,
#240140,#240141,#240142,#240143,#240144,#240145,#240146,#240147,#240148,
#240149,#240150,#240151,#240152,#240153,#240154,#240155,#240156,#240157,
#240158,#240159,#240160,#240161,#240162,#240163,#240164,#240165,#240166,
#240167,#240168,#240169,#240170,#240171,#240172,#240173,#240174,#240175,
#240176,#240177,#240178,#240179,#240180,#240181,#240182,#240183,#240184,
#240185,#240186,#240187,#240188,#240189,#240190,#240191,#240192,#240193,
#240194,#240195,#240196,#240197,#240198,#240199,#240200,#240201,#240202,
#240203,#240204,#240205,#240206,#240207,#240208,#240209,#240210,#240211,
#240212,#240213,#240214,#240215,#240216,#240217,#240218,#240219,#240220,
#240221,#240222,#240223,#240224,#240225,#240226,#240227,#240228,#240229,
#240230,#240231,#240232,#240233,#240234,#240235,#240236,#240237,#240238,
#240239,#240240,#240241,#240242,#240243,#240244,#240245,#240246,#240247,
#240248,#240249,#240250,#240251,#240252,#240253,#240254,#240255,#240256,
#240257,#240258,#240259,#240260,#240261,#240262,#240263,#240264,#240265,
#240266,#240267,#240268,#240269,#240270,#240271,#240272,#240273,#240274,
#240275,#240276,#240277,#240278,#240279,#240280,#240281,#240282)),
 .UNSPECIFIED.,.F.,.F.,.F.,(4,4),(4,1,1,1,1,1,1,1,1,1,1,1,1,1,1,1,1,1,1,
1,1,1,1,1,1,1,1,1,1,1,1,1,1,1,1,1,1,1,1,1,1,1,1,1,1,1,1,1,1,1,1,1,1,1,1,
1,1,1,1,1,1,1,1,1,1,1,1,1,1,1,1,1,1,1,1,1,1,1,1,1,1,1,1,1,1,1,1,1,1,1,1,
1,1,1,1,1,1,1,1,1,1,1,1,1,1,1,1,1,1,1,1,1,1,1,1,1,1,1,1,1,1,1,1,1,1,1,1,
1,1,1,1,1,1,1,1,1,1,1,1,1,1,1,1,1,1,1,1,1,1,1,1,1,1,1,1,1,1,1,1,1,1,1,1,
1,1,1,1,1,1,1,1,1,1,1,1,1,1,1,1,1,1,1,1,1,1,1,1,1,1,1,1,1,1,1,1,1,1,1,1,
1,1,1,1,1,1,1,1,1,1,1,1,1,1,1,1,1,1,1,1,1,1,1,1,1,1,1,1,1,1,1,1,1,1,1,1,
1,1,1,1,1,1,1,1,1,1,1,1,1,1,1,1,1,1,1,1,1,1,1,1,1,1,1,1,1,1,1,1,1,1,1,1,
1,1,1,1,1,1,1,1,1,1,1,1,1,1,1,1,1,1,1,1,1,1,1,1,1,1,1,1,1,1,1,1,1,1,1,1,
1,1,1,1,1,1,1,1,1,1,1,1,1,1,1,1,1,1,1,1,1,1,1,1,1,1,1,1,1,1,1,1,1,1,1,1,
1,1,1,1,1,1,1,1,1,1,1,1,1,1,1,1,1,1,1,1,1,1,1,1,1,1,1,1,1,1,1,1,1,1,1,1,
1,1,1,1,1,1,1,1,1,1,1,1,1,1,1,1,1,1,1,1,1,1,1,1,1,1,1,1,1,1,1,1,1,1,1,1,
1,1,1,1,1,1,1,1,1,1,1,1,1,1,1,1,1,1,1,1,1,1,1,1,1,1,1,1,1,1,1,1,1,1,1,1,
1,1,1,1,1,1,1,1,1,1,1,1,1,1,1,1,1,1,1,1,1,1,1,1,1,1,1,1,1,1,1,1,1,1,1,1,
1,1,1,1,1,1,1,1,1,1,1,1,1,1,1,1,1,1,1,1,1,1,1,1,1,1,1,1,1,1,1,1,1,1,1,1,
1,1,1,1,1,1,1,1,1,1,1,1,1,1,1,1,1,1,1,1,1,1,1,1,1,1,1,1,1,1,1,1,1,1,1,1,
1,1,1,1,1,1,1,1,1,1,1,1,1,1,1,1,1,1,1,1,1,1,1,1,1,1,1,1,1,1,1,1,1,1,1,1,
1,1,1,1,1,1,1,1,1,1,1,1,1,1,1,1,1,1,1,1,1,1,1,1,1,1,1,1,1,1,1,1,1,1,1,1,
1,1,1,1,1,1,1,1,1,1,1,1,1,1,1,1,1,1,1,1,1,1,1,1,1,1,1,1,1,1,1,1,1,1,1,1,
1,1,1,1,1,1,1,1,1,1,1,1,1,1,1,1,1,1,1,1,1,1,1,1,1,1,1,1,1,1,1,1,1,1,1,1,
1,1,1,1,1,1,1,1,1,1,1,1,1,1,1,1,1,1,1,1,1,1,1,1,1,1,1,1,1,1,1,1,1,1,1,1,
1,1,1,1,1,1,1,1,1,1,1,1,1,1,1,1,1,1,1,1,1,1,1,1,1,1,1,1,1,1,1,1,1,1,1,1,
1,1,1,1,1,1,1,1,1,1,1,1,1,1,1,1,1,1,1,1,1,1,1,1,1,1,1,1,1,1,1,1,1,1,1,1,
1,1,1,1,1,1,1,1,1,1,1,1,1,1,1,1,1,1,1,1,1,1,1,1,1,1,1,1,1,1,1,1,1,1,1,1,
1,1,1,1,1,1,1,1,1,1,1,1,1,1,1,1,1,1,1,1,1,1,1,1,1,1,1,1,1,1,1,1,1,1,1,1,
1,1,1,1,1,1,1,1,1,1,1,1,1,1,1,1,1,1,1,1,1,1,1,1,1,1,1,1,1,1,1,1,1,1,1,1,
1,1,1,1,1,1,1,1,1,1,1,1,1,1,1,1,1,1,1,1,1,1,1,1,1,1,1,1,1,1,1,1,1,1,1,1,
1,1,1,1,1,1,1,1,1,1,1,1,1,1,1,1,1,1,1,1,1,1,1,1,1,1,1,1,1,1,1,1,1,1,1,1,
1,1,1,1,1,1,1,1,1,1,1,1,1,1,1,1,1,1,1,1,1,1,1,1,1,1,1,1,1,1,1,1,1,1,1,1,
1,1,1,1,1,1,1,1,1,1,1,1,1,1,1,1,1,1,1,1,1,1,1,1,1,1,1,1,1,1,1,1,1,1,1,1,
1,1,1,1,1,1,1,1,1,1,1,1,1,1,1,1,1,1,1,1,1,1,1,1,1,1,1,1,1,1,1,1,1,1,1,1,
1,1,1,1,1,1,1,1,1,1,1,1,1,1,1,1,1,1,1,1,1,1,1,1,1,1,1,1,1,1,1,1,1,1,1,1,
1,1,1,1,1,1,1,1,1,1,1,1,1,1,1,1,1,1,1,1,1,1,1,1,1,1,1,1,1,1,1,1,1,1,1,1,
1,1,1,1,1,1,1,1,1,1,1,1,1,1,1,1,1,1,1,1,1,1,1,1,1,1,1,1,1,1,1,1,1,1,1,1,
1,1,1,1,1,1,1,1,1,1,1,1,1,1,1,1,1,1,1,1,1,1,1,1,1,1,1,1,1,1,1,1,1,1,1,1,
1,1,1,1,1,1,1,1,1,1,1,1,1,1,1,1,1,1,1,1,1,1,1,1,1,1,1,1,1,1,1,1,1,1,1,1,
1,1,1,1,1,1,1,1,1,1,1,1,1,1,1,1,1,1,1,1,1,1,1,1,1,1,1,1,1,1,1,1,1,1,1,1,
1,1,1,1,1,1,1,1,1,1,1,1,1,1,1,1,1,1,1,1,1,1,1,1,1,1,1,1,1,1,1,1,1,1,1,1,
1,1,1,1,1,1,1,1,1,1,1,1,1,1,1,1,1,1,1,1,1,1,1,1,1,1,1,1,1,1,1,1,1,1,1,1,
1,1,1,1,1,1,1,1,1,1,1,1,1,1,1,1,1,1,1,1,1,1,1,1,1,1,1,1,1,1,1,1,1,1,1,1,
1,1,1,1,1,1,1,1,1,1,1,1,1,1,1,1,1,1,1,1,1,1,1,1,1,1,1,1,1,1,1,1,1,1,1,1,
1,1,1,1,1,1,1,1,1,1,1,1,1,1,1,1,1,1,1,1,1,1,1,1,1,1,1,1,1,1,1,1,1,1,1,1,
1,1,1,1,1,1,1,1,1,1,1,1,1,1,1,1,1,1,1,1,1,1,1,1,1,1,1,1,1,1,1,1,1,1,1,1,
1,1,1,1,1,1,1,1,1,1,1,1,1,1,1,1,1,1,1,1,1,1,1,1,1,1,1,1,1,1,1,1,1,1,1,1,
1,1,1,1,1,1,1,1,1,1,1,1,1,1,1,1,1,1,1,1,1,1,1,1,1,1,1,1,1,1,1,1,1,1,1,1,
1,1,1,1,1,1,1,1,1,1,1,1,1,1,1,1,1,1,1,1,1,1,1,1,1,1,1,1,1,1,1,1,1,1,1,1,
1,1,1,1,1,1,1,1,1,1,1,1,1,1,1,1,1,1,1,1,1,1,1,1,1,1,1,1,1,1,1,1,1,1,1,1,
1,1,1,1,1,1,1,1,1,1,1,1,1,1,1,1,1,4),(-0.000587328099657093,0.1157205948422),
(8.30590413559005,8.80579087257276,9.30565887793282,10.305394888653,11.3051308993731,
12.3048669100932,13.3046029208133,14.3043389315335,15.3040749422536,16.3038109529737,
17.3035469636939,18.303282974414,19.3030189851341,20.3027549958542,21.3024910065744,
22.3022270172945,23.3019630280146,24.3016990387348,25.3014350494549,26.301171060175,
27.3009070708951,28.3006430816153,29.3003790923354,30.3001151030555,31.2998511137757,
32.2995871244958,33.2993231352159,34.299059145936,35.2987951566562,36.2985311673763,
37.2982671780964,38.2980031888166,39.2977391995367,40.2974752102568,41.2972112209769,
42.2969472316971,43.2966832424172,44.2964192531373,45.2961552638575,46.2958912745776,
47.2956272852977,48.2953632960178,49.295099306738,50.2948353174581,51.2945713281782,
52.2943073388984,53.2940433496185,54.2937793603386,55.2935153710587,56.2932513817789,
57.292987392499,58.2927234032191,59.2924594139393,60.2921954246594,61.2919314353795,
62.2916674460996,63.2914034568198,64.2911394675399,65.29087547826,66.2906114889802,
67.2903474997003,68.2900835104204,69.2898195211405,70.2895555318607,71.2892915425808,
72.2890275533009,73.2887635640211,74.2884995747412,75.2882355854613,76.2879715961814,
77.2877076069016,78.2874436176217,79.2871796283418,80.286915639062,81.2866516497821,
82.2863876605022,83.2861236712224,84.2858596819425,85.2855956926626,86.2853317033827,
87.2850677141029,88.284803724823,89.2845397355431,90.2842757462633,91.2840117569834,
92.2837477677035,93.2834837784236,94.2832197891438,95.2829557998639,96.282691810584,
97.2824278213041,98.2821638320243,99.2818998427444,100.281635853465,101.281371864185,
102.281107874905,103.280843885625,104.280579896345,105.280315907065,106.280051917785,
107.279787928505,108.279523939226,109.279259949946,110.278995960666,111.278731971386,
112.278467982106,113.278203992826,114.277940003546,115.277676014266,116.277412024987,
117.277148035707,118.276884046427,119.276620057147,120.276356067867,121.276092078587,
122.275828089307,123.275564100028,124.275300110748,125.275036121468,126.274772132188,
127.274508142908,128.274244153628,129.273980164348,130.273716175068,131.273452185789,
132.273188196509,133.272924207229,134.272660217949,135.272396228669,136.272132239389,
137.271868250109,138.271604260829,139.27134027155,140.27107628227,141.27081229299,
142.27054830371,143.27028431443,144.27002032515,145.26975633587,146.26949234659,
147.269228357311,148.268964368031,149.268700378751,150.268436389471,151.268172400191,
152.267908410911,153.267644421631,154.267380432352,155.267116443072,156.266852453792,
157.266588464512,158.266324475232,159.266060485952,160.265796496672,161.265532507392,
162.265268518113,163.265004528833,164.264740539553,165.264476550273,166.264212560993,
167.263948571713,168.263684582433,169.263420593153,170.263156603874,171.262892614594,
172.262628625314,173.262364636034,174.262100646754,175.261836657474,176.261572668194,
177.261308678914,178.261044689635,179.260780700355,180.260516711075,181.260252721795,
182.259988732515,183.259724743235,184.259460753955,185.259196764675,186.258932775396,
187.258668786116,188.258404796836,189.258140807556,190.257876818276,191.257612828996,
192.257348839716,193.257084850437,194.256820861157,195.256556871877,196.256292882597,
197.256028893317,198.255764904037,199.255500914757,200.255236925477,201.254972936198,
202.254708946918,203.254444957638,204.254180968358,205.253916979078,206.253652989798,
207.253389000518,208.253125011238,209.252861021959,210.252597032679,211.252333043399,
212.252069054119,213.251805064839,214.251541075559,215.251277086279,216.251013096999,
217.25074910772,218.25048511844,219.25022112916,220.24995713988,221.2496931506,
222.24942916132,223.24916517204,224.248901182761,225.248637193481,226.248373204201,
227.248109214921,228.247845225641,229.247581236361,230.247317247081,231.247053257801,
232.246789268522,233.246525279242,234.246261289962,235.245997300682,236.245733311402,
237.245469322122,238.245205332842,239.244941343562,240.244677354283,241.244413365003,
242.244149375723,243.243885386443,244.243621397163,245.243357407883,246.243093418603,
247.242829429323,248.242565440044,249.242301450764,250.242037461484,251.241773472204,
252.241509482924,253.241245493644,254.240981504364,255.240717515084,256.240453525805,
257.240189536525,258.239925547245,259.239661557965,260.239397568685,261.239133579405,
262.238869590125,263.238605600846,264.238341611566,265.238077622286,266.237813633006,
267.237549643726,268.237285654446,269.237021665166,270.236757675886,271.236493686607,
272.236229697327,273.235965708047,274.235701718767,275.235437729487,276.235173740207,
277.234909750927,278.234645761647,279.234381772368,280.234117783088,281.233853793808,
282.233589804528,283.233325815248,284.233061825968,285.232797836688,286.232533847408,
287.232269858129,288.232005868849,289.231741879569,290.231477890289,291.231213901009,
292.230949911729,293.230685922449,294.23042193317,295.23015794389,296.22989395461,
297.22962996533,298.22936597605,299.22910198677,300.22883799749,301.22857400821,
302.228310018931,303.228046029651,304.227782040371,305.227518051091,306.227254061811,
307.226990072531,308.226726083251,309.226462093971,310.226198104692,311.225934115412,
312.225670126132,313.225406136852,314.225142147572,315.224878158292,316.224614169012,
317.224350179732,318.224086190453,319.223822201173,320.223558211893,321.223294222613,
322.223030233333,323.222766244053,324.222502254773,325.222238265494,326.221974276214,
327.221710286934,328.221446297654,329.221182308374,330.220918319094,331.220654329814,
332.220390340534,333.220126351255,334.219862361975,335.219598372695,336.219334383415,
337.219070394135,338.218806404855,339.218542415575,340.218278426295,341.218014437016,
342.217750447736,343.217486458456,344.217222469176,345.216958479896,346.216694490616,
347.216430501336,348.216166512056,349.215902522777,350.215638533497,351.215374544217,
352.215110554937,353.214846565657,354.214582576377,355.214318587097,356.214054597817,
357.213790608538,358.213526619258,359.213262629978,360.212998640698,361.212734651418,
362.212470662138,363.212206672858,364.211942683579,365.211678694299,366.211414705019,
367.211150715739,368.210886726459,369.210622737179,370.210358747899,371.210094758619,
372.20983076934,373.20956678006,374.20930279078,375.2090388015,376.20877481222,
377.20851082294,378.20824683366,379.20798284438,380.207718855101,381.207454865821,
382.207190876541,383.206926887261,384.206662897981,385.206398908701,386.206134919421,
387.205870930141,388.205606940862,389.205342951582,390.205078962302,391.204814973022,
392.204550983742,393.204286994462,394.204023005182,395.203759015903,396.203495026623,
397.203231037343,398.202967048063,399.202703058783,400.202439069503,401.202175080223,
402.201911090943,403.201647101664,404.201383112384,405.201119123104,406.200855133824,
407.200591144544,408.200327155264,409.200063165984,410.199799176704,411.199535187425,
412.199271198145,413.199007208865,414.198743219585,415.198479230305,416.198215241025,
417.197951251745,418.197687262465,419.197423273186,420.197159283906,421.196895294626,
422.196631305346,423.196367316066,424.196103326786,425.195839337506,426.195575348226,
427.195311358947,428.195047369667,429.194783380387,430.194519391107,431.194255401827,
432.193991412547,433.193727423267,434.193463433988,435.193199444708,436.192935455428,
437.192671466148,438.192407476868,439.192143487588,440.191879498308,441.191615509028,
442.191351519749,443.191087530469,444.190823541189,445.190559551909,446.190295562629,
447.190031573349,448.189767584069,449.189503594789,450.18923960551,451.18897561623,
452.18871162695,453.18844763767,454.18818364839,455.18791965911,456.18765566983,
457.18739168055,458.187127691271,459.186863701991,460.186599712711,461.186335723431,
462.186071734151,463.185807744871,464.185543755591,465.185279766312,466.185015777032,
467.184751787752,468.184487798472,469.184223809192,470.183959819912,471.183695830632,
472.183431841352,473.183167852073,474.182903862793,475.182639873513,476.182375884233,
477.182111894953,478.181847905673,479.181583916393,480.181319927113,481.181055937834,
482.180791948554,483.180527959274,484.180263969994,485.179999980714,486.179735991434,
487.179472002154,488.179208012874,489.178944023595,490.178680034315,491.178416045035,
492.178152055755,493.177888066475,494.177624077195,495.177360087915,496.177096098636,
497.176832109356,498.176568120076,499.176304130796,500.176040141516,501.175776152236,
502.175512162956,503.175248173676,504.174984184397,505.174720195117,506.174456205837,
507.174192216557,508.173928227277,509.173664237997,510.173400248717,511.173136259437,
512.172872270158,513.172608280878,514.172344291598,515.172080302318,516.171816313038,
517.171552323758,518.171288334478,519.171024345198,520.170760355919,521.170496366639,
522.170232377359,523.169968388079,524.169704398799,525.169440409519,526.169176420239,
527.168912430959,528.16864844168,529.1683844524,530.16812046312,531.16785647384,
532.16759248456,533.16732849528,534.167064506,535.166800516721,536.166536527441,
537.166272538161,538.166008548881,539.165744559601,540.165480570321,541.165216581041,
542.164952591761,543.164688602482,544.164424613202,545.164160623922,546.163896634642,
547.163632645362,548.163368656082,549.163104666802,550.162840677522,551.162576688243,
552.162312698963,553.162048709683,554.161784720403,555.161520731123,556.161256741843,
557.160992752563,558.160728763283,559.160464774004,560.160200784724,561.159936795444,
562.159672806164,563.159408816884,564.159144827604,565.158880838324,566.158616849045,
567.158352859765,568.158088870485,569.157824881205,570.157560891925,571.157296902645,
572.157032913365,573.156768924085,574.156504934806,575.156240945526,576.155976956246,
577.155712966966,578.155448977686,579.155184988406,580.154920999126,581.154657009846,
582.154393020567,583.154129031287,584.153865042007,585.153601052727,586.153337063447,
587.153073074167,588.152809084887,589.152545095607,590.152281106328,591.152017117048,
592.151753127768,593.151489138488,594.151225149208,595.150961159928,596.150697170648,
597.150433181368,598.150169192089,599.149905202809,600.149641213529,601.149377224249,
602.149113234969,603.148849245689,604.148585256409,605.14832126713,606.14805727785,
607.14779328857,608.14752929929,609.14726531001,610.14700132073,611.14673733145,
612.14647334217,613.146209352891,614.145945363611,615.145681374331,616.145417385051,
617.145153395771,618.144889406491,619.144625417211,620.144361427931,621.144097438652,
622.143833449372,623.143569460092,624.143305470812,625.143041481532,626.142777492252,
627.142513502972,628.142249513692,629.141985524413,630.141721535133,631.141457545853,
632.141193556573,633.140929567293,634.140665578013,635.140401588733,636.140137599454,
637.139873610174,638.139609620894,639.139345631614,640.139081642334,641.138817653054,
642.138553663774,643.138289674494,644.138025685215,645.137761695935,646.137497706655,
647.137233717375,648.136969728095,649.136705738815,650.136441749535,651.136177760255,
652.135913770976,653.135649781696,654.135385792416,655.135121803136,656.134857813856,
657.134593824576,658.134329835296,659.134065846016,660.133801856737,661.133537867457,
662.133273878177,663.133009888897,664.132745899617,665.132481910337,666.132217921057,
667.131953931778,668.131689942498,669.131425953218,670.131161963938,671.130897974658,
672.130633985378,673.130369996098,674.130106006818,675.129842017539,676.129578028259,
677.129314038979,678.129050049699,679.128786060419,680.128522071139,681.128258081859,
682.127994092579,683.1277301033,684.12746611402,685.12720212474,686.12693813546,
687.12667414618,688.1264101569,689.12614616762,690.12588217834,691.125618189061,
692.125354199781,693.125090210501,694.124826221221,695.124562231941,696.124298242661,
697.124034253381,698.123770264101,699.123506274822,700.123242285542,701.122978296262,
702.122714306982,703.122450317702,704.122186328422,705.121922339142,706.121658349863,
707.121394360583,708.121130371303,709.120866382023,710.120602392743,711.120338403463,
712.120074414183,713.119810424903,714.119546435624,715.119282446344,716.119018457064,
717.118754467784,718.118490478504,719.118226489224,720.117962499944,721.117698510664,
722.117434521385,723.117170532105,724.116906542825,725.116642553545,726.116378564265,
727.116114574985,728.115850585705,729.115586596425,730.115322607146,731.115058617866,
732.114794628586,733.114530639306,734.114266650026,735.114002660746,736.113738671466,
737.113474682187,738.113210692907,739.112946703627,740.112682714347,741.112418725067,
742.112154735787,743.111890746507,744.111626757227,745.111362767948,746.111098778668,
747.110834789388,748.110570800108,749.110306810828,750.110042821548,751.109778832268,
752.109514842988,753.109250853709,754.108986864429,755.108722875149,756.108458885869,
757.108194896589,758.107930907309,759.107666918029,760.107402928749,761.10713893947,
762.10687495019,763.10661096091,764.10634697163,765.10608298235,766.10581899307,
767.10555500379,768.10529101451,769.105027025231,770.104763035951,771.104499046671,
772.104235057391,773.103971068111,774.103707078831,775.103443089551,776.103179100272,
777.102915110992,778.102651121712,779.102387132432,780.102123143152,781.101859153872,
782.101595164592,783.101331175312,784.101067186033,785.100803196753,786.100539207473,
787.100275218193,788.100011228913,789.099747239633,790.099483250353,791.099219261073,
792.098955271794,793.098691282514,794.098427293234,795.098163303954,796.097899314674,
797.097635325394,798.097371336114,799.097107346834,800.096843357555,801.096579368275,
802.096315378995,803.096051389715,804.095787400435,805.095523411155,806.095259421875,
807.094995432596,808.094731443316,809.094467454036,810.094203464756,811.093939475476,
812.093675486196,813.093411496916,814.093147507636,815.092883518357,816.092619529077,
817.092355539797,818.092091550517,819.091827561237,820.091563571957,821.091299582677,
822.091035593397,823.090771604118,824.090507614838,825.090243625558,826.089979636278,
827.089715646998,828.089451657718,829.089187668438,830.088923679158,831.088659689879,
832.088395700599,833.088131711319,834.087867722039,835.087603732759,836.087339743479,
837.087075754199,838.08681176492,839.08654777564,840.08628378636,841.08601979708,
842.0857558078,843.08549181852,844.08522782924,845.08496383996,846.084699850681,
847.084435861401,848.084171872121,849.083907882841,850.083643893561,851.083379904281,
852.083115915001,853.082851925721,854.082587936442,855.082323947162,856.082059957882,
857.081795968602,858.081531979322,859.081267990042,860.081004000762,861.080740011482,
862.080476022203,863.080212032923,864.079948043643,865.079684054363,866.079420065083,
867.079156075803,868.078892086523,869.078628097243,870.078364107964,871.078100118684,
872.077836129404,873.077572140124,874.077308150844,875.077044161564,876.076780172284,
877.076516183005,878.076252193725,879.075988204445,880.075724215165,881.075460225885,
882.075196236605,883.074932247325,884.074668258045,885.074404268766,886.074140279486,
887.073876290206,888.073612300926,889.073348311646,890.073084322366,891.072820333086,
892.072556343806,893.072292354527,894.072028365247,895.071764375967,896.071500386687,
897.071236397407,898.070972408127,899.070708418847,900.070444429567,901.070180440288,
902.069916451008,903.069652461728,904.069388472448,905.069124483168,906.068860493888,
907.068596504608,908.068332515329,909.068068526049,910.067804536769,911.067540547489,
912.067276558209,913.067012568929,914.066748579649,915.066484590369,916.06622060109,
917.06595661181,918.06569262253,919.06542863325,920.06516464397,921.06490065469,
922.06463666541,923.06437267613,924.064108686851,925.063844697571,926.063580708291,
927.063316719011,928.063052729731,929.062788740451,930.062524751171,931.062260761891,
932.061996772612,933.061732783332,934.061468794052,935.061204804772,936.060940815492,
937.060676826212,938.060412836932,939.060148847652,940.059884858373,941.059620869093,
942.059356879813,943.059092890533,944.058828901253,945.058564911973,946.058300922693,
947.058036933414,948.057772944134,949.057508954854,950.057244965574,951.056980976294,
952.056716987014,953.056452997734,954.056189008454,955.055925019175,956.055661029895,
957.055397040615,958.055133051335,959.054869062055,960.054605072775,961.054341083495,
962.054077094215,963.053813104936,964.053549115656,965.053285126376,966.053021137096,
967.052757147816,968.052493158536,969.052229169256,970.051965179976,971.051701190697,
972.051437201417,973.051173212137,974.050909222857,975.050645233577,976.050381244297,
977.050117255017,978.049853265738,979.049589276458,980.049325287178,981.049061297898,
982.048797308618,983.048533319338,984.048269330058,985.048005340778,986.047741351499,
987.047477362219,988.047213372939,989.046949383659,990.046685394379,991.046421405099,
992.046157415819,993.045893426539,994.04562943726,995.04536544798,996.0451014587,
997.04483746942,998.04457348014,999.04430949086,1000.04404550158,1001.0437815123,
1002.04351752302,1003.04325353374,1004.04298954446,1005.04272555518,1006.0424615659,
1007.04219757662,1008.04193358734,1009.04166959806,1010.04140560878,1011.0411416195,
1012.04087763022,1013.04061364094,1014.04034965166,1015.04008566238,1016.0398216731,
1017.03955768382,1018.03929369454,1019.03902970526,1020.03876571598,1021.0385017267,
1022.03823773742,1023.03797374814,1024.03770975886,1025.03744576958,1026.0371817803,
1027.03691779102,1028.03665380174,1029.03638981246,1030.03612582318,1031.0358618339,
1032.03559784462,1033.03533385534,1034.03506986606,1035.03480587678,1036.03454188751,
1037.03427789823,1038.03401390895,1039.03374991967,1040.03348593039,1041.03322194111,
1042.03295795183,1043.03269396255,1044.03242997327,1045.03216598399,1046.03190199471,
1047.03163800543,1048.03137401615,1049.03111002687,1050.03084603759,1051.03058204831,
1052.03031805903,1053.03005406975,1054.02979008047,1055.02952609119,1056.02926210191,
1057.02899811263,1058.02873412335,1059.02847013407,1060.02820614479,1061.02794215551,
1062.02767816623,1063.02741417695,1064.02715018767,1065.02688619839,1066.02662220911,
1067.02635821983,1068.02609423055,1069.02583024127,1070.02556625199,1071.02530226271,
1072.02503827343,1073.02477428415,1074.02451029487,1075.02424630559,1076.02398231631,
1077.02371832703,1078.02345433775,1079.02319034847,1080.02292635919,1081.02266236991,
1082.02239838063,1083.02213439135,1084.02187040207,1085.02160641279,1086.02134242351,
1087.02107843423,1088.02081444495,1089.02055045567,1090.02028646639,1091.02002247711,
1092.01975848783,1093.01949449855,1094.01923050927,1095.01896651999,1096.01870253071,
1097.01843854143,1098.01817455215,1099.01791056287,1100.01764657359,1101.01738258431,
1102.01711859503,1103.01685460575,1104.01659061647,1105.01632662719,1106.01606263791,
1107.01579864863,1108.01553465935,1109.01527067007,1110.01500668079,1111.01474269151,
1112.01447870223,1113.01421471295,1114.01395072368,1115.0136867344,1116.01342274512,
1117.01315875584,1118.01289476656,1119.01263077728,1120.012366788,1121.01210279872,
1122.01183880944,1123.01157482016,1124.01131083088,1125.0110468416,1126.01078285232,
1127.01051886304,1128.01025487376,1129.00999088448,1130.0097268952,1131.00946290592,
1132.00919891664,1133.00893492736,1134.00867093808,1135.0084069488,1136.00814295952,
1137.00787897024,1138.00761498096,1139.00735099168,1140.0070870024,1141.00682301312,
1142.00655902384,1143.00629503456,1144.00603104528,1145.005767056,1146.00550306672,
1147.00523907744,1148.00497508816,1149.00471109888,1150.0044471096,1151.00418312032,
1152.00391913104,1153.00365514176,1154.00339115248,1155.0031271632,1156.00286317392,
1157.00259918464,1158.00233519536,1159.00207120608,1160.0018072168,1161.00154322752,
1162.00127923824,1163.00101524896,1164.00075125968,1165.0004872704,1166.00022328112,
1166.99995929184,1167.99969530256,1168.99943131328,1169.999167324,1170.99890333472,
1171.99863934544,1172.99837535616,1173.99811136688,1174.9978473776,1175.99758338832,
1176.99731939904,1177.99705540976,1178.99679142048,1179.9965274312,1180.99626344192,
1181.99599945264,1182.99573546336,1183.99547147408,1184.9952074848,1185.99494349552,
1186.99467950624,1187.99441551696,1188.99415152768,1189.99388753841,1190.99362354913,
1191.99335955985,1192.99309557057,1193.99283158129,1194.99256759201,1195.99230360273,
1196.99203961345,1197.99177562417,1198.99151163489,1199.99124764561,1200.99098365633,
1201.99071966705,1202.99045567777,1203.99019168849,1204.98992769921,1205.98966370993,
1206.98939972065,1207.98913573137,1208.98887174209,1209.98860775281,1210.98834376353,
1211.98807977425,1212.98781578497,1213.98755179569,1214.98728780641,1215.98702381713,
1216.98675982785,1217.98649583857,1218.98623184929,1219.98596786001,1220.98570387073,
1221.98543988145,1222.98517589217,1223.98491190289,1224.98464791361,1225.98438392433,
1226.98411993505,1227.98385594577,1228.98359195649,1229.98332796721,1230.98306397793,
1231.98279998865,1232.98253599937,1233.98227201009,1234.98200802081,1235.98174403153,
1236.98148004225,1237.98121605297,1238.98095206369,1239.98068807441,1240.98042408513,
1241.98016009585,1242.97989610657,1243.97963211729,1244.97936812801,1245.97910413873,
1246.97884014945,1247.97857616017,1248.97831217089,1249.97804818161,1250.97778419233,
1251.97752020305,1252.97725621377,1253.97699222449,1254.97672823521,1255.97646424593,
1256.97620025665,1257.97593626737,1258.97567227809,1259.97540828881,1260.97514429953,
1261.97488031025,1262.97461632097,1263.97435233169,1264.97408834241,1265.97382435313,
1266.97356036385,1267.97329637458,1268.9730323853,1269.97276839602,1270.97250440674,
1271.97224041746,1272.97197642818,1273.9717124389,1274.97144844962,1275.97118446034,
1276.97092047106,1277.97065648178,1278.9703924925,1279.97012850322,1280.96986451394,
1281.96960052466,1282.96933653538,1283.9690725461,1284.96880855682,1285.96854456754,
1286.96828057826,1287.96801658898,1288.9677525997,1289.96748861042,1290.96722462114,
1291.96696063186,1292.96669664258,1293.9664326533,1294.96616866402,1295.96590467474,
1296.96564068546,1297.96537669618,1298.9651127069,1299.96484871762,1300.96458472834,
1301.96432073906,1302.96405674978,1303.9637927605,1304.96352877122,1305.96326478194,
1306.96300079266,1307.96273680338,1308.9624728141,1309.96220882482,1310.96194483554,
1311.96168084626,1312.96141685698,1313.9611528677,1314.96088887842,1315.96062488914,
1316.96036089986,1317.96009691058,1318.9598329213,1319.95956893202,1320.95930494274,
1321.95904095346,1322.95877696418,1323.9585129749,1324.95824898562,1325.95798499634,
1326.95772100706,1327.95745701778,1328.9571930285,1329.95692903922,1330.95666504994,
1331.95640106066,1332.95613707138,1333.9558730821,1334.95560909282,1335.95534510354,
1336.95508111426,1337.95481712498,1338.9545531357,1339.95428914642,1340.95402515714,
1341.95376116786,1342.95349717858,1343.9532331893,1344.95296920002,1345.95270521075,
1346.95244122147,1347.95217723219,1348.95191324291,1349.95164925363,1350.95138526435,
1351.95112127507,1352.95085728579,1353.95059329651,1354.95032930723,1355.95006531795,
1356.94980132867,1357.94953733939,1358.94927335011,1359.94900936083,1360.94874537155,
1361.94848138227,1362.94821739299,1363.94795340371,1364.94768941443,1365.94742542515,
1366.94716143587,1367.94689744659,1368.94663345731,1369.94636946803,1370.94610547875,
1371.94584148947,1372.94557750019,1373.94531351091,1374.94504952163,1375.94478553235,
1376.94452154307,1377.94425755379,1378.94399356451,1379.94372957523,1380.94346558595,
1381.94320159667,1382.94293760739,1383.94267361811,1384.94240962883,1385.94214563955,
1386.94188165027,1387.94161766099,1388.94135367171,1389.94108968243,1390.94082569315,
1391.94056170387,1392.94029771459,1393.94003372531,1394.93976973603,1395.93950574675,
1396.93924175747,1397.93897776819,1398.93871377891,1399.93844978963,1400.93818580035,
1401.93792181107,1402.93765782179,1403.93739383251,1404.93712984323,1405.93686585395,
1406.93660186467,1407.93633787539,1408.93607388611,1409.93580989683,1410.93554590755,
1411.93528191827,1412.93501792899,1413.93475393971,1414.93448995043,1415.93422596115,
1416.93396197187,1417.93369798259,1418.93343399331,1419.93317000403,1420.93290601475,
1421.93264202547,1422.93237803619,1423.93211404692,1424.93185005764,1425.93158606836,
1426.93132207908,1427.9310580898,1428.93079410052,1429.93053011124,1430.93026612196,
1431.93000213268,1432.9297381434,1433.92947415412,1434.92921016484,1435.92894617556,
1436.92868218628,1437.928418197,1438.92815420772,1439.92789021844,1440.92762622916,
1441.92736223988,1442.9270982506,1443.92683426132,1444.92657027204,1445.92630628276,
1446.92604229348,1447.9257783042,1448.92551431492,1449.92525032564,1450.92498633636,
1451.92472234708,1452.9244583578,1453.92419436852,1454.92393037924,1455.92366638996,
1456.92340240068,1457.9231384114,1458.92287442212,1459.92261043284,1460.92234644356,
1461.92208245428,1462.921818465,1463.92155447572,1464.92129048644,1465.92102649716,
1466.92076250788,1467.9204985186,1468.92023452932,1469.91997054004,1470.91970655076,
1471.91944256148,1472.9191785722,1473.91891458292,1474.91865059364,1475.91838660436,
1476.91812261508,1477.9178586258,1478.91759463652,1479.91733064724,1480.91706665796,
1481.91680266868,1482.9165386794,1483.91627469012,1484.91601070084,1485.91574671156,
1486.91548272228,1487.915218733,1488.91495474372,1489.91469075444,1490.91442676516,
1491.91416277588,1492.9138987866,1493.91363479732,1494.91337080804,1495.91310681876,
1496.91284282948,1497.9125788402,1498.91231485092,1499.91205086164,1500.91178687236,
1501.91152288309,1502.91125889381,1503.91099490453,1504.91073091525,1505.91046692597,
1506.91020293669,1507.90993894741,1508.90967495813,1509.90941096885,1510.90914697957,
1511.90888299029,1512.90861900101,1513.90835501173,1514.90809102245,1515.90782703317,
1516.90756304389,1517.90729905461,1518.90703506533,1519.90677107605,1520.90650708677,
1521.90624309749,1522.90597910821,1523.90571511893,1524.90545112965,1525.90518714037,
1526.90492315109,1527.90465916181,1528.90439517253,1529.90413118325,1530.90386719397,
1531.90360320469,1532.90333921541,1533.90307522613,1534.90281123685,1535.90254724757,
1536.90228325829,1537.90201926901,1538.90175527973,1539.90149129045,1540.90122730117,
1541.90096331189,1542.90069932261,1543.90043533333,1544.90017134405,1545.89990735477,
1546.89964336549,1547.89937937621,1548.89911538693,1549.89885139765,1550.89858740837,
1551.89832341909,1552.89805942981,1553.89779544053,1554.89753145125,1555.89726746197,
1556.89700347269,1557.89673948341,1558.89647549413,1559.89621150485,1560.89594751557,
1561.89568352629,1562.89541953701,1563.89515554773,1564.89489155845,1565.89462756917,
1566.89436357989,1567.89409959061,1568.89383560133,1569.89357161205,1570.89330762277,
1571.89304363349,1572.89277964421,1573.89251565493,1574.89225166565,1575.89198767637,
1576.89172368709,1577.89145969781,1578.89119570853,1579.89093171926,1580.89066772998,
1581.8904037407,1582.89013975142,1583.88987576214,1584.88961177286,1585.88934778358,
1586.8890837943,1587.88881980502,1588.88855581574,1589.88829182646,1590.88802783718,
1591.8877638479,1592.88749985862,1593.88723586934,1594.88697188006,1595.88670789078,
1596.8864439015,1597.88617991222,1598.88591592294,1599.88565193366,1600.88538794438,
1601.8851239551,1602.88485996582,1603.88459597654,1604.88433198726,1605.88406799798,
1606.8838040087,1607.88354001942,1608.88327603014,1609.88301204086,1610.88274805158,
1611.8824840623,1612.88222007302,1613.88195608374,1614.88169209446,1615.88142810518,
1616.8811641159,1617.88090012662,1618.88063613734,1619.88037214806,1620.88010815878,
1621.8798441695,1622.87958018022,1623.87931619094,1624.87905220166,1625.87878821238,
1626.8785242231,1627.87826023382,1628.87799624454,1629.87773225526,1630.87746826598,
1631.8772042767,1632.87694028742,1633.87667629814,1634.87641230886,1635.87614831958,
1636.8758843303,1637.87562034102,1638.87535635174,1639.87509236246,1640.87482837318,
1641.8745643839,1642.87430039462,1643.87403640534,1644.87377241606,1645.87350842678,
1646.8732444375,1647.87298044822,1648.87271645894,1649.87245246966,1650.87218848038,
1651.8719244911,1652.87166050182,1653.87139651254,1654.87113252326,1655.87086853399,
1656.8706045447,1657.87034055543,1658.87007656615,1659.86981257687,1660.86954858759,
1661.86928459831,1662.86902060903,1663.86875661975,1664.86849263047,1665.86822864119,
1666.86796465191,1667.86770066263,1668.86743667335,1669.86717268407,1670.86690869479,
1671.86664470551,1672.86638071623,1673.86611672695,1674.86585273767,1675.86558874839,
1676.86532475911,1677.86506076983,1678.86479678055,1679.86453279127,1680.86426880199,
1681.86400481271,1682.86374082343,1683.86347683415,1684.86321284487,1685.86294885559,
1686.86268486631,1687.86242087703,1688.86215688775,1689.86189289847,1690.86162890919,
1691.86136491991,1692.86110093063,1693.86083694135,1694.86057295207,1695.86030896279,
1696.86004497351,1697.35991297887,1697.85988790214),.UNSPECIFIED.);
#1675=B_SPLINE_CURVE_WITH_KNOTS('',3,(#202538,#202539,#202540,#202541,#202542,
#202543,#202544,#202545,#202546,#202547,#202548,#202549,#202550),
 .UNSPECIFIED.,.F.,.F.,(4,3,3,3,4),(122.271018544109,122.275828089307,122.386363683307,
122.494373601401,122.522113489845),.UNSPECIFIED.);
#1676=B_SPLINE_CURVE_WITH_KNOTS('',3,(#202552,#202553,#202554,#202555,#202556,
#202557,#202558,#202559,#202560,#202561,#202562,#202563,#202564,#202565,
#202566,#202567,#202568,#202569,#202570,#202571,#202572,#202573,#202574,
#202575,#202576,#202577,#202578,#202579,#202580,#202581,#202582,#202583,
#202584,#202585,#202586,#202587,#202588,#202589,#202590,#202591,#202592,
#202593,#202594,#202595,#202596,#202597,#202598,#202599,#202600,#202601,
#202602,#202603,#202604,#202605,#202606,#202607,#202608,#202609,#202610,
#202611,#202612,#202613,#202614,#202615,#202616,#202617,#202618,#202619,
#202620,#202621,#202622,#202623,#202624,#202625,#202626,#202627,#202628,
#202629,#202630,#202631,#202632,#202633,#202634,#202635,#202636,#202637,
#202638,#202639,#202640,#202641,#202642,#202643,#202644,#202645,#202646,
#202647,#202648,#202649,#202650,#202651,#202652,#202653,#202654,#202655,
#202656,#202657,#202658,#202659,#202660,#202661,#202662,#202663,#202664,
#202665,#202666,#202667,#202668,#202669,#202670,#202671,#202672,#202673,
#202674,#202675,#202676,#202677,#202678,#202679,#202680,#202681,#202682,
#202683,#202684,#202685,#202686,#202687),.UNSPECIFIED.,.F.,.F.,(4,3,3,3,
3,3,3,3,3,3,3,3,3,3,3,3,3,3,3,3,3,3,3,3,3,3,3,3,3,3,3,3,3,3,3,3,3,3,3,3,
3,3,3,3,3,4),(122.522113489983,122.604654564358,122.688518256317,122.770981109149,
122.853436233243,122.93590249609,123.020817897075,123.103407097541,123.189485598785,
123.275564100028,123.359302811874,123.442938323242,123.52649076664,123.609980202491,
123.693434153104,123.77687064695,123.860307756706,123.943763551624,124.027308044353,
124.110897127294,124.194620394852,124.275300110748,124.359038822594,124.442674333961,
124.52622677736,124.609716213211,124.693170163825,124.776606657671,124.860043767426,
124.943499562344,125.027044055074,125.110633138015,125.194356405572,125.275036121468,
125.358775798738,125.442412049688,125.52596500778,125.609454734154,125.692907813588,
125.776343116971,125.859778716762,125.943232681716,126.026770899361,126.110353575267,
126.194059974238,126.257648866041),.UNSPECIFIED.);
#1677=B_SPLINE_CURVE_WITH_KNOTS('',3,(#202689,#202690,#202691,#202692,#202693,
#202694),.UNSPECIFIED.,.F.,.F.,(4,2,4),(0.311503179138839,0.373508504209549,
0.467472020546751),.UNSPECIFIED.);
#1678=B_SPLINE_CURVE_WITH_KNOTS('',3,(#202696,#202697,#202698,#202699,#202700,
#202701,#202702,#202703,#202704,#202705,#202706,#202707,#202708,#202709,
#202710,#202711,#202712,#202713,#202714,#202715,#202716,#202717,#202718,
#202719,#202720,#202721,#202722,#202723,#202724,#202725,#202726,#202727,
#202728,#202729,#202730,#202731,#202732,#202733,#202734,#202735,#202736,
#202737,#202738,#202739,#202740,#202741,#202742,#202743,#202744,#202745,
#202746,#202747,#202748,#202749,#202750,#202751,#202752,#202753,#202754,
#202755,#202756,#202757,#202758,#202759,#202760,#202761,#202762,#202763,
#202764,#202765,#202766,#202767,#202768,#202769,#202770,#202771,#202772,
#202773,#202774,#202775,#202776,#202777,#202778,#202779,#202780,#202781,
#202782,#202783,#202784,#202785,#202786,#202787,#202788,#202789,#202790,
#202791,#202792,#202793,#202794,#202795,#202796,#202797,#202798,#202799,
#202800,#202801,#202802,#202803,#202804,#202805,#202806,#202807,#202808,
#202809,#202810,#202811,#202812,#202813,#202814,#202815,#202816,#202817,
#202818,#202819,#202820,#202821,#202822,#202823,#202824,#202825,#202826,
#202827,#202828,#202829,#202830,#202831,#202832,#202833,#202834,#202835,
#202836,#202837,#202838,#202839,#202840,#202841,#202842,#202843),
 .UNSPECIFIED.,.F.,.F.,(4,3,3,3,3,3,3,3,3,3,3,3,3,3,3,3,3,3,3,3,3,3,3,3,
3,3,3,3,3,3,3,3,3,3,3,3,3,3,3,3,3,3,3,3,3,3,3,3,3,4),(122.522113489987,
122.586118709022,122.669857420868,122.753492932236,122.837045375634,122.920534811485,
123.003988762099,123.087425255945,123.170862365701,123.254318160619,123.337862653349,
123.42145173629,123.505175003848,123.585854719742,123.669593431588,123.753228942956,
123.836781386354,123.920270822205,124.003724772819,124.087161266665,124.170598376421,
124.254054171338,124.337598664068,124.421187747009,124.504911014567,124.585590730463,
124.669329442309,124.752964953677,124.836517397075,124.920006832926,125.00346078354,
125.086897277386,125.170334387142,125.253790182059,125.337334674789,125.42092375773,
125.504647025288,125.585326741183,125.669066152481,125.752702199374,125.836255015062,
125.91974466049,126.003197973538,126.086633598068,126.170069606594,126.253524068008,
126.337063985111,126.420648396645,126.504359337024,126.572633808289),
 .UNSPECIFIED.);
#1679=B_SPLINE_CURVE_WITH_KNOTS('',3,(#202844,#202845,#202846,#202847,#202848,
#202849,#202850,#202851,#202852,#202853),.UNSPECIFIED.,.F.,.F.,(4,3,3,4),
(122.27028827519,122.35308028165,122.43759688576,122.52211348987),
 .UNSPECIFIED.);
#1680=B_SPLINE_CURVE_WITH_KNOTS('',3,(#202859,#202860,#202861,#202862,#202863,
#202864,#202865,#202866,#202867,#202868),.UNSPECIFIED.,.F.,.F.,(4,3,3,4),
(115.987147173825,116.070212549419,116.154570366029,116.238928182639),
 .UNSPECIFIED.);
#1681=B_SPLINE_CURVE_WITH_KNOTS('',3,(#202869,#202870,#202871,#202872,#202873,
#202874,#202875,#202876,#202877,#202878,#202879,#202880,#202881,#202882,
#202883,#202884,#202885,#202886,#202887,#202888,#202889,#202890,#202891,
#202892,#202893,#202894,#202895,#202896,#202897,#202898,#202899,#202900,
#202901,#202902,#202903,#202904,#202905,#202906,#202907,#202908,#202909,
#202910,#202911,#202912,#202913,#202914,#202915,#202916,#202917,#202918,
#202919,#202920,#202921,#202922,#202923,#202924,#202925,#202926,#202927,
#202928,#202929,#202930,#202931,#202932,#202933,#202934,#202935,#202936,
#202937,#202938,#202939,#202940,#202941,#202942,#202943,#202944,#202945,
#202946,#202947,#202948,#202949,#202950,#202951,#202952,#202953,#202954,
#202955,#202956,#202957,#202958,#202959,#202960,#202961,#202962,#202963,
#202964,#202965,#202966,#202967,#202968,#202969,#202970,#202971,#202972,
#202973,#202974,#202975,#202976,#202977,#202978,#202979,#202980,#202981,
#202982,#202983,#202984,#202985,#202986,#202987,#202988,#202989,#202990,
#202991,#202992,#202993,#202994,#202995,#202996,#202997,#202998,#202999,
#203000,#203001,#203002,#203003,#203004,#203005,#203006,#203007,#203008,
#203009,#203010,#203011,#203012,#203013,#203014,#203015,#203016,#203017,
#203018,#203019,#203020,#203021,#203022,#203023,#203024,#203025,#203026,
#203027,#203028,#203029,#203030,#203031,#203032,#203033,#203034,#203035,
#203036,#203037,#203038,#203039,#203040,#203041,#203042,#203043,#203044,
#203045,#203046,#203047,#203048,#203049,#203050,#203051,#203052,#203053,
#203054,#203055,#203056,#203057,#203058,#203059,#203060,#203061,#203062,
#203063,#203064,#203065,#203066,#203067,#203068,#203069,#203070,#203071,
#203072,#203073,#203074,#203075,#203076,#203077,#203078,#203079,#203080,
#203081,#203082,#203083,#203084,#203085,#203086,#203087,#203088),
 .UNSPECIFIED.,.F.,.F.,(4,3,3,3,3,3,3,3,3,3,3,3,3,3,3,3,3,3,3,3,3,3,3,3,
3,3,3,3,3,3,3,3,3,3,3,3,3,3,3,3,3,3,3,3,3,3,3,3,3,3,3,3,3,3,3,3,3,3,3,3,
3,3,3,3,3,3,3,3,3,3,3,3,3,4),(116.238928182803,116.277412024987,116.361150736833,
116.4447862482,116.528338691599,116.61182812745,116.695282078063,116.778718571909,
116.862155681664,116.945611476582,117.029155969311,117.112745052252,117.19646831981,
117.277148035707,117.360886747553,117.44452225892,117.528074702319,117.61156413817,
117.695018088784,117.77845458263,117.861891692385,117.945347487303,118.028891980033,
118.112481062974,118.196204330531,118.276884046427,118.360622758273,118.44425826964,
118.527810713039,118.61130014889,118.694754099503,118.77819059335,118.861627703105,
118.945083498023,119.028627990752,119.112217073693,119.195940341251,119.276620057147,
119.360358768993,119.44399428036,119.527546723759,119.61103615961,119.694490110224,
119.77792660407,119.861363713826,119.944819508743,120.028364001473,120.111953084414,
120.195676351972,120.276356067867,120.360094779713,120.44373029108,120.527282734479,
120.61077217033,120.694226120944,120.77766261479,120.861099724545,120.944555519463,
121.028100012192,121.111689095133,121.195412362691,121.276092078587,121.359831060277,
121.443466778056,121.5270193647,121.610508880833,121.693962581455,121.77739873563,
121.860835415973,121.944290691593,122.027833400628,122.111420662809,122.195139108014,
122.271018544109),.UNSPECIFIED.);
#1682=B_SPLINE_CURVE_WITH_KNOTS('',3,(#203090,#203091,#203092,#203093,#203094,
#203095,#203096,#203097,#203098,#203099,#203100,#203101,#203102,#203103,
#203104,#203105,#203106,#203107,#203108,#203109,#203110,#203111,#203112,
#203113,#203114,#203115,#203116,#203117,#203118,#203119,#203120,#203121,
#203122,#203123,#203124,#203125,#203126,#203127,#203128,#203129,#203130,
#203131,#203132,#203133,#203134,#203135,#203136,#203137,#203138,#203139,
#203140,#203141,#203142,#203143,#203144,#203145,#203146,#203147,#203148,
#203149,#203150,#203151,#203152,#203153,#203154,#203155,#203156,#203157,
#203158,#203159,#203160,#203161,#203162,#203163,#203164,#203165,#203166,
#203167,#203168,#203169,#203170,#203171,#203172,#203173,#203174,#203175,
#203176,#203177,#203178,#203179,#203180,#203181,#203182,#203183,#203184,
#203185,#203186,#203187,#203188,#203189,#203190,#203191,#203192,#203193,
#203194,#203195,#203196,#203197,#203198,#203199,#203200,#203201,#203202,
#203203,#203204,#203205,#203206,#203207,#203208,#203209,#203210,#203211,
#203212,#203213,#203214,#203215,#203216,#203217,#203218,#203219,#203220,
#203221,#203222,#203223,#203224,#203225,#203226,#203227,#203228,#203229,
#203230,#203231,#203232,#203233,#203234,#203235,#203236,#203237,#203238,
#203239,#203240,#203241,#203242,#203243,#203244,#203245,#203246,#203247,
#203248,#203249,#203250,#203251,#203252,#203253,#203254,#203255,#203256,
#203257,#203258,#203259,#203260,#203261,#203262,#203263,#203264,#203265,
#203266,#203267,#203268,#203269,#203270,#203271,#203272,#203273,#203274,
#203275,#203276,#203277,#203278,#203279,#203280,#203281,#203282,#203283,
#203284,#203285,#203286,#203287,#203288,#203289,#203290,#203291,#203292,
#203293,#203294,#203295,#203296,#203297,#203298,#203299,#203300,#203301,
#203302,#203303,#203304,#203305,#203306,#203307,#203308,#203309),
 .UNSPECIFIED.,.F.,.F.,(4,3,3,3,3,3,3,3,3,3,3,3,3,3,3,3,3,3,3,3,3,3,3,3,
3,3,3,3,3,3,3,3,3,3,3,3,3,3,3,3,3,3,3,3,3,3,3,3,3,3,3,3,3,3,3,3,3,3,3,3,
3,3,3,3,3,3,3,3,3,3,3,3,3,4),(116.238928183003,116.334849321083,116.431253899856,
116.528269407277,116.587702644701,116.671441356547,116.755076867914,116.838629311313,
116.922118747164,117.005572697778,117.089009191624,117.17244630138,117.255902096297,
117.339446589027,117.423035671968,117.506758939526,117.587438655422,117.671177367268,
117.754812878636,117.838365322034,117.921854757885,118.005308708499,118.088745202345,
118.172182312101,118.255638107018,118.339182599748,118.422771682689,118.506494950247,
118.587174666142,118.670913377988,118.754548889355,118.838101332754,118.921590768605,
119.005044719218,119.088481213064,119.17191832282,119.255374117737,119.338918610467,
119.422507693408,119.506230960966,119.586910676862,119.670649388708,119.754284900075,
119.837837343474,119.921326779325,120.004780729939,120.088217223785,120.17165433354,
120.255110128458,120.338654621188,120.422243704129,120.505966971687,120.586646687582,
120.670385399428,120.754020910795,120.837573354194,120.921062790045,121.004516740659,
121.087953234505,121.17139034426,121.254846139178,121.338390631908,121.421979714849,
121.505702982407,121.586382698302,121.671870895413,121.754714488921,121.837482997203,
121.920195242189,122.002869998466,122.085539448033,122.168206900628,122.250910091201,
122.27028827519),.UNSPECIFIED.);
#1683=B_SPLINE_CURVE_WITH_KNOTS('',3,(#203310,#203311,#203312,#203313,#203314,
#203315,#203316,#203317,#203318,#203319),.UNSPECIFIED.,.F.,.F.,(4,3,3,4),
(115.988071988884,116.071683453257,116.155305818032,116.238928182807),
 .UNSPECIFIED.);
#1684=B_SPLINE_CURVE_WITH_KNOTS('',3,(#203325,#203326,#203327,#203328,#203329,
#203330,#203331,#203332,#203333,#203334),.UNSPECIFIED.,.F.,.F.,(4,3,3,4),
(109.704756567473,109.787983735154,109.871863305389,109.955742875624),
 .UNSPECIFIED.);
#1685=B_SPLINE_CURVE_WITH_KNOTS('',3,(#203335,#203336,#203337,#203338,#203339,
#203340,#203341,#203342,#203343,#203344,#203345,#203346,#203347,#203348,
#203349,#203350,#203351,#203352,#203353,#203354,#203355,#203356,#203357,
#203358,#203359,#203360,#203361,#203362,#203363,#203364,#203365,#203366,
#203367,#203368,#203369,#203370,#203371,#203372,#203373,#203374,#203375,
#203376,#203377,#203378,#203379,#203380,#203381,#203382,#203383,#203384,
#203385,#203386,#203387,#203388,#203389,#203390,#203391,#203392,#203393,
#203394,#203395,#203396,#203397,#203398,#203399,#203400,#203401,#203402,
#203403,#203404,#203405,#203406,#203407,#203408,#203409,#203410,#203411,
#203412,#203413,#203414,#203415,#203416,#203417,#203418,#203419,#203420,
#203421,#203422,#203423,#203424,#203425,#203426,#203427,#203428,#203429,
#203430,#203431,#203432,#203433,#203434,#203435,#203436,#203437,#203438,
#203439,#203440,#203441,#203442,#203443,#203444,#203445,#203446,#203447,
#203448,#203449,#203450,#203451,#203452,#203453,#203454,#203455,#203456,
#203457,#203458,#203459,#203460,#203461,#203462,#203463,#203464,#203465,
#203466,#203467,#203468,#203469,#203470,#203471,#203472,#203473,#203474,
#203475,#203476,#203477,#203478,#203479,#203480,#203481,#203482,#203483,
#203484,#203485,#203486,#203487,#203488,#203489,#203490,#203491,#203492,
#203493,#203494,#203495,#203496,#203497,#203498,#203499,#203500,#203501,
#203502,#203503,#203504,#203505,#203506,#203507,#203508,#203509,#203510,
#203511,#203512,#203513,#203514,#203515,#203516,#203517,#203518,#203519,
#203520,#203521,#203522,#203523,#203524,#203525,#203526,#203527,#203528,
#203529,#203530,#203531,#203532,#203533,#203534,#203535,#203536,#203537,
#203538,#203539,#203540,#203541,#203542,#203543,#203544,#203545,#203546,
#203547,#203548,#203549,#203550,#203551,#203552,#203553,#203554),
 .UNSPECIFIED.,.F.,.F.,(4,3,3,3,3,3,3,3,3,3,3,3,3,3,3,3,3,3,3,3,3,3,3,3,
3,3,3,3,3,3,3,3,3,3,3,3,3,3,3,3,3,3,3,3,3,3,3,3,3,3,3,3,3,3,3,3,3,3,3,3,
3,3,3,3,3,3,3,3,3,3,3,3,3,4),(109.955742875801,110.053908632085,110.152728187028,
110.252279042651,110.278995960666,110.362734672512,110.446370183879,110.529922627278,
110.613412063129,110.696866013743,110.780302507589,110.863739617344,110.947195412262,
111.030739904991,111.114328987932,111.19805225549,111.278731971386,111.362470683232,
111.446106194599,111.529658637998,111.613148073849,111.696602024463,111.780038518309,
111.863475628064,111.946931422982,112.030475915712,112.114064998653,112.19778826621,
112.278467982106,112.362206693952,112.445842205319,112.529394648718,112.612884084569,
112.696338035182,112.779774529029,112.863211638784,112.946667433702,113.030211926431,
113.113801009372,113.19752427693,113.278203992826,113.361942704672,113.445578216039,
113.529130659438,113.612620095289,113.696074045903,113.779510539749,113.862947649505,
113.946403444422,114.029947937152,114.113537020093,114.197260287651,114.277940003546,
114.361678715392,114.44531422676,114.528866670158,114.612356106009,114.695810056623,
114.779246550469,114.862683660225,114.946139455142,115.029683947872,115.113273030813,
115.196996298371,115.277676014266,115.360916343682,115.444025174985,115.527058070878,
115.610033652872,115.692970496751,115.775902763453,115.858831416099,115.94180178495,
115.987147173825),.UNSPECIFIED.);
#1686=B_SPLINE_CURVE_WITH_KNOTS('',3,(#203556,#203557,#203558,#203559,#203560,
#203561,#203562,#203563,#203564,#203565,#203566,#203567,#203568,#203569,
#203570,#203571,#203572,#203573,#203574,#203575,#203576,#203577,#203578,
#203579,#203580,#203581,#203582,#203583,#203584,#203585,#203586,#203587,
#203588,#203589,#203590,#203591,#203592,#203593,#203594,#203595,#203596,
#203597,#203598,#203599,#203600,#203601,#203602,#203603,#203604,#203605,
#203606,#203607,#203608,#203609,#203610,#203611,#203612,#203613,#203614,
#203615,#203616,#203617,#203618,#203619,#203620,#203621,#203622,#203623,
#203624,#203625,#203626,#203627,#203628,#203629,#203630,#203631,#203632,
#203633,#203634,#203635,#203636,#203637,#203638,#203639,#203640,#203641,
#203642,#203643,#203644,#203645,#203646,#203647,#203648,#203649,#203650,
#203651,#203652,#203653,#203654,#203655,#203656,#203657,#203658,#203659,
#203660,#203661,#203662,#203663,#203664,#203665,#203666,#203667,#203668,
#203669,#203670,#203671,#203672,#203673,#203674,#203675,#203676,#203677,
#203678,#203679,#203680,#203681,#203682,#203683,#203684,#203685,#203686,
#203687,#203688,#203689,#203690,#203691,#203692,#203693,#203694,#203695,
#203696,#203697,#203698,#203699,#203700,#203701,#203702,#203703,#203704,
#203705,#203706,#203707,#203708,#203709,#203710,#203711,#203712,#203713,
#203714,#203715,#203716,#203717,#203718,#203719,#203720,#203721,#203722,
#203723,#203724,#203725,#203726,#203727,#203728,#203729,#203730,#203731,
#203732,#203733,#203734,#203735,#203736,#203737,#203738,#203739,#203740,
#203741,#203742,#203743,#203744,#203745,#203746,#203747,#203748,#203749,
#203750,#203751,#203752,#203753,#203754,#203755,#203756,#203757,#203758,
#203759,#203760,#203761,#203762,#203763,#203764,#203765,#203766,#203767,
#203768,#203769,#203770,#203771,#203772,#203773,#203774,#203775),
 .UNSPECIFIED.,.F.,.F.,(4,3,3,3,3,3,3,3,3,3,3,3,3,3,3,3,3,3,3,3,3,3,3,3,
3,3,3,3,3,3,3,3,3,3,3,3,3,3,3,3,3,3,3,3,3,3,3,3,3,3,3,3,3,3,3,3,3,3,3,3,
3,3,3,3,3,3,3,3,3,3,3,3,3,4),(109.955742875628,110.039648469011,110.123556652528,
110.207484832012,110.291450422462,110.375523162037,110.459655763239,110.543923584594,
110.589286580381,110.673025292227,110.756660803595,110.840213246993,110.923702682844,
111.007156633458,111.090593127304,111.17403023706,111.257486031977,111.341030524707,
111.424619607648,111.508342875206,111.589022591101,111.672761302947,111.756396814314,
111.839949257713,111.923438693564,112.006892644178,112.090329138024,112.173766247779,
112.257222042697,112.340766535426,112.424355618367,112.508078885925,112.588758601821,
112.672497313667,112.756132825034,112.839685268433,112.923174704284,113.006628654898,
113.090065148744,113.173502258499,113.256958053417,113.340502546147,113.424091629088,
113.507814896646,113.588494612541,113.672233324387,113.755868835754,113.839421279153,
113.922910715004,114.006364665617,114.089801159464,114.173238269219,114.256694064136,
114.340238556866,114.423827639807,114.507550907365,114.588230623261,114.671969335107,
114.755604846474,114.839157289873,114.922646725724,115.006100676337,115.089537170184,
115.172974279939,115.256430074857,115.339974567586,115.423563650527,115.507286918084,
115.587966633981,115.671933979496,115.755764025857,115.839515095663,115.923193376346,
115.988071988884),.UNSPECIFIED.);
#1687=B_SPLINE_CURVE_WITH_KNOTS('',3,(#203776,#203777,#203778,#203779,#203780,
#203781,#203782,#203783,#203784,#203785),.UNSPECIFIED.,.F.,.F.,(4,3,3,4),
(109.705270710528,109.800372858636,109.894864507288,109.955742875431),
 .UNSPECIFIED.);
#1688=B_SPLINE_CURVE_WITH_KNOTS('',3,(#203791,#203792,#203793,#203794,#203795,
#203796,#203797,#203798,#203799,#203800),.UNSPECIFIED.,.F.,.F.,(4,3,3,4),
(103.422164115585,103.515371370637,103.608104590454,103.672557568256),
 .UNSPECIFIED.);
#1689=B_SPLINE_CURVE_WITH_KNOTS('',3,(#203801,#203802,#203803,#203804,#203805,
#203806,#203807,#203808,#203809,#203810,#203811,#203812,#203813,#203814,
#203815,#203816,#203817,#203818,#203819,#203820,#203821,#203822,#203823,
#203824,#203825,#203826,#203827,#203828,#203829,#203830,#203831,#203832,
#203833,#203834,#203835,#203836,#203837,#203838,#203839,#203840,#203841,
#203842,#203843,#203844,#203845,#203846,#203847,#203848,#203849,#203850,
#203851,#203852,#203853,#203854,#203855,#203856,#203857,#203858,#203859,
#203860,#203861,#203862,#203863,#203864,#203865,#203866,#203867,#203868,
#203869,#203870,#203871,#203872,#203873,#203874,#203875,#203876,#203877,
#203878,#203879,#203880,#203881,#203882,#203883,#203884,#203885,#203886,
#203887,#203888,#203889,#203890,#203891,#203892,#203893,#203894,#203895,
#203896,#203897,#203898,#203899,#203900,#203901,#203902,#203903,#203904,
#203905,#203906,#203907,#203908,#203909,#203910,#203911,#203912,#203913,
#203914,#203915,#203916,#203917,#203918,#203919,#203920,#203921,#203922,
#203923,#203924,#203925,#203926,#203927,#203928,#203929,#203930,#203931,
#203932,#203933,#203934,#203935,#203936,#203937,#203938,#203939,#203940,
#203941,#203942,#203943,#203944,#203945,#203946,#203947,#203948,#203949,
#203950,#203951,#203952,#203953,#203954,#203955,#203956,#203957,#203958,
#203959,#203960,#203961,#203962,#203963,#203964,#203965,#203966,#203967,
#203968,#203969,#203970,#203971,#203972,#203973,#203974,#203975,#203976,
#203977,#203978,#203979,#203980,#203981,#203982,#203983,#203984,#203985,
#203986,#203987,#203988,#203989,#203990,#203991,#203992,#203993,#203994,
#203995,#203996,#203997,#203998,#203999,#204000,#204001,#204002,#204003,
#204004,#204005,#204006,#204007,#204008,#204009,#204010,#204011,#204012,
#204013,#204014,#204015,#204016,#204017,#204018,#204019,#204020),
 .UNSPECIFIED.,.F.,.F.,(4,3,3,3,3,3,3,3,3,3,3,3,3,3,3,3,3,3,3,3,3,3,3,3,
3,3,3,3,3,3,3,3,3,3,3,3,3,3,3,3,3,3,3,3,3,3,3,3,3,3,3,3,3,3,3,3,3,3,3,3,
3,3,3,3,3,3,3,3,3,3,3,3,3,4),(103.672557568444,103.756948747136,103.841357026278,
103.925799068812,104.014494275695,104.099107419003,104.18379133639,104.268605737223,
104.280579896345,104.364318608191,104.447954119558,104.531506562957,104.614995998808,
104.698449949422,104.781886443268,104.865323553023,104.948779347941,105.03232384067,
105.115912923611,105.199636191169,105.280315907065,105.364054618911,105.447690130278,
105.531242573677,105.614732009527,105.698185960141,105.781622453987,105.865059563743,
105.94851535866,106.03205985139,106.115648934331,106.199372201889,106.280051917785,
106.363790629631,106.447426140998,106.530978584397,106.614468020248,106.697921970862,
106.781358464708,106.864795574464,106.948251369382,107.031795862111,107.115384945052,
107.19910821261,107.279787928505,107.363526640351,107.447162151719,107.530714595117,
107.614204030968,107.697657981582,107.781094475428,107.864531585183,107.947987380101,
108.031531872831,108.115120955772,108.198844223329,108.279523939226,108.363262651072,
108.44689816244,108.530450605838,108.613940041689,108.697393992303,108.780830486149,
108.864267595905,108.947723390823,109.031267883552,109.114856966493,109.198580234051,
109.279259949946,109.362821357527,109.448305160013,109.531656885119,109.618206726296,
109.704756567473),.UNSPECIFIED.);
#1690=B_SPLINE_CURVE_WITH_KNOTS('',3,(#204022,#204023,#204024,#204025,#204026,
#204027,#204028,#204029,#204030,#204031,#204032,#204033,#204034,#204035,
#204036,#204037,#204038,#204039,#204040,#204041,#204042,#204043,#204044,
#204045,#204046,#204047,#204048,#204049,#204050,#204051,#204052,#204053,
#204054,#204055,#204056,#204057,#204058,#204059,#204060,#204061,#204062,
#204063,#204064,#204065,#204066,#204067,#204068,#204069,#204070,#204071,
#204072,#204073,#204074,#204075,#204076,#204077,#204078,#204079,#204080,
#204081,#204082,#204083,#204084,#204085,#204086,#204087,#204088,#204089,
#204090,#204091,#204092,#204093,#204094,#204095,#204096,#204097,#204098,
#204099,#204100,#204101,#204102,#204103,#204104,#204105,#204106,#204107,
#204108,#204109,#204110,#204111,#204112,#204113,#204114,#204115,#204116,
#204117,#204118,#204119,#204120,#204121,#204122,#204123,#204124,#204125,
#204126,#204127,#204128,#204129,#204130,#204131,#204132,#204133,#204134,
#204135,#204136,#204137,#204138,#204139,#204140,#204141,#204142,#204143,
#204144,#204145,#204146,#204147,#204148,#204149,#204150,#204151,#204152,
#204153,#204154,#204155,#204156,#204157,#204158,#204159,#204160,#204161,
#204162,#204163,#204164,#204165,#204166,#204167,#204168,#204169,#204170,
#204171,#204172,#204173,#204174,#204175,#204176,#204177,#204178,#204179,
#204180,#204181,#204182,#204183,#204184,#204185,#204186,#204187,#204188,
#204189,#204190,#204191,#204192,#204193,#204194,#204195,#204196,#204197,
#204198,#204199,#204200,#204201,#204202,#204203,#204204,#204205,#204206,
#204207,#204208,#204209,#204210,#204211,#204212,#204213,#204214,#204215,
#204216,#204217,#204218,#204219,#204220,#204221,#204222,#204223,#204224,
#204225,#204226,#204227,#204228,#204229,#204230,#204231,#204232,#204233,
#204234,#204235,#204236,#204237,#204238,#204239,#204240,#204241),
 .UNSPECIFIED.,.F.,.F.,(4,3,3,3,3,3,3,3,3,3,3,3,3,3,3,3,3,3,3,3,3,3,3,3,
3,3,3,3,3,3,3,3,3,3,3,3,3,3,3,3,3,3,3,3,3,3,3,3,3,3,3,3,3,3,3,3,3,3,3,3,
3,3,3,3,3,3,3,3,3,3,3,3,3,4),(103.672557568579,103.755338549975,103.838023743102,
103.920634109801,104.004413660583,104.086946693849,104.169472251958,104.252009159745,
104.336724498823,104.419384236231,104.505127376145,104.59087051606,104.674609227906,
104.758244739273,104.841797182672,104.925286618523,105.008740569137,105.092177062983,
105.175614172739,105.259069967657,105.342614460386,105.426203543327,105.509926810885,
105.59060652678,105.674345238626,105.757980749993,105.841533193392,105.925022629242,
106.008476579856,106.091913073702,106.175350183458,106.258805978375,106.342350471105,
106.425939554046,106.509662821604,106.5903425375,106.674081249346,106.757716760713,
106.841269204112,106.924758639964,107.008212590577,107.091649084424,107.175086194179,
107.258541989097,107.342086481826,107.425675564767,107.509398832325,107.59007854822,
107.673817260066,107.757452771433,107.841005214832,107.924494650683,108.007948601297,
108.091385095143,108.174822204899,108.258277999817,108.341822492546,108.425411575487,
108.509134843045,108.58981455894,108.673553270786,108.757188782154,108.840741225552,
108.924230661404,109.007684612017,109.091121105864,109.174558215619,109.258014010538,
109.341558503267,109.425147586208,109.508870853766,109.589550569661,109.68519153841,
109.705270710528),.UNSPECIFIED.);
#1691=B_SPLINE_CURVE_WITH_KNOTS('',3,(#204242,#204243,#204244,#204245,#204246,
#204247,#204248,#204249,#204250,#204251),.UNSPECIFIED.,.F.,.F.,(4,3,3,4),
(103.420910293148,103.506022399244,103.59113450534,103.672557568448),
 .UNSPECIFIED.);
#1692=B_SPLINE_CURVE_WITH_KNOTS('',3,(#204257,#204258,#204259,#204260,#204261,
#204262,#204263,#204264,#204265,#204266),.UNSPECIFIED.,.F.,.F.,(4,3,3,4),
(97.1377575899893,97.2214880297379,97.2824278213041,97.3893722612645),
 .UNSPECIFIED.);
#1693=B_SPLINE_CURVE_WITH_KNOTS('',3,(#204267,#204268,#204269,#204270,#204271,
#204272,#204273,#204274,#204275,#204276,#204277,#204278,#204279,#204280,
#204281,#204282,#204283,#204284,#204285,#204286,#204287,#204288,#204289,
#204290,#204291,#204292,#204293,#204294,#204295,#204296,#204297,#204298,
#204299,#204300,#204301,#204302,#204303,#204304,#204305,#204306,#204307,
#204308,#204309,#204310,#204311,#204312,#204313,#204314,#204315,#204316,
#204317,#204318,#204319,#204320,#204321,#204322,#204323,#204324,#204325,
#204326,#204327,#204328,#204329,#204330,#204331,#204332,#204333,#204334,
#204335,#204336,#204337,#204338,#204339,#204340,#204341,#204342,#204343,
#204344,#204345,#204346,#204347,#204348,#204349,#204350,#204351,#204352,
#204353,#204354,#204355,#204356,#204357,#204358,#204359,#204360,#204361,
#204362,#204363,#204364,#204365,#204366,#204367,#204368,#204369,#204370,
#204371,#204372,#204373,#204374,#204375,#204376,#204377,#204378,#204379,
#204380,#204381,#204382,#204383,#204384,#204385,#204386,#204387,#204388,
#204389,#204390,#204391,#204392,#204393,#204394,#204395,#204396,#204397,
#204398,#204399,#204400,#204401,#204402,#204403,#204404,#204405,#204406,
#204407,#204408,#204409,#204410,#204411,#204412,#204413,#204414,#204415,
#204416,#204417,#204418,#204419,#204420,#204421,#204422,#204423,#204424,
#204425,#204426,#204427,#204428,#204429,#204430,#204431,#204432,#204433,
#204434,#204435,#204436,#204437,#204438,#204439,#204440,#204441,#204442,
#204443,#204444,#204445,#204446,#204447,#204448,#204449,#204450,#204451,
#204452,#204453,#204454,#204455,#204456,#204457,#204458,#204459,#204460,
#204461,#204462,#204463,#204464,#204465,#204466,#204467,#204468,#204469,
#204470,#204471,#204472,#204473,#204474,#204475,#204476,#204477,#204478,
#204479,#204480,#204481,#204482,#204483,#204484,#204485,#204486),
 .UNSPECIFIED.,.F.,.F.,(4,3,3,3,3,3,3,3,3,3,3,3,3,3,3,3,3,3,3,3,3,3,3,3,
3,3,3,3,3,3,3,3,3,3,3,3,3,3,3,3,3,3,3,3,3,3,3,3,3,3,3,3,3,3,3,3,3,3,3,3,
3,3,3,3,3,3,3,3,3,3,3,3,3,4),(97.3893722614005,97.4719677846863,97.5544719674218,
97.6369058779297,97.7192955269354,97.8016628999257,97.884026934726,97.9664065640542,
98.0488700592945,98.1313770056035,98.2140118307161,98.2821638320243,98.3659025438702,
98.4495380552377,98.5330904986362,98.6165799344873,98.7000338851009,98.7834703789472,
98.8669074887027,98.9503632836207,99.0339077763503,99.1174968592912,99.2012201268488,
99.2818998427444,99.3656385545902,99.449274065958,99.5328265093568,99.6163159452077,
99.6997698958214,99.7832063896676,99.8666434994231,99.9500992943405,100.03364378707,
100.117232870011,100.200956137569,100.281635853465,100.365374565311,100.449010076678,
100.532562520077,100.616051955928,100.699505906542,100.782942400388,100.866379510144,
100.949835305062,101.033379797791,101.116968880732,101.20069214829,101.281371864185,
101.365110576031,101.448746087398,101.532298530797,101.615787966648,101.699241917262,
101.782678411108,101.866115520863,101.949571315781,102.033115808511,102.116704891452,
102.200428159009,102.281107874905,102.364846586751,102.448482098118,102.532034541517,
102.615523977367,102.698977927981,102.782414421827,102.865851531583,102.949307326501,
103.03285181923,103.116440902171,103.200164169729,103.280843885625,103.374544855062,
103.422164115585),.UNSPECIFIED.);
#1694=B_SPLINE_CURVE_WITH_KNOTS('',3,(#204488,#204489,#204490,#204491,#204492,
#204493,#204494,#204495,#204496,#204497,#204498,#204499,#204500,#204501,
#204502,#204503,#204504,#204505,#204506,#204507,#204508,#204509,#204510,
#204511,#204512,#204513,#204514,#204515,#204516,#204517,#204518,#204519,
#204520,#204521,#204522,#204523,#204524,#204525,#204526,#204527,#204528,
#204529,#204530,#204531,#204532,#204533,#204534,#204535,#204536,#204537,
#204538,#204539,#204540,#204541,#204542,#204543,#204544,#204545,#204546,
#204547,#204548,#204549,#204550,#204551,#204552,#204553,#204554,#204555,
#204556,#204557,#204558,#204559,#204560,#204561,#204562,#204563,#204564,
#204565,#204566,#204567,#204568,#204569,#204570,#204571,#204572,#204573,
#204574,#204575,#204576,#204577,#204578,#204579,#204580,#204581,#204582,
#204583,#204584,#204585,#204586,#204587,#204588,#204589,#204590,#204591,
#204592,#204593,#204594,#204595,#204596,#204597,#204598,#204599,#204600,
#204601,#204602,#204603,#204604,#204605,#204606,#204607,#204608,#204609,
#204610,#204611,#204612,#204613,#204614,#204615,#204616,#204617,#204618,
#204619,#204620,#204621,#204622,#204623,#204624,#204625,#204626,#204627,
#204628,#204629,#204630,#204631,#204632,#204633,#204634,#204635,#204636,
#204637,#204638,#204639,#204640,#204641,#204642,#204643,#204644,#204645,
#204646,#204647,#204648,#204649,#204650,#204651,#204652,#204653,#204654,
#204655,#204656,#204657,#204658,#204659,#204660,#204661,#204662,#204663,
#204664,#204665,#204666,#204667,#204668,#204669,#204670,#204671,#204672,
#204673,#204674,#204675,#204676,#204677,#204678,#204679,#204680,#204681,
#204682,#204683,#204684,#204685,#204686,#204687,#204688,#204689,#204690,
#204691,#204692,#204693,#204694,#204695,#204696,#204697,#204698,#204699,
#204700,#204701,#204702,#204703,#204704),.UNSPECIFIED.,.F.,.F.,(4,3,3,3,
3,3,3,3,3,3,3,3,3,3,3,3,3,3,3,3,3,3,3,3,3,3,3,3,3,3,3,3,3,3,3,3,3,3,3,3,
3,3,3,3,3,3,3,3,3,3,3,3,3,3,3,3,3,3,3,3,3,3,3,3,3,3,3,3,3,3,3,3,4),(97.3893722612683,
97.5085709008744,97.592718441019,97.676457152865,97.7600926642325,97.8436451076312,
97.9271345434824,98.0105884940961,98.0940249879424,98.177462097698,98.2609178926158,
98.3444623853455,98.4280514682866,98.5117747358442,98.5924544517391,98.676193163585,
98.7598286749525,98.843381118351,98.926870554202,99.0103245048157,99.0937609986619,
99.1771981084174,99.2606539033351,99.3441983960647,99.4277874790057,99.5115107465633,
99.5921904624593,99.6759291743052,99.7595646856727,99.8431171290711,99.9266065649221,
100.010060515536,100.093497009382,100.176934119137,100.260389914055,100.343934406785,
100.427523489726,100.511246757283,100.591926473179,100.675665185025,100.759300696393,
100.842853139791,100.926342575642,101.009796526256,101.093233020102,101.176670129858,
101.260125924776,101.343670417505,101.427259500446,101.510982768004,101.5916624839,
101.675401195746,101.759036707114,101.842589150512,101.926078586363,102.009532536977,
102.092969030823,102.176406140579,102.259861935497,102.343406428226,102.426995511167,
102.510718778725,102.59139849462,102.675147385514,102.758790830291,102.84233402803,
102.925820381412,103.009268009692,103.09269500225,103.176148517115,103.2596128892,
103.3431540916,103.420910293148),.UNSPECIFIED.);
#1695=B_SPLINE_CURVE_WITH_KNOTS('',3,(#204705,#204706,#204707,#204708,#204709,
#204710,#204711,#204712,#204713,#204714),.UNSPECIFIED.,.F.,.F.,(4,3,3,4),
(97.1377977613825,97.2200836147453,97.3047279379176,97.3893722610898),
 .UNSPECIFIED.);
#1696=B_SPLINE_CURVE_WITH_KNOTS('',3,(#204720,#204721,#204722,#204723,#204724,
#204725,#204726,#204727,#204728,#204729),.UNSPECIFIED.,.F.,.F.,(4,3,3,4),
(90.8545165002977,90.9367707195664,91.0214788367447,91.106186953923),
 .UNSPECIFIED.);
#1697=B_SPLINE_CURVE_WITH_KNOTS('',3,(#204730,#204731,#204732,#204733,#204734,
#204735,#204736,#204737,#204738,#204739,#204740,#204741,#204742,#204743,
#204744,#204745,#204746,#204747,#204748,#204749,#204750,#204751,#204752,
#204753,#204754,#204755,#204756,#204757,#204758,#204759,#204760,#204761,
#204762,#204763,#204764,#204765,#204766,#204767,#204768,#204769,#204770,
#204771,#204772,#204773,#204774,#204775,#204776,#204777,#204778,#204779,
#204780,#204781,#204782,#204783,#204784,#204785,#204786,#204787,#204788,
#204789,#204790,#204791,#204792,#204793,#204794,#204795,#204796,#204797,
#204798,#204799,#204800,#204801,#204802,#204803,#204804,#204805,#204806,
#204807,#204808,#204809,#204810,#204811,#204812,#204813,#204814,#204815,
#204816,#204817,#204818,#204819,#204820,#204821,#204822,#204823,#204824,
#204825,#204826,#204827,#204828,#204829,#204830,#204831,#204832,#204833,
#204834,#204835,#204836,#204837,#204838,#204839,#204840,#204841,#204842,
#204843,#204844,#204845,#204846,#204847,#204848,#204849,#204850,#204851,
#204852,#204853,#204854,#204855,#204856,#204857,#204858,#204859,#204860,
#204861,#204862,#204863,#204864,#204865,#204866,#204867,#204868,#204869,
#204870,#204871,#204872,#204873,#204874,#204875,#204876,#204877,#204878,
#204879,#204880,#204881,#204882,#204883,#204884,#204885,#204886,#204887,
#204888,#204889,#204890,#204891,#204892,#204893,#204894,#204895,#204896,
#204897,#204898,#204899,#204900,#204901,#204902,#204903,#204904,#204905,
#204906,#204907,#204908,#204909,#204910,#204911,#204912,#204913,#204914,
#204915,#204916,#204917,#204918,#204919,#204920,#204921,#204922,#204923,
#204924,#204925,#204926,#204927,#204928,#204929,#204930,#204931,#204932,
#204933,#204934,#204935,#204936,#204937,#204938,#204939,#204940,#204941,
#204942,#204943,#204944,#204945,#204946,#204947,#204948,#204949),
 .UNSPECIFIED.,.F.,.F.,(4,3,3,3,3,3,3,3,3,3,3,3,3,3,3,3,3,3,3,3,3,3,3,3,
3,3,3,3,3,3,3,3,3,3,3,3,3,3,3,3,3,3,3,3,3,3,3,3,3,3,3,3,3,3,3,3,3,3,3,3,
3,3,3,3,3,3,3,3,3,3,3,3,3,4),(91.1061869540849,91.2342698388801,91.2840117569834,
91.3677504688293,91.4513859801969,91.5349384235956,91.6184278594466,91.7018818100603,
91.7853183039066,91.8687554136621,91.95221120858,92.0357557013097,92.1193447842506,
92.2030680518082,92.2837477677035,92.3674864795494,92.4511219909169,92.5346744343155,
92.6181638701666,92.7016178207802,92.7850543146265,92.8684914243819,92.9519472192995,
93.0354917120292,93.1190807949702,93.2028040625277,93.2834837784236,93.3672224902695,
93.450858001637,93.5344104450355,93.6178998808865,93.7013538315002,93.7847903253464,
93.8682274351018,93.9516832300195,94.0352277227491,94.1188168056901,94.2025400732476,
94.2832197891438,94.3669585009898,94.4505940123573,94.5341464557559,94.6176358916069,
94.7010898422206,94.7845263360669,94.8679634458224,94.9514192407401,95.0349637334698,
95.1185528164108,95.2022760839684,95.2829557998639,95.3666945117099,95.4503300230774,
95.5338824664759,95.6173719023269,95.7008258529406,95.7842623467869,95.8676994565424,
95.9511552514601,96.0346997441898,96.1182888271308,96.2020120946884,96.282691810584,
96.3664390909035,96.4500812622947,96.5360408032565,96.6195259372999,96.7029733472777,
96.7864011215343,96.8698273312194,96.9532987109112,97.0367978149355,97.120372459563,
97.1377575899893),.UNSPECIFIED.);
#1698=B_SPLINE_CURVE_WITH_KNOTS('',3,(#204951,#204952,#204953,#204954,#204955,
#204956,#204957,#204958,#204959,#204960,#204961,#204962,#204963,#204964,
#204965,#204966,#204967,#204968,#204969,#204970,#204971,#204972,#204973,
#204974,#204975,#204976,#204977,#204978,#204979,#204980,#204981,#204982,
#204983,#204984,#204985,#204986,#204987,#204988,#204989,#204990,#204991,
#204992,#204993,#204994,#204995,#204996,#204997,#204998,#204999,#205000,
#205001,#205002,#205003,#205004,#205005,#205006,#205007,#205008,#205009,
#205010,#205011,#205012,#205013,#205014,#205015,#205016,#205017,#205018,
#205019,#205020,#205021,#205022,#205023,#205024,#205025,#205026,#205027,
#205028,#205029,#205030,#205031,#205032,#205033,#205034,#205035,#205036,
#205037,#205038,#205039,#205040,#205041,#205042,#205043,#205044,#205045,
#205046,#205047,#205048,#205049,#205050,#205051,#205052,#205053,#205054,
#205055,#205056,#205057,#205058,#205059,#205060,#205061,#205062,#205063,
#205064,#205065,#205066,#205067,#205068,#205069,#205070,#205071,#205072,
#205073,#205074,#205075,#205076,#205077,#205078,#205079,#205080,#205081,
#205082,#205083,#205084,#205085,#205086,#205087,#205088,#205089,#205090,
#205091,#205092,#205093,#205094,#205095,#205096,#205097,#205098,#205099,
#205100,#205101,#205102,#205103,#205104,#205105,#205106,#205107,#205108,
#205109,#205110,#205111,#205112,#205113,#205114,#205115,#205116,#205117,
#205118,#205119,#205120,#205121,#205122,#205123,#205124,#205125,#205126,
#205127,#205128,#205129,#205130,#205131,#205132,#205133,#205134,#205135,
#205136,#205137,#205138,#205139,#205140,#205141,#205142,#205143,#205144,
#205145,#205146,#205147,#205148,#205149,#205150,#205151,#205152,#205153,
#205154,#205155,#205156,#205157,#205158,#205159,#205160,#205161,#205162,
#205163,#205164,#205165,#205166,#205167,#205168,#205169,#205170),
 .UNSPECIFIED.,.F.,.F.,(4,3,3,3,3,3,3,3,3,3,3,3,3,3,3,3,3,3,3,3,3,3,3,3,
3,3,3,3,3,3,3,3,3,3,3,3,3,3,3,3,3,3,3,3,3,3,3,3,3,3,3,3,3,3,3,3,3,3,3,3,
3,3,3,3,3,3,3,3,3,3,3,3,3,4),(91.1061869542033,91.1940293877261,91.2820034417824,
91.3702005362681,91.4585174044926,91.5470388628258,91.5943023766982,91.6780410885441,
91.7616765999115,91.8452290433101,91.9287184791611,92.0121724297747,92.095608923621,
92.1790460333764,92.262501828294,92.3460463210237,92.4296354039646,92.5133586715222,
92.5940383874183,92.6777770992642,92.7614126106318,92.8449650540303,92.9284544898813,
93.011908440495,93.0953449343413,93.1787820440968,93.2622378390145,93.3457823317442,
93.4293714146852,93.5130946822428,93.5937743981385,93.6775131099844,93.7611486213519,
93.8447010647504,93.9281905006014,94.0116444512151,94.0950809450613,94.1785180548168,
94.2619738497344,94.3455183424641,94.429107425405,94.5128306929626,94.5935104088586,
94.6772491207046,94.7608846320721,94.8444370754706,94.9279265113217,95.0113804619354,
95.0948169557816,95.1782540655371,95.2617098604549,95.3452543531846,95.4288434361256,
95.5125667036832,95.5932464195787,95.6769851314246,95.7606206427921,95.8441730861908,
95.927662522042,96.0111164726556,96.0945529665019,96.1779900762574,96.2614458711751,
96.3449903639048,96.4285794468458,96.5123027144034,96.5929824302989,96.6755077426029,
96.7579368247763,96.8402888703964,96.9225805906639,97.0048367170366,97.0870887865323,
97.1377977613825),.UNSPECIFIED.);
#1699=B_SPLINE_CURVE_WITH_KNOTS('',3,(#205171,#205172,#205173,#205174,#205175,
#205176,#205177,#205178,#205179,#205180),.UNSPECIFIED.,.F.,.F.,(4,3,3,4),
(90.8558404966185,90.943003649067,91.0300245809721,91.1061869540887),
 .UNSPECIFIED.);
#1700=B_SPLINE_CURVE_WITH_KNOTS('',3,(#205186,#205187,#205188,#205189,#205190,
#205191,#205192,#205193,#205194,#205195),.UNSPECIFIED.,.F.,.F.,(4,3,3,4),
(84.5725992439732,84.6588962802708,84.7450885344468,84.8230016469053),
 .UNSPECIFIED.);
#1701=B_SPLINE_CURVE_WITH_KNOTS('',3,(#205196,#205197,#205198,#205199,#205200,
#205201,#205202,#205203,#205204,#205205,#205206,#205207,#205208,#205209,
#205210,#205211,#205212,#205213,#205214,#205215,#205216,#205217,#205218,
#205219,#205220,#205221,#205222,#205223,#205224,#205225,#205226,#205227,
#205228,#205229,#205230,#205231,#205232,#205233,#205234,#205235,#205236,
#205237,#205238,#205239,#205240,#205241,#205242,#205243,#205244,#205245,
#205246,#205247,#205248,#205249,#205250,#205251,#205252,#205253,#205254,
#205255,#205256,#205257,#205258,#205259,#205260,#205261,#205262,#205263,
#205264,#205265,#205266,#205267,#205268,#205269,#205270,#205271,#205272,
#205273,#205274,#205275,#205276,#205277,#205278,#205279,#205280,#205281,
#205282,#205283,#205284,#205285,#205286,#205287,#205288,#205289,#205290,
#205291,#205292,#205293,#205294,#205295,#205296,#205297,#205298,#205299,
#205300,#205301,#205302,#205303,#205304,#205305,#205306,#205307,#205308,
#205309,#205310,#205311,#205312,#205313,#205314,#205315,#205316,#205317,
#205318,#205319,#205320,#205321,#205322,#205323,#205324,#205325,#205326,
#205327,#205328,#205329,#205330,#205331,#205332,#205333,#205334,#205335,
#205336,#205337,#205338,#205339,#205340,#205341,#205342,#205343,#205344,
#205345,#205346,#205347,#205348,#205349,#205350,#205351,#205352,#205353,
#205354,#205355,#205356,#205357,#205358,#205359,#205360,#205361,#205362,
#205363,#205364,#205365,#205366,#205367,#205368,#205369,#205370,#205371,
#205372,#205373,#205374,#205375,#205376,#205377,#205378,#205379,#205380,
#205381,#205382,#205383,#205384,#205385,#205386,#205387,#205388,#205389,
#205390,#205391,#205392,#205393,#205394,#205395,#205396,#205397,#205398,
#205399,#205400,#205401,#205402,#205403,#205404,#205405,#205406,#205407,
#205408,#205409,#205410,#205411,#205412,#205413,#205414,#205415),
 .UNSPECIFIED.,.F.,.F.,(4,3,3,3,3,3,3,3,3,3,3,3,3,3,3,3,3,3,3,3,3,3,3,3,
3,3,3,3,3,3,3,3,3,3,3,3,3,3,3,3,3,3,3,3,3,3,3,3,3,3,3,3,3,3,3,3,3,3,3,3,
3,3,3,3,3,3,3,3,3,3,3,3,3,4),(84.8230016470632,84.9118882294179,85.0053150952291,
85.0946470022648,85.1841250841541,85.2738132970661,85.2855956926626,85.3693344045085,
85.452969915876,85.5365223592745,85.6200117951256,85.7034657457393,85.7869022395855,
85.8703393493409,85.9537951442584,86.0373396369881,86.1209287199291,86.2046519874867,
86.2853317033827,86.3690704152286,86.4527059265962,86.5362583699947,86.6197478058457,
86.7032017564594,86.7866382503057,86.8700753600612,86.9535311549789,87.0370756477086,
87.1206647306495,87.2043879982071,87.2850677141029,87.3688064259488,87.4524419373163,
87.5359943807148,87.6194838165659,87.7029377671795,87.7863742610257,87.8698113707812,
87.9532671656989,88.0368116584285,88.1204007413695,88.2041240089271,88.284803724823,
88.368542436669,88.4521779480365,88.535730391435,88.619219827286,88.7026737778997,
88.786110271746,88.8695473815015,88.9530031764193,89.036547669149,89.12013675209,
89.2038600196476,89.2845397355431,89.368278447389,89.4519139587565,89.5354664021551,
89.6189558380062,89.7024097886198,89.7858462824661,89.8692833922215,89.9527391871391,
90.0362836798687,90.1198727628097,90.2035960303673,90.2842757462633,90.3667505459319,
90.4491298248377,90.5314328034189,90.6136786176278,90.69588927706,90.7781041156691,
90.8545165002977),.UNSPECIFIED.);
#1702=B_SPLINE_CURVE_WITH_KNOTS('',3,(#205417,#205418,#205419,#205420,#205421,
#205422,#205423,#205424,#205425,#205426,#205427,#205428,#205429,#205430,
#205431,#205432,#205433,#205434,#205435,#205436,#205437,#205438,#205439,
#205440,#205441,#205442,#205443,#205444,#205445,#205446,#205447,#205448,
#205449,#205450,#205451,#205452,#205453,#205454,#205455,#205456,#205457,
#205458,#205459,#205460,#205461,#205462,#205463,#205464,#205465,#205466,
#205467,#205468,#205469,#205470,#205471,#205472,#205473,#205474,#205475,
#205476,#205477,#205478,#205479,#205480,#205481,#205482,#205483,#205484,
#205485,#205486,#205487,#205488,#205489,#205490,#205491,#205492,#205493,
#205494,#205495,#205496,#205497,#205498,#205499,#205500,#205501,#205502,
#205503,#205504,#205505,#205506,#205507,#205508,#205509,#205510,#205511,
#205512,#205513,#205514,#205515,#205516,#205517,#205518,#205519,#205520,
#205521,#205522,#205523,#205524,#205525,#205526,#205527,#205528,#205529,
#205530,#205531,#205532,#205533,#205534,#205535,#205536,#205537,#205538,
#205539,#205540,#205541,#205542,#205543,#205544,#205545,#205546,#205547,
#205548,#205549,#205550,#205551,#205552,#205553,#205554,#205555,#205556,
#205557,#205558,#205559,#205560,#205561,#205562,#205563,#205564,#205565,
#205566,#205567,#205568,#205569,#205570,#205571,#205572,#205573,#205574,
#205575,#205576,#205577,#205578,#205579,#205580,#205581,#205582,#205583,
#205584,#205585,#205586,#205587,#205588,#205589,#205590,#205591,#205592,
#205593,#205594,#205595,#205596,#205597,#205598,#205599,#205600,#205601,
#205602,#205603,#205604,#205605,#205606,#205607,#205608,#205609,#205610,
#205611,#205612,#205613,#205614,#205615,#205616,#205617,#205618,#205619,
#205620,#205621,#205622,#205623,#205624,#205625,#205626,#205627,#205628,
#205629,#205630,#205631,#205632,#205633,#205634,#205635,#205636),
 .UNSPECIFIED.,.F.,.F.,(4,3,3,3,3,3,3,3,3,3,3,3,3,3,3,3,3,3,3,3,3,3,3,3,
3,3,3,3,3,3,3,3,3,3,3,3,3,3,3,3,3,3,3,3,3,3,3,3,3,3,3,3,3,3,3,3,3,3,3,3,
3,3,3,3,3,3,3,3,3,3,3,3,3,4),(84.8230016470494,84.9054512045182,84.9917555930006,
85.0741114802006,85.1564545594353,85.2388037750452,85.3211780738551,85.4036410329863,
85.4861559906397,85.5687878473739,85.5958863123774,85.6796250242234,85.763260535591,
85.8468129789896,85.9303024148405,86.0137563654542,86.0971928593005,86.180629969056,
86.2640857639739,86.3476302567036,86.4312193396445,86.5149426072021,86.5956223230975,
86.6793610349434,86.762996546311,86.8465489897096,86.9300384255609,87.0134923761746,
87.0969288700208,87.1803659797762,87.2638217746938,87.3473662674234,87.4309553503644,
87.514678617922,87.5953583338177,87.6790970456637,87.7627325570311,87.8462850004296,
87.9297744362802,88.0132283868939,88.0966648807401,88.1801019904954,88.2635577854131,
88.3471022781427,88.4306913610839,88.5144146286414,88.5950943445378,88.6788330563837,
88.7624685677512,88.8460210111494,88.9295104470006,89.0129643976143,89.0964008914605,
89.1798380012159,89.2632937961336,89.3468382888634,89.4304273718043,89.5141506393619,
89.5948303552579,89.6785690671039,89.7622045784714,89.8457570218702,89.929246457721,
90.0127004083347,90.0961369021807,90.1795740119362,90.2630298068536,90.3465742995832,
90.430163382524,90.5138866500815,90.5945663659781,90.6821700263414,90.7695849001495,
90.8558404966185),.UNSPECIFIED.);
#1703=B_SPLINE_CURVE_WITH_KNOTS('',3,(#205637,#205638,#205639,#205640,#205641,
#205642,#205643,#205644,#205645,#205646),.UNSPECIFIED.,.F.,.F.,(4,3,3,4),
(84.571795089726,84.5961503016573,84.7095759742832,84.8230016469091),
 .UNSPECIFIED.);
#1704=B_SPLINE_CURVE_WITH_KNOTS('',3,(#205652,#205653,#205654,#205655,#205656,
#205657,#205658,#205659,#205660,#205661),.UNSPECIFIED.,.F.,.F.,(4,3,3,4),
(78.2887592231474,78.3981054868849,78.5051444124938,78.5398163395285),
 .UNSPECIFIED.);
#1705=B_SPLINE_CURVE_WITH_KNOTS('',3,(#205662,#205663,#205664,#205665,#205666,
#205667,#205668,#205669,#205670,#205671,#205672,#205673,#205674,#205675,
#205676,#205677,#205678,#205679,#205680,#205681,#205682,#205683,#205684,
#205685,#205686,#205687,#205688,#205689,#205690,#205691,#205692,#205693,
#205694,#205695,#205696,#205697,#205698,#205699,#205700,#205701,#205702,
#205703,#205704,#205705,#205706,#205707,#205708,#205709,#205710,#205711,
#205712,#205713,#205714,#205715,#205716,#205717,#205718,#205719,#205720,
#205721,#205722,#205723,#205724,#205725,#205726,#205727,#205728,#205729,
#205730,#205731,#205732,#205733,#205734,#205735,#205736,#205737,#205738,
#205739,#205740,#205741,#205742,#205743,#205744,#205745,#205746,#205747,
#205748,#205749,#205750,#205751,#205752,#205753,#205754,#205755,#205756,
#205757,#205758,#205759,#205760,#205761,#205762,#205763,#205764,#205765,
#205766,#205767,#205768,#205769,#205770,#205771,#205772,#205773,#205774,
#205775,#205776,#205777,#205778,#205779,#205780,#205781,#205782,#205783,
#205784,#205785,#205786,#205787,#205788,#205789,#205790,#205791,#205792,
#205793,#205794,#205795,#205796,#205797,#205798,#205799,#205800,#205801,
#205802,#205803,#205804,#205805,#205806,#205807,#205808,#205809,#205810,
#205811,#205812,#205813,#205814,#205815,#205816,#205817,#205818,#205819,
#205820,#205821,#205822,#205823,#205824,#205825,#205826,#205827,#205828,
#205829,#205830,#205831,#205832,#205833,#205834,#205835,#205836,#205837,
#205838,#205839,#205840,#205841,#205842,#205843,#205844,#205845,#205846,
#205847,#205848,#205849,#205850,#205851,#205852,#205853,#205854,#205855,
#205856,#205857,#205858,#205859,#205860,#205861,#205862,#205863,#205864,
#205865,#205866,#205867,#205868,#205869,#205870,#205871,#205872,#205873,
#205874,#205875,#205876,#205877,#205878,#205879,#205880,#205881),
 .UNSPECIFIED.,.F.,.F.,(4,3,3,3,3,3,3,3,3,3,3,3,3,3,3,3,3,3,3,3,3,3,3,3,
3,3,3,3,3,3,3,3,3,3,3,3,3,3,3,3,3,3,3,3,3,3,3,3,3,3,3,3,3,3,3,3,3,3,3,3,
3,3,3,3,3,3,3,3,3,3,3,3,3,4),(78.5398163397257,78.62239295459,78.705491288809,
78.7879946449525,78.8704919407165,78.9530020139644,79.0365464175588,79.1191811714259,
79.2031803998838,79.2871796283418,79.3709183401877,79.4545538515552,79.5381062949538,
79.6215957308051,79.7050496814187,79.788486175265,79.8719232850204,79.955379079938,
80.0389235726677,80.1225126556086,80.2062359231661,80.286915639062,80.3706543509079,
80.4542898622755,80.5378423056737,80.6213317415248,80.7047856921384,80.7882221859847,
80.8716592957401,80.9551150906578,81.0386595833875,81.1222486663285,81.2059719338861,
81.2866516497821,81.370390361628,81.4540258729957,81.5375783163942,81.6210677522452,
81.7045217028589,81.7879581967051,81.8713953064607,81.9548511013783,82.038395594108,
82.121984677049,82.2057079446065,82.2863876605022,82.3701263723481,82.4537618837154,
82.5373143271138,82.6208037629648,82.7042577135786,82.787694207425,82.8711313171803,
82.9545871120976,83.0381316048273,83.1217206877683,83.2054439553258,83.2861236712224,
83.3698623830682,83.4534978944356,83.5370503378342,83.6205397736848,83.7039937242985,
83.7874302181448,83.8708673279002,83.9543231228179,84.0378676155475,84.1214566984884,
84.2051799660461,84.2858596819425,84.3725698184977,84.4591613046955,84.5456123157065,
84.5725992439732),.UNSPECIFIED.);
#1706=B_SPLINE_CURVE_WITH_KNOTS('',3,(#205883,#205884,#205885,#205886,#205887,
#205888,#205889,#205890,#205891,#205892,#205893,#205894,#205895,#205896,
#205897,#205898,#205899,#205900,#205901,#205902,#205903,#205904,#205905,
#205906,#205907,#205908,#205909,#205910,#205911,#205912,#205913,#205914,
#205915,#205916,#205917,#205918,#205919,#205920,#205921,#205922,#205923,
#205924,#205925,#205926,#205927,#205928,#205929,#205930,#205931,#205932,
#205933,#205934,#205935,#205936,#205937,#205938,#205939,#205940,#205941,
#205942,#205943,#205944,#205945,#205946,#205947,#205948,#205949,#205950,
#205951,#205952,#205953,#205954,#205955,#205956,#205957,#205958,#205959,
#205960,#205961,#205962,#205963,#205964,#205965,#205966,#205967,#205968,
#205969,#205970,#205971,#205972,#205973,#205974,#205975,#205976,#205977,
#205978,#205979,#205980,#205981,#205982,#205983,#205984,#205985,#205986,
#205987,#205988,#205989,#205990,#205991,#205992,#205993,#205994,#205995,
#205996,#205997,#205998,#205999,#206000,#206001,#206002,#206003,#206004,
#206005,#206006,#206007,#206008,#206009,#206010,#206011,#206012,#206013,
#206014,#206015,#206016,#206017,#206018,#206019,#206020,#206021,#206022,
#206023,#206024,#206025,#206026,#206027,#206028,#206029,#206030,#206031,
#206032,#206033,#206034,#206035,#206036,#206037,#206038,#206039,#206040,
#206041,#206042,#206043,#206044,#206045,#206046,#206047,#206048,#206049,
#206050,#206051,#206052,#206053,#206054,#206055,#206056,#206057,#206058,
#206059,#206060,#206061,#206062,#206063,#206064,#206065,#206066,#206067,
#206068,#206069,#206070,#206071,#206072,#206073,#206074,#206075,#206076,
#206077,#206078,#206079,#206080,#206081,#206082,#206083,#206084,#206085,
#206086,#206087,#206088,#206089,#206090,#206091,#206092,#206093,#206094,
#206095,#206096,#206097,#206098,#206099,#206100,#206101,#206102),
 .UNSPECIFIED.,.F.,.F.,(4,3,3,3,3,3,3,3,3,3,3,3,3,3,3,3,3,3,3,3,3,3,3,3,
3,3,3,3,3,3,3,3,3,3,3,3,3,3,3,3,3,3,3,3,3,3,3,3,3,3,3,3,3,3,3,3,3,3,3,3,
3,3,3,3,3,3,3,3,3,3,3,3,3,4),(78.5398163397295,78.5977342373365,78.6814729491824,
78.7651084605499,78.8486609039486,78.9321503397996,79.0156042904133,79.0990407842595,
79.1824778940149,79.2659336889324,79.3494781816621,79.4330672646031,79.5167905321606,
79.5974702480566,79.6812089599025,79.76484447127,79.8483969146685,79.9318863505195,
80.0153403011332,80.0987767949795,80.1822139047349,80.2656696996526,80.3492141923823,
80.4328032753233,80.5165265428808,80.5972062587768,80.6809449706228,80.7645804819903,
80.8481329253889,80.93162236124,81.0150763118536,81.0985128056999,81.1819499154554,
81.2654057103731,81.3489502031028,81.4325392860438,81.5162625536014,81.5969422694969,
81.6806809813428,81.7643164927103,81.8478689361088,81.9313583719598,82.0148123225734,
82.0982488164197,82.1816859261751,82.2651417210928,82.3486862138224,82.4322752967634,
82.5159985643209,82.596678280217,82.680416992063,82.7640525034305,82.8476049468291,
82.9310943826802,83.0145483332938,83.0979848271401,83.1814219368956,83.2648777318133,
83.348422224543,83.432011307484,83.5157345750416,83.5964142909372,83.6801543798819,
83.7637909471208,83.847344126517,83.9308339795196,84.0142867067674,84.0977215231147,
84.1811565009327,84.264609708774,84.3481453391041,84.4317253719729,84.5154248974244,
84.571795089726),.UNSPECIFIED.);
#1707=B_SPLINE_CURVE_WITH_KNOTS('',3,(#206103,#206104,#206105,#206106),
 .UNSPECIFIED.,.F.,.F.,(4,4),(78.2879140477243,78.5398092039209),
 .UNSPECIFIED.);
#1708=B_SPLINE_CURVE_WITH_KNOTS('',3,(#206112,#206113,#206114,#206115,#206116,
#206117,#206118,#206119,#206120,#206121),.UNSPECIFIED.,.F.,.F.,(4,3,3,4),
(72.0048655224089,72.0880045572239,72.172317794814,72.256631032404),
 .UNSPECIFIED.);
#1709=B_SPLINE_CURVE_WITH_KNOTS('',3,(#206122,#206123,#206124,#206125,#206126,
#206127,#206128,#206129,#206130,#206131,#206132,#206133,#206134,#206135,
#206136,#206137,#206138,#206139,#206140,#206141,#206142,#206143,#206144,
#206145,#206146,#206147,#206148,#206149,#206150,#206151,#206152,#206153,
#206154,#206155,#206156,#206157,#206158,#206159,#206160,#206161,#206162,
#206163,#206164,#206165,#206166,#206167,#206168,#206169,#206170,#206171,
#206172,#206173,#206174,#206175,#206176,#206177,#206178,#206179,#206180,
#206181,#206182,#206183,#206184,#206185,#206186,#206187,#206188,#206189,
#206190,#206191,#206192,#206193,#206194,#206195,#206196,#206197,#206198,
#206199,#206200,#206201,#206202,#206203,#206204,#206205,#206206,#206207,
#206208,#206209,#206210,#206211,#206212,#206213,#206214,#206215,#206216,
#206217,#206218,#206219,#206220,#206221,#206222,#206223,#206224,#206225,
#206226,#206227,#206228,#206229,#206230,#206231,#206232,#206233,#206234,
#206235,#206236,#206237,#206238,#206239,#206240,#206241,#206242,#206243,
#206244,#206245,#206246,#206247,#206248,#206249,#206250,#206251,#206252,
#206253,#206254,#206255,#206256,#206257,#206258,#206259,#206260,#206261,
#206262,#206263,#206264,#206265,#206266,#206267,#206268,#206269,#206270,
#206271,#206272,#206273,#206274,#206275,#206276,#206277,#206278,#206279,
#206280,#206281,#206282,#206283,#206284,#206285,#206286,#206287,#206288,
#206289,#206290,#206291,#206292,#206293,#206294,#206295,#206296,#206297,
#206298,#206299,#206300,#206301,#206302,#206303,#206304,#206305,#206306,
#206307,#206308,#206309,#206310,#206311,#206312,#206313,#206314,#206315,
#206316,#206317,#206318,#206319,#206320,#206321,#206322,#206323,#206324,
#206325,#206326,#206327,#206328,#206329,#206330,#206331,#206332,#206333,
#206334,#206335,#206336,#206337,#206338,#206339,#206340,#206341,#206342,
#206343,#206344),.UNSPECIFIED.,.F.,.F.,(4,3,3,3,3,3,3,3,3,3,3,3,3,3,3,3,
3,3,3,3,3,3,3,3,3,3,3,3,3,3,3,3,3,3,3,3,3,3,3,3,3,3,3,3,3,3,3,3,3,3,3,3,
3,3,3,3,3,3,3,3,3,3,3,3,3,3,3,3,3,3,3,3,3,3,4),(72.2566310325461,72.2890275533009,
72.3727662651468,72.4564017765142,72.5399542199127,72.6234436557635,72.7068976063771,
72.7903341002233,72.8737712099786,72.9572270048961,73.0407714976257,73.1243605805666,
73.2080838481241,73.2887635640211,73.372502275867,73.4561377872345,73.539690230633,
73.6231796664841,73.7066336170977,73.790070110944,73.8735072206994,73.956963015617,
74.0405075083467,74.1240965912877,74.2078198588453,74.2884995747412,74.3722382865871,
74.4558737979546,74.5394262413532,74.6229156772043,74.7063696278179,74.7898061216642,
74.8732432314197,74.9566990263373,75.0402435190669,75.1238326020079,75.2075558695655,
75.2882355854613,75.3719742973073,75.4556098086748,75.5391622520734,75.6226516879244,
75.7061056385381,75.7895421323844,75.87297924214,75.9564350370577,76.0399795297874,
76.1235686127284,76.207291880286,76.2879715961814,76.3717103080273,76.4553458193948,
76.5388982627933,76.6223876986444,76.7058416492581,76.7892781431043,76.8727152528598,
76.9561710477774,77.0397155405071,77.1233046234481,77.2070278910057,77.2877076069016,
77.3714463187476,77.4550818301151,77.5386342735135,77.6221237093646,77.7055776599783,
77.7890141538246,77.8724512635801,77.9559070584978,78.0394515512275,78.1230406341685,
78.2067639017261,78.2874436176217,78.2887592231474),.UNSPECIFIED.);
#1710=B_SPLINE_CURVE_WITH_KNOTS('',3,(#206346,#206347,#206348,#206349,#206350,
#206351,#206352,#206353,#206354,#206355),.UNSPECIFIED.,.F.,.F.,(4,1,1,1,
1,1,1,4),(72.2566310325499,72.5993181730157,73.5990541837358,74.598790194456,
75.5985262051761,76.5982622158962,77.5979982266164,78.2879140477243),
 .UNSPECIFIED.);
#1711=B_SPLINE_CURVE_WITH_KNOTS('',3,(#206356,#206357,#206358,#206359),
 .UNSPECIFIED.,.F.,.F.,(4,4),(72.0060503087704,72.2566310325499),
 .UNSPECIFIED.);
#1712=B_SPLINE_CURVE_WITH_KNOTS('',3,(#206365,#206366,#206367,#206368,#206369,
#206370,#206371,#206372,#206373,#206374),.UNSPECIFIED.,.F.,.F.,(4,3,3,4),
(65.7224278061069,65.8055735571319,65.8895096412492,65.9734457253665),
 .UNSPECIFIED.);
#1713=B_SPLINE_CURVE_WITH_KNOTS('',3,(#206375,#206376,#206377,#206378,#206379,
#206380,#206381,#206382,#206383,#206384,#206385,#206386,#206387,#206388,
#206389,#206390,#206391,#206392,#206393,#206394,#206395,#206396,#206397,
#206398,#206399,#206400,#206401,#206402,#206403,#206404,#206405,#206406,
#206407,#206408,#206409,#206410,#206411,#206412,#206413,#206414,#206415,
#206416,#206417,#206418,#206419,#206420,#206421,#206422,#206423,#206424,
#206425,#206426,#206427,#206428,#206429,#206430,#206431,#206432,#206433,
#206434,#206435,#206436,#206437,#206438,#206439,#206440,#206441,#206442,
#206443,#206444,#206445,#206446,#206447,#206448,#206449,#206450,#206451,
#206452,#206453,#206454,#206455,#206456,#206457,#206458,#206459,#206460,
#206461,#206462,#206463,#206464,#206465,#206466,#206467,#206468,#206469,
#206470,#206471,#206472,#206473,#206474,#206475,#206476,#206477,#206478,
#206479,#206480,#206481,#206482,#206483,#206484,#206485,#206486,#206487,
#206488,#206489,#206490,#206491,#206492,#206493,#206494,#206495,#206496,
#206497,#206498,#206499,#206500,#206501,#206502,#206503,#206504,#206505,
#206506,#206507,#206508,#206509,#206510,#206511,#206512,#206513,#206514,
#206515,#206516,#206517,#206518,#206519,#206520,#206521,#206522,#206523,
#206524,#206525,#206526,#206527,#206528,#206529,#206530,#206531,#206532,
#206533,#206534,#206535,#206536,#206537,#206538,#206539,#206540,#206541,
#206542,#206543,#206544,#206545,#206546,#206547,#206548,#206549,#206550,
#206551,#206552,#206553,#206554,#206555,#206556,#206557,#206558,#206559,
#206560,#206561,#206562,#206563,#206564,#206565,#206566,#206567,#206568,
#206569,#206570,#206571,#206572,#206573,#206574,#206575,#206576,#206577,
#206578,#206579,#206580,#206581,#206582,#206583,#206584,#206585,#206586,
#206587,#206588,#206589,#206590,#206591,#206592,#206593,#206594),
 .UNSPECIFIED.,.F.,.F.,(4,3,3,3,3,3,3,3,3,3,3,3,3,3,3,3,3,3,3,3,3,3,3,3,
3,3,3,3,3,3,3,3,3,3,3,3,3,3,3,3,3,3,3,3,3,3,3,3,3,3,3,3,3,3,3,3,3,3,3,3,
3,3,3,3,3,3,3,3,3,3,3,3,3,4),(65.973445725537,66.0722016376632,66.1716623230831,
66.2718883360919,66.2906114889802,66.3743502008262,66.4579857121937,66.5415381555923,
66.6250275914434,66.7084815420572,66.7919180359034,66.875355145659,66.9588109405769,
67.0423554333066,67.1259445162477,67.2096677838053,67.2903474997003,67.3740862115462,
67.4577217229137,67.5412741663122,67.6247636021632,67.7082175527769,67.7916540466231,
67.8750911563786,67.9585469512962,68.0420914440259,68.1256805269669,68.2094037945244,
68.2900835104204,68.3738222222663,68.4574577336338,68.5410101770324,68.6244996128835,
68.7079535634972,68.7913900573434,68.8748271670989,68.9582829620166,69.0418274547463,
69.1254165376873,69.2091398052449,69.2898195211405,69.3735582329864,69.4571937443539,
69.5407461877524,69.6242356236035,69.7076895742171,69.7911260680634,69.8745631778188,
69.9580189727365,70.0415634654662,70.1251525484071,70.2088758159647,70.2895555318607,
70.3732942437067,70.4569297550742,70.5404821984727,70.6239716343238,70.7074255849375,
70.7908620787838,70.8742991885393,70.957754983457,71.0412994761868,71.1248885591278,
71.2086118266854,71.2892915425808,71.3726036548392,71.4557840971122,71.5388885214543,
71.6219354908015,71.7049435228024,71.7879472022301,71.8709469547149,71.9539898147039,
72.0048655224089),.UNSPECIFIED.);
#1714=B_SPLINE_CURVE_WITH_KNOTS('',3,(#206596,#206597,#206598,#206599,#206600,
#206601,#206602,#206603,#206604,#206605),.UNSPECIFIED.,.F.,.F.,(4,1,1,1,
1,1,1,4),(65.9734457253704,66.6009021086949,67.6006381194151,68.6003741301352,
69.6001101408553,70.5998461515754,71.5995821622956,72.0060503087704),
 .UNSPECIFIED.);
#1715=B_SPLINE_CURVE_WITH_KNOTS('',3,(#206606,#206607,#206608,#206609,#206610,
#206611,#206612,#206613,#206614,#206615),.UNSPECIFIED.,.F.,.F.,(4,3,3,4),
(65.7229944280855,65.8176176411345,65.9116665109351,65.9734457253704),
 .UNSPECIFIED.);
#1716=B_SPLINE_CURVE_WITH_KNOTS('',3,(#206621,#206622,#206623,#206624,#206625,
#206626,#206627,#206628,#206629,#206630),.UNSPECIFIED.,.F.,.F.,(4,3,3,4),
(59.4398822683535,59.5326783695403,59.6250277789513,59.6902604180037),
 .UNSPECIFIED.);
#1717=B_SPLINE_CURVE_WITH_KNOTS('',3,(#206631,#206632,#206633,#206634,#206635,
#206636,#206637,#206638,#206639,#206640,#206641,#206642,#206643,#206644,
#206645,#206646,#206647,#206648,#206649,#206650,#206651,#206652,#206653,
#206654,#206655,#206656,#206657,#206658,#206659,#206660,#206661,#206662,
#206663,#206664,#206665,#206666,#206667,#206668,#206669,#206670,#206671,
#206672,#206673,#206674,#206675,#206676,#206677,#206678,#206679,#206680,
#206681,#206682,#206683,#206684,#206685,#206686,#206687,#206688,#206689,
#206690,#206691,#206692,#206693,#206694,#206695,#206696,#206697,#206698,
#206699,#206700,#206701,#206702,#206703,#206704,#206705,#206706,#206707,
#206708,#206709,#206710,#206711,#206712,#206713,#206714,#206715,#206716,
#206717,#206718,#206719,#206720,#206721,#206722,#206723,#206724,#206725,
#206726,#206727,#206728,#206729,#206730,#206731,#206732,#206733,#206734,
#206735,#206736,#206737,#206738,#206739,#206740,#206741,#206742,#206743,
#206744,#206745,#206746,#206747,#206748,#206749,#206750,#206751,#206752,
#206753,#206754,#206755,#206756,#206757,#206758,#206759,#206760,#206761,
#206762,#206763,#206764,#206765,#206766,#206767,#206768,#206769,#206770,
#206771,#206772,#206773,#206774,#206775,#206776,#206777,#206778,#206779,
#206780,#206781,#206782,#206783,#206784,#206785,#206786,#206787,#206788,
#206789,#206790,#206791,#206792,#206793,#206794,#206795,#206796,#206797,
#206798,#206799,#206800,#206801,#206802,#206803,#206804,#206805,#206806,
#206807,#206808,#206809,#206810,#206811,#206812,#206813,#206814,#206815,
#206816,#206817,#206818,#206819,#206820,#206821,#206822,#206823,#206824,
#206825,#206826,#206827,#206828,#206829,#206830,#206831,#206832,#206833,
#206834,#206835,#206836,#206837,#206838,#206839,#206840,#206841,#206842,
#206843,#206844,#206845,#206846,#206847,#206848,#206849,#206850),
 .UNSPECIFIED.,.F.,.F.,(4,3,3,3,3,3,3,3,3,3,3,3,3,3,3,3,3,3,3,3,3,3,3,3,
3,3,3,3,3,3,3,3,3,3,3,3,3,3,3,3,3,3,3,3,3,3,3,3,3,3,3,3,3,3,3,3,3,3,3,3,
3,3,3,3,3,3,3,3,3,3,3,3,3,4),(59.6902604181869,59.7747787530522,59.8593179788568,
59.9438945410883,60.0309697619811,60.1157222054673,60.2039588150634,60.2921954246594,
60.3759341365053,60.4595696478729,60.5431220912715,60.6266115271223,60.710065477736,
60.7935019715823,60.8769390813379,60.9603948762555,61.0439393689852,61.1275284519262,
61.2112517194837,61.2919314353795,61.3756701472254,61.4593056585929,61.5428581019914,
61.6263475378422,61.7098014884559,61.7932379823021,61.8766750920576,61.9601308869752,
62.0436753797049,62.1272644626459,62.2109877302035,62.2916674460996,62.3754061579455,
62.459041669313,62.5425941127115,62.6260835485626,62.7095374991762,62.7929739930223,
62.8764111027777,62.959866897695,63.0434113904248,63.1270004733656,63.2107237409232,
63.2914034568198,63.3751421686657,63.4587776800333,63.5423301234322,63.6258195592835,
63.7092735098971,63.7927100037433,63.8761471134986,63.9596029084161,64.0431474011459,
64.1267364840869,64.2104597516445,64.2911394675399,64.3748781793858,64.4585136907535,
64.5420661341521,64.625555570003,64.7090095206166,64.792446014463,64.8758831242186,
64.9593389191362,65.0428834118659,65.1264724948068,65.2101957623644,65.29087547826,
65.3743504055609,65.4613697556974,65.544635511258,65.6278429630006,65.7110052807257,
65.7224278061069),.UNSPECIFIED.);
#1718=B_SPLINE_CURVE_WITH_KNOTS('',3,(#206852,#206853,#206854,#206855,#206856,
#206857,#206858,#206859,#206860,#206861,#206862,#206863,#206864,#206865,
#206866,#206867,#206868,#206869,#206870,#206871,#206872,#206873,#206874,
#206875,#206876,#206877,#206878,#206879,#206880,#206881,#206882,#206883,
#206884,#206885,#206886,#206887,#206888,#206889,#206890,#206891,#206892,
#206893,#206894,#206895,#206896,#206897,#206898,#206899,#206900,#206901,
#206902,#206903,#206904,#206905,#206906,#206907,#206908,#206909,#206910,
#206911,#206912,#206913,#206914,#206915,#206916,#206917,#206918,#206919,
#206920,#206921,#206922,#206923,#206924,#206925,#206926,#206927,#206928,
#206929,#206930,#206931,#206932,#206933,#206934,#206935,#206936,#206937,
#206938,#206939,#206940,#206941,#206942,#206943,#206944,#206945,#206946,
#206947,#206948,#206949,#206950,#206951,#206952,#206953,#206954,#206955,
#206956,#206957,#206958,#206959,#206960,#206961,#206962,#206963,#206964,
#206965,#206966,#206967,#206968,#206969,#206970,#206971,#206972,#206973,
#206974,#206975,#206976,#206977,#206978,#206979,#206980,#206981,#206982,
#206983,#206984,#206985,#206986,#206987,#206988,#206989,#206990,#206991,
#206992,#206993,#206994,#206995,#206996,#206997,#206998,#206999,#207000,
#207001,#207002,#207003,#207004,#207005,#207006,#207007,#207008,#207009,
#207010,#207011,#207012,#207013,#207014,#207015,#207016,#207017,#207018,
#207019,#207020,#207021,#207022,#207023,#207024,#207025,#207026,#207027,
#207028,#207029,#207030,#207031,#207032,#207033,#207034,#207035,#207036,
#207037,#207038,#207039,#207040,#207041,#207042,#207043,#207044,#207045,
#207046,#207047,#207048,#207049,#207050,#207051,#207052,#207053,#207054,
#207055,#207056,#207057,#207058,#207059,#207060,#207061,#207062,#207063,
#207064,#207065,#207066,#207067,#207068,#207069,#207070,#207071),
 .UNSPECIFIED.,.F.,.F.,(4,3,3,3,3,3,3,3,3,3,3,3,3,3,3,3,3,3,3,3,3,3,3,3,
3,3,3,3,3,3,3,3,3,3,3,3,3,3,3,3,3,3,3,3,3,3,3,3,3,3,3,3,3,3,3,3,3,3,3,3,
3,3,3,3,3,3,3,3,3,3,3,3,3,4),(59.690260418325,59.7729922509435,59.8556292811794,
59.9381925013212,60.0212291942028,60.1037176127869,60.1861993999656,60.2686934103523,
60.3521415688578,60.4347588661806,60.5186224552774,60.6024860443741,60.68622475622,
60.7698602675875,60.8534127109862,60.936902146837,61.0203560974506,61.1037925912969,
61.1872297010523,61.2706854959699,61.3542299886996,61.4378190716406,61.5215423391982,
61.6022220550943,61.6859607669403,61.7695962783077,61.8531487217063,61.9366381575571,
62.0200921081707,62.1035286020169,62.1869657117725,62.2704215066901,62.3539659994198,
62.4375550823607,62.5212783499182,62.6019580658144,62.6856967776603,62.7693322890281,
62.8528847324265,62.9363741682772,63.0198281188909,63.1032646127372,63.1867017224929,
63.2701575174107,63.3537020101404,63.4372910930814,63.521014360639,63.6016940765345,
63.6854327883804,63.7690682997479,63.8526207431468,63.9361101789976,64.0195641296113,
64.1030006234575,64.1864377332125,64.2698935281301,64.3534380208598,64.4370271038007,
64.5207503713583,64.6014300872547,64.6851687991007,64.7688043104682,64.8523567538665,
64.9358461897175,65.0193001403312,65.1027366341774,65.186173743933,65.269629538851,
65.3531740315807,65.4367631145216,65.5204863820792,65.6011660979748,65.6963168570349,
65.7229944280855),.UNSPECIFIED.);
#1719=B_SPLINE_CURVE_WITH_KNOTS('',3,(#207072,#207073,#207074,#207075,#207076,
#207077,#207078,#207079,#207080,#207081),.UNSPECIFIED.,.F.,.F.,(4,3,3,4),
(59.4386194045287,59.5223427634998,59.602750033654,59.6902604181908),
 .UNSPECIFIED.);
#1720=B_SPLINE_CURVE_WITH_KNOTS('',3,(#207087,#207088,#207089,#207090,#207091,
#207092,#207093,#207094,#207095,#207096),.UNSPECIFIED.,.F.,.F.,(4,3,3,4),
(53.1554707439118,53.2392036250967,53.2940433496185,53.4070751110074),
 .UNSPECIFIED.);
#1721=B_SPLINE_CURVE_WITH_KNOTS('',3,(#207097,#207098,#207099,#207100,#207101,
#207102,#207103,#207104,#207105,#207106,#207107,#207108,#207109,#207110,
#207111,#207112,#207113,#207114,#207115,#207116,#207117,#207118,#207119,
#207120,#207121,#207122,#207123,#207124,#207125,#207126,#207127,#207128,
#207129,#207130,#207131,#207132,#207133,#207134,#207135,#207136,#207137,
#207138,#207139,#207140,#207141,#207142,#207143,#207144,#207145,#207146,
#207147,#207148,#207149,#207150,#207151,#207152,#207153,#207154,#207155,
#207156,#207157,#207158,#207159,#207160,#207161,#207162,#207163,#207164,
#207165,#207166,#207167,#207168,#207169,#207170,#207171,#207172,#207173,
#207174,#207175,#207176,#207177,#207178,#207179,#207180,#207181,#207182,
#207183,#207184,#207185,#207186,#207187,#207188,#207189,#207190,#207191,
#207192,#207193,#207194,#207195,#207196,#207197,#207198,#207199,#207200,
#207201,#207202,#207203,#207204,#207205,#207206,#207207,#207208,#207209,
#207210,#207211,#207212,#207213,#207214,#207215,#207216,#207217,#207218,
#207219,#207220,#207221,#207222,#207223,#207224,#207225,#207226,#207227,
#207228,#207229,#207230,#207231,#207232,#207233,#207234,#207235,#207236,
#207237,#207238,#207239,#207240,#207241,#207242,#207243,#207244,#207245,
#207246,#207247,#207248,#207249,#207250,#207251,#207252,#207253,#207254,
#207255,#207256,#207257,#207258,#207259,#207260,#207261,#207262,#207263,
#207264,#207265,#207266,#207267,#207268,#207269,#207270,#207271,#207272,
#207273,#207274,#207275,#207276,#207277,#207278,#207279,#207280,#207281,
#207282,#207283,#207284,#207285,#207286,#207287,#207288,#207289,#207290,
#207291,#207292,#207293,#207294,#207295,#207296,#207297,#207298,#207299,
#207300,#207301,#207302,#207303,#207304,#207305,#207306,#207307,#207308,
#207309,#207310,#207311,#207312,#207313,#207314,#207315,#207316),
 .UNSPECIFIED.,.F.,.F.,(4,3,3,3,3,3,3,3,3,3,3,3,3,3,3,3,3,3,3,3,3,3,3,3,
3,3,3,3,3,3,3,3,3,3,3,3,3,3,3,3,3,3,3,3,3,3,3,3,3,3,3,3,3,3,3,3,3,3,3,3,
3,3,3,3,3,3,3,3,3,3,3,3,3,4),(53.4070751111425,53.4896343762135,53.5721034786018,
53.6545035043015,53.7368608751334,53.819197084156,53.9015310878447,53.9838818385131,
54.066316941824,54.1487965694145,54.2314023405145,54.2937793603386,54.3775180721845,
54.4611535835521,54.5447060269508,54.6281954628017,54.7116494134154,54.7950859072616,
54.8785230170172,54.9619788119348,55.0455233046645,55.1291123876056,55.2128356551632,
55.2935153710587,55.3772540829047,55.4608895942722,55.5444420376709,55.627931473522,
55.7113854241356,55.7948219179819,55.8782590277374,55.961714822655,56.0452593153847,
56.1288483983257,56.2125716658834,56.2932513817789,56.3769900936248,56.4606256049923,
56.5441780483911,56.6276674842419,56.7111214348556,56.7945579287019,56.8779950384574,
56.9614508333752,57.0449953261048,57.1285844090459,57.2123076766035,57.292987392499,
57.376726104345,57.4603616157126,57.5439140591111,57.6274034949616,57.7108574455754,
57.7942939394216,57.8777310491771,57.9611868440946,58.0447313368243,58.1283204197652,
58.2120436873228,58.2927234032191,58.3764621150651,58.4600976264325,58.5436500698315,
58.6271395056821,58.7105934562957,58.7940299501419,58.8774670598972,58.9609228548147,
59.0444673475445,59.1280564304858,59.2117796980434,59.2924594139393,59.3857393267099,
59.4398822683535),.UNSPECIFIED.);
#1722=B_SPLINE_CURVE_WITH_KNOTS('',3,(#207318,#207319,#207320,#207321,#207322,
#207323,#207324,#207325,#207326,#207327,#207328,#207329,#207330,#207331,
#207332,#207333,#207334,#207335,#207336,#207337,#207338,#207339,#207340,
#207341,#207342,#207343,#207344,#207345,#207346,#207347,#207348,#207349,
#207350,#207351,#207352,#207353,#207354,#207355,#207356,#207357,#207358,
#207359,#207360,#207361,#207362,#207363,#207364,#207365,#207366,#207367,
#207368,#207369,#207370,#207371,#207372,#207373,#207374,#207375,#207376,
#207377,#207378,#207379,#207380,#207381,#207382,#207383,#207384,#207385,
#207386,#207387,#207388,#207389,#207390,#207391,#207392,#207393,#207394,
#207395,#207396,#207397,#207398,#207399,#207400,#207401,#207402,#207403,
#207404,#207405,#207406,#207407,#207408,#207409,#207410,#207411,#207412,
#207413,#207414,#207415,#207416,#207417,#207418,#207419,#207420,#207421,
#207422,#207423,#207424,#207425,#207426,#207427,#207428,#207429,#207430,
#207431,#207432,#207433,#207434,#207435,#207436,#207437,#207438,#207439,
#207440,#207441,#207442,#207443,#207444,#207445,#207446,#207447,#207448,
#207449,#207450,#207451,#207452,#207453,#207454,#207455,#207456,#207457,
#207458,#207459,#207460,#207461,#207462,#207463,#207464,#207465,#207466,
#207467,#207468,#207469,#207470,#207471,#207472,#207473,#207474,#207475,
#207476,#207477,#207478,#207479,#207480,#207481,#207482,#207483,#207484,
#207485,#207486,#207487,#207488,#207489,#207490,#207491,#207492,#207493,
#207494,#207495,#207496,#207497,#207498,#207499,#207500,#207501,#207502,
#207503,#207504,#207505,#207506,#207507,#207508,#207509,#207510,#207511,
#207512,#207513,#207514,#207515,#207516,#207517,#207518,#207519,#207520,
#207521,#207522,#207523,#207524,#207525,#207526,#207527,#207528,#207529,
#207530,#207531,#207532,#207533,#207534),.UNSPECIFIED.,.F.,.F.,(4,3,3,3,
3,3,3,3,3,3,3,3,3,3,3,3,3,3,3,3,3,3,3,3,3,3,3,3,3,3,3,3,3,3,3,3,3,3,3,3,
3,3,3,3,3,3,3,3,3,3,3,3,3,3,3,3,3,3,3,3,3,3,3,3,3,3,3,3,3,3,3,3,4),(53.4070751110112,
53.5281266875687,53.6043339693332,53.6880726811791,53.7717081925466,53.8552606359451,
53.9387500717959,54.0222040224095,54.1056405162557,54.1890776260112,54.2725334209287,
54.3560779136583,54.4396669965993,54.5233902641568,54.6040699800534,54.6878086918993,
54.7714442032668,54.8549966466653,54.9384860825163,55.02194003313,55.1053765269762,
55.1888136367316,55.2722694316493,55.3558139243789,55.4394030073199,55.5231262748775,
55.6038059907735,55.6875447026194,55.771180213987,55.8547326573855,55.9382220932365,
56.0216760438502,56.1051125376965,56.188549647452,56.2720054423696,56.3555499350993,
56.4391390180403,56.522862285598,56.6035420014936,56.6872807133395,56.7709162247071,
56.8544686681056,56.9379581039566,57.0214120545703,57.1048485484165,57.188285658172,
57.2717414530897,57.3552859458194,57.4388750287604,57.522598296318,57.6032780122137,
57.6870167240596,57.7706522354271,57.8542046788257,57.9376941146768,58.0211480652904,
58.1045845591367,58.1880216688921,58.2714774638097,58.3550219565394,58.4386110394804,
58.522334307038,58.6030140229339,58.6867625271259,58.7704056656083,58.8539487725955,
58.9374351492175,59.0208829145339,59.1043101578345,59.1878874695081,59.2713533662358,
59.3549863853822,59.4386194045287),.UNSPECIFIED.);
#1723=B_SPLINE_CURVE_WITH_KNOTS('',3,(#207535,#207536,#207537,#207538,#207539,
#207540,#207541,#207542,#207543,#207544),.UNSPECIFIED.,.F.,.F.,(4,3,3,4),
(53.1554762266557,53.2377493943412,53.3224122526225,53.4070751109039),
 .UNSPECIFIED.);
#1724=B_SPLINE_CURVE_WITH_KNOTS('',3,(#207550,#207551,#207552,#207553,#207554,
#207555,#207556,#207557,#207558,#207559),.UNSPECIFIED.,.F.,.F.,(4,3,3,4),
(46.872199078263,46.9544540684318,47.039171936041,47.1238898036503),
 .UNSPECIFIED.);
#1725=B_SPLINE_CURVE_WITH_KNOTS('',3,(#207560,#207561,#207562,#207563,#207564,
#207565,#207566,#207567,#207568,#207569,#207570,#207571,#207572,#207573,
#207574,#207575,#207576,#207577,#207578,#207579,#207580,#207581,#207582,
#207583,#207584,#207585,#207586,#207587,#207588,#207589,#207590,#207591,
#207592,#207593,#207594,#207595,#207596,#207597,#207598,#207599,#207600,
#207601,#207602,#207603,#207604,#207605,#207606,#207607,#207608,#207609,
#207610,#207611,#207612,#207613,#207614,#207615,#207616,#207617,#207618,
#207619,#207620,#207621,#207622,#207623,#207624,#207625,#207626,#207627,
#207628,#207629,#207630,#207631,#207632,#207633,#207634,#207635,#207636,
#207637,#207638,#207639,#207640,#207641,#207642,#207643,#207644,#207645,
#207646,#207647,#207648,#207649,#207650,#207651,#207652,#207653,#207654,
#207655,#207656,#207657,#207658,#207659,#207660,#207661,#207662,#207663,
#207664,#207665,#207666,#207667,#207668,#207669,#207670,#207671,#207672,
#207673,#207674,#207675,#207676,#207677,#207678,#207679,#207680,#207681,
#207682,#207683,#207684,#207685,#207686,#207687,#207688,#207689,#207690,
#207691,#207692,#207693,#207694,#207695,#207696,#207697,#207698,#207699,
#207700,#207701,#207702,#207703,#207704,#207705,#207706,#207707,#207708,
#207709,#207710,#207711,#207712,#207713,#207714,#207715,#207716,#207717,
#207718,#207719,#207720,#207721,#207722,#207723,#207724,#207725,#207726,
#207727,#207728,#207729,#207730,#207731,#207732,#207733,#207734,#207735,
#207736,#207737,#207738,#207739,#207740,#207741,#207742,#207743,#207744,
#207745,#207746,#207747,#207748,#207749,#207750,#207751,#207752,#207753,
#207754,#207755,#207756,#207757,#207758,#207759,#207760,#207761,#207762,
#207763,#207764,#207765,#207766,#207767,#207768,#207769,#207770,#207771,
#207772,#207773,#207774,#207775,#207776,#207777,#207778,#207779),
 .UNSPECIFIED.,.F.,.F.,(4,3,3,3,3,3,3,3,3,3,3,3,3,3,3,3,3,3,3,3,3,3,3,3,
3,3,3,3,3,3,3,3,3,3,3,3,3,3,3,3,3,3,3,3,3,3,3,3,3,3,3,3,3,3,3,3,3,3,3,3,
3,3,3,3,3,3,3,3,3,3,3,3,3,4),(47.1238898038278,47.2546038085429,47.2956272852977,
47.3793659971438,47.4630015085113,47.54655395191,47.6300433877611,47.7134973383749,
47.7969338322212,47.8803709419768,47.9638267368945,48.0473712296243,48.1309603125654,
48.2146835801231,48.2953632960178,48.3791020078637,48.4627375192312,48.5462899626297,
48.6297793984807,48.7132333490943,48.7966698429405,48.880106952696,48.9635627476137,
49.0471072403433,49.1306963232843,49.2144195908419,49.295099306738,49.3788380185839,
49.4624735299514,49.54602597335,49.6295154092011,49.7129693598147,49.796405853661,
49.8798429634164,49.9632987583341,50.0468432510638,50.1304323340048,50.2141556015624,
50.2948353174581,50.3785740293041,50.4622095406716,50.5457619840702,50.6292514199212,
50.7127053705349,50.7961418643812,50.8795789741367,50.9630347690544,51.0465792617841,
51.1301683447251,51.2138916122827,51.2945713281782,51.3783100400241,51.4619455513916,
51.5454979947902,51.6289874306412,51.7124413812548,51.795877875101,51.8793149848565,
51.9627707797741,52.0463152725038,52.1299043554448,52.2136276230024,52.2943073388984,
52.3780542392129,52.4616961110549,52.548417940162,52.6319027033865,52.7153500216485,
52.7987779830063,52.8822046585315,52.9656778285902,53.0491789172906,53.1327580827016,
53.1554707439118),.UNSPECIFIED.);
#1726=B_SPLINE_CURVE_WITH_KNOTS('',3,(#207781,#207782,#207783,#207784,#207785,
#207786,#207787,#207788,#207789,#207790,#207791,#207792,#207793,#207794,
#207795,#207796,#207797,#207798,#207799,#207800,#207801,#207802,#207803,
#207804,#207805,#207806,#207807,#207808,#207809,#207810,#207811,#207812,
#207813,#207814,#207815,#207816,#207817,#207818,#207819,#207820,#207821,
#207822,#207823,#207824,#207825,#207826,#207827,#207828,#207829,#207830,
#207831,#207832,#207833,#207834,#207835,#207836,#207837,#207838,#207839,
#207840,#207841,#207842,#207843,#207844,#207845,#207846,#207847,#207848,
#207849,#207850,#207851,#207852,#207853,#207854,#207855,#207856,#207857,
#207858,#207859,#207860,#207861,#207862,#207863,#207864,#207865,#207866,
#207867,#207868,#207869,#207870,#207871,#207872,#207873,#207874,#207875,
#207876,#207877,#207878,#207879,#207880,#207881,#207882,#207883,#207884,
#207885,#207886,#207887,#207888,#207889,#207890,#207891,#207892,#207893,
#207894,#207895,#207896,#207897,#207898,#207899,#207900,#207901,#207902,
#207903,#207904,#207905,#207906,#207907,#207908,#207909,#207910,#207911,
#207912,#207913,#207914,#207915,#207916,#207917,#207918,#207919,#207920,
#207921,#207922,#207923,#207924,#207925,#207926,#207927,#207928,#207929,
#207930,#207931,#207932,#207933,#207934,#207935,#207936,#207937,#207938,
#207939,#207940,#207941,#207942,#207943,#207944,#207945,#207946,#207947,
#207948,#207949,#207950,#207951,#207952,#207953,#207954,#207955,#207956,
#207957,#207958,#207959,#207960,#207961,#207962,#207963,#207964,#207965,
#207966,#207967,#207968,#207969,#207970,#207971,#207972,#207973,#207974,
#207975,#207976,#207977,#207978,#207979,#207980,#207981,#207982,#207983,
#207984,#207985,#207986,#207987,#207988,#207989,#207990,#207991,#207992,
#207993,#207994,#207995,#207996,#207997,#207998,#207999,#208000),
 .UNSPECIFIED.,.F.,.F.,(4,3,3,3,3,3,3,3,3,3,3,3,3,3,3,3,3,3,3,3,3,3,3,3,
3,3,3,3,3,3,3,3,3,3,3,3,3,3,3,3,3,3,3,3,3,3,3,3,3,3,3,3,3,3,3,3,3,3,3,3,
3,3,3,3,3,3,3,3,3,3,3,3,3,4),(47.123889804,47.2119695169777,47.3001901238871,
47.3886427955167,47.4772210930821,47.5660058086749,47.6059179050124,47.6896566168586,
47.7732921282264,47.8568445716251,47.9403340074762,48.0237879580902,48.1072244519367,
48.1906615616924,48.2741173566102,48.3576618493402,48.4412509322814,48.5249741998393,
48.6056539157326,48.6893926275784,48.7730281389457,48.8565805823441,48.940070018195,
49.0235239688085,49.1069604626546,49.1903975724099,49.2738533673274,49.3573978600569,
49.4409869429977,49.5247102105551,49.6053899264527,49.6891286382987,49.7727641496662,
49.8563165930648,49.9398060289159,50.0232599795296,50.1066964733759,50.1901335831314,
50.2735893780492,50.3571338707789,50.4407229537199,50.5244462212776,50.6051259371728,
50.6888646490187,50.7725001603863,50.8560526037849,50.9395420396359,51.0229959902495,
51.1064324840958,51.1898695938513,51.273325388769,51.3568698814987,51.4404589644397,
51.5241822319973,51.604861947893,51.688600659739,51.7722361711065,51.8557886145051,
51.939278050356,52.0227320009698,52.1061684948161,52.1896056045716,52.2730613994893,
52.356605892219,52.44019497516,52.5239182427177,52.6045979586131,52.6871060320478,
52.7695180670308,52.8518532668798,52.934128908709,53.0163690882775,53.0986070875677,
53.1554762266557),.UNSPECIFIED.);
#1727=B_SPLINE_CURVE_WITH_KNOTS('',3,(#208001,#208002,#208003,#208004,#208005,
#208006,#208007,#208008,#208009,#208010),.UNSPECIFIED.,.F.,.F.,(4,3,3,4),
(46.873531912371,46.960478001365,47.047291421921,47.1238898038316),
 .UNSPECIFIED.);
#1728=B_SPLINE_CURVE_WITH_KNOTS('',3,(#208016,#208017,#208018,#208019,#208020,
#208021,#208022,#208023,#208024,#208025),.UNSPECIFIED.,.F.,.F.,(4,3,3,4),
(40.5902857429648,40.6763925853647,40.7624026469278,40.8407044966482),
 .UNSPECIFIED.);
#1729=B_SPLINE_CURVE_WITH_KNOTS('',3,(#208026,#208027,#208028,#208029,#208030,
#208031,#208032,#208033,#208034,#208035,#208036,#208037,#208038,#208039,
#208040,#208041,#208042,#208043,#208044,#208045,#208046,#208047,#208048,
#208049,#208050,#208051,#208052,#208053,#208054,#208055,#208056,#208057,
#208058,#208059,#208060,#208061,#208062,#208063,#208064,#208065,#208066,
#208067,#208068,#208069,#208070,#208071,#208072,#208073,#208074,#208075,
#208076,#208077,#208078,#208079,#208080,#208081,#208082,#208083,#208084,
#208085,#208086,#208087,#208088,#208089,#208090,#208091,#208092,#208093,
#208094,#208095,#208096,#208097,#208098,#208099,#208100,#208101,#208102,
#208103,#208104,#208105,#208106,#208107,#208108,#208109,#208110,#208111,
#208112,#208113,#208114,#208115,#208116,#208117,#208118,#208119,#208120,
#208121,#208122,#208123,#208124,#208125,#208126,#208127,#208128,#208129,
#208130,#208131,#208132,#208133,#208134,#208135,#208136,#208137,#208138,
#208139,#208140,#208141,#208142,#208143,#208144,#208145,#208146,#208147,
#208148,#208149,#208150,#208151,#208152,#208153,#208154,#208155,#208156,
#208157,#208158,#208159,#208160,#208161,#208162,#208163,#208164,#208165,
#208166,#208167,#208168,#208169,#208170,#208171,#208172,#208173,#208174,
#208175,#208176,#208177,#208178,#208179,#208180,#208181,#208182,#208183,
#208184,#208185,#208186,#208187,#208188,#208189,#208190,#208191,#208192,
#208193,#208194,#208195,#208196,#208197,#208198,#208199,#208200,#208201,
#208202,#208203,#208204,#208205,#208206,#208207,#208208,#208209,#208210,
#208211,#208212,#208213,#208214,#208215,#208216,#208217,#208218,#208219,
#208220,#208221,#208222,#208223,#208224,#208225,#208226,#208227,#208228,
#208229,#208230,#208231,#208232,#208233,#208234,#208235,#208236,#208237,
#208238,#208239,#208240,#208241,#208242),.UNSPECIFIED.,.F.,.F.,(4,3,3,3,
3,3,3,3,3,3,3,3,3,3,3,3,3,3,3,3,3,3,3,3,3,3,3,3,3,3,3,3,3,3,3,3,3,3,3,3,
3,3,3,3,3,3,3,3,3,3,3,3,3,3,3,3,3,3,3,3,3,3,3,3,3,3,3,3,3,3,3,3,4),(40.8407044968307,
40.9298601171088,41.0216978930758,41.1113188688309,41.2042650449039,41.2972112209769,
41.3809499328246,41.4645854441938,41.5481378875942,41.631627323447,41.7150812740625,
41.7985177679105,41.8819548776678,41.9654106725873,42.0489551653189,42.1325442482617,
42.2162675158211,42.2969472316971,42.3806859435423,42.4643214549091,42.547873898307,
42.6313633341573,42.7148172847703,42.7982537786158,42.8816908883705,42.9651466832875,
43.0486911760164,43.1322802589567,43.2160035265135,43.2966832424172,43.380421954263,
43.4640574656304,43.5476099090288,43.6310993448798,43.7145532954933,43.7979897893395,
43.8814268990948,43.9648826940124,44.0484271867419,44.1320162696828,44.2157395372403,
44.2964192531373,44.3801579649835,44.4637934763512,44.54734591975,44.6308353556013,
44.7142893062153,44.7977258000618,44.8811629098175,44.9646187047355,45.0481631974655,
45.1317522804067,45.2154755479646,45.2961552638575,45.3798939757033,45.4635294870707,
45.5470819304692,45.6305713663201,45.7140253169337,45.7974618107799,45.8808989205352,
45.9643547154527,46.0478992081823,46.1314882911231,46.2152115586806,46.2958912745776,
46.3783624320973,46.4607382036819,46.5430378108789,46.625328127725,46.7075361957602,
46.7898676370116,46.872199078263),.UNSPECIFIED.);
#1730=B_SPLINE_CURVE_WITH_KNOTS('',3,(#208244,#208245,#208246,#208247,#208248,
#208249,#208250,#208251,#208252,#208253,#208254,#208255,#208256,#208257,
#208258,#208259,#208260,#208261,#208262,#208263,#208264,#208265,#208266,
#208267,#208268,#208269,#208270,#208271,#208272,#208273,#208274,#208275,
#208276,#208277,#208278,#208279,#208280,#208281,#208282,#208283,#208284,
#208285,#208286,#208287,#208288,#208289,#208290,#208291,#208292,#208293,
#208294,#208295,#208296,#208297,#208298,#208299,#208300,#208301,#208302,
#208303,#208304,#208305,#208306,#208307,#208308,#208309,#208310,#208311,
#208312,#208313,#208314,#208315,#208316,#208317,#208318,#208319,#208320,
#208321,#208322,#208323,#208324,#208325,#208326,#208327,#208328,#208329,
#208330,#208331,#208332,#208333,#208334,#208335,#208336,#208337,#208338,
#208339,#208340,#208341,#208342,#208343,#208344,#208345,#208346,#208347,
#208348,#208349,#208350,#208351,#208352,#208353,#208354,#208355,#208356,
#208357,#208358,#208359,#208360,#208361,#208362,#208363,#208364,#208365,
#208366,#208367,#208368,#208369,#208370,#208371,#208372,#208373,#208374,
#208375,#208376,#208377,#208378,#208379,#208380,#208381,#208382,#208383,
#208384,#208385,#208386,#208387,#208388,#208389,#208390,#208391,#208392,
#208393,#208394,#208395,#208396,#208397,#208398,#208399,#208400,#208401,
#208402,#208403,#208404,#208405,#208406,#208407,#208408,#208409,#208410,
#208411,#208412,#208413,#208414,#208415,#208416,#208417,#208418,#208419,
#208420,#208421,#208422,#208423,#208424,#208425,#208426,#208427,#208428,
#208429,#208430,#208431,#208432,#208433,#208434,#208435,#208436,#208437,
#208438,#208439,#208440,#208441,#208442,#208443,#208444,#208445,#208446,
#208447,#208448,#208449,#208450,#208451,#208452,#208453,#208454,#208455,
#208456,#208457,#208458,#208459,#208460,#208461,#208462,#208463),
 .UNSPECIFIED.,.F.,.F.,(4,3,3,3,3,3,3,3,3,3,3,3,3,3,3,3,3,3,3,3,3,3,3,3,
3,3,3,3,3,3,3,3,3,3,3,3,3,3,3,3,3,3,3,3,3,3,3,3,3,3,3,3,3,3,3,3,3,3,3,3,
3,3,3,3,3,3,3,3,3,3,3,3,3,4),(40.840704496652,40.9231791511788,41.0087194873679,
41.0911052472321,41.1734797508196,41.2558619211434,41.3382706848019,41.4207689799329,
41.5033205891009,41.5859878354084,41.6075018406916,41.6912405525498,41.7748760639297,
41.8584285073409,41.9419179432047,42.0253718938312,42.1088083876904,42.1922454974588,
42.2757012923896,42.3592457851324,42.4428348680864,42.526558135657,42.6072378514118,
42.6909765632536,42.7746120746171,42.8581645180118,42.9416539538587,43.0251079044681,
43.1085443983101,43.1919815080613,43.2754373029746,43.3589817957001,43.4425708786367,
43.5262941461901,43.6069738621319,43.6907125739767,43.774348085343,43.8579005287403,
43.9413899645904,44.0248439152029,44.1082804090481,44.1917175188026,44.2751733137188,
44.3587178064472,44.442306889387,44.5260301569433,44.606709872852,44.6904485846998,
44.7740840960691,44.8576365394695,44.9411259753222,45.0245799259379,45.1080164197859,
45.191453529543,45.2749093244626,45.3584538171943,45.4420429001373,45.5257661676968,
45.6064458835722,45.6901845954174,45.7738201067842,45.8573725501822,45.9408619860327,
46.0243159366455,46.1077524304912,46.1911895402463,46.2746453351632,46.3581898278923,
46.4417789108326,46.5255021783895,46.6061818942923,46.6935617353949,46.7835468238829,
46.873531912371),.UNSPECIFIED.);
#1731=B_SPLINE_CURVE_WITH_KNOTS('',3,(#208464,#208465,#208466,#208467,#208468,
#208469,#208470,#208471,#208472,#208473,#208474,#208475,#208476),
 .UNSPECIFIED.,.F.,.F.,(4,3,3,3,4),(40.5895313989693,40.6077658299715,40.7242351632557,
40.8344463524574,40.8407044965399),.UNSPECIFIED.);
#1732=B_SPLINE_CURVE_WITH_KNOTS('',3,(#208482,#208483,#208484,#208485,#208486,
#208487,#208488,#208489,#208490,#208491),.UNSPECIFIED.,.F.,.F.,(4,3,3,4),
(34.3065000825424,34.4146795617861,34.5207421559751,34.557519189341),
 .UNSPECIFIED.);
#1733=B_SPLINE_CURVE_WITH_KNOTS('',3,(#208492,#208493,#208494,#208495,#208496,
#208497,#208498,#208499,#208500,#208501,#208502,#208503,#208504,#208505,
#208506,#208507,#208508,#208509,#208510,#208511,#208512,#208513,#208514,
#208515,#208516,#208517,#208518,#208519,#208520,#208521,#208522,#208523,
#208524,#208525,#208526,#208527,#208528,#208529,#208530,#208531,#208532,
#208533,#208534,#208535,#208536,#208537,#208538,#208539,#208540,#208541,
#208542,#208543,#208544,#208545,#208546,#208547,#208548,#208549,#208550,
#208551,#208552,#208553,#208554,#208555,#208556,#208557,#208558,#208559,
#208560,#208561,#208562,#208563,#208564,#208565,#208566,#208567,#208568,
#208569,#208570,#208571,#208572,#208573,#208574,#208575,#208576,#208577,
#208578,#208579,#208580,#208581,#208582,#208583,#208584,#208585,#208586,
#208587,#208588,#208589,#208590,#208591,#208592,#208593,#208594,#208595,
#208596,#208597,#208598,#208599,#208600,#208601,#208602,#208603,#208604,
#208605,#208606,#208607,#208608,#208609,#208610,#208611,#208612,#208613,
#208614,#208615,#208616,#208617,#208618,#208619,#208620,#208621,#208622,
#208623,#208624,#208625,#208626,#208627,#208628,#208629,#208630,#208631,
#208632,#208633,#208634,#208635,#208636,#208637,#208638,#208639,#208640,
#208641,#208642,#208643,#208644,#208645,#208646,#208647,#208648,#208649,
#208650,#208651,#208652,#208653,#208654,#208655,#208656,#208657,#208658,
#208659,#208660,#208661,#208662,#208663,#208664,#208665,#208666,#208667,
#208668,#208669,#208670,#208671,#208672,#208673,#208674,#208675,#208676,
#208677,#208678,#208679,#208680,#208681,#208682,#208683,#208684,#208685,
#208686,#208687,#208688,#208689,#208690,#208691,#208692,#208693,#208694,
#208695,#208696,#208697,#208698,#208699,#208700,#208701,#208702,#208703,
#208704,#208705,#208706,#208707,#208708,#208709,#208710,#208711),
 .UNSPECIFIED.,.F.,.F.,(4,3,3,3,3,3,3,3,3,3,3,3,3,3,3,3,3,3,3,3,3,3,3,3,
3,3,3,3,3,3,3,3,3,3,3,3,3,3,3,3,3,3,3,3,3,3,3,3,3,3,3,3,3,3,3,3,3,3,3,3,
3,3,3,3,3,3,3,3,3,3,3,3,3,4),(34.5575191894685,34.6401346660436,34.7227049790521,
34.8052521817043,34.8877950853622,34.9703524953451,35.0529944964819,35.1356787053279,
35.2184958070966,35.2987951566562,35.3825338685851,35.4661693800365,35.5497218235198,
35.6332112594563,35.7166652101566,35.8001017040901,35.8835388139334,35.9669946089394,
36.0505391017574,36.134128184787,36.2178514524327,36.2985311673763,36.3822698791994,
36.465905390544,36.5494578339196,36.6329472697474,36.7164012203379,36.7998377141608,
36.8832748238929,36.9667306187873,37.0502751114939,37.1338641944118,37.2175874619467,
37.2982671780964,37.3820058899321,37.4656414012895,37.5491938446774,37.632683280518,
37.7161372311207,37.7995737249558,37.8830108347001,37.9664666296065,38.0500111223246,
38.1336002052539,38.2173234727998,38.2980031888166,38.3817419006748,38.4653774120547,
38.548929855466,38.6324192913301,38.7158732419566,38.7993097358158,38.8827468455844,
38.9662026405151,39.049747133258,39.133336216212,39.2170594837827,39.2977391995367,
39.3814779113784,39.4651134227418,39.5486658661357,39.6321553019831,39.7156092525924,
39.7990457464345,39.8824828561857,39.9659386510992,40.0494831438246,40.1330722267613,
40.2167954943148,40.2974752102568,40.3839889562121,40.4703860712489,40.5566452121474,
40.5902857429648),.UNSPECIFIED.);
#1734=B_SPLINE_CURVE_WITH_KNOTS('',3,(#208713,#208714,#208715,#208716,#208717,
#208718,#208719,#208720,#208721,#208722,#208723,#208724,#208725,#208726,
#208727,#208728,#208729,#208730,#208731,#208732,#208733,#208734,#208735,
#208736,#208737,#208738,#208739,#208740,#208741,#208742,#208743,#208744,
#208745,#208746,#208747,#208748,#208749,#208750,#208751,#208752,#208753,
#208754,#208755,#208756,#208757,#208758,#208759,#208760,#208761,#208762,
#208763,#208764,#208765,#208766,#208767,#208768,#208769,#208770,#208771,
#208772,#208773,#208774,#208775,#208776,#208777,#208778,#208779,#208780,
#208781,#208782,#208783,#208784,#208785,#208786,#208787,#208788,#208789,
#208790,#208791,#208792,#208793,#208794,#208795,#208796,#208797,#208798,
#208799,#208800,#208801,#208802,#208803,#208804,#208805,#208806,#208807,
#208808,#208809,#208810,#208811,#208812,#208813,#208814,#208815,#208816,
#208817,#208818,#208819,#208820,#208821,#208822,#208823,#208824,#208825,
#208826,#208827,#208828,#208829,#208830,#208831,#208832,#208833,#208834,
#208835,#208836,#208837,#208838,#208839,#208840,#208841,#208842,#208843,
#208844,#208845,#208846,#208847,#208848,#208849,#208850,#208851,#208852,
#208853,#208854,#208855,#208856,#208857,#208858,#208859,#208860,#208861,
#208862,#208863,#208864,#208865,#208866,#208867,#208868,#208869,#208870,
#208871,#208872,#208873,#208874,#208875,#208876,#208877,#208878,#208879,
#208880,#208881,#208882,#208883,#208884,#208885,#208886,#208887,#208888,
#208889,#208890,#208891,#208892,#208893,#208894,#208895,#208896,#208897,
#208898,#208899,#208900,#208901,#208902,#208903,#208904,#208905,#208906,
#208907,#208908,#208909,#208910,#208911,#208912,#208913,#208914,#208915,
#208916,#208917,#208918,#208919,#208920,#208921,#208922,#208923,#208924,
#208925,#208926,#208927,#208928,#208929,#208930,#208931,#208932),
 .UNSPECIFIED.,.F.,.F.,(4,3,3,3,3,3,3,3,3,3,3,3,3,3,3,3,3,3,3,3,3,3,3,3,
3,3,3,3,3,3,3,3,3,3,3,3,3,3,3,3,3,3,3,3,3,3,3,3,3,3,3,3,3,3,3,3,3,3,3,3,
3,3,3,3,3,3,3,3,3,3,3,3,3,4),(34.5575191894724,34.6093497656507,34.6930884767872,
34.7767239874333,34.8602764300995,34.9437658652082,35.0272198150664,35.1106563081493,
35.1940934171344,35.2775492112753,35.3610937032224,35.4446827853765,35.5284060521475,
35.6090857763709,35.6928244887674,35.776460000692,35.8600124446535,35.9435018810726,
36.0269558322605,36.1103923266845,36.1938294370208,36.2772852325218,36.3608297258354,
36.4444188093616,36.5281420775006,36.608821787091,36.6925604988207,36.7761960100715,
36.8597484533532,36.9432378890873,37.0266918395841,37.1101283333137,37.1935654429527,
37.2770212377544,37.3605657303692,37.4441548131959,37.5278780806412,37.6085577978111,
37.6922965095691,37.7759320208472,37.8594844641547,37.9429738999134,38.0264278504329,
38.1098643441839,38.1933014538431,38.2767572486637,38.3603017412953,38.4438908241376,
38.5276140915964,38.6082938085313,38.6920325204602,38.7756680319116,38.859220475395,
38.9427099113317,39.026163862032,39.1096003559656,39.1930374658088,39.2764932608146,
39.3600377536327,39.4436268366622,39.5273501043079,39.6080298192514,39.6917695595991,
39.7754058589717,39.8589588508911,39.9424485965472,40.0259016212374,40.109336849158,
40.1927723527529,40.2762262007468,40.3597640184065,40.4433462857643,40.5270516189311,
40.5895313989693),.UNSPECIFIED.);
#1735=B_SPLINE_CURVE_WITH_KNOTS('',3,(#208933,#208934,#208935,#208936,#208937,
#208938,#208939,#208940,#208941,#208942),.UNSPECIFIED.,.F.,.F.,(4,3,3,4),
(34.3057109399742,34.3886262459297,34.4730727175991,34.5575191892685),
 .UNSPECIFIED.);
#1736=B_SPLINE_CURVE_WITH_KNOTS('',3,(#208948,#208949,#208950,#208951,#208952,
#208953,#208954,#208955,#208956,#208957),.UNSPECIFIED.,.F.,.F.,(4,3,3,4),
(28.0225858316167,28.1058018123903,28.1900678472803,28.2743338821704),
 .UNSPECIFIED.);
#1737=B_SPLINE_CURVE_WITH_KNOTS('',3,(#208958,#208959,#208960,#208961,#208962,
#208963,#208964,#208965,#208966,#208967,#208968,#208969,#208970,#208971,
#208972,#208973,#208974,#208975,#208976,#208977,#208978,#208979,#208980,
#208981,#208982,#208983,#208984,#208985,#208986,#208987,#208988,#208989,
#208990,#208991,#208992,#208993,#208994,#208995,#208996,#208997,#208998,
#208999,#209000,#209001,#209002,#209003,#209004,#209005,#209006,#209007,
#209008,#209009,#209010,#209011,#209012,#209013,#209014,#209015,#209016,
#209017,#209018,#209019,#209020,#209021,#209022,#209023,#209024,#209025,
#209026,#209027,#209028,#209029,#209030,#209031,#209032,#209033,#209034,
#209035,#209036,#209037,#209038,#209039,#209040,#209041,#209042,#209043,
#209044,#209045,#209046,#209047,#209048,#209049,#209050,#209051,#209052,
#209053,#209054,#209055,#209056,#209057,#209058,#209059,#209060,#209061,
#209062,#209063,#209064,#209065,#209066,#209067,#209068,#209069,#209070,
#209071,#209072,#209073,#209074,#209075,#209076,#209077,#209078,#209079,
#209080,#209081,#209082,#209083,#209084,#209085,#209086,#209087,#209088,
#209089,#209090,#209091,#209092,#209093,#209094,#209095,#209096,#209097,
#209098,#209099,#209100,#209101,#209102,#209103,#209104,#209105,#209106,
#209107,#209108,#209109,#209110,#209111,#209112,#209113,#209114,#209115,
#209116,#209117,#209118,#209119,#209120,#209121,#209122,#209123,#209124,
#209125,#209126,#209127,#209128,#209129,#209130,#209131,#209132,#209133,
#209134,#209135,#209136,#209137,#209138,#209139,#209140,#209141,#209142,
#209143,#209144,#209145,#209146,#209147,#209148,#209149,#209150,#209151,
#209152,#209153,#209154,#209155,#209156,#209157,#209158,#209159,#209160,
#209161,#209162,#209163,#209164,#209165,#209166,#209167,#209168,#209169,
#209170,#209171,#209172,#209173,#209174,#209175,#209176,#209177,#209178,
#209179,#209180),.UNSPECIFIED.,.F.,.F.,(4,3,3,3,3,3,3,3,3,3,3,3,3,3,3,3,
3,3,3,3,3,3,3,3,3,3,3,3,3,3,3,3,3,3,3,3,3,3,3,3,3,3,3,3,3,3,3,3,3,3,3,3,
3,3,3,3,3,3,3,3,3,3,3,3,3,3,3,3,3,3,3,3,3,3,4),(28.2743338822889,28.3006430816153,
28.3843817879882,28.468017293797,28.5515697315575,28.6350591616976,28.7185131065089,
28.8019495944981,28.8853866983471,28.9688424873144,29.0523869740573,29.1359760509821,
29.2196993125341,29.3003790923354,29.3841178077619,29.4677533227502,29.5513057698054,
29.6347952093454,29.7182491636837,29.801685661276,29.8851227747951,29.9685785734908,
30.0521230699997,30.1357121567266,30.2194354280432,30.3001151030555,30.3838538143865,
30.4674893252401,30.5510417681263,30.6345312034672,30.7179851535757,30.80142164692,
30.8848587561773,30.9683145506009,31.051859042846,31.1354481253068,31.2191713923966,
31.2998511137757,31.3835898249122,31.4672253355584,31.5507777782246,31.6342672133331,
31.7177211631913,31.8011576562743,31.8845947652594,31.9680505594003,32.0515950513474,
32.1351841335015,32.2189074002725,32.2995871244958,32.3833258368923,32.466961348817,
32.5505137927785,32.6340032291978,32.7174571803857,32.8008936748098,32.884330785146,
32.967786580647,33.0513310739606,33.1349201574868,33.2186434256259,33.2993231352159,
33.3830618469456,33.4666973581966,33.5502498014783,33.6337392372124,33.7171931877092,
33.8006296814388,33.8840667910778,33.9675225858795,34.0510670784944,34.1346561613211,
34.2183794287664,34.299059145936,34.3065000825424),.UNSPECIFIED.);
#1738=B_SPLINE_CURVE_WITH_KNOTS('',3,(#209182,#209183,#209184,#209185,#209186,
#209187,#209188,#209189,#209190,#209191,#209192,#209193,#209194,#209195,
#209196,#209197,#209198,#209199,#209200,#209201,#209202,#209203,#209204,
#209205,#209206,#209207,#209208,#209209,#209210,#209211,#209212,#209213,
#209214,#209215,#209216,#209217,#209218,#209219,#209220,#209221,#209222,
#209223,#209224,#209225,#209226,#209227,#209228,#209229,#209230,#209231,
#209232,#209233,#209234,#209235,#209236,#209237,#209238,#209239,#209240,
#209241,#209242,#209243,#209244,#209245,#209246,#209247,#209248,#209249,
#209250,#209251,#209252,#209253,#209254,#209255,#209256,#209257,#209258,
#209259,#209260,#209261,#209262,#209263,#209264,#209265,#209266,#209267,
#209268,#209269,#209270,#209271,#209272,#209273,#209274,#209275,#209276,
#209277,#209278,#209279,#209280,#209281,#209282,#209283,#209284,#209285,
#209286,#209287,#209288,#209289,#209290,#209291,#209292,#209293,#209294,
#209295,#209296,#209297,#209298,#209299,#209300,#209301,#209302,#209303,
#209304,#209305,#209306,#209307,#209308,#209309,#209310,#209311,#209312,
#209313,#209314,#209315,#209316,#209317,#209318,#209319,#209320,#209321,
#209322,#209323,#209324,#209325,#209326,#209327,#209328,#209329,#209330,
#209331,#209332,#209333,#209334,#209335,#209336,#209337,#209338,#209339,
#209340,#209341,#209342,#209343,#209344,#209345,#209346,#209347,#209348,
#209349,#209350,#209351,#209352,#209353,#209354,#209355,#209356,#209357,
#209358,#209359,#209360,#209361,#209362,#209363,#209364,#209365,#209366,
#209367,#209368,#209369,#209370,#209371,#209372,#209373,#209374,#209375,
#209376,#209377,#209378,#209379,#209380,#209381,#209382,#209383,#209384,
#209385,#209386,#209387,#209388,#209389,#209390,#209391,#209392,#209393,
#209394,#209395,#209396,#209397,#209398,#209399,#209400,#209401),
 .UNSPECIFIED.,.F.,.F.,(4,3,3,3,3,3,3,3,3,3,3,3,3,3,3,3,3,3,3,3,3,3,3,3,
3,3,3,3,3,3,3,3,3,3,3,3,3,3,3,3,3,3,3,3,3,3,3,3,3,3,3,3,3,3,3,3,3,3,3,3,
3,3,3,3,3,3,3,3,3,3,3,3,3,4),(28.2743338824827,28.3712824055307,28.4687879362423,
28.5669577034657,28.6109337013299,28.6946723723872,28.7783078423616,28.8618602438099,
28.9453496371999,29.0288035447238,29.1122399951033,29.1956770610554,29.2791328118729,
29.3626772602797,29.4462662987062,29.5299895218703,29.6106697120501,29.6944084466627,
29.7780439810379,29.8615964476591,29.9450859069223,30.0285398811537,30.1119763987395,
30.1954135323339,30.2788693511678,30.362413867801,30.4460029746765,30.5297262659791,
30.6104057227702,30.694144433022,30.777779942827,30.8613323846962,30.9448218190526,
31.0282757682304,31.1117122606767,31.1951493690697,31.2786051626639,31.3621496541399,
31.4457387358632,31.5294620022777,31.6101417334903,31.6938804398633,31.7775159456722,
31.8610683834328,31.9445578135729,32.0280117583843,32.1114482463736,32.1948853502228,
32.2783411391901,32.3618856259331,32.4454747028581,32.5291979644102,32.6098777442105,
32.693616459637,32.7772519746252,32.8608044216806,32.9442938612206,33.0277478155589,
33.1111843131511,33.1946214266703,33.2780772253658,33.3616217218747,33.4452108086016,
33.5289340799181,33.6096137549306,33.696625903061,33.7795858721787,33.8624709514653,
33.9452998737482,34.0280913257695,34.1108784301918,34.1936633276373,34.2764866832596,
34.3057109399742),.UNSPECIFIED.);
#1739=B_SPLINE_CURVE_WITH_KNOTS('',3,(#209402,#209403,#209404,#209405,#209406,
#209407,#209408,#209409,#209410,#209411),.UNSPECIFIED.,.F.,.F.,(4,3,3,4),
(28.0234162092491,28.1068355155373,28.190584698915,28.2743338822928),
 .UNSPECIFIED.);
#1740=B_SPLINE_CURVE_WITH_KNOTS('',3,(#209417,#209418,#209419,#209420,#209421,
#209422,#209423,#209424,#209425,#209426,#209427,#209428,#209429,#209430,
#209431,#209432,#209433,#209434,#209435,#209436,#209437,#209438,#209439,
#209440,#209441,#209442,#209443,#209444,#209445,#209446,#209447),
 .UNSPECIFIED.,.F.,.F.,(4,3,3,3,3,3,3,3,3,3,4),(20.99221161231,21.0756590159651,
21.1590986605133,21.2425486105237,21.3260269334585,21.4095983367567,21.4932230327364,
21.5769691760559,21.612781626289,21.7074539497444,21.740715980233),
 .UNSPECIFIED.);
#1741=B_SPLINE_CURVE_WITH_KNOTS('',3,(#209449,#209450,#209451,#209452,#209453,
#209454),.UNSPECIFIED.,.F.,.F.,(4,2,4),(0.0691804534626763,0.186754252104775,
0.270033766278533),.UNSPECIFIED.);
#1742=B_SPLINE_CURVE_WITH_KNOTS('',3,(#209455,#209456,#209457,#209458,#209459,
#209460,#209461,#209462,#209463,#209464,#209465,#209466,#209467,#209468,
#209469,#209470,#209471,#209472,#209473,#209474,#209475,#209476,#209477,
#209478,#209479,#209480,#209481,#209482,#209483,#209484,#209485,#209486,
#209487,#209488,#209489,#209490,#209491,#209492,#209493,#209494,#209495,
#209496,#209497,#209498,#209499,#209500),.UNSPECIFIED.,.F.,.F.,(4,3,3,3,
3,3,3,3,3,3,3,3,3,3,3,4),(20.5644249259299,20.6479085815111,20.731360149683,
20.8147965890331,20.8982359703094,20.9816963623492,21.0652465555357,21.1488434281147,
21.2325713349974,21.3024910065744,21.3858830961901,21.4691722628339,21.5523598572504,
21.6354890394005,21.718573857478,21.7400988072349),.UNSPECIFIED.);
#1743=B_SPLINE_CURVE_WITH_KNOTS('',3,(#216282,#216283,#216284,#216285,#216286,
#216287,#216288,#216289,#216290,#216291),.UNSPECIFIED.,.F.,.F.,(4,2,2,2,
4),(0.000592050309002955,0.00995120211491283,0.0520685380789643,0.0963518572333416,
0.180104991815336),.UNSPECIFIED.);
#1744=B_SPLINE_CURVE_WITH_KNOTS('',3,(#216293,#216294,#216295,#216296,#216297,
#216298,#216299,#216300,#216301),.UNSPECIFIED.,.F.,.F.,(4,1,1,1,1,1,4),
(-115.221526233207,-114.969641232815,-113.969905222095,-112.970169211375,
-111.970433200655,-110.970697189935,-110.906691970895),.UNSPECIFIED.);
#1745=B_SPLINE_CURVE_WITH_KNOTS('',3,(#216303,#216304,#216305,#216306,#216307,
#216308,#216309,#216310,#216311,#216312,#216313,#216314,#216315,#216316,
#216317,#216318,#216319,#216320,#216321,#216322,#216323,#216324,#216325,
#216326,#216327,#216328,#216329,#216330,#216331,#216332,#216333,#216334,
#216335,#216336,#216337,#216338,#216339,#216340,#216341,#216342,#216343,
#216344,#216345,#216346,#216347,#216348,#216349,#216350,#216351,#216352,
#216353,#216354,#216355,#216356,#216357,#216358,#216359,#216360,#216361,
#216362,#216363,#216364,#216365,#216366,#216367,#216368,#216369,#216370,
#216371,#216372,#216373,#216374,#216375,#216376,#216377,#216378,#216379,
#216380,#216381,#216382,#216383,#216384,#216385,#216386,#216387,#216388,
#216389,#216390,#216391,#216392,#216393,#216394,#216395,#216396,#216397,
#216398,#216399,#216400,#216401,#216402,#216403,#216404,#216405,#216406,
#216407,#216408,#216409,#216410,#216411,#216412,#216413,#216414,#216415,
#216416,#216417,#216418,#216419,#216420,#216421,#216422,#216423,#216424,
#216425,#216426,#216427,#216428,#216429,#216430,#216431,#216432,#216433,
#216434,#216435,#216436,#216437,#216438,#216439,#216440,#216441,#216442,
#216443,#216444,#216445,#216446,#216447,#216448,#216449,#216450,#216451,
#216452,#216453,#216454,#216455,#216456,#216457,#216458,#216459,#216460,
#216461,#216462,#216463,#216464,#216465,#216466,#216467,#216468,#216469,
#216470,#216471,#216472,#216473,#216474,#216475,#216476,#216477,#216478,
#216479,#216480,#216481,#216482,#216483,#216484,#216485,#216486,#216487,
#216488,#216489,#216490,#216491,#216492,#216493,#216494,#216495,#216496,
#216497,#216498,#216499,#216500,#216501,#216502,#216503,#216504,#216505,
#216506,#216507,#216508,#216509,#216510,#216511,#216512,#216513,#216514,
#216515,#216516,#216517,#216518,#216519,#216520,#216521,#216522,#216523,
#216524,#216525,#216526,#216527,#216528,#216529,#216530,#216531,#216532,
#216533,#216534,#216535,#216536,#216537,#216538,#216539,#216540,#216541,
#216542,#216543,#216544,#216545,#216546),.UNSPECIFIED.,.F.,.F.,(4,3,3,3,
3,3,3,3,3,3,3,3,3,3,3,3,3,3,3,3,3,3,3,3,3,3,3,3,3,3,3,3,3,3,3,3,3,3,3,3,
3,3,3,3,3,3,3,3,3,3,3,3,3,3,3,3,3,3,3,3,3,3,3,3,3,3,3,3,3,3,3,3,3,3,3,3,
3,3,3,3,3,4),(-110.906691970895,-110.82749856315,-110.748395230993,-110.669363816888,
-110.590386228964,-110.511436604536,-110.432499965624,-110.35356001131,
-110.27460044075,-110.195558870897,-110.116474582147,-110.037271099244,
-109.970961179214,-109.891003879083,-109.81114108184,-109.731355259369,
-109.651628944173,-109.571944715879,-109.492273729658,-109.412606276133,
-109.332926625316,-109.253219042922,-109.173423813846,-109.093579472138,
-109.013621045091,-108.971225168494,-108.891267868363,-108.81140507112,
-108.731619248648,-108.651892933453,-108.572208705159,-108.492537718938,
-108.412870265412,-108.333190614595,-108.253483032201,-108.173687803125,
-108.093843461418,-108.013885034371,-107.971489157774,-107.891531857643,
-107.8116690604,-107.731883237929,-107.652156922733,-107.572472694439,-107.492801708218,
-107.413134254692,-107.333454603876,-107.253747021481,-107.173951792405,
-107.094107450698,-107.01414902365,-106.971753147054,-106.891795846923,
-106.81193304968,-106.732147227209,-106.652420912013,-106.572736683719,
-106.493065697498,-106.413398243972,-106.333718593156,-106.254011010761,
-106.174215781686,-106.094371439978,-106.014413012931,-105.972017136334,
-105.892059836203,-105.81219703896,-105.732411216489,-105.652684901294,
-105.573000672999,-105.493329686778,-105.413662233252,-105.333982582435,
-105.254275000041,-105.174479770965,-105.094635429257,-105.01467700221,
-104.972281125614,-104.879689190256,-104.787448241979,-104.695893518158,
-104.623506786484),.UNSPECIFIED.);
#1746=B_SPLINE_CURVE_WITH_KNOTS('',3,(#216548,#216549,#216550,#216551,#216552,
#216553,#216554,#216555,#216556,#216557),.UNSPECIFIED.,.F.,.F.,(4,1,1,1,
1,1,1,4),(-104.623506663716,-103.972545114894,-102.972809104174,-101.973073093453,
-100.973337082733,-99.9736010720131,-98.973865061293,-98.340321356536),
 .UNSPECIFIED.);
#1747=B_SPLINE_CURVE_WITH_KNOTS('',3,(#216559,#216560,#216561,#216562,#216563,
#216564,#216565,#216566,#216567,#216568),.UNSPECIFIED.,.F.,.F.,(4,1,1,1,
1,1,1,4),(-98.340321356536,-97.9741290505729,-96.9743930398527,-95.9746570291326,
-94.9749210184124,-93.9751850076923,-92.9754489969722,-92.0571360493564),
 .UNSPECIFIED.);
#1748=B_SPLINE_CURVE_WITH_KNOTS('',3,(#216570,#216571,#216572,#216573,#216574,
#216575,#216576,#216577,#216578,#216579,#216580),.UNSPECIFIED.,.F.,.F.,
(4,1,1,1,1,1,1,1,4),(-92.0571360493564,-91.9757129862521,-90.9759769755319,
-89.9762409648118,-88.9765049540917,-87.9767689433716,-86.9770329326514,
-85.9772969219313,-85.7739507421768),.UNSPECIFIED.);
#1749=B_SPLINE_CURVE_WITH_KNOTS('',3,(#216582,#216583,#216584,#216585,#216586,
#216587,#216588,#216589,#216590,#216591,#216592,#216593,#216594,#216595,
#216596,#216597,#216598,#216599,#216600,#216601,#216602,#216603,#216604,
#216605,#216606,#216607,#216608,#216609,#216610,#216611,#216612,#216613,
#216614,#216615,#216616,#216617,#216618,#216619,#216620,#216621,#216622,
#216623,#216624,#216625,#216626,#216627,#216628,#216629,#216630,#216631,
#216632,#216633,#216634,#216635,#216636,#216637,#216638,#216639,#216640,
#216641,#216642,#216643,#216644,#216645,#216646,#216647,#216648,#216649,
#216650,#216651,#216652,#216653,#216654,#216655,#216656,#216657,#216658,
#216659,#216660,#216661,#216662,#216663,#216664,#216665,#216666,#216667,
#216668,#216669,#216670,#216671,#216672,#216673,#216674,#216675,#216676,
#216677,#216678,#216679,#216680,#216681,#216682,#216683,#216684,#216685,
#216686,#216687,#216688,#216689,#216690,#216691,#216692,#216693,#216694,
#216695,#216696,#216697,#216698,#216699,#216700,#216701,#216702,#216703,
#216704,#216705,#216706,#216707,#216708,#216709,#216710,#216711,#216712,
#216713,#216714,#216715,#216716,#216717,#216718,#216719,#216720,#216721,
#216722,#216723,#216724,#216725,#216726,#216727,#216728,#216729,#216730,
#216731,#216732,#216733,#216734,#216735,#216736,#216737,#216738,#216739,
#216740,#216741,#216742,#216743,#216744,#216745,#216746,#216747,#216748,
#216749,#216750,#216751,#216752,#216753,#216754,#216755,#216756,#216757,
#216758,#216759,#216760,#216761,#216762,#216763,#216764,#216765,#216766,
#216767,#216768,#216769,#216770,#216771,#216772,#216773,#216774,#216775,
#216776,#216777,#216778,#216779,#216780,#216781,#216782,#216783,#216784,
#216785,#216786,#216787,#216788,#216789,#216790,#216791,#216792,#216793,
#216794,#216795,#216796,#216797,#216798,#216799,#216800,#216801,#216802,
#216803,#216804,#216805,#216806,#216807,#216808,#216809,#216810,#216811,
#216812,#216813,#216814,#216815,#216816,#216817,#216818,#216819,#216820,
#216821,#216822,#216823,#216824,#216825),.UNSPECIFIED.,.F.,.F.,(4,3,3,3,
3,3,3,3,3,3,3,3,3,3,3,3,3,3,3,3,3,3,3,3,3,3,3,3,3,3,3,3,3,3,3,3,3,3,3,3,
3,3,3,3,3,3,3,3,3,3,3,3,3,3,3,3,3,3,3,3,3,3,3,3,3,3,3,3,3,3,3,3,3,3,3,3,
3,3,3,3,3,4),(-85.7739507421768,-85.6952881601577,-85.616687997987,-85.53679711214,
-85.4582566003864,-85.379719530466,-85.3011693595009,-85.2202672474284,
-85.1416009943376,-85.0595809527744,-84.9775609112112,-84.89760361108,-84.8177408138373,
-84.7379549913655,-84.6582286761703,-84.5785444478759,-84.498873461655,
-84.419206008129,-84.3395263573124,-84.2598187749181,-84.1800235458425,
-84.1001792041348,-84.0202207770874,-83.977824900491,-83.8978676003597,
-83.8180048031171,-83.7382189806452,-83.6584926654501,-83.5788084371562,
-83.4991374509353,-83.4194699974093,-83.3397903465929,-83.2600827641988,
-83.1802875351232,-83.1004431934156,-83.0204847663682,-82.9780888897709,
-82.8981315896397,-82.8182687923971,-82.7384829699253,-82.65875665473,-82.579072426436,
-82.4994014402152,-82.4197339866892,-82.3400543358726,-82.2603467534779,
-82.1805515244024,-82.1007071826946,-82.0207487556472,-81.9783528790508,
-81.8983955789195,-81.818532781677,-81.7387469592052,-81.65902064401,-81.5793364157154,
-81.4996654294946,-81.4199979759686,-81.3403183251522,-81.2606107427579,
-81.1808155136824,-81.100971171975,-81.0210127449277,-80.9786168683306,
-80.8986595681993,-80.818796770957,-80.7390109484849,-80.6592846332902,
-80.5796004049962,-80.4999294187752,-80.4202619652489,-80.3405823144325,
-80.2608747320383,-80.1810795029628,-80.1012351612554,-80.0212767342081,
-79.9788808576105,-79.894345483959,-79.8099558941397,-79.7257670174106,
-79.6416970903594,-79.5577926852418,-79.4907654351257),.UNSPECIFIED.);
#1750=B_SPLINE_CURVE_WITH_KNOTS('',3,(#216827,#216828,#216829,#216830,#216831,
#216832,#216833,#216834,#216835,#216836,#216837,#216838,#216839,#216840,
#216841,#216842,#216843,#216844,#216845,#216846,#216847,#216848,#216849,
#216850,#216851,#216852,#216853,#216854,#216855,#216856,#216857,#216858,
#216859,#216860,#216861,#216862,#216863,#216864,#216865,#216866,#216867,
#216868,#216869,#216870,#216871,#216872,#216873,#216874,#216875,#216876,
#216877,#216878,#216879,#216880,#216881,#216882,#216883,#216884,#216885,
#216886,#216887,#216888,#216889,#216890,#216891,#216892,#216893,#216894,
#216895,#216896,#216897,#216898,#216899,#216900,#216901,#216902,#216903,
#216904,#216905,#216906,#216907,#216908,#216909,#216910,#216911,#216912,
#216913,#216914,#216915,#216916,#216917,#216918,#216919,#216920,#216921,
#216922,#216923,#216924,#216925,#216926,#216927,#216928,#216929,#216930,
#216931,#216932,#216933,#216934,#216935,#216936,#216937,#216938,#216939,
#216940,#216941,#216942,#216943,#216944,#216945,#216946,#216947,#216948,
#216949,#216950,#216951,#216952,#216953,#216954,#216955,#216956,#216957,
#216958,#216959,#216960,#216961,#216962,#216963,#216964,#216965,#216966,
#216967,#216968,#216969,#216970,#216971,#216972,#216973,#216974,#216975,
#216976,#216977,#216978,#216979,#216980,#216981,#216982,#216983,#216984,
#216985,#216986,#216987,#216988,#216989,#216990,#216991,#216992,#216993,
#216994,#216995,#216996,#216997,#216998,#216999,#217000,#217001,#217002,
#217003,#217004,#217005,#217006,#217007,#217008,#217009,#217010,#217011,
#217012,#217013,#217014,#217015,#217016,#217017,#217018,#217019,#217020,
#217021,#217022,#217023,#217024,#217025,#217026,#217027,#217028,#217029,
#217030,#217031,#217032,#217033,#217034,#217035,#217036,#217037,#217038,
#217039,#217040,#217041,#217042,#217043,#217044,#217045,#217046,#217047,
#217048,#217049,#217050,#217051,#217052,#217053,#217054,#217055,#217056,
#217057,#217058,#217059,#217060,#217061,#217062,#217063,#217064,#217065,
#217066,#217067,#217068,#217069,#217070),.UNSPECIFIED.,.F.,.F.,(4,3,3,3,
3,3,3,3,3,3,3,3,3,3,3,3,3,3,3,3,3,3,3,3,3,3,3,3,3,3,3,3,3,3,3,3,3,3,3,3,
3,3,3,3,3,3,3,3,3,3,3,3,3,3,3,3,3,3,3,3,3,3,3,3,3,3,3,3,3,3,3,3,3,3,3,3,
3,3,3,3,3,4),(-79.4907654349973,-79.4077034724819,-79.3245504349086,-79.2381990379041,
-79.1547733841094,-79.0669591154998,-78.9791448468903,-78.8991875467591,
-78.8193247495167,-78.7395389270448,-78.6598126118496,-78.5801283835557,
-78.5004573973348,-78.4207899438089,-78.3411102929926,-78.2614027105983,
-78.1816074815228,-78.101763139815,-78.0218047127677,-77.9794088361702,
-77.8994515360389,-77.8195887387963,-77.7398029163244,-77.6600766011291,
-77.5803923728351,-77.5007213866142,-77.4210539330884,-77.3413742822718,
-77.2616666998774,-77.1818714708018,-77.1020271290941,-77.0220687020468,
-76.9796728254501,-76.8997155253188,-76.819852728076,-76.7400669056043,
-76.6603405904092,-76.5806563621158,-76.5009853758948,-76.4213179223689,
-76.3416382715525,-76.2619306891576,-76.182135460082,-76.1022911183746,
-76.0223326913272,-75.97993681473,-75.8999795145987,-75.820116717356,-75.7403308948843,
-75.6606045796891,-75.5809203513952,-75.5012493651742,-75.4215819116484,
-75.3419022608322,-75.2621946784377,-75.1823994493621,-75.1025551076547,
-75.0225966806073,-74.9802008040098,-74.9002435038785,-74.8203807066359,
-74.7405948841641,-74.6608685689692,-74.5811843406744,-74.5015133544535,
-74.4218459009276,-74.3421662501111,-74.2624586677158,-74.1826634386403,
-74.1028190969327,-74.0228606698853,-73.9804647932897,-73.9015581804217,
-73.8227469663865,-73.7440261147531,-73.6653563569114,-73.5867211558266,
-73.5081040028306,-73.4294628808362,-73.3508110774882,-73.2720919472877,
-73.2075801278176),.UNSPECIFIED.);
#1751=B_SPLINE_CURVE_WITH_KNOTS('',3,(#217072,#217073,#217074,#217075,#217076,
#217077,#217078,#217079,#217080,#217081,#217082),.UNSPECIFIED.,.F.,.F.,
(4,1,1,1,1,1,1,1,4),(-73.2075801278176,-72.9807287825696,-71.9809927718494,
-70.9812567611293,-69.9815207504092,-68.981784739689,-67.9820487289689,
-66.9823127182488,-66.9243948206381),.UNSPECIFIED.);
#1752=B_SPLINE_CURVE_WITH_KNOTS('',3,(#217084,#217085,#217086,#217087,#217088,
#217089,#217090,#217091,#217092,#217093,#217094,#217095,#217096,#217097,
#217098,#217099,#217100,#217101,#217102,#217103,#217104,#217105,#217106,
#217107,#217108,#217109,#217110,#217111,#217112,#217113,#217114,#217115,
#217116,#217117,#217118,#217119,#217120,#217121,#217122,#217123,#217124,
#217125,#217126,#217127,#217128,#217129,#217130,#217131,#217132,#217133,
#217134,#217135,#217136,#217137,#217138,#217139,#217140,#217141,#217142,
#217143,#217144,#217145,#217146,#217147,#217148,#217149,#217150,#217151,
#217152,#217153,#217154,#217155,#217156,#217157,#217158,#217159,#217160,
#217161,#217162,#217163,#217164,#217165,#217166,#217167,#217168,#217169,
#217170,#217171,#217172,#217173,#217174,#217175,#217176,#217177,#217178,
#217179,#217180,#217181,#217182,#217183,#217184,#217185,#217186,#217187,
#217188,#217189,#217190,#217191,#217192,#217193,#217194,#217195,#217196,
#217197,#217198,#217199,#217200,#217201,#217202,#217203,#217204,#217205,
#217206,#217207,#217208,#217209,#217210,#217211,#217212,#217213,#217214,
#217215,#217216,#217217,#217218,#217219,#217220,#217221,#217222,#217223,
#217224,#217225,#217226,#217227,#217228,#217229,#217230,#217231,#217232,
#217233,#217234,#217235,#217236,#217237,#217238,#217239,#217240,#217241,
#217242,#217243,#217244,#217245,#217246,#217247,#217248,#217249,#217250,
#217251,#217252,#217253,#217254,#217255,#217256,#217257,#217258,#217259,
#217260,#217261,#217262,#217263,#217264,#217265,#217266,#217267,#217268,
#217269,#217270,#217271,#217272,#217273,#217274,#217275,#217276,#217277,
#217278,#217279,#217280,#217281,#217282,#217283,#217284,#217285,#217286,
#217287,#217288,#217289,#217290,#217291,#217292,#217293,#217294,#217295,
#217296,#217297,#217298,#217299,#217300,#217301,#217302,#217303,#217304,
#217305,#217306,#217307,#217308,#217309,#217310,#217311,#217312,#217313,
#217314,#217315,#217316,#217317,#217318,#217319,#217320,#217321,#217322,
#217323,#217324,#217325,#217326,#217327),.UNSPECIFIED.,.F.,.F.,(4,3,3,3,
3,3,3,3,3,3,3,3,3,3,3,3,3,3,3,3,3,3,3,3,3,3,3,3,3,3,3,3,3,3,3,3,3,3,3,3,
3,3,3,3,3,3,3,3,3,3,3,3,3,3,3,3,3,3,3,3,3,3,3,3,3,3,3,3,3,3,3,3,3,3,3,3,
3,3,3,3,3,4),(-66.9243948206381,-66.8451430614651,-66.7659820906656,-66.68689378965,
-66.6078601052444,-66.5288554488661,-66.4498645624908,-66.3708711811437,
-66.2918590405673,-66.2127651323194,-66.1336293443134,-66.054372687672,
-65.9825767075287,-65.9026194073974,-65.8227566101546,-65.7429707876828,
-65.6632444724872,-65.5835602441933,-65.5038892579723,-65.4242218044462,
-65.3445421536298,-65.2648345712352,-65.1850393421596,-65.105195000452,
-65.0252365734045,-64.9828406968085,-64.9028833966772,-64.8230205994346,
-64.7432347769627,-64.6635084617673,-64.5838242334732,-64.5041532472523,
-64.4244857937264,-64.3448061429098,-64.2650985605154,-64.1853033314399,
-64.1054589897322,-64.0255005626848,-63.9831046860884,-63.9031473859572,
-63.8232845887147,-63.7434987662427,-63.6637724510475,-63.5840882227535,
-63.5044172365327,-63.4247497830068,-63.3450701321903,-63.2653625497957,
-63.1855673207202,-63.1057229790125,-63.0257645519651,-62.9833686753683,
-62.903411375237,-62.8235485779942,-62.7437627555225,-62.6640364403274,
-62.5843522120328,-62.5046812258119,-62.425013772286,-62.3453341214695,
-62.2656265390753,-62.1858313099998,-62.1059869682922,-62.0260285412449,
-61.9836326646481,-61.9036753645168,-61.823812567274,-61.7440267448023,
-61.6643004296077,-61.5846162013138,-61.5049452150927,-61.4252777615666,
-61.3455981107502,-61.2658905283563,-61.1860952992806,-61.1062509575726,
-61.0262925305251,-60.983896653928,-60.8907777178953,-60.798032881653,-60.7060135811139,
-60.6412095135729),.UNSPECIFIED.);
#1753=B_SPLINE_CURVE_WITH_KNOTS('',3,(#217329,#217330,#217331,#217332,#217333,
#217334,#217335,#217336,#217337,#217338,#217339,#217340,#217341,#217342,
#217343,#217344,#217345,#217346,#217347,#217348,#217349,#217350,#217351,
#217352,#217353,#217354,#217355,#217356,#217357,#217358,#217359,#217360,
#217361,#217362,#217363,#217364,#217365,#217366,#217367,#217368,#217369,
#217370,#217371,#217372,#217373,#217374,#217375,#217376,#217377,#217378,
#217379,#217380,#217381,#217382,#217383,#217384,#217385,#217386,#217387,
#217388,#217389,#217390,#217391,#217392,#217393,#217394,#217395,#217396,
#217397,#217398,#217399,#217400,#217401,#217402,#217403,#217404,#217405,
#217406,#217407,#217408,#217409,#217410,#217411,#217412,#217413,#217414,
#217415,#217416,#217417,#217418,#217419,#217420,#217421,#217422,#217423,
#217424,#217425,#217426,#217427,#217428,#217429,#217430,#217431,#217432,
#217433,#217434,#217435,#217436,#217437,#217438,#217439,#217440,#217441,
#217442,#217443,#217444,#217445,#217446,#217447,#217448,#217449,#217450,
#217451,#217452,#217453,#217454,#217455,#217456,#217457,#217458,#217459,
#217460,#217461,#217462,#217463,#217464,#217465,#217466,#217467,#217468,
#217469,#217470,#217471,#217472,#217473,#217474,#217475,#217476,#217477,
#217478,#217479,#217480,#217481,#217482,#217483,#217484,#217485,#217486,
#217487,#217488,#217489,#217490,#217491,#217492,#217493,#217494,#217495,
#217496,#217497,#217498,#217499,#217500,#217501,#217502,#217503,#217504,
#217505,#217506,#217507,#217508,#217509,#217510,#217511,#217512,#217513,
#217514,#217515,#217516,#217517,#217518,#217519,#217520,#217521,#217522,
#217523,#217524,#217525,#217526,#217527,#217528,#217529,#217530,#217531,
#217532,#217533,#217534,#217535,#217536,#217537,#217538,#217539,#217540,
#217541,#217542,#217543,#217544,#217545,#217546,#217547,#217548,#217549,
#217550,#217551,#217552,#217553,#217554,#217555,#217556,#217557,#217558,
#217559,#217560,#217561,#217562,#217563,#217564,#217565,#217566,#217567,
#217568,#217569,#217570,#217571,#217572,#217573,#217574,#217575),
 .UNSPECIFIED.,.F.,.F.,(4,3,3,3,3,3,3,3,3,3,3,3,3,3,3,3,3,3,3,3,3,3,3,3,
3,3,3,3,3,3,3,3,3,3,3,3,3,3,3,3,3,3,3,3,3,3,3,3,3,3,3,3,3,3,3,3,3,3,3,3,
3,3,3,3,3,3,3,3,3,3,3,3,3,3,3,3,3,3,3,3,3,3,4),(-60.6412095134584,-60.5590784046771,
-60.4793357811508,-60.3995857810152,-60.3198128184427,-60.235899774634,
-60.1559884534018,-60.0760181955046,-59.995936002992,-59.9841606432079,
-59.9042033430767,-59.8243405458341,-59.7445547233624,-59.664828408167,
-59.5851441798728,-59.5054731936519,-59.4258057401261,-59.3461260893097,
-59.2664185069152,-59.1866232778397,-59.106778936132,-59.0268205090847,
-58.9844246324877,-58.9044673323564,-58.8246045351137,-58.7448187126417,
-58.6650923974462,-58.5854081691519,-58.5057371829309,-58.4260697294049,
-58.3463900785883,-58.2666824961936,-58.186887267118,-58.1070429254103,
-58.0270844983627,-57.9846886217676,-57.9047313216364,-57.8248685243939,
-57.7450827019221,-57.6653563867272,-57.5856721584333,-57.5060011722124,
-57.4263337186865,-57.3466540678699,-57.2669464854756,-57.1871512564001,
-57.1073069146926,-57.0273484876453,-56.9849526110475,-56.9049953109163,
-56.8251325136738,-56.7453466912019,-56.6656203760066,-56.5859361477129,
-56.5062651614919,-56.4265977079658,-56.3469180571494,-56.2672104747552,
-56.1874152456796,-56.1075709039718,-56.0276124769243,-55.9852166003274,
-55.9052593001963,-55.8253965029537,-55.7456106804819,-55.665884365286,
-55.5862001369919,-55.506529150771,-55.426861697245,-55.3471820464283,-55.2674744640334,
-55.1876792349578,-55.1078348932506,-55.0278764662033,-54.9854805896072,
-54.9049169077671,-54.8244508849754,-54.7440673257589,-54.6637510888401,
-54.5834913281942,-54.5032654666035,-54.4230482427655,-54.3580242062788),
 .UNSPECIFIED.);
#1754=B_SPLINE_CURVE_WITH_KNOTS('',3,(#217577,#217578,#217579,#217580,#217581,
#217582,#217583,#217584,#217585,#217586),.UNSPECIFIED.,.F.,.F.,(4,1,1,1,
1,1,1,4),(-54.3580165317574,-53.9857445788871,-52.9860085681669,-51.9862725574468,
-50.9865365467267,-49.9868005360066,-48.9870645252864,-48.0748476368028),
 .UNSPECIFIED.);
#1755=B_SPLINE_CURVE_WITH_KNOTS('',3,(#217588,#217589,#217590,#217591,#217592,
#217593,#217594,#217595,#217596,#217597,#217598,#217599,#217600,#217601,
#217602,#217603,#217604,#217605,#217606,#217607,#217608,#217609,#217610,
#217611,#217612,#217613,#217614,#217615,#217616,#217617,#217618,#217619,
#217620,#217621,#217622,#217623,#217624,#217625,#217626,#217627,#217628,
#217629,#217630,#217631,#217632,#217633,#217634,#217635,#217636,#217637,
#217638,#217639,#217640,#217641,#217642,#217643,#217644,#217645,#217646,
#217647,#217648,#217649,#217650,#217651,#217652,#217653,#217654,#217655,
#217656,#217657,#217658,#217659,#217660,#217661,#217662,#217663,#217664,
#217665,#217666,#217667,#217668,#217669,#217670,#217671,#217672,#217673,
#217674,#217675,#217676,#217677,#217678,#217679,#217680,#217681,#217682,
#217683,#217684,#217685,#217686,#217687,#217688,#217689,#217690,#217691,
#217692,#217693,#217694,#217695,#217696,#217697,#217698,#217699,#217700,
#217701,#217702,#217703,#217704,#217705,#217706,#217707,#217708,#217709,
#217710,#217711,#217712,#217713,#217714,#217715,#217716,#217717,#217718,
#217719,#217720,#217721,#217722,#217723,#217724,#217725,#217726,#217727,
#217728,#217729,#217730,#217731,#217732,#217733,#217734,#217735,#217736,
#217737,#217738,#217739,#217740,#217741,#217742,#217743,#217744,#217745,
#217746,#217747,#217748,#217749,#217750,#217751,#217752,#217753,#217754,
#217755,#217756,#217757,#217758,#217759,#217760,#217761,#217762,#217763,
#217764,#217765,#217766,#217767,#217768,#217769,#217770,#217771,#217772,
#217773,#217774,#217775,#217776,#217777,#217778,#217779,#217780,#217781,
#217782,#217783,#217784,#217785,#217786,#217787,#217788,#217789,#217790,
#217791,#217792,#217793,#217794,#217795,#217796,#217797,#217798,#217799,
#217800,#217801,#217802,#217803,#217804,#217805,#217806,#217807,#217808,
#217809,#217810,#217811,#217812,#217813,#217814,#217815,#217816,#217817,
#217818,#217819,#217820,#217821,#217822,#217823,#217824,#217825,#217826,
#217827,#217828,#217829,#217830,#217831),.UNSPECIFIED.,.F.,.F.,(4,3,3,3,
3,3,3,3,3,3,3,3,3,3,3,3,3,3,3,3,3,3,3,3,3,3,3,3,3,3,3,3,3,3,3,3,3,3,3,3,
3,3,3,3,3,3,3,3,3,3,3,3,3,3,3,3,3,3,3,3,3,3,3,3,3,3,3,3,3,3,3,3,3,3,3,3,
3,3,3,3,3,4),(-48.0748388990992,-47.9873285145663,-47.9073712144349,-47.8275084171922,
-47.7477225947202,-47.6679962795249,-47.5883120512307,-47.5086410650096,
-47.4289736114836,-47.3492939606671,-47.2695863782722,-47.1897911491966,
-47.1099468074887,-47.0299883804412,-46.9875925038462,-46.9076352037149,
-46.8277724064724,-46.7479865840006,-46.6682602688053,-46.5885760405113,
-46.5089050542904,-46.4292376007644,-46.3495579499479,-46.2698503675534,
-46.1900551384779,-46.1102107967703,-46.0302523697229,-45.987856493126,
-45.9078991929947,-45.8280363957522,-45.7482505732803,-45.668524258085,
-45.5888400297908,-45.5091690435699,-45.429501590044,-45.3498219392276,
-45.270114356833,-45.1903191277575,-45.1104747860499,-45.0305163590025,
-44.9881204824059,-44.9081631822747,-44.8283003850321,-44.7485145625602,
-44.668788247365,-44.5891040190709,-44.50943303285,-44.4297655793241,-44.3500859285076,
-44.2703783461131,-44.1905831170376,-44.1107387753299,-44.0307803482826,
-43.9883844716858,-43.9084271715545,-43.8285643743119,-43.74877855184,-43.6690522366447,
-43.5893680083507,-43.5096970221298,-43.4300295686039,-43.3503499177874,
-43.2706423353929,-43.1908471063174,-43.1110027646097,-43.0310443375623,
-42.9886484609656,-42.9086911608343,-42.8288283635917,-42.7490425411198,
-42.6693162259245,-42.5896319976304,-42.5099610114094,-42.4302935578836,
-42.3506139070671,-42.2709063246724,-42.1911110955969,-42.1112667538892,
-42.0313083268418,-41.9889124502455,-41.8733272325874,-41.7916535919196),
 .UNSPECIFIED.);
#1756=B_SPLINE_CURVE_WITH_KNOTS('',3,(#217833,#217834,#217835,#217836,#217837,
#217838,#217839,#217840,#217841,#217842),.UNSPECIFIED.,.F.,.F.,(4,1,1,1,
1,1,1,4),(-41.7916500544357,-40.9891764395254,-39.9894404288052,-38.9897044180851,
-37.989968407365,-36.9902323966448,-35.9904963859247,-35.50846828474),
 .UNSPECIFIED.);
#1757=B_SPLINE_CURVE_WITH_KNOTS('',3,(#217844,#217845,#217846,#217847,#217848,
#217849,#217850,#217851,#217852,#217853),.UNSPECIFIED.,.F.,.F.,(4,1,1,1,
1,1,1,4),(-35.50846828474,-34.9907603752046,-33.9910243644845,-32.9912883537643,
-31.9915523430442,-30.9918163323241,-29.9920803216039,-29.2252829775605),
 .UNSPECIFIED.);
#1758=B_SPLINE_CURVE_WITH_KNOTS('',3,(#217855,#217856,#217857,#217858,#217859,
#217860,#217861,#217862,#217863,#217864,#217865),.UNSPECIFIED.,.F.,.F.,
(4,1,1,1,1,1,1,1,4),(-29.2252829775605,-28.9923443108838,-27.9926083001637,
-26.9928722894435,-25.9931362787234,-24.9934002680033,-23.9936642572832,
-22.993928246563,-22.9420976703809),.UNSPECIFIED.);
#1759=B_SPLINE_CURVE_WITH_KNOTS('',3,(#217867,#217868,#217869,#217870,#217871,
#217872,#217873,#217874,#217875,#217876),.UNSPECIFIED.,.F.,.F.,(4,1,1,1,
1,1,1,4),(-22.9420976703809,-21.9941922358429,-20.9944562251228,-19.9947202144026,
-18.9949842036825,-17.9952481929624,-16.9955121822422,-16.6589198685825),
 .UNSPECIFIED.);
#1760=B_SPLINE_CURVE_WITH_KNOTS('',3,(#217878,#217879,#217880,#217881,#217882,
#217883,#217884,#217885,#217886,#217887,#217888,#217889,#217890,#217891,
#217892,#217893,#217894,#217895,#217896,#217897,#217898,#217899,#217900,
#217901,#217902,#217903,#217904,#217905,#217906,#217907,#217908,#217909,
#217910,#217911,#217912,#217913,#217914,#217915,#217916,#217917,#217918,
#217919,#217920,#217921,#217922,#217923,#217924,#217925,#217926,#217927,
#217928,#217929,#217930,#217931,#217932,#217933,#217934,#217935,#217936,
#217937,#217938,#217939,#217940,#217941,#217942,#217943,#217944,#217945,
#217946,#217947,#217948,#217949,#217950,#217951,#217952,#217953,#217954,
#217955,#217956,#217957,#217958,#217959,#217960,#217961,#217962,#217963,
#217964,#217965,#217966,#217967,#217968,#217969,#217970,#217971,#217972,
#217973,#217974,#217975,#217976,#217977,#217978,#217979,#217980,#217981,
#217982,#217983,#217984,#217985,#217986,#217987,#217988,#217989,#217990,
#217991,#217992,#217993,#217994,#217995,#217996,#217997,#217998,#217999,
#218000,#218001,#218002,#218003,#218004,#218005,#218006,#218007,#218008,
#218009,#218010,#218011,#218012,#218013,#218014,#218015,#218016,#218017,
#218018,#218019,#218020,#218021,#218022,#218023,#218024,#218025,#218026,
#218027,#218028,#218029,#218030,#218031,#218032,#218033,#218034,#218035,
#218036,#218037,#218038,#218039,#218040,#218041,#218042,#218043),
 .UNSPECIFIED.,.F.,.F.,(4,3,3,3,3,3,3,3,3,3,3,3,3,3,3,3,3,3,3,3,3,3,3,3,
3,3,3,3,3,3,3,3,3,3,3,3,3,3,3,3,3,3,3,3,3,3,3,3,3,3,3,3,3,3,3,4),(-16.6589123632013,
-16.5760203392414,-16.4963658357425,-16.4167062586062,-16.3370259313394,
-16.257309167994,-16.1774967883031,-16.0976279107091,-16.0176451019278,
-15.9957761715221,-15.9158187324329,-15.8359557956803,-15.7561698332831,
-15.6764433778821,-15.5967590092361,-15.5170878828934,-15.4374202894017,
-15.3577404988956,-15.2780327772076,-15.198237410145,-15.118392930983,-15.0384343685027,
-14.996040160802,-14.9160831648467,-14.8362206718143,-14.7564351533039,
-14.6767091415404,-14.5970252158687,-14.5173545301081,-14.4376873756752,
-14.3580080223317,-14.278300735536,-14.1985057977278,-14.1186617452726,
-14.0387036018344,-13.9963041500818,-13.9163467244748,-13.8364838036546,
-13.7566978595943,-13.6769714248905,-13.5972870792609,-13.5176159792981,
-13.4379484142657,-13.3582686542656,-13.2785609651003,-13.1987656334386,
-13.1189211913589,-13.0389626682522,-12.9965681393617,-12.9166104714522,
-12.8367437733771,-12.7569521629902,-12.6772283666737,-12.5975435612502,
-12.5178804549894,-12.4923778478243),.UNSPECIFIED.);
#1761=B_SPLINE_CURVE_WITH_KNOTS('',3,(#218045,#218046,#218047,#218048,#218049,
#218050,#218051,#218052,#218053,#218054,#218055,#218056,#218057,#218058,
#218059,#218060,#218061,#218062,#218063,#218064,#218065,#218066,#218067,
#218068,#218069,#218070,#218071,#218072,#218073,#218074,#218075,#218076,
#218077,#218078,#218079,#218080),.UNSPECIFIED.,.F.,.F.,(4,2,2,2,2,2,2,2,
2,2,2,2,2,2,2,2,2,4),(0.00526237292542417,0.138566189979076,0.366294164048727,
0.418967542934504,0.430275546436095,0.431328859894763,0.431533790643745,
0.431789609184076,0.431892486759413,0.431959062395792,0.43202128231436,
0.432103906517542,0.432281648026571,0.434594111412943,0.465840068485782,
0.538620422200195,0.640014286401001,0.807590978544382),.UNSPECIFIED.);
#1762=B_SPLINE_CURVE_WITH_KNOTS('',3,(#218082,#218083,#218084,#218085,#218086,
#218087,#218088,#218089,#218090,#218091,#218092,#218093,#218094,#218095,
#218096,#218097,#218098,#218099,#218100,#218101,#218102,#218103,#218104,
#218105,#218106,#218107,#218108,#218109),.UNSPECIFIED.,.F.,.F.,(4,3,3,3,
3,3,3,3,3,4),(-11.06261597483,-10.9970961179214,-10.9164104612955,-10.8358235390976,
-10.7553203015422,-10.6748857539058,-10.5945105281497,-10.5141705799321,
-10.4338432861682,-10.3757270560217),.UNSPECIFIED.);
#1763=B_SPLINE_CURVE_WITH_KNOTS('',3,(#218111,#218112,#218113,#218114,#218115),
 .UNSPECIFIED.,.F.,.F.,(4,1,4),(-10.3757194590647,-9.99736010720131,-9.9877456995066),
 .UNSPECIFIED.);
#1764=B_SPLINE_CURVE_WITH_KNOTS('',3,(#218116,#218117,#218118,#218119,#218120,
#218121,#218122,#218123,#218124,#218125),.UNSPECIFIED.,.F.,.F.,(4,2,2,2,
4),(0.00246287485863373,0.0946583498619244,0.18080663761715,0.264674289446545,
0.349802769075605),.UNSPECIFIED.);
#1765=B_SPLINE_CURVE_WITH_KNOTS('',3,(#218127,#218128,#218129,#218130,#218131,
#218132,#218133,#218134,#218135,#218136),.UNSPECIFIED.,.F.,.F.,(4,3,3,4),
(21.740715980233,21.8348722215429,21.9284884766943,21.9911485749198),
 .UNSPECIFIED.);
#1766=B_SPLINE_CURVE_WITH_KNOTS('',3,(#218137,#218138,#218139,#218140,#218141,
#218142,#218143,#218144,#218145,#218146,#218147,#218148,#218149,#218150,
#218151,#218152,#218153,#218154,#218155,#218156,#218157,#218158,#218159,
#218160,#218161,#218162,#218163,#218164,#218165,#218166,#218167,#218168,
#218169,#218170,#218171,#218172,#218173,#218174,#218175,#218176,#218177,
#218178,#218179,#218180,#218181,#218182,#218183,#218184,#218185,#218186,
#218187,#218188,#218189,#218190,#218191,#218192,#218193,#218194,#218195,
#218196,#218197,#218198,#218199,#218200,#218201,#218202,#218203,#218204,
#218205,#218206,#218207,#218208,#218209,#218210,#218211,#218212,#218213,
#218214,#218215,#218216,#218217,#218218,#218219,#218220,#218221,#218222,
#218223,#218224,#218225,#218226,#218227,#218228,#218229,#218230,#218231,
#218232,#218233,#218234,#218235,#218236,#218237,#218238,#218239,#218240,
#218241,#218242,#218243,#218244,#218245,#218246,#218247,#218248,#218249,
#218250,#218251,#218252,#218253,#218254,#218255,#218256,#218257,#218258,
#218259,#218260,#218261,#218262,#218263,#218264,#218265,#218266,#218267,
#218268,#218269,#218270,#218271,#218272,#218273,#218274,#218275,#218276,
#218277,#218278,#218279,#218280,#218281,#218282,#218283,#218284,#218285,
#218286,#218287,#218288,#218289,#218290,#218291,#218292,#218293,#218294,
#218295,#218296,#218297,#218298,#218299,#218300,#218301,#218302,#218303,
#218304,#218305,#218306,#218307,#218308,#218309,#218310,#218311,#218312,
#218313,#218314,#218315,#218316,#218317,#218318,#218319,#218320,#218321,
#218322,#218323,#218324,#218325,#218326,#218327,#218328,#218329,#218330,
#218331,#218332,#218333,#218334,#218335,#218336,#218337,#218338,#218339,
#218340,#218341,#218342,#218343,#218344,#218345,#218346,#218347,#218348,
#218349,#218350,#218351,#218352,#218353,#218354,#218355,#218356),
 .UNSPECIFIED.,.F.,.F.,(4,3,3,3,3,3,3,3,3,3,3,3,3,3,3,3,3,3,3,3,3,3,3,3,
3,3,3,3,3,3,3,3,3,3,3,3,3,3,3,3,3,3,3,3,3,3,3,3,3,3,3,3,3,3,3,3,3,3,3,3,
3,3,3,3,3,3,3,3,3,3,3,3,3,4),(21.9911485751133,22.0752803066499,22.1594213519125,
22.2435887880297,22.327799705763,22.412122635211,22.496510193649,22.5810312627201,
22.6125176370092,22.6962542579476,22.7798876501835,22.8634379486364,22.9469252160963,
23.0303769702507,23.1138112508511,23.1972461326295,23.2806996868859,23.3642419314503,
23.4478287585743,23.531549780005,23.6122536477293,23.6959932091553,23.7796295777105,
23.8631828849443,23.946673190331,24.0301280160616,24.113565388298,24.1970033788866,
24.2804600562506,24.3640054289813,24.4475953919903,24.5313195307922,24.6119896584494,
24.6957284703853,24.7793640854067,24.8629166358964,24.9464061821532,25.0298602478526,
25.11329685962,25.1967340900312,25.2801900082394,25.3637346277638,25.4473238396068,
25.5310472383997,25.6117256691696,25.6954640854281,25.7790992970342,25.8626514368397,
25.9461405656013,26.0295942048811,26.1130303848521,26.196467178482,26.2799226553132,
26.3634668286356,26.4470555909439,26.5307785390076,26.6114616798897,26.6952005328961,
26.7788361868141,26.8623887739932,26.9458783546974,27.0293324512814,27.1127690917577,
27.1962063486646,27.2796622911176,27.3632069311557,27.4467961615158,27.530519575186,
27.6111976906098,27.6949624620804,27.7785925584211,27.8621451536583,27.9456293039383,
28.0234162092491),.UNSPECIFIED.);
#1767=B_SPLINE_CURVE_WITH_KNOTS('',3,(#225139,#225140,#225141,#225142,#225143,
#225144,#225145,#225146,#225147,#225148),.UNSPECIFIED.,.F.,.F.,(4,2,2,2,
4),(0.00207047843994134,0.0654884822806935,0.146439093390922,0.270589396385427,
0.30899941932235),.UNSPECIFIED.);
#1768=B_SPLINE_CURVE_WITH_KNOTS('',3,(#225150,#225151,#225152,#225153,#225154,
#225155,#225156,#225157,#225158,#225159,#225160,#225161,#225162,#225163,
#225164,#225165,#225166,#225167,#225168,#225169,#225170,#225171),
 .UNSPECIFIED.,.F.,.F.,(4,3,3,3,3,3,3,4),(-117.731943690408,-117.653301723801,
-117.574693912514,-117.496103732189,-117.417487955491,-117.338861162405,
-117.260163820455,-117.189877278075),.UNSPECIFIED.);
#1769=B_SPLINE_CURVE_WITH_KNOTS('',3,(#225173,#225174,#225175,#225176,#225177),
 .UNSPECIFIED.,.F.,.F.,(4,1,4),(-117.189877278075,-116.969113254255,-116.302843017259),
 .UNSPECIFIED.);
#1770=B_SPLINE_CURVE_WITH_KNOTS('',3,(#225178,#225179,#225180,#225181,#225182,
#225183,#225184,#225185,#225186,#225187,#225188,#225189,#225190,#225191,
#225192,#225193,#225194,#225195,#225196,#225197,#225198,#225199,#225200,
#225201,#225202,#225203,#225204,#225205,#225206,#225207,#225208,#225209,
#225210,#225211),.UNSPECIFIED.,.F.,.F.,(4,2,2,2,2,2,2,2,2,2,2,2,2,2,2,2,
4),(0.30899941932235,0.382261953082336,0.394186641374844,0.394544069032282,
0.394634720258392,0.394685917699195,0.394729273851375,0.394781112651507,
0.394874741417267,0.39532213142483,0.396149736574269,0.399586578362255,
0.423862460061527,0.495493129981234,0.635502803715609,0.721928150979562,
0.797536521561463),.UNSPECIFIED.);
#1771=B_SPLINE_CURVE_WITH_KNOTS('',3,(#225214,#225215,#225216,#225217,#225218,
#225219),.UNSPECIFIED.,.F.,.F.,(4,2,4),(0.0641900250749046,0.225569656006002,
0.227853963255062),.UNSPECIFIED.);
#1772=B_SPLINE_CURVE_WITH_KNOTS('',3,(#225221,#225222,#225223,#225224,#225225,
#225226,#225227,#225228,#225229,#225230,#225231,#225232,#225233,#225234,
#225235,#225236,#225237,#225238,#225239,#225240,#225241,#225242,#225243,
#225244,#225245,#225246,#225247,#225248,#225249,#225250,#225251,#225252,
#225253,#225254,#225255,#225256,#225257,#225258,#225259,#225260,#225261,
#225262,#225263,#225264,#225265,#225266,#225267,#225268,#225269,#225270,
#225271,#225272,#225273,#225274,#225275,#225276,#225277,#225278,#225279,
#225280,#225281,#225282,#225283,#225284,#225285,#225286,#225287,#225288,
#225289,#225290,#225291,#225292,#225293,#225294,#225295,#225296,#225297,
#225298,#225299,#225300,#225301,#225302,#225303,#225304,#225305,#225306,
#225307,#225308,#225309,#225310,#225311,#225312,#225313,#225314,#225315,
#225316,#225317,#225318,#225319,#225320,#225321,#225322,#225323,#225324,
#225325,#225326,#225327,#225328,#225329,#225330,#225331,#225332,#225333,
#225334,#225335,#225336,#225337,#225338,#225339,#225340,#225341,#225342,
#225343,#225344,#225345,#225346,#225347,#225348,#225349,#225350,#225351,
#225352,#225353,#225354,#225355,#225356,#225357,#225358,#225359,#225360,
#225361,#225362,#225363,#225364,#225365,#225366,#225367,#225368,#225369,
#225370,#225371,#225372,#225373,#225374,#225375,#225376,#225377,#225378,
#225379,#225380,#225381,#225382,#225383,#225384,#225385,#225386,#225387,
#225388,#225389,#225390,#225391,#225392,#225393,#225394,#225395,#225396,
#225397,#225398,#225399,#225400,#225401),.UNSPECIFIED.,.F.,.F.,(4,3,3,3,
3,3,3,3,3,3,3,3,3,3,3,3,3,3,3,3,3,3,3,3,3,3,3,3,3,3,3,3,3,3,3,3,3,3,3,3,
3,3,3,3,3,3,3,3,3,3,3,3,3,3,3,3,3,3,3,3,4),(107.933005315568,107.971489157774,
108.051446457905,108.131309255148,108.21109507762,108.290821392815,108.370505621109,
108.45017660733,108.529844060856,108.609523711672,108.689231294067,108.769026523142,
108.84887086485,108.928829291897,108.971225168494,109.051182468625,109.131045265868,
109.21083108834,109.290557403535,109.370241631829,109.44991261805,109.529580071576,
109.609259722392,109.688967304787,109.768762533862,109.84860687557,109.928565302617,
109.970961179214,110.050918479345,110.130781276588,110.21056709906,110.290293414255,
110.369977642549,110.44964862877,110.529316082296,110.608995733112,110.688703315507,
110.768498544582,110.84834288629,110.928301313337,110.970697189934,111.050654490065,
111.130517287308,111.210303109779,111.290029424975,111.369713653269,111.449384639489,
111.529052093015,111.608731743832,111.688439326226,111.768234555301,111.848078897009,
111.928037324056,111.970433200654,112.05038393002,112.130244727001,112.210031469601,
112.29129664253,112.370980493117,112.453036327217,112.535092161318),
 .UNSPECIFIED.);
#1773=B_SPLINE_CURVE_WITH_KNOTS('',3,(#225403,#225404,#225405,#225406,#225407,
#225408,#225409,#225410,#225411,#225412),.UNSPECIFIED.,.F.,.F.,(4,1,1,1,
1,1,1,4),(101.649820008388,101.973073093453,102.972809104173,103.972545114893,
104.972281125613,105.972017136334,106.971753147054,107.93300001923),
 .UNSPECIFIED.);
#1774=B_SPLINE_CURVE_WITH_KNOTS('',3,(#225414,#225415,#225416,#225417,#225418,
#225419,#225420,#225421,#225422,#225423),.UNSPECIFIED.,.F.,.F.,(4,1,1,1,
1,1,1,4),(95.3666347012089,95.9746570291324,96.9743930398526,97.9741290505727,
98.9738650612928,99.973601072013,100.973337082733,101.649820008388),
 .UNSPECIFIED.);
#1775=B_SPLINE_CURVE_WITH_KNOTS('',3,(#225425,#225426,#225427,#225428,#225429,
#225430,#225431,#225432,#225433,#225434),.UNSPECIFIED.,.F.,.F.,(4,1,1,1,
1,1,1,4),(89.0834493940292,89.9762409648117,90.9759769755319,91.975712986252,
92.9754489969721,93.9751850076922,94.9749210184123,95.3666347012089),
 .UNSPECIFIED.);
#1776=B_SPLINE_CURVE_WITH_KNOTS('',3,(#225436,#225437,#225438,#225439,#225440,
#225441,#225442,#225443,#225444,#225445,#225446),.UNSPECIFIED.,.F.,.F.,
(4,1,1,1,1,1,1,1,4),(82.8002640868496,82.9780888897707,83.9778249004908,
84.977560911211,85.9772969219311,86.9770329326513,87.9767689433714,88.9765049540916,
89.0834493940292),.UNSPECIFIED.);
#1777=B_SPLINE_CURVE_WITH_KNOTS('',3,(#225448,#225449,#225450,#225451,#225452,
#225453,#225454,#225455,#225456,#225457,#225458,#225459,#225460,#225461,
#225462,#225463,#225464,#225465,#225466,#225467,#225468,#225469,#225470,
#225471,#225472,#225473,#225474,#225475,#225476,#225477,#225478,#225479,
#225480,#225481,#225482,#225483,#225484,#225485,#225486,#225487,#225488,
#225489,#225490,#225491,#225492,#225493,#225494,#225495,#225496,#225497,
#225498,#225499,#225500,#225501,#225502,#225503,#225504,#225505,#225506,
#225507,#225508,#225509,#225510,#225511,#225512,#225513,#225514,#225515,
#225516,#225517,#225518,#225519,#225520,#225521,#225522,#225523,#225524,
#225525,#225526,#225527,#225528,#225529,#225530,#225531,#225532,#225533,
#225534,#225535,#225536,#225537,#225538,#225539,#225540,#225541,#225542,
#225543,#225544,#225545,#225546,#225547,#225548,#225549,#225550,#225551,
#225552,#225553,#225554,#225555,#225556,#225557,#225558,#225559,#225560,
#225561,#225562,#225563,#225564,#225565,#225566,#225567,#225568,#225569,
#225570,#225571,#225572,#225573,#225574,#225575,#225576,#225577,#225578,
#225579,#225580,#225581,#225582,#225583,#225584,#225585,#225586,#225587,
#225588,#225589,#225590,#225591,#225592,#225593,#225594,#225595,#225596,
#225597,#225598,#225599,#225600,#225601,#225602,#225603,#225604,#225605,
#225606,#225607,#225608,#225609,#225610,#225611,#225612,#225613,#225614,
#225615,#225616,#225617,#225618,#225619,#225620,#225621,#225622,#225623,
#225624,#225625,#225626,#225627,#225628,#225629,#225630,#225631,#225632,
#225633,#225634,#225635,#225636,#225637,#225638,#225639,#225640,#225641,
#225642,#225643,#225644,#225645,#225646,#225647,#225648,#225649,#225650,
#225651,#225652,#225653,#225654,#225655,#225656,#225657,#225658,#225659,
#225660,#225661,#225662,#225663,#225664,#225665,#225666,#225667,#225668,
#225669,#225670,#225671,#225672,#225673,#225674,#225675,#225676,#225677,
#225678,#225679,#225680,#225681,#225682,#225683,#225684,#225685,#225686,
#225687,#225688,#225689,#225690,#225691,#225692,#225693,#225694),
 .UNSPECIFIED.,.F.,.F.,(4,3,3,3,3,3,3,3,3,3,3,3,3,3,3,3,3,3,3,3,3,3,3,3,
3,3,3,3,3,3,3,3,3,3,3,3,3,3,3,3,3,3,3,3,3,3,3,3,3,3,3,3,3,3,3,3,3,3,3,3,
3,3,3,3,3,3,3,3,3,3,3,3,3,3,3,3,3,3,3,3,3,3,4),(76.5170789829915,76.6019516902264,
76.6869832338072,76.7722619244241,76.8576735508233,76.9432918856119,76.97967282545,
77.0596301255811,77.1394929228235,77.2192787452951,77.2990050604903,77.3786892887841,
77.4583602750048,77.5380277285305,77.6177073793468,77.6974149617411,77.7772101908165,
77.8570545325239,77.9370129595711,77.9794088361701,78.0593661363013,78.1392289335439,
78.2190147560157,78.298741071211,78.3784252995052,78.4580962857261,78.537763739252,
78.6174433900685,78.6971509724629,78.7769462015385,78.8567905432461,78.9367489702935,
78.9791448468902,79.0591021470215,79.1389649442642,79.2187507667361,79.2984770819315,
79.3781613102257,79.4578322964467,79.5374997499727,79.6171794007892,79.6968869831838,
79.7766822122594,79.8565265539671,79.9364849810146,79.9788808576104,80.0588381577416,
80.1387009549841,80.2184867774559,80.2982130926512,80.3778973209452,80.4575683071661,
80.537235760692,80.6169154115085,80.696622993903,80.7764182229785,80.856262564686,
80.9362209917334,80.9786168683304,81.0585741684617,81.1384369657043,81.2182227881762,
81.2979491033716,81.3776333316657,81.4573043178867,81.5369717714127,81.6166514222292,
81.6963590046238,81.7761542336994,81.8559985754071,81.9359570024545,81.9783528790506,
82.0571196435331,82.1357922323713,82.2143891387368,82.2929249535672,82.37142792239,
82.4499146286459,82.5284016410875,82.6069360191478,82.6854971762447,82.764138078185,
82.8002640868496),.UNSPECIFIED.);
#1778=B_SPLINE_CURVE_WITH_KNOTS('',3,(#225696,#225697,#225698,#225699,#225700,
#225701,#225702,#225703,#225704,#225705),.UNSPECIFIED.,.F.,.F.,(4,1,1,1,
1,1,1,4),(70.2338934724905,70.9812567611292,71.9809927718493,72.9807287825695,
73.9804647932896,74.9802008040097,75.9799368147299,76.5170787796701),
 .UNSPECIFIED.);
#1779=B_SPLINE_CURVE_WITH_KNOTS('',3,(#225707,#225708,#225709,#225710,#225711,
#225712,#225713,#225714,#225715,#225716,#225717,#225718,#225719,#225720,
#225721,#225722,#225723,#225724,#225725,#225726,#225727,#225728,#225729,
#225730,#225731,#225732,#225733,#225734,#225735,#225736,#225737,#225738,
#225739,#225740,#225741,#225742,#225743,#225744,#225745,#225746,#225747,
#225748,#225749,#225750,#225751,#225752,#225753,#225754,#225755,#225756,
#225757,#225758,#225759,#225760,#225761,#225762,#225763,#225764,#225765,
#225766,#225767,#225768,#225769,#225770,#225771,#225772,#225773,#225774,
#225775,#225776,#225777,#225778,#225779,#225780,#225781,#225782,#225783,
#225784,#225785,#225786,#225787,#225788,#225789,#225790,#225791,#225792,
#225793,#225794,#225795,#225796,#225797,#225798,#225799,#225800,#225801,
#225802,#225803,#225804,#225805,#225806,#225807,#225808,#225809,#225810,
#225811,#225812,#225813,#225814,#225815,#225816,#225817,#225818,#225819,
#225820,#225821,#225822,#225823,#225824,#225825,#225826,#225827,#225828,
#225829,#225830,#225831,#225832,#225833,#225834,#225835,#225836,#225837,
#225838,#225839,#225840,#225841,#225842,#225843,#225844,#225845,#225846,
#225847,#225848,#225849,#225850,#225851,#225852,#225853,#225854,#225855,
#225856,#225857,#225858,#225859,#225860,#225861,#225862,#225863,#225864,
#225865,#225866,#225867,#225868,#225869,#225870,#225871,#225872,#225873,
#225874,#225875,#225876,#225877,#225878,#225879,#225880,#225881,#225882,
#225883,#225884,#225885,#225886,#225887,#225888,#225889,#225890,#225891,
#225892,#225893,#225894,#225895,#225896,#225897,#225898,#225899,#225900,
#225901,#225902,#225903,#225904,#225905,#225906,#225907,#225908,#225909,
#225910,#225911,#225912,#225913,#225914,#225915,#225916,#225917,#225918,
#225919,#225920,#225921,#225922,#225923,#225924,#225925,#225926,#225927,
#225928,#225929,#225930,#225931,#225932,#225933,#225934,#225935,#225936,
#225937,#225938,#225939,#225940,#225941,#225942,#225943,#225944,#225945,
#225946,#225947,#225948,#225949,#225950,#225951,#225952,#225953),
 .UNSPECIFIED.,.F.,.F.,(4,3,3,3,3,3,3,3,3,3,3,3,3,3,3,3,3,3,3,3,3,3,3,3,
3,3,3,3,3,3,3,3,3,3,3,3,3,3,3,3,3,3,3,3,3,3,3,3,3,3,3,3,3,3,3,3,3,3,3,3,
3,3,3,3,3,3,3,3,3,3,3,3,3,3,3,3,3,3,3,3,3,3,4),(63.9507081653109,63.9831046860883,
64.0630619862195,64.142924783462,64.2227106059338,64.3024369211289,64.382121149423,
64.4617921356438,64.5414595891696,64.621139239986,64.7008468223806,64.7806420514561,
64.8604863931635,64.9404448202108,64.9828406968084,65.0627979969396,65.1426607941822,
65.2224466166541,65.3021729318493,65.3818571601433,65.4615281463642,65.5411955998901,
65.6208752507066,65.7005828331011,65.7803780621766,65.8602224038843,65.9401808309317,
65.9825767075286,66.0625340076599,66.1423968049025,66.2221826273744,66.3019089425698,
66.381593170864,66.461264157085,66.540931610611,66.6206112614275,66.7003188438221,
66.7801140728977,66.8599584146054,66.9399168416528,66.9823127182487,67.0622700183799,
67.1421328156224,67.2219186380942,67.3016449532894,67.3813291815834,67.4610001678043,
67.5406676213301,67.6203472721465,67.700054854541,67.7798500836165,67.8596944253241,
67.9396528523714,67.9820487289688,68.0620060291001,68.1418688263428,68.2216546488147,
68.30138096401,68.381065192304,68.460736178525,68.540403632051,68.6200832828675,
68.6997908652621,68.7795860943376,68.8594304360453,68.9393888630927,68.9817847396889,
69.0617420398201,69.1416048370627,69.2213906595346,69.3011169747299,69.3808012030239,
69.4604721892448,69.5401396427707,69.6198192935872,69.6995268759819,69.7793221050574,
69.8591664467649,69.9391248738123,69.981520750409,70.0859426319418,70.1882149143938,
70.2338934108873),.UNSPECIFIED.);
#1780=B_SPLINE_CURVE_WITH_KNOTS('',3,(#225955,#225956,#225957,#225958,#225959,
#225960,#225961,#225962,#225963,#225964),.UNSPECIFIED.,.F.,.F.,(4,1,1,1,
1,1,1,4),(57.6675228581313,57.9846886217673,58.9844246324875,59.9841606432076,
60.9838966539278,61.983632664648,62.9833686753681,63.9507037176747),
 .UNSPECIFIED.);
#1781=B_SPLINE_CURVE_WITH_KNOTS('',3,(#225966,#225967,#225968,#225969,#225970,
#225971,#225972,#225973,#225974,#225975),.UNSPECIFIED.,.F.,.F.,(4,1,1,1,
1,1,1,4),(51.3843375509517,51.9862725574467,52.9860085681668,53.9857445788869,
54.985480589607,55.9852166003271,56.9849526110472,57.6675228581313),
 .UNSPECIFIED.);
#1782=B_SPLINE_CURVE_WITH_KNOTS('',3,(#225977,#225978,#225979,#225980,#225981,
#225982,#225983,#225984,#225985,#225986),.UNSPECIFIED.,.F.,.F.,(4,1,1,1,
1,1,1,4),(45.1011522437721,45.9878564931259,46.9875925038461,47.9873285145662,
48.9870645252863,49.9868005360065,50.9865365467266,51.3843375509517),
 .UNSPECIFIED.);
#1783=B_SPLINE_CURVE_WITH_KNOTS('',3,(#225988,#225989,#225990,#225991,#225992,
#225993,#225994,#225995,#225996,#225997,#225998),.UNSPECIFIED.,.F.,.F.,
(4,1,1,1,1,1,1,1,4),(38.8179669365925,38.9897044180849,39.9894404288051,
40.9891764395252,41.9889124502454,42.9886484609655,43.9883844716856,44.9881204824058,
45.1011522437721),.UNSPECIFIED.);
#1784=B_SPLINE_CURVE_WITH_KNOTS('',3,(#226000,#226001,#226002,#226003,#226004,
#226005,#226006,#226007,#226008,#226009),.UNSPECIFIED.,.F.,.F.,(4,1,1,1,
1,1,1,4),(32.534781629413,32.9912883537643,33.9910243644844,34.9907603752045,
35.9904963859246,36.9902323966447,37.9899684073648,38.8179669365925),
 .UNSPECIFIED.);
#1785=B_SPLINE_CURVE_WITH_KNOTS('',3,(#226011,#226012,#226013,#226014,#226015,
#226016,#226017,#226018,#226019,#226020),.UNSPECIFIED.,.F.,.F.,(4,1,1,1,
1,1,1,4),(26.2515963222334,26.9928722894435,27.9926083001636,28.9923443108837,
29.9920803216039,30.991816332324,31.9915523430441,32.534781629413),
 .UNSPECIFIED.);
#1786=B_SPLINE_CURVE_WITH_KNOTS('',3,(#226022,#226023,#226024,#226025,#226026,
#226027,#226028,#226029,#226030,#226031,#226032,#226033),.UNSPECIFIED.,
 .F.,.F.,(4,2,1,1,1,1,1,1,4),(19.9684110150538,19.9947202144025,20.9944562251227,
21.9941922358428,22.9939282465629,23.9936642572831,24.9934002680032,25.9931362787233,
26.2515963222334),.UNSPECIFIED.);
#1787=B_SPLINE_CURVE_WITH_KNOTS('',3,(#226035,#226036,#226037,#226038,#226039,
#226040,#226041,#226042,#226043,#226044,#226045,#226046,#226047,#226048,
#226049,#226050,#226051,#226052,#226053,#226054,#226055,#226056,#226057,
#226058,#226059,#226060,#226061,#226062,#226063,#226064,#226065,#226066,
#226067,#226068,#226069,#226070,#226071,#226072,#226073,#226074,#226075,
#226076,#226077,#226078,#226079,#226080,#226081,#226082,#226083,#226084,
#226085,#226086,#226087,#226088,#226089,#226090,#226091,#226092,#226093,
#226094,#226095,#226096,#226097,#226098,#226099,#226100,#226101,#226102,
#226103,#226104,#226105,#226106,#226107,#226108,#226109,#226110,#226111,
#226112,#226113,#226114,#226115,#226116,#226117,#226118,#226119,#226120,
#226121,#226122,#226123,#226124,#226125,#226126,#226127,#226128,#226129,
#226130,#226131,#226132,#226133,#226134,#226135,#226136,#226137,#226138,
#226139,#226140,#226141,#226142,#226143,#226144,#226145,#226146,#226147,
#226148,#226149,#226150,#226151,#226152,#226153,#226154,#226155,#226156,
#226157,#226158,#226159,#226160,#226161,#226162,#226163,#226164,#226165,
#226166,#226167,#226168,#226169,#226170,#226171,#226172,#226173,#226174,
#226175,#226176,#226177,#226178,#226179,#226180,#226181,#226182,#226183,
#226184,#226185,#226186,#226187,#226188,#226189,#226190,#226191,#226192,
#226193,#226194,#226195,#226196,#226197,#226198,#226199,#226200,#226201,
#226202,#226203,#226204,#226205,#226206,#226207,#226208,#226209,#226210,
#226211,#226212,#226213,#226214,#226215,#226216,#226217,#226218,#226219,
#226220,#226221,#226222,#226223,#226224,#226225,#226226,#226227,#226228,
#226229,#226230,#226231,#226232,#226233,#226234,#226235,#226236,#226237,
#226238,#226239,#226240,#226241,#226242,#226243,#226244,#226245,#226246,
#226247,#226248,#226249,#226250,#226251,#226252,#226253,#226254,#226255,
#226256,#226257,#226258,#226259,#226260,#226261,#226262,#226263,#226264,
#226265,#226266,#226267,#226268,#226269,#226270,#226271,#226272,#226273,
#226274,#226275,#226276,#226277,#226278,#226279,#226280,#226281),
 .UNSPECIFIED.,.F.,.F.,(4,3,3,3,3,3,3,3,3,3,3,3,3,3,3,3,3,3,3,3,3,3,3,3,
3,3,3,3,3,3,3,3,3,3,3,3,3,3,3,3,3,3,3,3,3,3,3,3,3,3,3,3,3,3,3,3,3,3,3,3,
3,3,3,3,3,3,3,3,3,3,3,3,3,3,3,3,3,3,3,3,3,3,4),(13.6852259127505,13.7801099435782,
13.8756905427146,13.9720376507108,13.9963041500819,14.0762611679736,14.1561236791645,
14.2359092120701,14.3156352344774,14.3953191670501,14.4749898540935,14.5546570063244,
14.6343363539807,14.7140436316013,14.7938385549703,14.8736825899846,14.9536407114316,
14.996040160802,15.0759975957193,15.1558605290186,15.2356464886784,15.3153729420553,
15.3950573093886,15.4747284354873,15.5543960293979,15.6340758209858,15.7137835444186,
15.7935789142272,15.8734233967061,15.9533819633687,15.9957761715221,16.075733473648,
16.1555962732271,16.2353820983737,16.3151084165785,16.3947926482139,16.4744636382654,
16.5541310959256,16.6338107511781,16.7135183383086,16.7933135725563,16.873157919691,
16.9531163525208,16.9955121822422,17.0754694434268,17.1553322011706,17.2351179836328,
17.314844258348,17.3945284457316,17.4741993905267,17.5538668023107,17.633546411104,
17.713253951229,17.7930491378706,17.8728934369877,17.9528518215654,17.9952481929623,
18.0752055148322,18.1550683340336,18.2348541786619,18.3145805161891,18.3942647669683,
18.4739357758324,18.5536032520972,18.6332829257289,18.7129905309957,18.7927857829151,
18.8726301474848,18.9525885972255,18.9949842036824,19.0745911127166,19.1541037254495,
19.2335398970435,19.3129174188851,19.3948541184062,19.4741786590968,19.5535018339292,
19.6328396635326,19.7122081748832,19.7916638055052,19.8711715970075,19.9507856857916,
19.9684110150538),.UNSPECIFIED.);
#1788=B_SPLINE_CURVE_WITH_KNOTS('',3,(#226283,#226284,#226285,#226286,#226287,
#226288,#226289,#226290),.UNSPECIFIED.,.F.,.F.,(4,1,1,1,1,4),(9.69384021421591,
9.99736010720132,10.9970961179215,11.9968321286416,12.9965681393618,13.6852257078742),
 .UNSPECIFIED.);
#1789=B_SPLINE_CURVE_WITH_KNOTS('',3,(#226291,#226292,#226293,#226294),
 .UNSPECIFIED.,.F.,.F.,(4,4),(2.11499176853536,2.21729342848466),
 .UNSPECIFIED.);
#1790=B_SPLINE_CURVE_WITH_KNOTS('',3,(#226297,#226298,#226299,#226300),
 .UNSPECIFIED.,.F.,.F.,(4,4),(0.680042556218447,0.864704436494292),
 .UNSPECIFIED.);
#1791=B_SPLINE_CURVE_WITH_KNOTS('',3,(#226302,#226303,#226304,#226305,#226306,
#226307),.UNSPECIFIED.,.F.,.F.,(4,2,4),(1.08095347481491,1.12724697765872,
1.29160843392453),.UNSPECIFIED.);
#1792=B_SPLINE_CURVE_WITH_KNOTS('',3,(#226309,#226310,#226311,#226312),
 .UNSPECIFIED.,.F.,.F.,(4,4),(7.40204040069455,7.71374059257392),
 .UNSPECIFIED.);
#1793=B_SPLINE_CURVE_WITH_KNOTS('',3,(#226313,#226314,#226315,#226316),
 .UNSPECIFIED.,.F.,.F.,(4,4),(7.33678677271359,7.40204018020966),
 .UNSPECIFIED.);
#1794=B_SPLINE_CURVE_WITH_KNOTS('',3,(#233097,#233098,#233099,#233100,#233101,
#233102,#233103,#233104,#233105,#233106,#233107,#233108,#233109,#233110,
#233111,#233112,#233113,#233114,#233115,#233116,#233117,#233118,#233119,
#233120,#233121,#233122),.UNSPECIFIED.,.F.,.F.,(4,2,2,2,2,2,2,2,2,2,2,2,
4),(0.00142388210668726,0.102461957337261,0.113522908460601,0.113690938992141,
0.113757861101401,0.113798818001596,0.113835523929253,0.113882073960433,
0.113974496333833,0.114650839173592,0.121077466272109,0.143151309422213,
0.224602262057577),.UNSPECIFIED.);
#1795=B_SPLINE_CURVE_WITH_KNOTS('',3,(#233126,#233127,#233128,#233129,#233130,
#233131,#233132,#233133),.UNSPECIFIED.,.F.,.F.,(4,2,2,4),(2.33046280664109,
2.42727660829376,2.61395533624592,2.74540526220401),.UNSPECIFIED.);
#1796=B_SPLINE_CURVE_WITH_KNOTS('',3,(#233135,#233136,#233137,#233138,#233139,
#233140,#233141,#233142),.UNSPECIFIED.,.F.,.F.,(4,2,2,4),(2.00538747380151,
2.05391915238944,2.2405978803416,2.32226381429565),.UNSPECIFIED.);
#1797=B_SPLINE_CURVE_WITH_KNOTS('',3,(#233143,#233144,#233145,#233146,#233147,
#233148,#233149,#233150,#233151,#233152,#233153,#233154,#233155,#233156,
#233157,#233158,#233159,#233160,#233161,#233162,#233163,#233164,#233165,
#233166,#233167,#233168,#233169,#233170,#233171,#233172,#233173,#233174,
#233175,#233176,#233177,#233178,#233179,#233180,#233181,#233182,#233183,
#233184,#233185,#233186,#233187,#233188,#233189,#233190,#233191,#233192,
#233193,#233194,#233195,#233196,#233197,#233198,#233199,#233200,#233201,
#233202,#233203),.UNSPECIFIED.,.F.,.F.,(4,3,3,3,3,3,3,3,3,3,3,3,3,3,3,3,
3,3,3,3,4),(18.355181505216,18.4388551554013,18.5224381182464,18.6059504780618,
18.6930840414458,18.7765257696782,18.8599620560646,18.9434109684692,19.0268905791748,
19.1104642874994,19.1940933848967,19.277841130172,19.3030189851341,19.3867448283189,
19.4703731737785,19.5539222575379,19.6374102562577,19.7208568886211,19.804280273106,
19.8877082391123,19.907870678554),.UNSPECIFIED.);
#1798=B_SPLINE_CURVE_WITH_KNOTS('',3,(#233206,#233207,#233208,#233209),
 .UNSPECIFIED.,.F.,.F.,(4,4),(2.29240291271631,2.39658298756549),
 .UNSPECIFIED.);
#1799=B_SPLINE_CURVE_WITH_KNOTS('',3,(#233211,#233212,#233213,#233214),
 .UNSPECIFIED.,.F.,.F.,(4,4),(114.216190622748,114.937428679585),
 .UNSPECIFIED.);
#1800=B_SPLINE_CURVE_WITH_KNOTS('',3,(#233216,#233217,#233218,#233219,#233220,
#233221,#233222,#233223,#233224,#233225,#233226,#233227,#233228,#233229,
#233230,#233231,#233232,#233233,#233234,#233235,#233236,#233237,#233238,
#233239,#233240,#233241,#233242,#233243,#233244,#233245,#233246,#233247,
#233248,#233249,#233250,#233251,#233252,#233253,#233254,#233255,#233256,
#233257,#233258,#233259,#233260,#233261,#233262,#233263,#233264),
 .UNSPECIFIED.,.F.,.F.,(4,3,3,3,3,3,3,3,3,3,3,3,3,3,3,3,4),(112.983899304452,
113.06383913655,113.143687478933,113.223461848315,113.303179703167,113.386520393033,
113.466189271689,113.545858040054,113.625542428248,113.705258172749,113.785062875852,
113.864919771647,113.944886163636,113.969905222095,114.075449330658,114.178641043672,
114.216190536642),.UNSPECIFIED.);
#1801=B_SPLINE_CURVE_WITH_KNOTS('',3,(#233265,#233266,#233267,#233268,#233269,
#233270),.UNSPECIFIED.,.F.,.F.,(4,2,4),(3.21716342272831,3.38194136709993,
3.40990698571987),.UNSPECIFIED.);
#1802=B_SPLINE_CURVE_WITH_KNOTS('',3,(#233273,#233274,#233275,#233276,#233277,
#233278,#233279,#233280,#233281,#233282),.UNSPECIFIED.,.F.,.F.,(4,3,3,4),
(21.7400988072349,21.8231667809187,21.907157678014,21.9911485751093),
 .UNSPECIFIED.);
#1803=B_SPLINE_CURVE_WITH_KNOTS('',3,(#233283,#233284,#233285,#233286,#233287,
#233288,#233289,#233290,#233291,#233292,#233293,#233294,#233295,#233296,
#233297,#233298,#233299,#233300,#233301,#233302,#233303,#233304,#233305,
#233306,#233307,#233308,#233309,#233310,#233311,#233312,#233313,#233314,
#233315,#233316,#233317,#233318,#233319,#233320,#233321,#233322,#233323,
#233324,#233325,#233326,#233327,#233328,#233329,#233330,#233331,#233332,
#233333,#233334,#233335,#233336,#233337,#233338,#233339,#233340,#233341,
#233342,#233343,#233344,#233345,#233346,#233347,#233348,#233349,#233350,
#233351,#233352,#233353,#233354,#233355,#233356,#233357,#233358,#233359,
#233360,#233361,#233362,#233363,#233364,#233365,#233366,#233367,#233368,
#233369,#233370,#233371,#233372,#233373,#233374,#233375,#233376,#233377,
#233378,#233379,#233380,#233381,#233382,#233383,#233384,#233385,#233386,
#233387,#233388,#233389,#233390,#233391,#233392,#233393,#233394,#233395,
#233396,#233397,#233398,#233399,#233400,#233401,#233402,#233403,#233404,
#233405,#233406,#233407,#233408,#233409,#233410,#233411,#233412,#233413,
#233414,#233415,#233416,#233417,#233418,#233419,#233420,#233421,#233422,
#233423,#233424,#233425,#233426,#233427,#233428,#233429,#233430,#233431,
#233432,#233433,#233434,#233435,#233436,#233437,#233438,#233439,#233440,
#233441,#233442,#233443,#233444,#233445,#233446,#233447,#233448,#233449,
#233450,#233451,#233452,#233453,#233454,#233455,#233456,#233457,#233458,
#233459,#233460,#233461,#233462,#233463,#233464,#233465,#233466,#233467,
#233468,#233469,#233470,#233471,#233472,#233473,#233474,#233475,#233476,
#233477,#233478,#233479,#233480,#233481,#233482,#233483,#233484,#233485,
#233486,#233487,#233488,#233489,#233490,#233491,#233492,#233493,#233494,
#233495,#233496,#233497,#233498,#233499,#233500,#233501,#233502),
 .UNSPECIFIED.,.F.,.F.,(4,3,3,3,3,3,3,3,3,3,3,3,3,3,3,3,3,3,3,3,3,3,3,3,
3,3,3,3,3,3,3,3,3,3,3,3,3,3,3,3,3,3,3,3,3,3,3,3,3,3,3,3,3,3,3,3,3,3,3,3,
3,3,3,3,3,3,3,3,3,3,3,3,3,4),(21.9911485752722,22.0905199443307,22.1906522436346,
22.2915864234119,22.3022270172945,22.3859654335529,22.4696006451592,22.5531527849645,
22.6366419137261,22.7200955530059,22.8035317329769,22.8869685266068,22.9704240034381,
23.0539681767605,23.1375569390688,23.2212798871326,23.3019630280146,23.385701881021,
23.4693375349391,23.5528901221183,23.6363797028221,23.719833799406,23.8032704398822,
23.8867076967894,23.9701636392423,24.0537082792805,24.1372975096405,24.2210209233106,
24.3016990387348,24.3854377526698,24.4690732665012,24.5526257127343,24.6361151517867,
24.7195691061525,24.803005604086,24.8864427182613,24.9698985179291,25.0534430159093,
25.1370321043811,25.2207553778982,25.3014350494549,25.3851737205122,25.4688091904866,
25.5523615919349,25.6358509853249,25.7193048928488,25.8027413432284,25.8861784091806,
25.9696341599982,26.0531786084049,26.1367676468314,26.2204908699956,26.301171060175,
26.3849097947876,26.4685453291628,26.5520977957841,26.6355872550472,26.7190412292786,
26.8024777468644,26.8859148804588,26.9693706992928,27.052915215926,27.1365043228015,
27.2202276141041,27.3009070708951,27.3842944828408,27.4675500501445,27.550729511587,
27.633851366961,27.7169340711784,27.8000126126222,27.8830868940955,27.9662056561429,
28.0225858316167),.UNSPECIFIED.);
#1804=B_SPLINE_CURVE_WITH_KNOTS('',3,(#240284,#240285,#240286,#240287,#240288,
#240289,#240290,#240291,#240292,#240293,#240294,#240295),.UNSPECIFIED.,
 .F.,.F.,(4,2,2,2,2,4),(6.24097663211903E-6,0.021580083937109,0.110840866786185,
0.217918405967283,0.317351591624377,0.326345639146483),.UNSPECIFIED.);
#1805=B_SPLINE_CURVE_WITH_KNOTS('',3,(#240296,#240297,#240298,#240299,#240300,
#240301,#240302,#240303,#240304,#240305,#240306,#240307,#240308,#240309,
#240310,#240311,#240312,#240313,#240314,#240315,#240316,#240317,#240318,
#240319,#240320,#240321,#240322,#240323,#240324,#240325,#240326,#240327,
#240328,#240329,#240330,#240331,#240332,#240333,#240334,#240335),
 .UNSPECIFIED.,.F.,.F.,(4,2,2,2,2,2,2,2,2,2,2,2,2,2,2,2,2,2,2,4),(0.00239488436222245,
0.102201826640357,0.181209549188827,0.193475035579474,0.193971074266331,
0.194663958026065,0.195057404656709,0.19519989369731,0.195235582116475,
0.195270182708239,0.19528749027832,0.195301045811009,0.195315937093886,
0.195340101780065,0.19542079041973,0.199626232853206,0.219414959447415,
0.256408927732008,0.309909372043629,0.350021811302258),.UNSPECIFIED.);
#1806=B_SPLINE_CURVE_WITH_KNOTS('',3,(#240336,#240337,#240338,#240339,#240340,
#240341,#240342,#240343,#240344,#240345),.UNSPECIFIED.,.F.,.F.,(4,2,2,2,
4),(0.000659999465871507,0.0472322359860498,0.0984434332088515,0.155288380275565,
0.220269663386073),.UNSPECIFIED.);
#1807=B_SPLINE_CURVE_WITH_KNOTS('',3,(#240346,#240347,#240348,#240349,#240350,
#240351,#240352,#240353,#240354,#240355,#240356,#240357,#240358,#240359,
#240360,#240361,#240362,#240363,#240364,#240365,#240366,#240367,#240368,
#240369,#240370,#240371,#240372,#240373,#240374,#240375),.UNSPECIFIED.,
 .F.,.F.,(4,2,2,2,2,2,2,2,2,2,2,2,2,2,4),(0.0120072812196319,0.124651425623479,
0.129299183636369,0.137626079649342,0.137766129259384,0.138318251653115,
0.138447846329851,0.138519129454569,0.138578433547788,0.138648094876172,
0.138770572390779,0.139302371484231,0.149636581332025,0.170304854177609,
0.277058970671051),.UNSPECIFIED.);
#1808=B_SPLINE_CURVE_WITH_KNOTS('',3,(#240376,#240377,#240378,#240379,#240380,
#240381,#240382,#240383,#240384,#240385,#240386,#240387,#240388,#240389,
#240390,#240391,#240392,#240393,#240394,#240395,#240396,#240397,#240398,
#240399,#240400,#240401,#240402,#240403,#240404,#240405,#240406,#240407,
#240408,#240409,#240410,#240411,#240412,#240413,#240414,#240415,#240416,
#240417,#240418,#240419,#240420,#240421,#240422,#240423,#240424,#240425,
#240426,#240427,#240428,#240429,#240430,#240431,#240432,#240433,#240434,
#240435,#240436,#240437,#240438,#240439,#240440,#240441),.UNSPECIFIED.,
 .F.,.F.,(4,2,2,2,2,2,2,2,2,2,2,2,2,2,2,2,2,2,2,2,2,2,2,2,2,2,2,2,2,2,2,
2,4),(0.326345639146483,0.39717698474622,0.401652761356229,0.402004293626876,
0.402088366886084,0.402134901523776,0.402173777520773,0.402219222079272,
0.402299830966666,0.402652644059501,0.421430642133052,0.478736005391261,
0.57626086556828,0.720833256739961,0.847312020492082,0.931615895673563,
1.06112874522252,1.06509356720185,1.0700343312839,1.07436288411271,1.07465542728212,
1.07475922918139,1.07482626368171,1.07488881226853,1.07497172318178,1.07514950344775,
1.07739277037847,1.10748082532148,1.17423178070239,1.27214718241461,1.40528589051194,
1.50493087009919,1.61754120424573),.UNSPECIFIED.);
#1945=SHAPE_REPRESENTATION_RELATIONSHIP('SRR','None',#279304,#1954);
#1954=ADVANCED_BREP_SHAPE_REPRESENTATION('',(#1972),#279260);
#1963=STYLED_ITEM('',(#279355),#1972);
#1972=MANIFOLD_SOLID_BREP('Body1',#14941);
#1995=FACE_BOUND('',#2957,.T.);
#2061=PLANE('',#15472);
#2062=PLANE('',#15473);
#2443=FACE_OUTER_BOUND('',#2930,.T.);
#2444=FACE_OUTER_BOUND('',#2931,.T.);
#2445=FACE_OUTER_BOUND('',#2932,.T.);
#2446=FACE_OUTER_BOUND('',#2933,.T.);
#2447=FACE_OUTER_BOUND('',#2934,.T.);
#2448=FACE_OUTER_BOUND('',#2935,.T.);
#2449=FACE_OUTER_BOUND('',#2936,.T.);
#2450=FACE_OUTER_BOUND('',#2937,.T.);
#2451=FACE_OUTER_BOUND('',#2938,.T.);
#2452=FACE_OUTER_BOUND('',#2939,.T.);
#2453=FACE_OUTER_BOUND('',#2940,.T.);
#2454=FACE_OUTER_BOUND('',#2941,.T.);
#2455=FACE_OUTER_BOUND('',#2942,.T.);
#2456=FACE_OUTER_BOUND('',#2943,.T.);
#2457=FACE_OUTER_BOUND('',#2944,.T.);
#2458=FACE_OUTER_BOUND('',#2945,.T.);
#2459=FACE_OUTER_BOUND('',#2946,.T.);
#2460=FACE_OUTER_BOUND('',#2947,.T.);
#2461=FACE_OUTER_BOUND('',#2948,.T.);
#2462=FACE_OUTER_BOUND('',#2949,.T.);
#2463=FACE_OUTER_BOUND('',#2950,.T.);
#2464=FACE_OUTER_BOUND('',#2951,.T.);
#2465=FACE_OUTER_BOUND('',#2952,.T.);
#2466=FACE_OUTER_BOUND('',#2953,.T.);
#2467=FACE_OUTER_BOUND('',#2954,.T.);
#2468=FACE_OUTER_BOUND('',#2955,.T.);
#2469=FACE_OUTER_BOUND('',#2956,.T.);
#2470=FACE_OUTER_BOUND('',#2958,.T.);
#2471=FACE_OUTER_BOUND('',#2959,.T.);
#2930=EDGE_LOOP('',(#13064,#13065,#13066,#13067,#13068,#13069));
#2931=EDGE_LOOP('',(#13070,#13071,#13072,#13073,#13074,#13075));
#2932=EDGE_LOOP('',(#13076,#13077,#13078,#13079,#13080,#13081));
#2933=EDGE_LOOP('',(#13082,#13083,#13084,#13085,#13086,#13087));
#2934=EDGE_LOOP('',(#13088,#13089,#13090,#13091,#13092,#13093));
#2935=EDGE_LOOP('',(#13094,#13095,#13096,#13097,#13098,#13099));
#2936=EDGE_LOOP('',(#13100,#13101,#13102,#13103,#13104,#13105));
#2937=EDGE_LOOP('',(#13106,#13107,#13108,#13109,#13110,#13111));
#2938=EDGE_LOOP('',(#13112,#13113,#13114,#13115,#13116,#13117));
#2939=EDGE_LOOP('',(#13118,#13119,#13120,#13121,#13122,#13123));
#2940=EDGE_LOOP('',(#13124,#13125,#13126,#13127,#13128,#13129));
#2941=EDGE_LOOP('',(#13130,#13131,#13132,#13133,#13134,#13135));
#2942=EDGE_LOOP('',(#13136,#13137,#13138,#13139,#13140,#13141));
#2943=EDGE_LOOP('',(#13142,#13143,#13144,#13145,#13146,#13147));
#2944=EDGE_LOOP('',(#13148,#13149,#13150,#13151,#13152,#13153));
#2945=EDGE_LOOP('',(#13154,#13155,#13156,#13157,#13158,#13159));
#2946=EDGE_LOOP('',(#13160,#13161,#13162,#13163));
#2947=EDGE_LOOP('',(#13164,#13165,#13166,#13167,#13168,#13169,#13170,#13171,
#13172,#13173,#13174,#13175,#13176,#13177,#13178,#13179,#13180,#13181,#13182,
#13183,#13184,#13185,#13186,#13187,#13188,#13189,#13190,#13191,#13192,#13193,
#13194,#13195,#13196,#13197,#13198,#13199,#13200,#13201,#13202,#13203,#13204,
#13205,#13206,#13207,#13208,#13209,#13210,#13211,#13212,#13213,#13214,#13215,
#13216,#13217,#13218,#13219,#13220));
#2948=EDGE_LOOP('',(#13221,#13222,#13223,#13224));
#2949=EDGE_LOOP('',(#13225,#13226,#13227,#13228,#13229,#13230,#13231,#13232,
#13233,#13234,#13235,#13236,#13237,#13238,#13239,#13240,#13241,#13242,#13243,
#13244,#13245,#13246,#13247,#13248,#13249,#13250,#13251,#13252,#13253,#13254,
#13255,#13256,#13257,#13258,#13259,#13260));
#2950=EDGE_LOOP('',(#13261,#13262,#13263,#13264,#13265,#13266));
#2951=EDGE_LOOP('',(#13267,#13268,#13269));
#2952=EDGE_LOOP('',(#13270,#13271,#13272));
#2953=EDGE_LOOP('',(#13273,#13274,#13275,#13276,#13277,#13278));
#2954=EDGE_LOOP('',(#13279,#13280,#13281,#13282,#13283,#13284));
#2955=EDGE_LOOP('',(#13285,#13286,#13287,#13288,#13289,#13290,#13291,#13292,
#13293,#13294,#13295,#13296,#13297,#13298,#13299,#13300,#13301,#13302,#13303,
#13304,#13305,#13306,#13307,#13308,#13309,#13310,#13311,#13312,#13313,#13314,
#13315,#13316,#13317,#13318,#13319,#13320,#13321,#13322,#13323,#13324,#13325,
#13326,#13327,#13328,#13329,#13330,#13331,#13332,#13333,#13334,#13335,#13336,
#13337,#13338,#13339,#13340,#13341,#13342,#13343,#13344));
#2956=EDGE_LOOP('',(#13345,#13346,#13347,#13348,#13349,#13350,#13351,#13352,
#13353,#13354,#13355,#13356,#13357,#13358,#13359,#13360));
#2957=EDGE_LOOP('',(#13361,#13362,#13363,#13364,#13365,#13366,#13367,#13368,
#13369,#13370,#13371));
#2958=EDGE_LOOP('',(#13372));
#2959=EDGE_LOOP('',(#13373));
#3460=LINE('',#202536,#3988);
#3461=LINE('',#202857,#3989);
#3462=LINE('',#203323,#3990);
#3463=LINE('',#203789,#3991);
#3464=LINE('',#204255,#3992);
#3465=LINE('',#204718,#3993);
#3466=LINE('',#205184,#3994);
#3467=LINE('',#205650,#3995);
#3468=LINE('',#206110,#3996);
#3469=LINE('',#206363,#3997);
#3470=LINE('',#206619,#3998);
#3471=LINE('',#207085,#3999);
#3472=LINE('',#207548,#4000);
#3473=LINE('',#208014,#4001);
#3474=LINE('',#208480,#4002);
#3475=LINE('',#208946,#4003);
#3476=LINE('',#209415,#4004);
#3477=LINE('',#240445,#4005);
#3478=LINE('',#240447,#4006);
#3988=VECTOR('',#16840,4.91825);
#3989=VECTOR('',#16843,4.91825);
#3990=VECTOR('',#16846,4.91825);
#3991=VECTOR('',#16849,4.91825);
#3992=VECTOR('',#16852,4.91825);
#3993=VECTOR('',#16855,4.91825);
#3994=VECTOR('',#16858,4.91825);
#3995=VECTOR('',#16861,4.91825);
#3996=VECTOR('',#16864,4.91825);
#3997=VECTOR('',#16867,4.91825);
#3998=VECTOR('',#16870,4.91825);
#3999=VECTOR('',#16873,4.91825);
#4000=VECTOR('',#16876,4.91825);
#4001=VECTOR('',#16879,4.91825);
#4002=VECTOR('',#16882,4.91825);
#4003=VECTOR('',#16885,4.91825);
#4004=VECTOR('',#16888,4.91825);
#4005=VECTOR('',#16903,15.2420394990918);
#4006=VECTOR('',#16904,15.2420394990918);
#4216=CIRCLE('',#15470,15.2420394990918);
#4217=CIRCLE('',#15471,15.2420394990918);
#6022=VERTEX_POINT('',#202534);
#6023=VERTEX_POINT('',#202535);
#6024=VERTEX_POINT('',#202537);
#6025=VERTEX_POINT('',#202551);
#6026=VERTEX_POINT('',#202688);
#6027=VERTEX_POINT('',#202695);
#6028=VERTEX_POINT('',#202855);
#6029=VERTEX_POINT('',#202856);
#6030=VERTEX_POINT('',#202858);
#6031=VERTEX_POINT('',#203089);
#6032=VERTEX_POINT('',#203321);
#6033=VERTEX_POINT('',#203322);
#6034=VERTEX_POINT('',#203324);
#6035=VERTEX_POINT('',#203555);
#6036=VERTEX_POINT('',#203787);
#6037=VERTEX_POINT('',#203788);
#6038=VERTEX_POINT('',#203790);
#6039=VERTEX_POINT('',#204021);
#6040=VERTEX_POINT('',#204253);
#6041=VERTEX_POINT('',#204254);
#6042=VERTEX_POINT('',#204256);
#6043=VERTEX_POINT('',#204487);
#6044=VERTEX_POINT('',#204716);
#6045=VERTEX_POINT('',#204717);
#6046=VERTEX_POINT('',#204719);
#6047=VERTEX_POINT('',#204950);
#6048=VERTEX_POINT('',#205182);
#6049=VERTEX_POINT('',#205183);
#6050=VERTEX_POINT('',#205185);
#6051=VERTEX_POINT('',#205416);
#6052=VERTEX_POINT('',#205648);
#6053=VERTEX_POINT('',#205649);
#6054=VERTEX_POINT('',#205651);
#6055=VERTEX_POINT('',#205882);
#6056=VERTEX_POINT('',#206108);
#6057=VERTEX_POINT('',#206109);
#6058=VERTEX_POINT('',#206111);
#6059=VERTEX_POINT('',#206345);
#6060=VERTEX_POINT('',#206361);
#6061=VERTEX_POINT('',#206362);
#6062=VERTEX_POINT('',#206364);
#6063=VERTEX_POINT('',#206595);
#6064=VERTEX_POINT('',#206617);
#6065=VERTEX_POINT('',#206618);
#6066=VERTEX_POINT('',#206620);
#6067=VERTEX_POINT('',#206851);
#6068=VERTEX_POINT('',#207083);
#6069=VERTEX_POINT('',#207084);
#6070=VERTEX_POINT('',#207086);
#6071=VERTEX_POINT('',#207317);
#6072=VERTEX_POINT('',#207546);
#6073=VERTEX_POINT('',#207547);
#6074=VERTEX_POINT('',#207549);
#6075=VERTEX_POINT('',#207780);
#6076=VERTEX_POINT('',#208012);
#6077=VERTEX_POINT('',#208013);
#6078=VERTEX_POINT('',#208015);
#6079=VERTEX_POINT('',#208243);
#6080=VERTEX_POINT('',#208478);
#6081=VERTEX_POINT('',#208479);
#6082=VERTEX_POINT('',#208481);
#6083=VERTEX_POINT('',#208712);
#6084=VERTEX_POINT('',#208944);
#6085=VERTEX_POINT('',#208945);
#6086=VERTEX_POINT('',#208947);
#6087=VERTEX_POINT('',#209181);
#6088=VERTEX_POINT('',#209413);
#6089=VERTEX_POINT('',#209414);
#6090=VERTEX_POINT('',#209416);
#6091=VERTEX_POINT('',#209448);
#6092=VERTEX_POINT('',#216281);
#6093=VERTEX_POINT('',#216292);
#6094=VERTEX_POINT('',#216302);
#6095=VERTEX_POINT('',#216547);
#6096=VERTEX_POINT('',#216558);
#6097=VERTEX_POINT('',#216569);
#6098=VERTEX_POINT('',#216581);
#6099=VERTEX_POINT('',#216826);
#6100=VERTEX_POINT('',#217071);
#6101=VERTEX_POINT('',#217083);
#6102=VERTEX_POINT('',#217328);
#6103=VERTEX_POINT('',#217576);
#6104=VERTEX_POINT('',#217587);
#6105=VERTEX_POINT('',#217832);
#6106=VERTEX_POINT('',#217843);
#6107=VERTEX_POINT('',#217854);
#6108=VERTEX_POINT('',#217866);
#6109=VERTEX_POINT('',#217877);
#6110=VERTEX_POINT('',#218044);
#6111=VERTEX_POINT('',#218081);
#6112=VERTEX_POINT('',#218110);
#6113=VERTEX_POINT('',#218126);
#6114=VERTEX_POINT('',#225137);
#6115=VERTEX_POINT('',#225138);
#6116=VERTEX_POINT('',#225149);
#6117=VERTEX_POINT('',#225172);
#6118=VERTEX_POINT('',#225213);
#6119=VERTEX_POINT('',#225220);
#6120=VERTEX_POINT('',#225402);
#6121=VERTEX_POINT('',#225413);
#6122=VERTEX_POINT('',#225424);
#6123=VERTEX_POINT('',#225435);
#6124=VERTEX_POINT('',#225447);
#6125=VERTEX_POINT('',#225695);
#6126=VERTEX_POINT('',#225706);
#6127=VERTEX_POINT('',#225954);
#6128=VERTEX_POINT('',#225965);
#6129=VERTEX_POINT('',#225976);
#6130=VERTEX_POINT('',#225987);
#6131=VERTEX_POINT('',#225999);
#6132=VERTEX_POINT('',#226010);
#6133=VERTEX_POINT('',#226021);
#6134=VERTEX_POINT('',#226034);
#6135=VERTEX_POINT('',#226282);
#6136=VERTEX_POINT('',#226296);
#6137=VERTEX_POINT('',#226301);
#6138=VERTEX_POINT('',#226308);
#6139=VERTEX_POINT('',#233124);
#6140=VERTEX_POINT('',#233125);
#6141=VERTEX_POINT('',#233134);
#6142=VERTEX_POINT('',#233205);
#6143=VERTEX_POINT('',#233210);
#6144=VERTEX_POINT('',#233215);
#6145=VERTEX_POINT('',#233272);
#6146=VERTEX_POINT('',#240283);
#6147=VERTEX_POINT('',#240443);
#6148=VERTEX_POINT('',#240446);
#8457=EDGE_CURVE('',#6022,#6023,#3460,.T.);
#8458=EDGE_CURVE('',#6023,#6024,#1675,.T.);
#8459=EDGE_CURVE('',#6024,#6025,#1676,.T.);
#8460=EDGE_CURVE('',#6026,#6025,#1677,.T.);
#8461=EDGE_CURVE('',#6027,#6026,#1678,.T.);
#8462=EDGE_CURVE('',#6022,#6027,#1679,.T.);
#8463=EDGE_CURVE('',#6028,#6029,#3461,.T.);
#8464=EDGE_CURVE('',#6029,#6030,#1680,.T.);
#8465=EDGE_CURVE('',#6030,#6023,#1681,.T.);
#8466=EDGE_CURVE('',#6031,#6022,#1682,.T.);
#8467=EDGE_CURVE('',#6028,#6031,#1683,.T.);
#8468=EDGE_CURVE('',#6032,#6033,#3462,.T.);
#8469=EDGE_CURVE('',#6033,#6034,#1684,.T.);
#8470=EDGE_CURVE('',#6034,#6029,#1685,.T.);
#8471=EDGE_CURVE('',#6035,#6028,#1686,.T.);
#8472=EDGE_CURVE('',#6032,#6035,#1687,.T.);
#8473=EDGE_CURVE('',#6036,#6037,#3463,.T.);
#8474=EDGE_CURVE('',#6037,#6038,#1688,.T.);
#8475=EDGE_CURVE('',#6038,#6033,#1689,.T.);
#8476=EDGE_CURVE('',#6039,#6032,#1690,.T.);
#8477=EDGE_CURVE('',#6036,#6039,#1691,.T.);
#8478=EDGE_CURVE('',#6040,#6041,#3464,.T.);
#8479=EDGE_CURVE('',#6041,#6042,#1692,.T.);
#8480=EDGE_CURVE('',#6042,#6037,#1693,.T.);
#8481=EDGE_CURVE('',#6043,#6036,#1694,.T.);
#8482=EDGE_CURVE('',#6040,#6043,#1695,.T.);
#8483=EDGE_CURVE('',#6044,#6045,#3465,.T.);
#8484=EDGE_CURVE('',#6045,#6046,#1696,.T.);
#8485=EDGE_CURVE('',#6046,#6041,#1697,.T.);
#8486=EDGE_CURVE('',#6047,#6040,#1698,.T.);
#8487=EDGE_CURVE('',#6044,#6047,#1699,.T.);
#8488=EDGE_CURVE('',#6048,#6049,#3466,.T.);
#8489=EDGE_CURVE('',#6049,#6050,#1700,.T.);
#8490=EDGE_CURVE('',#6050,#6045,#1701,.T.);
#8491=EDGE_CURVE('',#6051,#6044,#1702,.T.);
#8492=EDGE_CURVE('',#6048,#6051,#1703,.T.);
#8493=EDGE_CURVE('',#6052,#6053,#3467,.T.);
#8494=EDGE_CURVE('',#6053,#6054,#1704,.T.);
#8495=EDGE_CURVE('',#6054,#6049,#1705,.T.);
#8496=EDGE_CURVE('',#6055,#6048,#1706,.T.);
#8497=EDGE_CURVE('',#6052,#6055,#1707,.T.);
#8498=EDGE_CURVE('',#6056,#6057,#3468,.T.);
#8499=EDGE_CURVE('',#6057,#6058,#1708,.T.);
#8500=EDGE_CURVE('',#6058,#6053,#1709,.T.);
#8501=EDGE_CURVE('',#6059,#6052,#1710,.T.);
#8502=EDGE_CURVE('',#6056,#6059,#1711,.T.);
#8503=EDGE_CURVE('',#6060,#6061,#3469,.T.);
#8504=EDGE_CURVE('',#6061,#6062,#1712,.T.);
#8505=EDGE_CURVE('',#6062,#6057,#1713,.T.);
#8506=EDGE_CURVE('',#6063,#6056,#1714,.T.);
#8507=EDGE_CURVE('',#6060,#6063,#1715,.T.);
#8508=EDGE_CURVE('',#6064,#6065,#3470,.T.);
#8509=EDGE_CURVE('',#6065,#6066,#1716,.T.);
#8510=EDGE_CURVE('',#6066,#6061,#1717,.T.);
#8511=EDGE_CURVE('',#6067,#6060,#1718,.T.);
#8512=EDGE_CURVE('',#6064,#6067,#1719,.T.);
#8513=EDGE_CURVE('',#6068,#6069,#3471,.T.);
#8514=EDGE_CURVE('',#6069,#6070,#1720,.T.);
#8515=EDGE_CURVE('',#6070,#6065,#1721,.T.);
#8516=EDGE_CURVE('',#6071,#6064,#1722,.T.);
#8517=EDGE_CURVE('',#6068,#6071,#1723,.T.);
#8518=EDGE_CURVE('',#6072,#6073,#3472,.T.);
#8519=EDGE_CURVE('',#6073,#6074,#1724,.T.);
#8520=EDGE_CURVE('',#6074,#6069,#1725,.T.);
#8521=EDGE_CURVE('',#6075,#6068,#1726,.T.);
#8522=EDGE_CURVE('',#6072,#6075,#1727,.T.);
#8523=EDGE_CURVE('',#6076,#6077,#3473,.T.);
#8524=EDGE_CURVE('',#6077,#6078,#1728,.T.);
#8525=EDGE_CURVE('',#6078,#6073,#1729,.T.);
#8526=EDGE_CURVE('',#6079,#6072,#1730,.T.);
#8527=EDGE_CURVE('',#6076,#6079,#1731,.T.);
#8528=EDGE_CURVE('',#6080,#6081,#3474,.T.);
#8529=EDGE_CURVE('',#6081,#6082,#1732,.T.);
#8530=EDGE_CURVE('',#6082,#6077,#1733,.T.);
#8531=EDGE_CURVE('',#6083,#6076,#1734,.T.);
#8532=EDGE_CURVE('',#6080,#6083,#1735,.T.);
#8533=EDGE_CURVE('',#6084,#6085,#3475,.T.);
#8534=EDGE_CURVE('',#6085,#6086,#1736,.T.);
#8535=EDGE_CURVE('',#6086,#6081,#1737,.T.);
#8536=EDGE_CURVE('',#6087,#6080,#1738,.T.);
#8537=EDGE_CURVE('',#6084,#6087,#1739,.T.);
#8538=EDGE_CURVE('',#6088,#6089,#3476,.T.);
#8539=EDGE_CURVE('',#6090,#6088,#1740,.T.);
#8540=EDGE_CURVE('',#6091,#6090,#1741,.T.);
#8541=EDGE_CURVE('',#6091,#6089,#1742,.T.);
#8542=EDGE_CURVE('',#6092,#6026,#1743,.T.);
#8543=EDGE_CURVE('',#6092,#6093,#1744,.T.);
#8544=EDGE_CURVE('',#6093,#6094,#1745,.T.);
#8545=EDGE_CURVE('',#6094,#6095,#1746,.T.);
#8546=EDGE_CURVE('',#6095,#6096,#1747,.T.);
#8547=EDGE_CURVE('',#6096,#6097,#1748,.T.);
#8548=EDGE_CURVE('',#6097,#6098,#1749,.T.);
#8549=EDGE_CURVE('',#6098,#6099,#1750,.T.);
#8550=EDGE_CURVE('',#6099,#6100,#1751,.T.);
#8551=EDGE_CURVE('',#6100,#6101,#1752,.T.);
#8552=EDGE_CURVE('',#6101,#6102,#1753,.T.);
#8553=EDGE_CURVE('',#6102,#6103,#1754,.T.);
#8554=EDGE_CURVE('',#6103,#6104,#1755,.T.);
#8555=EDGE_CURVE('',#6104,#6105,#1756,.T.);
#8556=EDGE_CURVE('',#6105,#6106,#1757,.T.);
#8557=EDGE_CURVE('',#6106,#6107,#1758,.T.);
#8558=EDGE_CURVE('',#6107,#6108,#1759,.T.);
#8559=EDGE_CURVE('',#6108,#6109,#1760,.T.);
#8560=EDGE_CURVE('',#6110,#6109,#1761,.T.);
#8561=EDGE_CURVE('',#6110,#6111,#1762,.T.);
#8562=EDGE_CURVE('',#6111,#6112,#1763,.T.);
#8563=EDGE_CURVE('',#6090,#6112,#1764,.T.);
#8564=EDGE_CURVE('',#6088,#6113,#1765,.T.);
#8565=EDGE_CURVE('',#6113,#6084,#1766,.T.);
#8566=EDGE_CURVE('',#6114,#6115,#1767,.T.);
#8567=EDGE_CURVE('',#6114,#6116,#1768,.T.);
#8568=EDGE_CURVE('',#6116,#6117,#1769,.T.);
#8569=EDGE_CURVE('',#6115,#6117,#1770,.T.);
#8570=EDGE_CURVE('',#6118,#6092,#1771,.T.);
#8571=EDGE_CURVE('',#6119,#6118,#1772,.T.);
#8572=EDGE_CURVE('',#6120,#6119,#1773,.T.);
#8573=EDGE_CURVE('',#6121,#6120,#1774,.T.);
#8574=EDGE_CURVE('',#6122,#6121,#1775,.T.);
#8575=EDGE_CURVE('',#6123,#6122,#1776,.T.);
#8576=EDGE_CURVE('',#6124,#6123,#1777,.T.);
#8577=EDGE_CURVE('',#6125,#6124,#1778,.T.);
#8578=EDGE_CURVE('',#6126,#6125,#1779,.T.);
#8579=EDGE_CURVE('',#6127,#6126,#1780,.T.);
#8580=EDGE_CURVE('',#6128,#6127,#1781,.T.);
#8581=EDGE_CURVE('',#6129,#6128,#1782,.T.);
#8582=EDGE_CURVE('',#6130,#6129,#1783,.T.);
#8583=EDGE_CURVE('',#6131,#6130,#1784,.T.);
#8584=EDGE_CURVE('',#6132,#6131,#1785,.T.);
#8585=EDGE_CURVE('',#6133,#6132,#1786,.T.);
#8586=EDGE_CURVE('',#6134,#6133,#1787,.T.);
#8587=EDGE_CURVE('',#6135,#6134,#1788,.T.);
#8588=EDGE_CURVE('',#6109,#6135,#1789,.T.);
#8589=EDGE_CURVE('',#6112,#6136,#1790,.T.);
#8590=EDGE_CURVE('',#6137,#6110,#1791,.T.);
#8591=EDGE_CURVE('',#6138,#6137,#1792,.T.);
#8592=EDGE_CURVE('',#6136,#6138,#1793,.T.);
#8593=EDGE_CURVE('',#6136,#6137,#1794,.T.);
#8594=EDGE_CURVE('',#6139,#6140,#1795,.T.);
#8595=EDGE_CURVE('',#6141,#6139,#1796,.T.);
#8596=EDGE_CURVE('',#6141,#6140,#1797,.T.);
#8597=EDGE_CURVE('',#6142,#6114,#1798,.T.);
#8598=EDGE_CURVE('',#6143,#6142,#1799,.T.);
#8599=EDGE_CURVE('',#6144,#6143,#1800,.T.);
#8600=EDGE_CURVE('',#6117,#6144,#1801,.T.);
#8601=EDGE_CURVE('',#6089,#6145,#1802,.T.);
#8602=EDGE_CURVE('',#6145,#6085,#1803,.T.);
#8603=EDGE_CURVE('',#6025,#6146,#1804,.T.);
#8604=EDGE_CURVE('',#6140,#6091,#1805,.T.);
#8605=EDGE_CURVE('',#6135,#6141,#1806,.T.);
#8606=EDGE_CURVE('',#6144,#6118,#1807,.T.);
#8607=EDGE_CURVE('',#6146,#6142,#1808,.T.);
#8608=EDGE_CURVE('',#6147,#6147,#4216,.T.);
#8609=EDGE_CURVE('',#6147,#6115,#3477,.T.);
#8610=EDGE_CURVE('',#6146,#6148,#3478,.T.);
#8611=EDGE_CURVE('',#6148,#6148,#4217,.T.);
#13064=ORIENTED_EDGE('',*,*,#8457,.T.);
#13065=ORIENTED_EDGE('',*,*,#8458,.T.);
#13066=ORIENTED_EDGE('',*,*,#8459,.T.);
#13067=ORIENTED_EDGE('',*,*,#8460,.F.);
#13068=ORIENTED_EDGE('',*,*,#8461,.F.);
#13069=ORIENTED_EDGE('',*,*,#8462,.F.);
#13070=ORIENTED_EDGE('',*,*,#8463,.T.);
#13071=ORIENTED_EDGE('',*,*,#8464,.T.);
#13072=ORIENTED_EDGE('',*,*,#8465,.T.);
#13073=ORIENTED_EDGE('',*,*,#8457,.F.);
#13074=ORIENTED_EDGE('',*,*,#8466,.F.);
#13075=ORIENTED_EDGE('',*,*,#8467,.F.);
#13076=ORIENTED_EDGE('',*,*,#8468,.T.);
#13077=ORIENTED_EDGE('',*,*,#8469,.T.);
#13078=ORIENTED_EDGE('',*,*,#8470,.T.);
#13079=ORIENTED_EDGE('',*,*,#8463,.F.);
#13080=ORIENTED_EDGE('',*,*,#8471,.F.);
#13081=ORIENTED_EDGE('',*,*,#8472,.F.);
#13082=ORIENTED_EDGE('',*,*,#8473,.T.);
#13083=ORIENTED_EDGE('',*,*,#8474,.T.);
#13084=ORIENTED_EDGE('',*,*,#8475,.T.);
#13085=ORIENTED_EDGE('',*,*,#8468,.F.);
#13086=ORIENTED_EDGE('',*,*,#8476,.F.);
#13087=ORIENTED_EDGE('',*,*,#8477,.F.);
#13088=ORIENTED_EDGE('',*,*,#8478,.T.);
#13089=ORIENTED_EDGE('',*,*,#8479,.T.);
#13090=ORIENTED_EDGE('',*,*,#8480,.T.);
#13091=ORIENTED_EDGE('',*,*,#8473,.F.);
#13092=ORIENTED_EDGE('',*,*,#8481,.F.);
#13093=ORIENTED_EDGE('',*,*,#8482,.F.);
#13094=ORIENTED_EDGE('',*,*,#8483,.T.);
#13095=ORIENTED_EDGE('',*,*,#8484,.T.);
#13096=ORIENTED_EDGE('',*,*,#8485,.T.);
#13097=ORIENTED_EDGE('',*,*,#8478,.F.);
#13098=ORIENTED_EDGE('',*,*,#8486,.F.);
#13099=ORIENTED_EDGE('',*,*,#8487,.F.);
#13100=ORIENTED_EDGE('',*,*,#8488,.T.);
#13101=ORIENTED_EDGE('',*,*,#8489,.T.);
#13102=ORIENTED_EDGE('',*,*,#8490,.T.);
#13103=ORIENTED_EDGE('',*,*,#8483,.F.);
#13104=ORIENTED_EDGE('',*,*,#8491,.F.);
#13105=ORIENTED_EDGE('',*,*,#8492,.F.);
#13106=ORIENTED_EDGE('',*,*,#8493,.T.);
#13107=ORIENTED_EDGE('',*,*,#8494,.T.);
#13108=ORIENTED_EDGE('',*,*,#8495,.T.);
#13109=ORIENTED_EDGE('',*,*,#8488,.F.);
#13110=ORIENTED_EDGE('',*,*,#8496,.F.);
#13111=ORIENTED_EDGE('',*,*,#8497,.F.);
#13112=ORIENTED_EDGE('',*,*,#8498,.T.);
#13113=ORIENTED_EDGE('',*,*,#8499,.T.);
#13114=ORIENTED_EDGE('',*,*,#8500,.T.);
#13115=ORIENTED_EDGE('',*,*,#8493,.F.);
#13116=ORIENTED_EDGE('',*,*,#8501,.F.);
#13117=ORIENTED_EDGE('',*,*,#8502,.F.);
#13118=ORIENTED_EDGE('',*,*,#8503,.T.);
#13119=ORIENTED_EDGE('',*,*,#8504,.T.);
#13120=ORIENTED_EDGE('',*,*,#8505,.T.);
#13121=ORIENTED_EDGE('',*,*,#8498,.F.);
#13122=ORIENTED_EDGE('',*,*,#8506,.F.);
#13123=ORIENTED_EDGE('',*,*,#8507,.F.);
#13124=ORIENTED_EDGE('',*,*,#8508,.T.);
#13125=ORIENTED_EDGE('',*,*,#8509,.T.);
#13126=ORIENTED_EDGE('',*,*,#8510,.T.);
#13127=ORIENTED_EDGE('',*,*,#8503,.F.);
#13128=ORIENTED_EDGE('',*,*,#8511,.F.);
#13129=ORIENTED_EDGE('',*,*,#8512,.F.);
#13130=ORIENTED_EDGE('',*,*,#8513,.T.);
#13131=ORIENTED_EDGE('',*,*,#8514,.T.);
#13132=ORIENTED_EDGE('',*,*,#8515,.T.);
#13133=ORIENTED_EDGE('',*,*,#8508,.F.);
#13134=ORIENTED_EDGE('',*,*,#8516,.F.);
#13135=ORIENTED_EDGE('',*,*,#8517,.F.);
#13136=ORIENTED_EDGE('',*,*,#8518,.T.);
#13137=ORIENTED_EDGE('',*,*,#8519,.T.);
#13138=ORIENTED_EDGE('',*,*,#8520,.T.);
#13139=ORIENTED_EDGE('',*,*,#8513,.F.);
#13140=ORIENTED_EDGE('',*,*,#8521,.F.);
#13141=ORIENTED_EDGE('',*,*,#8522,.F.);
#13142=ORIENTED_EDGE('',*,*,#8523,.T.);
#13143=ORIENTED_EDGE('',*,*,#8524,.T.);
#13144=ORIENTED_EDGE('',*,*,#8525,.T.);
#13145=ORIENTED_EDGE('',*,*,#8518,.F.);
#13146=ORIENTED_EDGE('',*,*,#8526,.F.);
#13147=ORIENTED_EDGE('',*,*,#8527,.F.);
#13148=ORIENTED_EDGE('',*,*,#8528,.T.);
#13149=ORIENTED_EDGE('',*,*,#8529,.T.);
#13150=ORIENTED_EDGE('',*,*,#8530,.T.);
#13151=ORIENTED_EDGE('',*,*,#8523,.F.);
#13152=ORIENTED_EDGE('',*,*,#8531,.F.);
#13153=ORIENTED_EDGE('',*,*,#8532,.F.);
#13154=ORIENTED_EDGE('',*,*,#8533,.T.);
#13155=ORIENTED_EDGE('',*,*,#8534,.T.);
#13156=ORIENTED_EDGE('',*,*,#8535,.T.);
#13157=ORIENTED_EDGE('',*,*,#8528,.F.);
#13158=ORIENTED_EDGE('',*,*,#8536,.F.);
#13159=ORIENTED_EDGE('',*,*,#8537,.F.);
#13160=ORIENTED_EDGE('',*,*,#8538,.F.);
#13161=ORIENTED_EDGE('',*,*,#8539,.F.);
#13162=ORIENTED_EDGE('',*,*,#8540,.F.);
#13163=ORIENTED_EDGE('',*,*,#8541,.T.);
#13164=ORIENTED_EDGE('',*,*,#8542,.F.);
#13165=ORIENTED_EDGE('',*,*,#8543,.T.);
#13166=ORIENTED_EDGE('',*,*,#8544,.T.);
#13167=ORIENTED_EDGE('',*,*,#8545,.T.);
#13168=ORIENTED_EDGE('',*,*,#8546,.T.);
#13169=ORIENTED_EDGE('',*,*,#8547,.T.);
#13170=ORIENTED_EDGE('',*,*,#8548,.T.);
#13171=ORIENTED_EDGE('',*,*,#8549,.T.);
#13172=ORIENTED_EDGE('',*,*,#8550,.T.);
#13173=ORIENTED_EDGE('',*,*,#8551,.T.);
#13174=ORIENTED_EDGE('',*,*,#8552,.T.);
#13175=ORIENTED_EDGE('',*,*,#8553,.T.);
#13176=ORIENTED_EDGE('',*,*,#8554,.T.);
#13177=ORIENTED_EDGE('',*,*,#8555,.T.);
#13178=ORIENTED_EDGE('',*,*,#8556,.T.);
#13179=ORIENTED_EDGE('',*,*,#8557,.T.);
#13180=ORIENTED_EDGE('',*,*,#8558,.T.);
#13181=ORIENTED_EDGE('',*,*,#8559,.T.);
#13182=ORIENTED_EDGE('',*,*,#8560,.F.);
#13183=ORIENTED_EDGE('',*,*,#8561,.T.);
#13184=ORIENTED_EDGE('',*,*,#8562,.T.);
#13185=ORIENTED_EDGE('',*,*,#8563,.F.);
#13186=ORIENTED_EDGE('',*,*,#8539,.T.);
#13187=ORIENTED_EDGE('',*,*,#8564,.T.);
#13188=ORIENTED_EDGE('',*,*,#8565,.T.);
#13189=ORIENTED_EDGE('',*,*,#8537,.T.);
#13190=ORIENTED_EDGE('',*,*,#8536,.T.);
#13191=ORIENTED_EDGE('',*,*,#8532,.T.);
#13192=ORIENTED_EDGE('',*,*,#8531,.T.);
#13193=ORIENTED_EDGE('',*,*,#8527,.T.);
#13194=ORIENTED_EDGE('',*,*,#8526,.T.);
#13195=ORIENTED_EDGE('',*,*,#8522,.T.);
#13196=ORIENTED_EDGE('',*,*,#8521,.T.);
#13197=ORIENTED_EDGE('',*,*,#8517,.T.);
#13198=ORIENTED_EDGE('',*,*,#8516,.T.);
#13199=ORIENTED_EDGE('',*,*,#8512,.T.);
#13200=ORIENTED_EDGE('',*,*,#8511,.T.);
#13201=ORIENTED_EDGE('',*,*,#8507,.T.);
#13202=ORIENTED_EDGE('',*,*,#8506,.T.);
#13203=ORIENTED_EDGE('',*,*,#8502,.T.);
#13204=ORIENTED_EDGE('',*,*,#8501,.T.);
#13205=ORIENTED_EDGE('',*,*,#8497,.T.);
#13206=ORIENTED_EDGE('',*,*,#8496,.T.);
#13207=ORIENTED_EDGE('',*,*,#8492,.T.);
#13208=ORIENTED_EDGE('',*,*,#8491,.T.);
#13209=ORIENTED_EDGE('',*,*,#8487,.T.);
#13210=ORIENTED_EDGE('',*,*,#8486,.T.);
#13211=ORIENTED_EDGE('',*,*,#8482,.T.);
#13212=ORIENTED_EDGE('',*,*,#8481,.T.);
#13213=ORIENTED_EDGE('',*,*,#8477,.T.);
#13214=ORIENTED_EDGE('',*,*,#8476,.T.);
#13215=ORIENTED_EDGE('',*,*,#8472,.T.);
#13216=ORIENTED_EDGE('',*,*,#8471,.T.);
#13217=ORIENTED_EDGE('',*,*,#8467,.T.);
#13218=ORIENTED_EDGE('',*,*,#8466,.T.);
#13219=ORIENTED_EDGE('',*,*,#8462,.T.);
#13220=ORIENTED_EDGE('',*,*,#8461,.T.);
#13221=ORIENTED_EDGE('',*,*,#8566,.F.);
#13222=ORIENTED_EDGE('',*,*,#8567,.T.);
#13223=ORIENTED_EDGE('',*,*,#8568,.T.);
#13224=ORIENTED_EDGE('',*,*,#8569,.F.);
#13225=ORIENTED_EDGE('',*,*,#8570,.F.);
#13226=ORIENTED_EDGE('',*,*,#8571,.F.);
#13227=ORIENTED_EDGE('',*,*,#8572,.F.);
#13228=ORIENTED_EDGE('',*,*,#8573,.F.);
#13229=ORIENTED_EDGE('',*,*,#8574,.F.);
#13230=ORIENTED_EDGE('',*,*,#8575,.F.);
#13231=ORIENTED_EDGE('',*,*,#8576,.F.);
#13232=ORIENTED_EDGE('',*,*,#8577,.F.);
#13233=ORIENTED_EDGE('',*,*,#8578,.F.);
#13234=ORIENTED_EDGE('',*,*,#8579,.F.);
#13235=ORIENTED_EDGE('',*,*,#8580,.F.);
#13236=ORIENTED_EDGE('',*,*,#8581,.F.);
#13237=ORIENTED_EDGE('',*,*,#8582,.F.);
#13238=ORIENTED_EDGE('',*,*,#8583,.F.);
#13239=ORIENTED_EDGE('',*,*,#8584,.F.);
#13240=ORIENTED_EDGE('',*,*,#8585,.F.);
#13241=ORIENTED_EDGE('',*,*,#8586,.F.);
#13242=ORIENTED_EDGE('',*,*,#8587,.F.);
#13243=ORIENTED_EDGE('',*,*,#8588,.F.);
#13244=ORIENTED_EDGE('',*,*,#8559,.F.);
#13245=ORIENTED_EDGE('',*,*,#8558,.F.);
#13246=ORIENTED_EDGE('',*,*,#8557,.F.);
#13247=ORIENTED_EDGE('',*,*,#8556,.F.);
#13248=ORIENTED_EDGE('',*,*,#8555,.F.);
#13249=ORIENTED_EDGE('',*,*,#8554,.F.);
#13250=ORIENTED_EDGE('',*,*,#8553,.F.);
#13251=ORIENTED_EDGE('',*,*,#8552,.F.);
#13252=ORIENTED_EDGE('',*,*,#8551,.F.);
#13253=ORIENTED_EDGE('',*,*,#8550,.F.);
#13254=ORIENTED_EDGE('',*,*,#8549,.F.);
#13255=ORIENTED_EDGE('',*,*,#8548,.F.);
#13256=ORIENTED_EDGE('',*,*,#8547,.F.);
#13257=ORIENTED_EDGE('',*,*,#8546,.F.);
#13258=ORIENTED_EDGE('',*,*,#8545,.F.);
#13259=ORIENTED_EDGE('',*,*,#8544,.F.);
#13260=ORIENTED_EDGE('',*,*,#8543,.F.);
#13261=ORIENTED_EDGE('',*,*,#8589,.F.);
#13262=ORIENTED_EDGE('',*,*,#8562,.F.);
#13263=ORIENTED_EDGE('',*,*,#8561,.F.);
#13264=ORIENTED_EDGE('',*,*,#8590,.F.);
#13265=ORIENTED_EDGE('',*,*,#8591,.F.);
#13266=ORIENTED_EDGE('',*,*,#8592,.F.);
#13267=ORIENTED_EDGE('',*,*,#8593,.F.);
#13268=ORIENTED_EDGE('',*,*,#8592,.T.);
#13269=ORIENTED_EDGE('',*,*,#8591,.T.);
#13270=ORIENTED_EDGE('',*,*,#8594,.F.);
#13271=ORIENTED_EDGE('',*,*,#8595,.F.);
#13272=ORIENTED_EDGE('',*,*,#8596,.T.);
#13273=ORIENTED_EDGE('',*,*,#8597,.F.);
#13274=ORIENTED_EDGE('',*,*,#8598,.F.);
#13275=ORIENTED_EDGE('',*,*,#8599,.F.);
#13276=ORIENTED_EDGE('',*,*,#8600,.F.);
#13277=ORIENTED_EDGE('',*,*,#8568,.F.);
#13278=ORIENTED_EDGE('',*,*,#8567,.F.);
#13279=ORIENTED_EDGE('',*,*,#8538,.T.);
#13280=ORIENTED_EDGE('',*,*,#8601,.T.);
#13281=ORIENTED_EDGE('',*,*,#8602,.T.);
#13282=ORIENTED_EDGE('',*,*,#8533,.F.);
#13283=ORIENTED_EDGE('',*,*,#8565,.F.);
#13284=ORIENTED_EDGE('',*,*,#8564,.F.);
#13285=ORIENTED_EDGE('',*,*,#8603,.F.);
#13286=ORIENTED_EDGE('',*,*,#8459,.F.);
#13287=ORIENTED_EDGE('',*,*,#8458,.F.);
#13288=ORIENTED_EDGE('',*,*,#8465,.F.);
#13289=ORIENTED_EDGE('',*,*,#8464,.F.);
#13290=ORIENTED_EDGE('',*,*,#8470,.F.);
#13291=ORIENTED_EDGE('',*,*,#8469,.F.);
#13292=ORIENTED_EDGE('',*,*,#8475,.F.);
#13293=ORIENTED_EDGE('',*,*,#8474,.F.);
#13294=ORIENTED_EDGE('',*,*,#8480,.F.);
#13295=ORIENTED_EDGE('',*,*,#8479,.F.);
#13296=ORIENTED_EDGE('',*,*,#8485,.F.);
#13297=ORIENTED_EDGE('',*,*,#8484,.F.);
#13298=ORIENTED_EDGE('',*,*,#8490,.F.);
#13299=ORIENTED_EDGE('',*,*,#8489,.F.);
#13300=ORIENTED_EDGE('',*,*,#8495,.F.);
#13301=ORIENTED_EDGE('',*,*,#8494,.F.);
#13302=ORIENTED_EDGE('',*,*,#8500,.F.);
#13303=ORIENTED_EDGE('',*,*,#8499,.F.);
#13304=ORIENTED_EDGE('',*,*,#8505,.F.);
#13305=ORIENTED_EDGE('',*,*,#8504,.F.);
#13306=ORIENTED_EDGE('',*,*,#8510,.F.);
#13307=ORIENTED_EDGE('',*,*,#8509,.F.);
#13308=ORIENTED_EDGE('',*,*,#8515,.F.);
#13309=ORIENTED_EDGE('',*,*,#8514,.F.);
#13310=ORIENTED_EDGE('',*,*,#8520,.F.);
#13311=ORIENTED_EDGE('',*,*,#8519,.F.);
#13312=ORIENTED_EDGE('',*,*,#8525,.F.);
#13313=ORIENTED_EDGE('',*,*,#8524,.F.);
#13314=ORIENTED_EDGE('',*,*,#8530,.F.);
#13315=ORIENTED_EDGE('',*,*,#8529,.F.);
#13316=ORIENTED_EDGE('',*,*,#8535,.F.);
#13317=ORIENTED_EDGE('',*,*,#8534,.F.);
#13318=ORIENTED_EDGE('',*,*,#8602,.F.);
#13319=ORIENTED_EDGE('',*,*,#8601,.F.);
#13320=ORIENTED_EDGE('',*,*,#8541,.F.);
#13321=ORIENTED_EDGE('',*,*,#8604,.F.);
#13322=ORIENTED_EDGE('',*,*,#8596,.F.);
#13323=ORIENTED_EDGE('',*,*,#8605,.F.);
#13324=ORIENTED_EDGE('',*,*,#8587,.T.);
#13325=ORIENTED_EDGE('',*,*,#8586,.T.);
#13326=ORIENTED_EDGE('',*,*,#8585,.T.);
#13327=ORIENTED_EDGE('',*,*,#8584,.T.);
#13328=ORIENTED_EDGE('',*,*,#8583,.T.);
#13329=ORIENTED_EDGE('',*,*,#8582,.T.);
#13330=ORIENTED_EDGE('',*,*,#8581,.T.);
#13331=ORIENTED_EDGE('',*,*,#8580,.T.);
#13332=ORIENTED_EDGE('',*,*,#8579,.T.);
#13333=ORIENTED_EDGE('',*,*,#8578,.T.);
#13334=ORIENTED_EDGE('',*,*,#8577,.T.);
#13335=ORIENTED_EDGE('',*,*,#8576,.T.);
#13336=ORIENTED_EDGE('',*,*,#8575,.T.);
#13337=ORIENTED_EDGE('',*,*,#8574,.T.);
#13338=ORIENTED_EDGE('',*,*,#8573,.T.);
#13339=ORIENTED_EDGE('',*,*,#8572,.T.);
#13340=ORIENTED_EDGE('',*,*,#8571,.T.);
#13341=ORIENTED_EDGE('',*,*,#8606,.F.);
#13342=ORIENTED_EDGE('',*,*,#8599,.T.);
#13343=ORIENTED_EDGE('',*,*,#8598,.T.);
#13344=ORIENTED_EDGE('',*,*,#8607,.F.);
#13345=ORIENTED_EDGE('',*,*,#8608,.F.);
#13346=ORIENTED_EDGE('',*,*,#8609,.T.);
#13347=ORIENTED_EDGE('',*,*,#8569,.T.);
#13348=ORIENTED_EDGE('',*,*,#8600,.T.);
#13349=ORIENTED_EDGE('',*,*,#8606,.T.);
#13350=ORIENTED_EDGE('',*,*,#8570,.T.);
#13351=ORIENTED_EDGE('',*,*,#8542,.T.);
#13352=ORIENTED_EDGE('',*,*,#8460,.T.);
#13353=ORIENTED_EDGE('',*,*,#8603,.T.);
#13354=ORIENTED_EDGE('',*,*,#8610,.T.);
#13355=ORIENTED_EDGE('',*,*,#8611,.T.);
#13356=ORIENTED_EDGE('',*,*,#8610,.F.);
#13357=ORIENTED_EDGE('',*,*,#8607,.T.);
#13358=ORIENTED_EDGE('',*,*,#8597,.T.);
#13359=ORIENTED_EDGE('',*,*,#8566,.T.);
#13360=ORIENTED_EDGE('',*,*,#8609,.F.);
#13361=ORIENTED_EDGE('',*,*,#8595,.T.);
#13362=ORIENTED_EDGE('',*,*,#8594,.T.);
#13363=ORIENTED_EDGE('',*,*,#8604,.T.);
#13364=ORIENTED_EDGE('',*,*,#8540,.T.);
#13365=ORIENTED_EDGE('',*,*,#8563,.T.);
#13366=ORIENTED_EDGE('',*,*,#8589,.T.);
#13367=ORIENTED_EDGE('',*,*,#8593,.T.);
#13368=ORIENTED_EDGE('',*,*,#8590,.T.);
#13369=ORIENTED_EDGE('',*,*,#8560,.T.);
#13370=ORIENTED_EDGE('',*,*,#8588,.T.);
#13371=ORIENTED_EDGE('',*,*,#8605,.T.);
#13372=ORIENTED_EDGE('',*,*,#8608,.T.);
#13373=ORIENTED_EDGE('',*,*,#8611,.F.);
#14388=CYLINDRICAL_SURFACE('',#15447,4.91825);
#14389=CYLINDRICAL_SURFACE('',#15448,4.91825);
#14390=CYLINDRICAL_SURFACE('',#15449,4.91825);
#14391=CYLINDRICAL_SURFACE('',#15450,4.91825);
#14392=CYLINDRICAL_SURFACE('',#15451,4.91825);
#14393=CYLINDRICAL_SURFACE('',#15452,4.91825);
#14394=CYLINDRICAL_SURFACE('',#15453,4.91825);
#14395=CYLINDRICAL_SURFACE('',#15454,4.91825);
#14396=CYLINDRICAL_SURFACE('',#15455,4.91825);
#14397=CYLINDRICAL_SURFACE('',#15456,4.91825);
#14398=CYLINDRICAL_SURFACE('',#15457,4.91825);
#14399=CYLINDRICAL_SURFACE('',#15458,4.91825);
#14400=CYLINDRICAL_SURFACE('',#15459,4.91825);
#14401=CYLINDRICAL_SURFACE('',#15460,4.91825);
#14402=CYLINDRICAL_SURFACE('',#15461,4.91825);
#14403=CYLINDRICAL_SURFACE('',#15462,4.91825);
#14404=CYLINDRICAL_SURFACE('',#15463,4.91825);
#14405=CYLINDRICAL_SURFACE('',#15464,5.91675);
#14406=CYLINDRICAL_SURFACE('',#15465,5.91675);
#14407=CYLINDRICAL_SURFACE('',#15466,4.91825);
#14408=CYLINDRICAL_SURFACE('',#15467,5.91675);
#14409=CYLINDRICAL_SURFACE('',#15468,4.91825);
#14410=CYLINDRICAL_SURFACE('',#15469,15.2420394990918);
#14801=ADVANCED_FACE('',(#2443),#14388,.F.);
#14802=ADVANCED_FACE('',(#2444),#14389,.F.);
#14803=ADVANCED_FACE('',(#2445),#14390,.F.);
#14804=ADVANCED_FACE('',(#2446),#14391,.F.);
#14805=ADVANCED_FACE('',(#2447),#14392,.F.);
#14806=ADVANCED_FACE('',(#2448),#14393,.F.);
#14807=ADVANCED_FACE('',(#2449),#14394,.F.);
#14808=ADVANCED_FACE('',(#2450),#14395,.F.);
#14809=ADVANCED_FACE('',(#2451),#14396,.F.);
#14810=ADVANCED_FACE('',(#2452),#14397,.F.);
#14811=ADVANCED_FACE('',(#2453),#14398,.F.);
#14812=ADVANCED_FACE('',(#2454),#14399,.F.);
#14813=ADVANCED_FACE('',(#2455),#14400,.F.);
#14814=ADVANCED_FACE('',(#2456),#14401,.F.);
#14815=ADVANCED_FACE('',(#2457),#14402,.F.);
#14816=ADVANCED_FACE('',(#2458),#14403,.F.);
#14817=ADVANCED_FACE('',(#2459),#14404,.F.);
#14818=ADVANCED_FACE('',(#2460),#49,.T.);
#14819=ADVANCED_FACE('',(#2461),#50,.T.);
#14820=ADVANCED_FACE('',(#2462),#14405,.F.);
#14821=ADVANCED_FACE('',(#2463),#14406,.F.);
#14822=ADVANCED_FACE('',(#2464),#51,.T.);
#14823=ADVANCED_FACE('',(#2465),#14407,.F.);
#14824=ADVANCED_FACE('',(#2466),#14408,.F.);
#14825=ADVANCED_FACE('',(#2467),#14409,.F.);
#14826=ADVANCED_FACE('',(#2468),#52,.T.);
#14827=ADVANCED_FACE('',(#2469,#1995),#14410,.T.);
#14828=ADVANCED_FACE('',(#2470),#2061,.T.);
#14829=ADVANCED_FACE('',(#2471),#2062,.F.);
#14941=CLOSED_SHELL('',(#14801,#14802,#14803,#14804,#14805,#14806,#14807,
#14808,#14809,#14810,#14811,#14812,#14813,#14814,#14815,#14816,#14817,#14818,
#14819,#14820,#14821,#14822,#14823,#14824,#14825,#14826,#14827,#14828,#14829));
#15446=AXIS2_PLACEMENT_3D('',#202532,#16836,#16837);
#15447=AXIS2_PLACEMENT_3D('',#202533,#16838,#16839);
#15448=AXIS2_PLACEMENT_3D('',#202854,#16841,#16842);
#15449=AXIS2_PLACEMENT_3D('',#203320,#16844,#16845);
#15450=AXIS2_PLACEMENT_3D('',#203786,#16847,#16848);
#15451=AXIS2_PLACEMENT_3D('',#204252,#16850,#16851);
#15452=AXIS2_PLACEMENT_3D('',#204715,#16853,#16854);
#15453=AXIS2_PLACEMENT_3D('',#205181,#16856,#16857);
#15454=AXIS2_PLACEMENT_3D('',#205647,#16859,#16860);
#15455=AXIS2_PLACEMENT_3D('',#206107,#16862,#16863);
#15456=AXIS2_PLACEMENT_3D('',#206360,#16865,#16866);
#15457=AXIS2_PLACEMENT_3D('',#206616,#16868,#16869);
#15458=AXIS2_PLACEMENT_3D('',#207082,#16871,#16872);
#15459=AXIS2_PLACEMENT_3D('',#207545,#16874,#16875);
#15460=AXIS2_PLACEMENT_3D('',#208011,#16877,#16878);
#15461=AXIS2_PLACEMENT_3D('',#208477,#16880,#16881);
#15462=AXIS2_PLACEMENT_3D('',#208943,#16883,#16884);
#15463=AXIS2_PLACEMENT_3D('',#209412,#16886,#16887);
#15464=AXIS2_PLACEMENT_3D('',#225212,#16889,#16890);
#15465=AXIS2_PLACEMENT_3D('',#226295,#16891,#16892);
#15466=AXIS2_PLACEMENT_3D('',#233123,#16893,#16894);
#15467=AXIS2_PLACEMENT_3D('',#233204,#16895,#16896);
#15468=AXIS2_PLACEMENT_3D('',#233271,#16897,#16898);
#15469=AXIS2_PLACEMENT_3D('',#240442,#16899,#16900);
#15470=AXIS2_PLACEMENT_3D('',#240444,#16901,#16902);
#15471=AXIS2_PLACEMENT_3D('',#240448,#16905,#16906);
#15472=AXIS2_PLACEMENT_3D('',#240449,#16907,#16908);
#15473=AXIS2_PLACEMENT_3D('',#240450,#16909,#16910);
#16836=DIRECTION('axis',(0.,0.,1.));
#16837=DIRECTION('refdir',(1.,0.,0.));
#16838=DIRECTION('center_axis',(-1.,0.,0.));
#16839=DIRECTION('ref_axis',(0.,0.968648305440766,0.248436028721142));
#16840=DIRECTION('',(-1.,0.,0.));
#16841=DIRECTION('center_axis',(-1.,0.,0.));
#16842=DIRECTION('ref_axis',(0.,0.968648305440766,0.248436028721142));
#16843=DIRECTION('',(-1.,0.,0.));
#16844=DIRECTION('center_axis',(-1.,0.,0.));
#16845=DIRECTION('ref_axis',(0.,0.968648305440766,0.248436028721142));
#16846=DIRECTION('',(-1.,0.,0.));
#16847=DIRECTION('center_axis',(-1.,0.,0.));
#16848=DIRECTION('ref_axis',(0.,0.968648305440766,0.248436028721142));
#16849=DIRECTION('',(-1.,0.,0.));
#16850=DIRECTION('center_axis',(-1.,0.,0.));
#16851=DIRECTION('ref_axis',(0.,0.968648305440766,0.248436028721142));
#16852=DIRECTION('',(-1.,0.,0.));
#16853=DIRECTION('center_axis',(-1.,0.,0.));
#16854=DIRECTION('ref_axis',(0.,0.968648305440766,0.248436028721142));
#16855=DIRECTION('',(-1.,0.,0.));
#16856=DIRECTION('center_axis',(-1.,0.,0.));
#16857=DIRECTION('ref_axis',(0.,0.968648305440766,0.248436028721142));
#16858=DIRECTION('',(-1.,0.,0.));
#16859=DIRECTION('center_axis',(-1.,0.,0.));
#16860=DIRECTION('ref_axis',(0.,0.968648305440766,0.248436028721142));
#16861=DIRECTION('',(-1.,0.,0.));
#16862=DIRECTION('center_axis',(-1.,0.,0.));
#16863=DIRECTION('ref_axis',(0.,0.968648305440766,0.248436028721142));
#16864=DIRECTION('',(-1.,0.,0.));
#16865=DIRECTION('center_axis',(-1.,0.,0.));
#16866=DIRECTION('ref_axis',(0.,0.968648305440766,0.248436028721142));
#16867=DIRECTION('',(-1.,0.,0.));
#16868=DIRECTION('center_axis',(-1.,0.,0.));
#16869=DIRECTION('ref_axis',(0.,0.968648305440766,0.248436028721142));
#16870=DIRECTION('',(-1.,0.,0.));
#16871=DIRECTION('center_axis',(-1.,0.,0.));
#16872=DIRECTION('ref_axis',(0.,0.968648305440766,0.248436028721142));
#16873=DIRECTION('',(-1.,0.,0.));
#16874=DIRECTION('center_axis',(-1.,0.,0.));
#16875=DIRECTION('ref_axis',(0.,0.968648305440766,0.248436028721142));
#16876=DIRECTION('',(-1.,0.,0.));
#16877=DIRECTION('center_axis',(-1.,0.,0.));
#16878=DIRECTION('ref_axis',(0.,0.968648305440766,0.248436028721142));
#16879=DIRECTION('',(-1.,0.,0.));
#16880=DIRECTION('center_axis',(-1.,0.,0.));
#16881=DIRECTION('ref_axis',(0.,0.968648305440766,0.248436028721142));
#16882=DIRECTION('',(-1.,0.,0.));
#16883=DIRECTION('center_axis',(-1.,0.,0.));
#16884=DIRECTION('ref_axis',(0.,0.968648305440766,0.248436028721142));
#16885=DIRECTION('',(-1.,0.,0.));
#16886=DIRECTION('center_axis',(-1.,0.,0.));
#16887=DIRECTION('ref_axis',(0.,0.968648305440766,0.248436028721142));
#16888=DIRECTION('',(-1.,0.,0.));
#16889=DIRECTION('center_axis',(-1.,0.,0.));
#16890=DIRECTION('ref_axis',(0.,1.,0.));
#16891=DIRECTION('center_axis',(-1.,0.,0.));
#16892=DIRECTION('ref_axis',(0.,-0.988910129220642,0.148515172035763));
#16893=DIRECTION('center_axis',(-1.,0.,0.));
#16894=DIRECTION('ref_axis',(0.,0.968648305440766,0.248436028721142));
#16895=DIRECTION('center_axis',(-1.,0.,0.));
#16896=DIRECTION('ref_axis',(0.,-0.967688737574893,-0.252147788351813));
#16897=DIRECTION('center_axis',(-1.,0.,0.));
#16898=DIRECTION('ref_axis',(0.,0.968648305440766,0.248436028721142));
#16899=DIRECTION('center_axis',(0.,-1.,0.));
#16900=DIRECTION('ref_axis',(1.,0.,0.));
#16901=DIRECTION('center_axis',(0.,-1.,0.));
#16902=DIRECTION('ref_axis',(1.,0.,0.));
#16903=DIRECTION('',(0.,1.,0.));
#16904=DIRECTION('',(0.,1.,0.));
#16905=DIRECTION('center_axis',(0.,-1.,0.));
#16906=DIRECTION('ref_axis',(1.,0.,0.));
#16907=DIRECTION('center_axis',(0.,-1.,0.));
#16908=DIRECTION('ref_axis',(1.,0.,0.));
#16909=DIRECTION('center_axis',(0.,-1.,0.));
#16910=DIRECTION('ref_axis',(1.,0.,0.));
#202532=CARTESIAN_POINT('',(0.,0.,0.));
#202533=CARTESIAN_POINT('Origin',(213.235140564004,0.,130.804360617566));
#202534=CARTESIAN_POINT('',(179.180279212536,-4.76405452823405,129.582490119308));
#202535=CARTESIAN_POINT('',(178.834794689177,-4.76405452823405,129.582490119308));
#202536=CARTESIAN_POINT('',(213.235140564004,-4.76405452823405,129.582490119308));
#202537=CARTESIAN_POINT('',(178.764859436029,-4.91824789753406,130.799812991619));
#202538=CARTESIAN_POINT('Ctrl Pts',(178.834794689177,-4.76405452823405,
129.582490119308));
#202539=CARTESIAN_POINT('Ctrl Pts',(178.834348169157,-4.76600152135323,
129.59008141593));
#202540=CARTESIAN_POINT('Ctrl Pts',(178.833901649136,-4.76793019492675,
129.597676684138));
#202541=CARTESIAN_POINT('Ctrl Pts',(178.833455129116,-4.76984053507245,
129.605275828037));
#202542=CARTESIAN_POINT('Ctrl Pts',(178.823192962182,-4.81374501544364,
129.779923502642));
#202543=CARTESIAN_POINT('Ctrl Pts',(178.812930795248,-4.84807446073973,
129.95706774057));
#202544=CARTESIAN_POINT('Ctrl Pts',(178.802668628314,-4.87259841686327,
130.13580416484));
#202545=CARTESIAN_POINT('Ctrl Pts',(178.792640946099,-4.89656201443736,
130.310456562743));
#202546=CARTESIAN_POINT('Ctrl Pts',(178.782613263885,-4.91116315740482,
130.486629512172));
#202547=CARTESIAN_POINT('Ctrl Pts',(178.772585581671,-4.9162311945412,130.663456734298));
#202548=CARTESIAN_POINT('Ctrl Pts',(178.77001019979,-4.91753280449775,130.708870780548));
#202549=CARTESIAN_POINT('Ctrl Pts',(178.76743481791,-4.91820583999571,130.754327852339));
#202550=CARTESIAN_POINT('Ctrl Pts',(178.764859436029,-4.91824789753406,
130.799812991619));
#202551=CARTESIAN_POINT('',(177.723712521315,4.07640974993461,128.054215600239));
#202552=CARTESIAN_POINT('Ctrl Pts',(178.764859435991,-4.91824789753469,
130.799812992297));
#202553=CARTESIAN_POINT('Ctrl Pts',(178.757196290994,-4.9183730412926,130.935155723463));
#202554=CARTESIAN_POINT('Ctrl Pts',(178.749533145997,-4.91290734326878,
131.070645942394));
#202555=CARTESIAN_POINT('Ctrl Pts',(178.741870001,-4.90184112669081,131.205778892166));
#202556=CARTESIAN_POINT('Ctrl Pts',(178.734084063679,-4.89059758781915,
131.343077178612));
#202557=CARTESIAN_POINT('Ctrl Pts',(178.726298126358,-4.87357245610437,
131.480006229492));
#202558=CARTESIAN_POINT('Ctrl Pts',(178.718512189038,-4.85081073812513,
131.61603681248));
#202559=CARTESIAN_POINT('Ctrl Pts',(178.710856306159,-4.82842922645917,
131.749795173024));
#202560=CARTESIAN_POINT('Ctrl Pts',(178.70320042328,-4.80050136400255,131.882684439534));
#202561=CARTESIAN_POINT('Ctrl Pts',(178.695544540401,-4.76712209381898,
132.01420771746));
#202562=CARTESIAN_POINT('Ctrl Pts',(178.687889375061,-4.73374595206982,
132.145718668516));
#202563=CARTESIAN_POINT('Ctrl Pts',(178.680234209721,-4.69491951717209,
132.27586349683));
#202564=CARTESIAN_POINT('Ctrl Pts',(178.672579044381,-4.65078839204757,
132.404157603091));
#202565=CARTESIAN_POINT('Ctrl Pts',(178.664922844915,-4.60665130530803,
132.532469040433));
#202566=CARTESIAN_POINT('Ctrl Pts',(178.657266645449,-4.55720823398827,
132.65892887934));
#202567=CARTESIAN_POINT('Ctrl Pts',(178.649610445982,-4.50265380566106,
132.783070239735));
#202568=CARTESIAN_POINT('Ctrl Pts',(178.641726867593,-4.44647918349511,
132.910898433141));
#202569=CARTESIAN_POINT('Ctrl Pts',(178.633843289203,-4.3848850536798,133.036267873534));
#202570=CARTESIAN_POINT('Ctrl Pts',(178.625959710813,-4.31813542196403,
133.158694820707));
#202571=CARTESIAN_POINT('Ctrl Pts',(178.618292097771,-4.25321435168799,
133.277767963686));
#202572=CARTESIAN_POINT('Ctrl Pts',(178.610624484729,-4.18341682154212,
133.394057413434));
#202573=CARTESIAN_POINT('Ctrl Pts',(178.602956871687,-4.10902994539855,
133.507147322121));
#202574=CARTESIAN_POINT('Ctrl Pts',(178.594965310623,-4.03150030744991,
133.625015152183));
#202575=CARTESIAN_POINT('Ctrl Pts',(178.586973749559,-3.94898534362607,
133.739406770363));
#202576=CARTESIAN_POINT('Ctrl Pts',(178.578982188495,-3.861856090724,133.849890226195));
#202577=CARTESIAN_POINT('Ctrl Pts',(178.570990627431,-3.77472683782194,
133.960373682027));
#202578=CARTESIAN_POINT('Ctrl Pts',(178.562999066367,-3.68298366963375,
134.066948657916));
#202579=CARTESIAN_POINT('Ctrl Pts',(178.555007505303,-3.58703931231371,
134.169227930614));
#202580=CARTESIAN_POINT('Ctrl Pts',(178.547233171184,-3.493702918501,134.268727043871));
#202581=CARTESIAN_POINT('Ctrl Pts',(178.539458837065,-3.39607561388428,
134.364497295231));
#202582=CARTESIAN_POINT('Ctrl Pts',(178.531684502946,-3.2944872852368,134.456146015137));
#202583=CARTESIAN_POINT('Ctrl Pts',(178.523919749999,-3.19302415512523,
134.547681786186));
#202584=CARTESIAN_POINT('Ctrl Pts',(178.516154997052,-3.08761000143176,
134.635105872937));
#202585=CARTESIAN_POINT('Ctrl Pts',(178.508390244105,-2.97861348023738,
134.718060248075));
#202586=CARTESIAN_POINT('Ctrl Pts',(178.50063320322,-2.86972521592481,134.800932231759));
#202587=CARTESIAN_POINT('Ctrl Pts',(178.492876162335,-2.75726197390471,
134.879343103152));
#202588=CARTESIAN_POINT('Ctrl Pts',(178.48511912145,-2.64162734560113,134.952973401313));
#202589=CARTESIAN_POINT('Ctrl Pts',(178.47736793021,-2.52607991827016,135.026548174295));
#202590=CARTESIAN_POINT('Ctrl Pts',(178.46961673897,-2.40736619337517,135.095349340572));
#202591=CARTESIAN_POINT('Ctrl Pts',(178.46186554773,-2.28592046387358,135.159099495541));
#202592=CARTESIAN_POINT('Ctrl Pts',(178.454117650953,-2.16452635204637,
135.222822554993));
#202593=CARTESIAN_POINT('Ctrl Pts',(178.446369754175,-2.04040289054619,
135.281498691652));
#202594=CARTESIAN_POINT('Ctrl Pts',(178.438621857398,-1.91401061513348,
135.334895511776));
#202595=CARTESIAN_POINT('Ctrl Pts',(178.430875581314,-1.78764477826022,
135.388281162436));
#202596=CARTESIAN_POINT('Ctrl Pts',(178.42312930523,-1.6590114313704,135.436389541058));
#202597=CARTESIAN_POINT('Ctrl Pts',(178.415383029146,-1.52859245082243,
135.479035812891));
#202598=CARTESIAN_POINT('Ctrl Pts',(178.407636695881,-1.39817250755127,
135.521682399529));
#202599=CARTESIAN_POINT('Ctrl Pts',(178.399890362615,-1.26596727592271,
135.55886667741));
#202600=CARTESIAN_POINT('Ctrl Pts',(178.39214402935,-1.1324748224956,135.590453370419));
#202601=CARTESIAN_POINT('Ctrl Pts',(178.384395961347,-0.998952474358899,
135.62204713705));
#202602=CARTESIAN_POINT('Ctrl Pts',(178.376647893344,-0.864142711197707,
135.648040734402));
#202603=CARTESIAN_POINT('Ctrl Pts',(178.368899825341,-0.728554452264122,
135.668349872549));
#202604=CARTESIAN_POINT('Ctrl Pts',(178.361143522599,-0.592822088515468,
135.688680595488));
#202605=CARTESIAN_POINT('Ctrl Pts',(178.353387219857,-0.456309963453038,
135.703314732646));
#202606=CARTESIAN_POINT('Ctrl Pts',(178.345630917115,-0.319533349451039,
135.712219774173));
#202607=CARTESIAN_POINT('Ctrl Pts',(178.337870474601,-0.182683733651767,
135.721129568589));
#202608=CARTESIAN_POINT('Ctrl Pts',(178.330110032087,-0.045569738297517,
135.724304165422));
#202609=CARTESIAN_POINT('Ctrl Pts',(178.322349589573,0.0912936838562829,
135.721763237424));
#202610=CARTESIAN_POINT('Ctrl Pts',(178.314576689307,0.228376811325325,
135.719218230503));
#202611=CARTESIAN_POINT('Ctrl Pts',(178.306803789042,0.365208171309374,
135.710939387667));
#202612=CARTESIAN_POINT('Ctrl Pts',(178.299030888776,0.501277348038855,
135.696998360424));
#202613=CARTESIAN_POINT('Ctrl Pts',(178.291540553014,0.632400067457702,
135.683564124637));
#202614=CARTESIAN_POINT('Ctrl Pts',(178.284050217252,0.762814751203412,
135.664872270292));
#202615=CARTESIAN_POINT('Ctrl Pts',(178.27655988149,0.89207580184942,135.641031355404));
#202616=CARTESIAN_POINT('Ctrl Pts',(178.268785547371,1.02623782451768,135.616286504981));
#202617=CARTESIAN_POINT('Ctrl Pts',(178.261011213252,1.15958199216667,135.585916048837));
#202618=CARTESIAN_POINT('Ctrl Pts',(178.253236879133,1.29159962891666,135.549985282569));
#202619=CARTESIAN_POINT('Ctrl Pts',(178.245472126186,1.4234545657279,135.514098797758));
#202620=CARTESIAN_POINT('Ctrl Pts',(178.237707373239,1.55398585084488,135.472665739113));
#202621=CARTESIAN_POINT('Ctrl Pts',(178.229942620292,1.68269299813225,135.425802744926));
#202622=CARTESIAN_POINT('Ctrl Pts',(178.222185579407,1.8112723116667,135.378986295725));
#202623=CARTESIAN_POINT('Ctrl Pts',(178.214428538522,1.93803072786065,135.326750776369));
#202624=CARTESIAN_POINT('Ctrl Pts',(178.206671497637,2.0624813241539,135.269263063311));
#202625=CARTESIAN_POINT('Ctrl Pts',(178.198920306396,2.18683807128473,135.211818702184));
#202626=CARTESIAN_POINT('Ctrl Pts',(178.191169115156,2.30889010907467,135.149130194217));
#202627=CARTESIAN_POINT('Ctrl Pts',(178.183417923916,2.42816930322083,135.081412978409));
#202628=CARTESIAN_POINT('Ctrl Pts',(178.175670027139,2.54739780052724,135.013724544225));
#202629=CARTESIAN_POINT('Ctrl Pts',(178.167922130362,2.66385545891838,134.941011845815));
#202630=CARTESIAN_POINT('Ctrl Pts',(178.160174233585,2.77709782812851,134.863536730462));
#202631=CARTESIAN_POINT('Ctrl Pts',(178.152427957501,2.89031650947627,134.786077821233));
#202632=CARTESIAN_POINT('Ctrl Pts',(178.144681681417,3.00032091694935,134.703858697166));
#202633=CARTESIAN_POINT('Ctrl Pts',(178.136935405333,3.10669507789434,134.617184866792));
#202634=CARTESIAN_POINT('Ctrl Pts',(178.129189072067,3.21307002406919,134.530510396612));
#202635=CARTESIAN_POINT('Ctrl Pts',(178.121442738802,3.3158143671513,134.439381401467));
#202636=CARTESIAN_POINT('Ctrl Pts',(178.113696405536,3.41454507837369,134.344143798815));
#202637=CARTESIAN_POINT('Ctrl Pts',(178.105948337533,3.51329789965441,134.248884868363));
#202638=CARTESIAN_POINT('Ctrl Pts',(178.098200269531,3.60803501918443,134.149515770902));
#202639=CARTESIAN_POINT('Ctrl Pts',(178.090452201528,3.69841043817239,134.046419113848));
#202640=CARTESIAN_POINT('Ctrl Pts',(178.082695898786,3.78888190923111,133.943212884441));
#202641=CARTESIAN_POINT('Ctrl Pts',(178.074939596044,3.87498216137204,133.836271475994));
#202642=CARTESIAN_POINT('Ctrl Pts',(178.067183293302,3.95640532583523,133.726010829382));
#202643=CARTESIAN_POINT('Ctrl Pts',(178.059422850788,4.03787194829287,133.615691333343));
#202644=CARTESIAN_POINT('Ctrl Pts',(178.051662408274,4.11465629020245,133.502049392914));
#202645=CARTESIAN_POINT('Ctrl Pts',(178.04390196576,4.18649655826397,133.385528886034));
#202646=CARTESIAN_POINT('Ctrl Pts',(178.036129065494,4.2584521507015,133.268821330092));
#202647=CARTESIAN_POINT('Ctrl Pts',(178.028356165229,4.32544761811758,133.149226314897));
#202648=CARTESIAN_POINT('Ctrl Pts',(178.020583264963,4.38726735076475,133.027211997081));
#202649=CARTESIAN_POINT('Ctrl Pts',(178.013092929201,4.44683978041561,132.909633207055));
#202650=CARTESIAN_POINT('Ctrl Pts',(178.005602593439,4.50160611609358,132.789808236237));
#202651=CARTESIAN_POINT('Ctrl Pts',(177.998112257677,4.5514168344388,132.668170656622));
#202652=CARTESIAN_POINT('Ctrl Pts',(177.990337833928,4.6031167373512,132.541919695675));
#202653=CARTESIAN_POINT('Ctrl Pts',(177.982563410178,4.64964146881412,132.413315987716));
#202654=CARTESIAN_POINT('Ctrl Pts',(177.974788986429,4.69077100477924,132.282822806201));
#202655=CARTESIAN_POINT('Ctrl Pts',(177.967024164819,4.73184974192762,132.152490795947));
#202656=CARTESIAN_POINT('Ctrl Pts',(177.959259343209,4.76754642582505,132.020274324827));
#202657=CARTESIAN_POINT('Ctrl Pts',(177.951494521598,4.79768865878615,131.886657525006));
#202658=CARTESIAN_POINT('Ctrl Pts',(177.943737432929,4.82780087327161,131.753173793384));
#202659=CARTESIAN_POINT('Ctrl Pts',(177.93598034426,4.85236955970395,131.618292887302));
#202660=CARTESIAN_POINT('Ctrl Pts',(177.928223255591,4.87127192133961,131.482514678874));
#202661=CARTESIAN_POINT('Ctrl Pts',(177.920472037378,4.89015997793087,131.346839225505));
#202662=CARTESIAN_POINT('Ctrl Pts',(177.912720819166,4.90339019157259,131.210268207127));
#202663=CARTESIAN_POINT('Ctrl Pts',(177.904969600953,4.91089077987771,131.073311934001));
#202664=CARTESIAN_POINT('Ctrl Pts',(177.897221785057,4.91838807587815,130.936415776397));
#202665=CARTESIAN_POINT('Ctrl Pts',(177.88947396916,4.92016072820489,130.799135089998));
#202666=CARTESIAN_POINT('Ctrl Pts',(177.881726153264,4.91618880208696,130.661985322185));
#202667=CARTESIAN_POINT('Ctrl Pts',(177.873979987703,4.91221772201521,130.524864768168));
#202668=CARTESIAN_POINT('Ctrl Pts',(177.866233822142,4.90250450894667,130.387875467793));
#202669=CARTESIAN_POINT('Ctrl Pts',(177.858487656581,4.88708135175385,130.251532503375));
#202670=CARTESIAN_POINT('Ctrl Pts',(177.850741463501,4.87165813976965,130.115189054594));
#202671=CARTESIAN_POINT('Ctrl Pts',(177.842995270422,4.85052498725969,129.979492334791));
#202672=CARTESIAN_POINT('Ctrl Pts',(177.835249077342,4.82376588322583,129.844951546144));
#202673=CARTESIAN_POINT('Ctrl Pts',(177.827501179234,4.79700088919644,129.710381143477));
#202674=CARTESIAN_POINT('Ctrl Pts',(177.819753281125,4.76460755599529,129.576967561547));
#202675=CARTESIAN_POINT('Ctrl Pts',(177.812005383017,4.72672075122141,129.445208675187));
#202676=CARTESIAN_POINT('Ctrl Pts',(177.804249662856,4.68879569703309,129.313316768893));
#202677=CARTESIAN_POINT('Ctrl Pts',(177.796493942696,4.64536620236076,129.183083270921));
#202678=CARTESIAN_POINT('Ctrl Pts',(177.788738222535,4.59661683543853,129.054990236354));
#202679=CARTESIAN_POINT('Ctrl Pts',(177.780978374852,4.54784152455826,128.926829031869));
#202680=CARTESIAN_POINT('Ctrl Pts',(177.77321852717,4.49374085422359,128.800810919526));
#202681=CARTESIAN_POINT('Ctrl Pts',(177.765458679487,4.43454670577277,128.677395978269));
#202682=CARTESIAN_POINT('Ctrl Pts',(177.757687345308,4.37526493531858,128.553798352327));
#202683=CARTESIAN_POINT('Ctrl Pts',(177.749916011129,4.31087480777823,128.432811940594));
#202684=CARTESIAN_POINT('Ctrl Pts',(177.742144676949,4.24165347448646,128.314870937958));
#202685=CARTESIAN_POINT('Ctrl Pts',(177.73624105985,4.18906839225497,128.225275187238));
#202686=CARTESIAN_POINT('Ctrl Pts',(177.73033744275,4.13369619242487,128.137436378276));
#202687=CARTESIAN_POINT('Ctrl Pts',(177.724433825651,4.07567416841541,128.051532410901));
#202688=CARTESIAN_POINT('',(177.982416834316,3.01851762861496,126.922258965043));
#202689=CARTESIAN_POINT('Ctrl Pts',(177.981069942749,3.00973836756106,126.914545966284));
#202690=CARTESIAN_POINT('Ctrl Pts',(177.946908021577,3.17701395531151,127.043975206374));
#202691=CARTESIAN_POINT('Ctrl Pts',(177.912210265842,3.33354615464498,127.18245091907));
#202692=CARTESIAN_POINT('Ctrl Pts',(177.827217622719,3.69622248758502,127.54512725201));
#202693=CARTESIAN_POINT('Ctrl Pts',(177.774439956054,3.90152846520454,127.792270849974));
#202694=CARTESIAN_POINT('Ctrl Pts',(177.725138528175,4.08258754759718,128.06179576351));
#202695=CARTESIAN_POINT('',(179.11014056404,-4.9182496345238,130.80625666781));
#202696=CARTESIAN_POINT('Ctrl Pts',(179.110140564008,-4.91824963452358,
130.806256668381));
#202697=CARTESIAN_POINT('Ctrl Pts',(179.104198294929,-4.9182094084543,130.910600839437));
#202698=CARTESIAN_POINT('Ctrl Pts',(179.09825602585,-4.91484884784317,131.014877292883));
#202699=CARTESIAN_POINT('Ctrl Pts',(179.09231375677,-4.90817921990328,131.11893939595));
#202700=CARTESIAN_POINT('Ctrl Pts',(179.084539422651,-4.89945327441634,
131.255084957113));
#202701=CARTESIAN_POINT('Ctrl Pts',(179.076765088532,-4.88504450286705,
131.391082820901));
#202702=CARTESIAN_POINT('Ctrl Pts',(179.068990754413,-4.86495766475957,
131.526420159846));
#202703=CARTESIAN_POINT('Ctrl Pts',(179.061226001466,-4.84489558188487,
131.661590707615));
#202704=CARTESIAN_POINT('Ctrl Pts',(179.053461248519,-4.81916941265581,
131.796101967218));
#202705=CARTESIAN_POINT('Ctrl Pts',(179.045696495572,-4.78783586718883,
131.929443179585));
#202706=CARTESIAN_POINT('Ctrl Pts',(179.037939454687,-4.75653344264092,
132.062651955581));
#202707=CARTESIAN_POINT('Ctrl Pts',(179.030182413802,-4.71963481392058,
132.194692618852));
#202708=CARTESIAN_POINT('Ctrl Pts',(179.022425372917,-4.67724817964733,
132.325061945403));
#202709=CARTESIAN_POINT('Ctrl Pts',(179.014674181676,-4.63489350946472,
132.455332959431));
#202710=CARTESIAN_POINT('Ctrl Pts',(179.006922990436,-4.58705919165299,
132.583934775123));
#202711=CARTESIAN_POINT('Ctrl Pts',(178.999171799196,-4.53390386652968,
132.710377089574));
#202712=CARTESIAN_POINT('Ctrl Pts',(178.991423902419,-4.48077113383746,
132.836765662669));
#202713=CARTESIAN_POINT('Ctrl Pts',(178.983676005642,-4.42232204312134,
132.960996200391));
#202714=CARTESIAN_POINT('Ctrl Pts',(178.975928108865,-4.35876411544756,
133.082596436876));
#202715=CARTESIAN_POINT('Ctrl Pts',(178.968181832781,-4.29521948272209,
133.204171237213));
#202716=CARTESIAN_POINT('Ctrl Pts',(178.960435556697,-4.22656831964791,
133.323116484425));
#202717=CARTESIAN_POINT('Ctrl Pts',(178.952689280612,-4.15306486639283,
133.438983034163));
#202718=CARTESIAN_POINT('Ctrl Pts',(178.944942947347,-4.07956087055197,
133.554850439201));
#202719=CARTESIAN_POINT('Ctrl Pts',(178.937196614082,-4.00120472249036,
133.667638771277));
#202720=CARTESIAN_POINT('Ctrl Pts',(178.929450280816,-3.91829467942949,
133.776926826695));
#202721=CARTESIAN_POINT('Ctrl Pts',(178.921702212813,-3.83536606923948,
133.886239356415));
#202722=CARTESIAN_POINT('Ctrl Pts',(178.91395414481,-3.74788177099222,133.992049738264));
#202723=CARTESIAN_POINT('Ctrl Pts',(178.906206076807,-3.65618084862433,
134.093969205932));
#202724=CARTESIAN_POINT('Ctrl Pts',(178.898449774065,-3.56438246542475,
134.195996994824));
#202725=CARTESIAN_POINT('Ctrl Pts',(178.890693471324,-3.4683587677859,134.294125317703));
#202726=CARTESIAN_POINT('Ctrl Pts',(178.882937168582,-3.3684866595003,134.388001320436));
#202727=CARTESIAN_POINT('Ctrl Pts',(178.875176726068,-3.2685612464633,134.481927427618));
#202728=CARTESIAN_POINT('Ctrl Pts',(178.867416283553,-3.1647836256717,134.571596436813));
#202729=CARTESIAN_POINT('Ctrl Pts',(178.859655841039,-3.0575636481392,134.656695961235));
#202730=CARTESIAN_POINT('Ctrl Pts',(178.851882940774,-2.95017155158026,
134.741932094967));
#202731=CARTESIAN_POINT('Ctrl Pts',(178.844110040508,-2.83932637193757,
134.822583855418));
#202732=CARTESIAN_POINT('Ctrl Pts',(178.836337140243,-2.7254675236648,134.898381848575));
#202733=CARTESIAN_POINT('Ctrl Pts',(178.828846804481,-2.61574773132176,
134.971424393755));
#202734=CARTESIAN_POINT('Ctrl Pts',(178.821356468719,-2.50322983824925,
135.039959777996));
#202735=CARTESIAN_POINT('Ctrl Pts',(178.813866132957,-2.38832672171129,
135.10378831586));
#202736=CARTESIAN_POINT('Ctrl Pts',(178.806091798838,-2.26906701858384,
135.170036932139));
#202737=CARTESIAN_POINT('Ctrl Pts',(178.798317464719,-2.1468598711432,135.231424591867));
#202738=CARTESIAN_POINT('Ctrl Pts',(178.7905431306,-2.02213930829118,135.287678103576));
#202739=CARTESIAN_POINT('Ctrl Pts',(178.782778377653,-1.8975724523863,135.34386228786));
#202740=CARTESIAN_POINT('Ctrl Pts',(178.775013624706,-1.77049869726083,
135.39492475452));
#202741=CARTESIAN_POINT('Ctrl Pts',(178.767248871759,-1.64137841218754,
135.440637137631));
#202742=CARTESIAN_POINT('Ctrl Pts',(178.759491830874,-1.51238637120182,
135.486304118559));
#202743=CARTESIAN_POINT('Ctrl Pts',(178.751734789989,-1.38135221148386,
135.526631460963));
#202744=CARTESIAN_POINT('Ctrl Pts',(178.743977749104,-1.24875779362943,
135.561438190546));
#202745=CARTESIAN_POINT('Ctrl Pts',(178.736226557863,-1.11626336625679,
135.596218672103));
#202746=CARTESIAN_POINT('Ctrl Pts',(178.728475366623,-0.982211399327259,
135.625486728446));
#202747=CARTESIAN_POINT('Ctrl Pts',(178.720724175383,-0.847100147526754,
135.649110807468));
#202748=CARTESIAN_POINT('Ctrl Pts',(178.712976278606,-0.712046321612475,
135.672724845628));
#202749=CARTESIAN_POINT('Ctrl Pts',(178.705228381829,-0.575934490605304,
135.690699610382));
#202750=CARTESIAN_POINT('Ctrl Pts',(178.697480485052,-0.439274155356607,
135.702954423847));
#202751=CARTESIAN_POINT('Ctrl Pts',(178.689734208968,-0.302642406504035,
135.715206673869));
#202752=CARTESIAN_POINT('Ctrl Pts',(178.681987932884,-0.165462770780643,
135.721741317591));
#202753=CARTESIAN_POINT('Ctrl Pts',(178.6742416568,-0.0282505490694401,
135.722529480972));
#202754=CARTESIAN_POINT('Ctrl Pts',(178.666495323534,0.10896268551119,135.723317650172));
#202755=CARTESIAN_POINT('Ctrl Pts',(178.658748990269,0.246208115600862,
135.718359252141));
#202756=CARTESIAN_POINT('Ctrl Pts',(178.651002657004,0.382970155287087,
135.707677548243));
#202757=CARTESIAN_POINT('Ctrl Pts',(178.643254589001,0.519762821883836,
135.69699345225));
#202758=CARTESIAN_POINT('Ctrl Pts',(178.635506520998,0.6560714929648,135.680583530403));
#202759=CARTESIAN_POINT('Ctrl Pts',(178.627758452995,0.791385816082687,
135.658522909105));
#202760=CARTESIAN_POINT('Ctrl Pts',(178.620002150253,0.926843952873513,
135.636438841517));
#202761=CARTESIAN_POINT('Ctrl Pts',(178.612245847511,1.06130524413376,135.608692140596));
#202762=CARTESIAN_POINT('Ctrl Pts',(178.604489544769,1.19426909797958,135.575409179896));
#202763=CARTESIAN_POINT('Ctrl Pts',(178.596729102255,1.32730391863779,135.542108455078));
#202764=CARTESIAN_POINT('Ctrl Pts',(178.588968659741,1.45883933457868,135.503265693328));
#202765=CARTESIAN_POINT('Ctrl Pts',(178.581208217227,1.58839099146788,135.459056861224));
#202766=CARTESIAN_POINT('Ctrl Pts',(178.573435316961,1.71815061617768,135.414777061178));
#202767=CARTESIAN_POINT('Ctrl Pts',(178.565662416696,1.84591975356253,135.365114118798));
#202768=CARTESIAN_POINT('Ctrl Pts',(178.55788951643,1.97123424056386,135.310292111866));
#202769=CARTESIAN_POINT('Ctrl Pts',(178.550399180668,2.09199323031518,135.257463022974));
#202770=CARTESIAN_POINT('Ctrl Pts',(178.542908844906,2.21047265971088,135.199843582111));
#202771=CARTESIAN_POINT('Ctrl Pts',(178.535418509144,2.32628135749008,135.137673219755));
#202772=CARTESIAN_POINT('Ctrl Pts',(178.527644175025,2.44648097724423,135.073145649215));
#202773=CARTESIAN_POINT('Ctrl Pts',(178.519869840906,2.56418410222925,135.003510844547));
#202774=CARTESIAN_POINT('Ctrl Pts',(178.512095506787,2.67892628550298,134.928986299897));
#202775=CARTESIAN_POINT('Ctrl Pts',(178.50433075384,2.7935270592906,134.854553600087));
#202776=CARTESIAN_POINT('Ctrl Pts',(178.496566000893,2.90517382725016,134.775243361484));
#202777=CARTESIAN_POINT('Ctrl Pts',(178.488801247946,3.01342561782393,134.691319468434));
#202778=CARTESIAN_POINT('Ctrl Pts',(178.481044207061,3.12156989119321,134.607478929778));
#202779=CARTESIAN_POINT('Ctrl Pts',(178.473287166176,3.22632559050266,134.519034093746));
#202780=CARTESIAN_POINT('Ctrl Pts',(178.465530125291,3.32727999952759,134.426292542277));
#202781=CARTESIAN_POINT('Ctrl Pts',(178.457778934051,3.42815827804732,134.333620927934));
#202782=CARTESIAN_POINT('Ctrl Pts',(178.45002774281,3.52524068528896,134.236659310972));
#202783=CARTESIAN_POINT('Ctrl Pts',(178.44227655157,3.61814722391349,134.135755780045));
#202784=CARTESIAN_POINT('Ctrl Pts',(178.434528654793,3.7110142747808,134.03489513581));
#202785=CARTESIAN_POINT('Ctrl Pts',(178.426780758016,3.79970872281605,133.930096196904));
#202786=CARTESIAN_POINT('Ctrl Pts',(178.419032861239,3.88388729377466,133.821744012456));
#202787=CARTESIAN_POINT('Ctrl Pts',(178.411286585155,3.9680482563909,133.713414492949));
#202788=CARTESIAN_POINT('Ctrl Pts',(178.403540309071,4.04769498113156,133.601533514834));
#202789=CARTESIAN_POINT('Ctrl Pts',(178.395794032987,4.12252464273607,133.486519008216));
#202790=CARTESIAN_POINT('Ctrl Pts',(178.388047699721,4.19735485671612,133.371503652587));
#202791=CARTESIAN_POINT('Ctrl Pts',(178.380301366456,4.26736772339354,133.253355050009));
#202792=CARTESIAN_POINT('Ctrl Pts',(178.372555033191,4.33230412643066,133.132519550846));
#202793=CARTESIAN_POINT('Ctrl Pts',(178.364806965188,4.39725507152499,133.011656991411));
#202794=CARTESIAN_POINT('Ctrl Pts',(178.357058897185,4.45712710576501,132.888106682375));
#202795=CARTESIAN_POINT('Ctrl Pts',(178.349310829182,4.5117075771597,132.762338605364));
#202796=CARTESIAN_POINT('Ctrl Pts',(178.34155452644,4.56634605732893,132.636436860543));
#202797=CARTESIAN_POINT('Ctrl Pts',(178.333798223698,4.61568158434171,132.508312998465));
#202798=CARTESIAN_POINT('Ctrl Pts',(178.326041920956,4.65954989770888,132.378456489253));
#202799=CARTESIAN_POINT('Ctrl Pts',(178.318281478442,4.70344162491577,132.248530671712));
#202800=CARTESIAN_POINT('Ctrl Pts',(178.310521035928,4.74186021461865,132.116870739491));
#202801=CARTESIAN_POINT('Ctrl Pts',(178.302760593414,4.77469190713373,131.983979307843));
#202802=CARTESIAN_POINT('Ctrl Pts',(178.294987693148,4.80757630399628,131.850874547072));
#202803=CARTESIAN_POINT('Ctrl Pts',(178.287214792883,4.83485580373609,131.716534719739));
#202804=CARTESIAN_POINT('Ctrl Pts',(178.279441892618,4.85646803786489,131.581471458886));
#202805=CARTESIAN_POINT('Ctrl Pts',(178.271951556856,4.87729461284501,131.451318087769));
#202806=CARTESIAN_POINT('Ctrl Pts',(178.264461221094,4.89285877098853,131.320493273089));
#202807=CARTESIAN_POINT('Ctrl Pts',(178.256970885332,4.90315051431672,131.189455536327));
#202808=CARTESIAN_POINT('Ctrl Pts',(178.249196486275,4.91383256144549,131.053448327918));
#202809=CARTESIAN_POINT('Ctrl Pts',(178.241422087219,4.91886823705911,130.916780895422));
#202810=CARTESIAN_POINT('Ctrl Pts',(178.233647688162,4.91818947873383,130.779961564882));
#202811=CARTESIAN_POINT('Ctrl Pts',(178.225882885497,4.91751155823925,130.643311118365));
#202812=CARTESIAN_POINT('Ctrl Pts',(178.218118082831,4.91113324050394,130.50650953409));
#202813=CARTESIAN_POINT('Ctrl Pts',(178.210353280166,4.89903818329087,130.37007045977));
#202814=CARTESIAN_POINT('Ctrl Pts',(178.202596204717,4.88695516258868,130.233767164089));
#202815=CARTESIAN_POINT('Ctrl Pts',(178.194839129269,4.86916675831516,130.097826047365));
#202816=CARTESIAN_POINT('Ctrl Pts',(178.18708205382,4.84570866602806,129.962760601834));
#202817=CARTESIAN_POINT('Ctrl Pts',(178.179330843123,4.822268309275,129.827797272782));
#202818=CARTESIAN_POINT('Ctrl Pts',(178.171579632426,4.79316686341908,129.693708680778));
#202819=CARTESIAN_POINT('Ctrl Pts',(178.163828421728,4.75849178917548,129.561002682436));
#202820=CARTESIAN_POINT('Ctrl Pts',(178.156080584143,4.72383180456287,129.428354434066));
#202821=CARTESIAN_POINT('Ctrl Pts',(178.148332746558,4.68360311496809,129.297087959994));
#202822=CARTESIAN_POINT('Ctrl Pts',(178.140584908972,4.63794412274852,129.167700183401));
#202823=CARTESIAN_POINT('Ctrl Pts',(178.132838713596,4.59229480827461,129.038339831459));
#202824=CARTESIAN_POINT('Ctrl Pts',(178.125092518219,4.54121761075637,128.910857753318));
#202825=CARTESIAN_POINT('Ctrl Pts',(178.117346322843,4.48490045673777,128.785734610686));
#202826=CARTESIAN_POINT('Ctrl Pts',(178.109600091816,4.42858304352998,128.660610892198));
#202827=CARTESIAN_POINT('Ctrl Pts',(178.101853860789,4.36702578624526,128.537846487337));
#202828=CARTESIAN_POINT('Ctrl Pts',(178.094107629763,4.30046414392161,128.41790064318));
#202829=CARTESIAN_POINT('Ctrl Pts',(178.086359685563,4.23388778068198,128.297928271543));
#202830=CARTESIAN_POINT('Ctrl Pts',(178.078611741363,4.16230501986083,128.180776042692));
#202831=CARTESIAN_POINT('Ctrl Pts',(178.070863797163,4.08599631251719,128.066876883076));
#202832=CARTESIAN_POINT('Ctrl Pts',(178.063107919224,4.00960946659292,127.952861093014));
#202833=CARTESIAN_POINT('Ctrl Pts',(178.055352041285,3.92848722617181,127.842105350861));
#202834=CARTESIAN_POINT('Ctrl Pts',(178.047596163346,3.84295255436162,127.735012359804));
#202835=CARTESIAN_POINT('Ctrl Pts',(178.039836154527,3.75737232568789,127.627862329646));
#202836=CARTESIAN_POINT('Ctrl Pts',(178.032076145708,3.6673752392277,127.524379232517));
#202837=CARTESIAN_POINT('Ctrl Pts',(178.024316136889,3.57332260510824,127.424930396016));
#202838=CARTESIAN_POINT('Ctrl Pts',(178.016544381083,3.47912759550359,127.325331015339));
#202839=CARTESIAN_POINT('Ctrl Pts',(178.008772625278,3.38086505267233,127.229778369216));
#202840=CARTESIAN_POINT('Ctrl Pts',(178.001000869473,3.27893153455889,127.138601343667));
#202841=CARTESIAN_POINT('Ctrl Pts',(177.994662241379,3.19579476627145,127.064237548652));
#202842=CARTESIAN_POINT('Ctrl Pts',(177.988323613286,3.11021677117177,126.992783713995));
#202843=CARTESIAN_POINT('Ctrl Pts',(177.981984985192,3.02242700330697,126.924396948641));
#202844=CARTESIAN_POINT('Ctrl Pts',(179.180279212536,-4.76405452823405,
129.582490119308));
#202845=CARTESIAN_POINT('Ctrl Pts',(179.172592770908,-4.79783235438911,
129.714189350837));
#202846=CARTESIAN_POINT('Ctrl Pts',(179.16490632928,-4.82611955095255,129.847191517955));
#202847=CARTESIAN_POINT('Ctrl Pts',(179.157219887652,-4.84884024883698,
129.980994779218));
#202848=CARTESIAN_POINT('Ctrl Pts',(179.149373333716,-4.87203422987842,
130.117585227311));
#202849=CARTESIAN_POINT('Ctrl Pts',(179.141526779781,-4.88942719215613,
130.255010073371));
#202850=CARTESIAN_POINT('Ctrl Pts',(179.133680225846,-4.90099431101235,
130.392732355751));
#202851=CARTESIAN_POINT('Ctrl Pts',(179.125833671911,-4.91256142986858,
130.530454638131));
#202852=CARTESIAN_POINT('Ctrl Pts',(179.117987117976,-4.91830275159455,
130.668473919319));
#202853=CARTESIAN_POINT('Ctrl Pts',(179.11014056404,-4.9182496345238,130.80625666781));
#202854=CARTESIAN_POINT('Origin',(213.235140564004,0.,130.804360617566));
#202855=CARTESIAN_POINT('',(180.930009319727,-4.76405452823406,129.582490119308));
#202856=CARTESIAN_POINT('',(180.584985772263,-4.76405452823404,129.582490119308));
#202857=CARTESIAN_POINT('',(213.235140564004,-4.76405452823405,129.582490119308));
#202858=CARTESIAN_POINT('',(180.514859436037,-4.91824986164052,130.805527225028));
#202859=CARTESIAN_POINT('Ctrl Pts',(180.584985772263,-4.76405452823404,
129.582490119308));
#202860=CARTESIAN_POINT('Ctrl Pts',(180.57727395094,-4.79793105739994,129.714574192378));
#202861=CARTESIAN_POINT('Ctrl Pts',(180.569562129616,-4.82628395215226,
129.847965328554));
#202862=CARTESIAN_POINT('Ctrl Pts',(180.561850308293,-4.84903779404517,
129.982158979024));
#202863=CARTESIAN_POINT('Ctrl Pts',(180.55401849625,-4.8721456703155,130.118440591857));
#202864=CARTESIAN_POINT('Ctrl Pts',(180.546186684208,-4.889478756331,130.255549475578));
#202865=CARTESIAN_POINT('Ctrl Pts',(180.538354872165,-4.90101294444811,
130.392954272389));
#202866=CARTESIAN_POINT('Ctrl Pts',(180.530523060122,-4.91254713256523,
130.5303590692));
#202867=CARTESIAN_POINT('Ctrl Pts',(180.522691248079,-4.91828246897984,
130.668059355764));
#202868=CARTESIAN_POINT('Ctrl Pts',(180.514859436037,-4.91824986164052,
130.805527225028));
#202869=CARTESIAN_POINT('Ctrl Pts',(180.514859435991,-4.91824986164033,
130.805527225829));
#202870=CARTESIAN_POINT('Ctrl Pts',(180.511286581325,-4.91823498623681,
130.86823975205));
#202871=CARTESIAN_POINT('Ctrl Pts',(180.507713726659,-4.91702069103772,
130.930936615505));
#202872=CARTESIAN_POINT('Ctrl Pts',(180.504140871993,-4.9146084703115,130.993587058748));
#202873=CARTESIAN_POINT('Ctrl Pts',(180.496366537874,-4.90935961144405,
131.129910957714));
#202874=CARTESIAN_POINT('Ctrl Pts',(180.488592203755,-4.89842600811054,
131.266232225206));
#202875=CARTESIAN_POINT('Ctrl Pts',(180.480817869636,-4.88179933162287,
131.402038079301));
#202876=CARTESIAN_POINT('Ctrl Pts',(180.473053116689,-4.86519314602801,
131.537676564819));
#202877=CARTESIAN_POINT('Ctrl Pts',(180.465288363742,-4.84290789448837,
131.672800516459));
#202878=CARTESIAN_POINT('Ctrl Pts',(180.457523610795,-4.81498723479294,
131.80689789432));
#202879=CARTESIAN_POINT('Ctrl Pts',(180.44976656991,-4.78709430629035,131.940862084775));
#202880=CARTESIAN_POINT('Ctrl Pts',(180.442009529025,-4.75357718742527,
132.073801350235));
#202881=CARTESIAN_POINT('Ctrl Pts',(180.43425248814,-4.714531200007,132.205209869506));
#202882=CARTESIAN_POINT('Ctrl Pts',(180.4265012969,-4.67551465747153,132.33651929259));
#202883=CARTESIAN_POINT('Ctrl Pts',(180.41875010566,-4.63097765615341,132.466299893888));
#202884=CARTESIAN_POINT('Ctrl Pts',(180.41099891442,-4.58106627286169,132.594057481884));
#202885=CARTESIAN_POINT('Ctrl Pts',(180.403251017643,-4.53117610323931,
132.721760769497));
#202886=CARTESIAN_POINT('Ctrl Pts',(180.395503120866,-4.47591623682387,
132.847442390555));
#202887=CARTESIAN_POINT('Ctrl Pts',(180.387755224089,-4.41548207553511,
132.970624937341));
#202888=CARTESIAN_POINT('Ctrl Pts',(180.380008948005,-4.35506055577006,
133.093781716993));
#202889=CARTESIAN_POINT('Ctrl Pts',(180.37226267192,-4.28946706608026,133.21444011138));
#202890=CARTESIAN_POINT('Ctrl Pts',(180.364516395836,-4.21894430230164,
133.332144634561));
#202891=CARTESIAN_POINT('Ctrl Pts',(180.356770062571,-4.14842101794008,
133.449850026611));
#202892=CARTESIAN_POINT('Ctrl Pts',(180.349023729306,-4.07296858782303,
133.56460116857));
#202893=CARTESIAN_POINT('Ctrl Pts',(180.34127739604,-3.99287442351235,133.675969382799));
#202894=CARTESIAN_POINT('Ctrl Pts',(180.333529328037,-3.91276232266898,
133.787362537167));
#202895=CARTESIAN_POINT('Ctrl Pts',(180.325781260035,-3.82800664740718,
133.895370938959));
#202896=CARTESIAN_POINT('Ctrl Pts',(180.318033192032,-3.73893643047199,
133.999597296028));
#202897=CARTESIAN_POINT('Ctrl Pts',(180.31027688929,-3.64977154865013,134.10393442611));
#202898=CARTESIAN_POINT('Ctrl Pts',(180.302520586548,-3.55628321943548,
134.204481184188));
#202899=CARTESIAN_POINT('Ctrl Pts',(180.294764283806,-3.45883921953503,
134.300875212975));
#202900=CARTESIAN_POINT('Ctrl Pts',(180.287003841292,-3.36134321083779,
134.397320690157));
#202901=CARTESIAN_POINT('Ctrl Pts',(180.279243398778,-3.25988761365962,
134.489608758661));
#202902=CARTESIAN_POINT('Ctrl Pts',(180.271482956264,-3.15487417386967,
134.577416674604));
#202903=CARTESIAN_POINT('Ctrl Pts',(180.263710055998,-3.04969215718354,
134.665365547608));
#202904=CARTESIAN_POINT('Ctrl Pts',(180.255937155733,-2.94094119510187,
134.748819658113));
#202905=CARTESIAN_POINT('Ctrl Pts',(180.248164255467,-2.82905368442206,
134.827498486588));
#202906=CARTESIAN_POINT('Ctrl Pts',(180.240673919705,-2.72123356658074,
134.90331714147));
#202907=CARTESIAN_POINT('Ctrl Pts',(180.233183583943,-2.61050124275258,
134.974701506813));
#202908=CARTESIAN_POINT('Ctrl Pts',(180.225693248181,-2.49726436005296,
135.041441426155));
#202909=CARTESIAN_POINT('Ctrl Pts',(180.217918914062,-2.37973406653057,
135.110711809822));
#202910=CARTESIAN_POINT('Ctrl Pts',(180.210144579943,-2.259133243701,135.175198034593));
#202911=CARTESIAN_POINT('Ctrl Pts',(180.202370245824,-2.13588880765785,
135.234615922153));
#202912=CARTESIAN_POINT('Ctrl Pts',(180.194605492877,-2.01279625936746,
135.293960582477));
#202913=CARTESIAN_POINT('Ctrl Pts',(180.186840739929,-1.88706692913862,
135.348249165653));
#202914=CARTESIAN_POINT('Ctrl Pts',(180.179075986982,-1.75915520874346,
135.397241632142));
#202915=CARTESIAN_POINT('Ctrl Pts',(180.171318946097,-1.63137053207232,
135.446185438622));
#202916=CARTESIAN_POINT('Ctrl Pts',(180.163561905212,-1.5014081415564,135.48984345747));
#202917=CARTESIAN_POINT('Ctrl Pts',(180.155804864327,-1.36974512266039,
135.528022476913));
#202918=CARTESIAN_POINT('Ctrl Pts',(180.148053673087,-1.23818139187112,
135.56617270526));
#202919=CARTESIAN_POINT('Ctrl Pts',(180.140302481847,-1.10491995933232,
135.598852049766));
#202920=CARTESIAN_POINT('Ctrl Pts',(180.132551290607,-0.970455560445589,
135.625916286404));
#202921=CARTESIAN_POINT('Ctrl Pts',(180.12480339383,-0.836048312515253,
135.652969020018));
#202922=CARTESIAN_POINT('Ctrl Pts',(180.117055497053,-0.700439497635642,
135.674411315488));
#202923=CARTESIAN_POINT('Ctrl Pts',(180.109307600276,-0.564136391950636,
135.69014951945));
#202924=CARTESIAN_POINT('Ctrl Pts',(180.101561324192,-0.427861797936961,
135.705884431319));
#202925=CARTESIAN_POINT('Ctrl Pts',(180.093815048108,-0.290893590128375,
135.71591758015));
#202926=CARTESIAN_POINT('Ctrl Pts',(180.086068772024,-0.153746164773559,
135.720206951547));
#202927=CARTESIAN_POINT('Ctrl Pts',(180.078322438758,-0.0165977270276053,
135.724496354607));
#202928=CARTESIAN_POINT('Ctrl Pts',(180.070576105493,0.120729540130282,
135.723041883407));
#202929=CARTESIAN_POINT('Ctrl Pts',(180.062829772227,0.257719625092028,
135.715853634699));
#202930=CARTESIAN_POINT('Ctrl Pts',(180.055081704225,0.394740388033409,
135.708663776232));
#202931=CARTESIAN_POINT('Ctrl Pts',(180.047333636222,0.531423428169907,
135.695737605649));
#202932=CARTESIAN_POINT('Ctrl Pts',(180.039585568219,0.667256642130682,
135.677137201407));
#202933=CARTESIAN_POINT('Ctrl Pts',(180.031829265477,0.803234221247715,
135.658517028435));
#202934=CARTESIAN_POINT('Ctrl Pts',(180.024072962735,0.93835978197096,135.634210628072));
#202935=CARTESIAN_POINT('Ctrl Pts',(180.016316659993,1.07212967055861,135.604331558312));
#202936=CARTESIAN_POINT('Ctrl Pts',(180.008556217479,1.20597095616365,135.574436541194));
#202937=CARTESIAN_POINT('Ctrl Pts',(180.000795774965,1.33845475039577,135.538963029203));
#202938=CARTESIAN_POINT('Ctrl Pts',(179.99303533245,1.46909236623006,135.498074571567));
#202939=CARTESIAN_POINT('Ctrl Pts',(179.985262432185,1.59993969316269,135.457120476149));
#202940=CARTESIAN_POINT('Ctrl Pts',(179.97748953192,1.72893455126841,135.41073419697));
#202941=CARTESIAN_POINT('Ctrl Pts',(179.969716631654,1.85560721049188,135.359127894044));
#202942=CARTESIAN_POINT('Ctrl Pts',(179.962226295892,1.97767499948376,135.309397610217));
#202943=CARTESIAN_POINT('Ctrl Pts',(179.95473596013,2.09758621357152,135.254820363207));
#202944=CARTESIAN_POINT('Ctrl Pts',(179.947245624368,2.21494369894812,135.195625523375));
#202945=CARTESIAN_POINT('Ctrl Pts',(179.939471290249,2.33675082905244,135.134186293199));
#202946=CARTESIAN_POINT('Ctrl Pts',(179.93169695613,2.45619260687545,135.067577785012));
#202947=CARTESIAN_POINT('Ctrl Pts',(179.923922622011,2.57279918657586,134.996005570094));
#202948=CARTESIAN_POINT('Ctrl Pts',(179.916157869064,2.68926205908817,134.924521561534));
#202949=CARTESIAN_POINT('Ctrl Pts',(179.908393116117,2.8028963557451,134.848086220452));
#202950=CARTESIAN_POINT('Ctrl Pts',(179.900628363169,2.9132545146317,134.76695209228));
#202951=CARTESIAN_POINT('Ctrl Pts',(179.892871322284,3.02350306423898,134.685898547668));
#202952=CARTESIAN_POINT('Ctrl Pts',(179.8851142814,3.1304816385372,134.600155733395));
#202953=CARTESIAN_POINT('Ctrl Pts',(179.877357240515,3.2337698066414,134.51002059929));
#202954=CARTESIAN_POINT('Ctrl Pts',(179.869606049274,3.33698008433468,134.419953436792));
#202955=CARTESIAN_POINT('Ctrl Pts',(179.861854858034,3.43650520177386,134.32550080338));
#202956=CARTESIAN_POINT('Ctrl Pts',(179.854103666794,3.53195640262972,134.22700097735));
#202957=CARTESIAN_POINT('Ctrl Pts',(179.846355770017,3.627367034179,134.128543016374));
#202958=CARTESIAN_POINT('Ctrl Pts',(179.83860787324,3.71870692150715,134.026041564233));
#202959=CARTESIAN_POINT('Ctrl Pts',(179.830859976463,3.8056230762406,133.919872784784));
#202960=CARTESIAN_POINT('Ctrl Pts',(179.823113700379,3.89252104998818,133.813726213555));
#202961=CARTESIAN_POINT('Ctrl Pts',(179.815367424295,3.97499688420821,133.703914143201));
#202962=CARTESIAN_POINT('Ctrl Pts',(179.807621148211,4.05273718726214,133.590846640047));
#202963=CARTESIAN_POINT('Ctrl Pts',(179.799874814945,4.13047806417734,133.477778302254));
#202964=CARTESIAN_POINT('Ctrl Pts',(179.79212848168,4.20348311866762,133.361454805873));
#202965=CARTESIAN_POINT('Ctrl Pts',(179.784382148415,4.27148192853796,133.242315743624));
#202966=CARTESIAN_POINT('Ctrl Pts',(179.776634080412,4.33949596627027,133.123150001009));
#202967=CARTESIAN_POINT('Ctrl Pts',(179.768886012409,4.40250133473337,133.001167777338));
#202968=CARTESIAN_POINT('Ctrl Pts',(179.761137944406,4.4602734579108,132.876833474603));
#202969=CARTESIAN_POINT('Ctrl Pts',(179.753381641664,4.51810698198826,132.752367027892));
#202970=CARTESIAN_POINT('Ctrl Pts',(179.745625338922,4.57069598516582,132.625543863588));
#202971=CARTESIAN_POINT('Ctrl Pts',(179.73786903618,4.61786376985074,132.496849100717));
#202972=CARTESIAN_POINT('Ctrl Pts',(179.730108593666,4.66505672940257,132.368085649577));
#202973=CARTESIAN_POINT('Ctrl Pts',(179.722348151152,4.7068225859822,132.237448981634));
#202974=CARTESIAN_POINT('Ctrl Pts',(179.714587708638,4.74303479091117,132.105438645474));
#202975=CARTESIAN_POINT('Ctrl Pts',(179.706814808372,4.77930512688626,131.973216394604));
#202976=CARTESIAN_POINT('Ctrl Pts',(179.699041908107,4.81000390816578,131.839616450211));
#202977=CARTESIAN_POINT('Ctrl Pts',(179.691269007841,4.83505573040974,131.705148687165));
#202978=CARTESIAN_POINT('Ctrl Pts',(179.683778672079,4.85919685581355,131.575569166008));
#202979=CARTESIAN_POINT('Ctrl Pts',(179.676288336317,4.8780944124047,131.445184130401));
#202980=CARTESIAN_POINT('Ctrl Pts',(179.668798000555,4.89172670463108,131.314451697373));
#202981=CARTESIAN_POINT('Ctrl Pts',(179.661023666436,4.90587586936059,131.178762504413));
#202982=CARTESIAN_POINT('Ctrl Pts',(179.653249332317,4.91439744341293,131.042269228285));
#202983=CARTESIAN_POINT('Ctrl Pts',(179.645474998198,4.917210416574,130.905478279901));
#202984=CARTESIAN_POINT('Ctrl Pts',(179.637710245251,4.92001992299706,130.768855914136));
#202985=CARTESIAN_POINT('Ctrl Pts',(179.629945492304,4.91713481879837,130.631936993176));
#202986=CARTESIAN_POINT('Ctrl Pts',(179.622180739356,4.9085256594554,130.495234570511));
#202987=CARTESIAN_POINT('Ctrl Pts',(179.614423698471,4.89992505085085,130.358667922619));
#202988=CARTESIAN_POINT('Ctrl Pts',(179.606666657586,4.88561172534523,130.222317732772));
#202989=CARTESIAN_POINT('Ctrl Pts',(179.598909616701,4.86560826207741,130.086698230016));
#202990=CARTESIAN_POINT('Ctrl Pts',(179.591158425461,4.84561988357684,129.951180998982));
#202991=CARTESIAN_POINT('Ctrl Pts',(179.583407234221,4.81994996506197,129.81639374349));
#202992=CARTESIAN_POINT('Ctrl Pts',(179.575656042981,4.78867297735071,129.68284638293));
#202993=CARTESIAN_POINT('Ctrl Pts',(179.567908146204,4.75740928319356,129.549355783561));
#202994=CARTESIAN_POINT('Ctrl Pts',(179.560160249427,4.7205433487172,129.417104410853));
#202995=CARTESIAN_POINT('Ctrl Pts',(179.55241235265,4.67820085238921,129.286592569673));
#202996=CARTESIAN_POINT('Ctrl Pts',(179.544666076566,4.63586721319865,129.156108028757));
#202997=CARTESIAN_POINT('Ctrl Pts',(179.536919800482,4.58805941135035,129.027362667255));
#202998=CARTESIAN_POINT('Ctrl Pts',(179.529173524397,4.53495305142171,128.900841801294));
#202999=CARTESIAN_POINT('Ctrl Pts',(179.521427191132,4.48184629947401,128.774320001385));
#203000=CARTESIAN_POINT('Ctrl Pts',(179.513680857867,4.42344106271525,128.650023090278));
#203001=CARTESIAN_POINT('Ctrl Pts',(179.505934524601,4.35996101314982,128.528416192429));
#203002=CARTESIAN_POINT('Ctrl Pts',(179.498186456598,4.29646674766747,128.406782061558));
#203003=CARTESIAN_POINT('Ctrl Pts',(179.490438388595,4.22789558882288,128.28783948919));
#203004=CARTESIAN_POINT('Ctrl Pts',(179.482690320592,4.15451686234194,128.172028438107));
#203005=CARTESIAN_POINT('Ctrl Pts',(179.474934017851,4.08106014807724,128.056094301661));
#203006=CARTESIAN_POINT('Ctrl Pts',(179.467177715109,4.00278586890444,127.943298665755));
#203007=CARTESIAN_POINT('Ctrl Pts',(179.459421412367,3.92000665983544,127.834052409762));
#203008=CARTESIAN_POINT('Ctrl Pts',(179.451660969853,3.83718326901008,127.724747845754));
#203009=CARTESIAN_POINT('Ctrl Pts',(179.443900527339,3.74985040611597,127.618996737741));
#203010=CARTESIAN_POINT('Ctrl Pts',(179.436140084824,3.65835995287435,127.517175572926));
#203011=CARTESIAN_POINT('Ctrl Pts',(179.428367184559,3.56672263103505,127.415190955737));
#203012=CARTESIAN_POINT('Ctrl Pts',(179.420594284294,3.47091465521116,127.317149168308));
#203013=CARTESIAN_POINT('Ctrl Pts',(179.412821384028,3.37132423968277,127.223389250265));
#203014=CARTESIAN_POINT('Ctrl Pts',(179.405331048266,3.27535418661257,127.133037741411));
#203015=CARTESIAN_POINT('Ctrl Pts',(179.397840712504,3.17587215439751,127.046662395268));
#203016=CARTESIAN_POINT('Ctrl Pts',(179.390350376742,3.07325184289293,126.964529088364));
#203017=CARTESIAN_POINT('Ctrl Pts',(179.382576042623,2.96674065108638,126.879281672164));
#203018=CARTESIAN_POINT('Ctrl Pts',(179.374801708504,2.85651111111605,126.798334280789));
#203019=CARTESIAN_POINT('Ctrl Pts',(179.367027374385,2.74294549282422,126.722028797895));
#203020=CARTESIAN_POINT('Ctrl Pts',(179.359262621438,2.62951983400729,126.645817354689));
#203021=CARTESIAN_POINT('Ctrl Pts',(179.351497868491,2.51276659876644,126.574236653353));
#203022=CARTESIAN_POINT('Ctrl Pts',(179.343733115544,2.39310151804933,126.507588784339));
#203023=CARTESIAN_POINT('Ctrl Pts',(179.335976074659,2.27355529037732,126.441007110929));
#203024=CARTESIAN_POINT('Ctrl Pts',(179.328219033774,2.15110331196261,126.3793487089));
#203025=CARTESIAN_POINT('Ctrl Pts',(179.320461992889,2.0261904228423,126.322872535145));
#203026=CARTESIAN_POINT('Ctrl Pts',(179.312710801649,1.90137173150333,126.266438950512));
#203027=CARTESIAN_POINT('Ctrl Pts',(179.304959610409,1.77409617810434,126.215179976013));
#203028=CARTESIAN_POINT('Ctrl Pts',(179.297208419168,1.64483302556683,126.169308581126));
#203029=CARTESIAN_POINT('Ctrl Pts',(179.289460522391,1.51562481331742,126.123456682806));
#203030=CARTESIAN_POINT('Ctrl Pts',(179.281712625614,1.3844310498194,126.08298794021));
#203031=CARTESIAN_POINT('Ctrl Pts',(179.273964728837,1.25174058800957,126.048067043487));
#203032=CARTESIAN_POINT('Ctrl Pts',(179.266218452753,1.11907788218387,126.013153451461));
#203033=CARTESIAN_POINT('Ctrl Pts',(179.258472176669,0.984919478625015,
125.983785496472));
#203034=CARTESIAN_POINT('Ctrl Pts',(179.250725900585,0.849768606098465,
125.960077762634));
#203035=CARTESIAN_POINT('Ctrl Pts',(179.24297956732,0.714616735918967,125.936369853791));
#203036=CARTESIAN_POINT('Ctrl Pts',(179.235233234054,0.578472767238265,
125.918322317024));
#203037=CARTESIAN_POINT('Ctrl Pts',(179.227486900789,0.441848922615117,
125.905998381871));
#203038=CARTESIAN_POINT('Ctrl Pts',(179.219738832786,0.305194482029227,
125.893671686858));
#203039=CARTESIAN_POINT('Ctrl Pts',(179.211990764783,0.168060340967948,
125.887071179131));
#203040=CARTESIAN_POINT('Ctrl Pts',(179.20424269678,0.0309622297147287,
125.88620807796));
#203041=CARTESIAN_POINT('Ctrl Pts',(179.196486394038,-0.10628159104269,
125.885344059475));
#203042=CARTESIAN_POINT('Ctrl Pts',(179.188730091296,-0.243488913916986,
125.890229630992));
#203043=CARTESIAN_POINT('Ctrl Pts',(179.180973788555,-0.38014506759449,
125.900823854159));
#203044=CARTESIAN_POINT('Ctrl Pts',(179.17321334604,-0.51687415877599,125.911423731781));
#203045=CARTESIAN_POINT('Ctrl Pts',(179.165452903526,-0.653051106591565,
125.927738285734));
#203046=CARTESIAN_POINT('Ctrl Pts',(179.157692461012,-0.788168961031706,
125.949674968488));
#203047=CARTESIAN_POINT('Ctrl Pts',(179.149919560747,-0.923503718646903,
125.971646865952));
#203048=CARTESIAN_POINT('Ctrl Pts',(179.142146660481,-1.05777560227164,
125.999258848526));
#203049=CARTESIAN_POINT('Ctrl Pts',(179.134373760216,-1.19048952896382,
126.032367559741));
#203050=CARTESIAN_POINT('Ctrl Pts',(179.126883424454,-1.3183789701352,126.064272685909));
#203051=CARTESIAN_POINT('Ctrl Pts',(179.119393088692,-1.44482146351932,
126.101281752664));
#203052=CARTESIAN_POINT('Ctrl Pts',(179.11190275293,-1.56939132576419,126.143224068492));
#203053=CARTESIAN_POINT('Ctrl Pts',(179.104128393758,-1.69868470883825,
126.186756780254));
#203054=CARTESIAN_POINT('Ctrl Pts',(179.096354034586,-1.82637020688291,
126.235742147257));
#203055=CARTESIAN_POINT('Ctrl Pts',(179.088579675415,-1.95195355254964,
126.290043350117));
#203056=CARTESIAN_POINT('Ctrl Pts',(179.080814903304,-2.07738203333556,
126.34427759068));
#203057=CARTESIAN_POINT('Ctrl Pts',(179.073050131194,-2.2007131642445,126.403814470295));
#203058=CARTESIAN_POINT('Ctrl Pts',(179.065285359084,-2.32146807181828,
126.46846750841));
#203059=CARTESIAN_POINT('Ctrl Pts',(179.0575283049,-2.44210295301114,126.533056283545));
#203060=CARTESIAN_POINT('Ctrl Pts',(179.049771250716,-2.56016636431176,
126.602750913835));
#203061=CARTESIAN_POINT('Ctrl Pts',(179.042014196532,-2.6751999888338,126.677317113768));
#203062=CARTESIAN_POINT('Ctrl Pts',(179.034262997838,-2.79014677906578,
126.751827026654));
#203063=CARTESIAN_POINT('Ctrl Pts',(179.026511799144,-2.9020680080604,126.831200977799));
#203064=CARTESIAN_POINT('Ctrl Pts',(179.018760600451,-3.01053084945795,
126.915159277064));
#203065=CARTESIAN_POINT('Ctrl Pts',(179.011012726883,-3.11894716223425,
126.999081559718));
#203066=CARTESIAN_POINT('Ctrl Pts',(179.003264853315,-3.22390772980016,
127.087584040042));
#203067=CARTESIAN_POINT('Ctrl Pts',(178.995516979748,-3.32500976055551,
127.180344453873));
#203068=CARTESIAN_POINT('Ctrl Pts',(178.987770735199,-3.42609053423857,
127.273085364487));
#203069=CARTESIAN_POINT('Ctrl Pts',(178.98002449065,-3.5233140969294,127.370082163717));
#203070=CARTESIAN_POINT('Ctrl Pts',(178.972278246101,-3.61631204294623,
127.470973410753));
#203071=CARTESIAN_POINT('Ctrl Pts',(178.964531952702,-3.70931057542868,
127.571865294032));
#203072=CARTESIAN_POINT('Ctrl Pts',(178.956785659304,-3.79808317311763,
127.676651386634));
#203073=CARTESIAN_POINT('Ctrl Pts',(178.949039365905,-3.8822997754526,127.784934924488));
#203074=CARTESIAN_POINT('Ctrl Pts',(178.941291346114,-3.96653514688435,
127.893242595163));
#203075=CARTESIAN_POINT('Ctrl Pts',(178.933543326323,-4.04621226256158,
128.005048953545));
#203076=CARTESIAN_POINT('Ctrl Pts',(178.925795306531,-4.12104292365446,
128.11992617361));
#203077=CARTESIAN_POINT('Ctrl Pts',(178.918039169389,-4.19595198242991,
128.234923746853));
#203078=CARTESIAN_POINT('Ctrl Pts',(178.910283032246,-4.26600423054555,
128.352998280208));
#203079=CARTESIAN_POINT('Ctrl Pts',(178.902526895103,-4.33095593282109,
128.473694667572));
#203080=CARTESIAN_POINT('Ctrl Pts',(178.894766621628,-4.39594227369947,
128.594455422059));
#203081=CARTESIAN_POINT('Ctrl Pts',(178.887006348154,-4.4558224781109,128.717840465114));
#203082=CARTESIAN_POINT('Ctrl Pts',(178.87924607468,-4.51040040079451,128.843373293024));
#203083=CARTESIAN_POINT('Ctrl Pts',(178.871473622124,-4.56506397883664,
128.969103133919));
#203084=CARTESIAN_POINT('Ctrl Pts',(178.863701169567,-4.61440850661788,
129.096987130188));
#203085=CARTESIAN_POINT('Ctrl Pts',(178.855928717011,-4.658287010806,129.226531353211));
#203086=CARTESIAN_POINT('Ctrl Pts',(178.848884041066,-4.69805693422395,
129.343945652631));
#203087=CARTESIAN_POINT('Ctrl Pts',(178.841839365122,-4.73333712484633,
129.462723429701));
#203088=CARTESIAN_POINT('Ctrl Pts',(178.834794689177,-4.76405452823405,
129.582490119308));
#203089=CARTESIAN_POINT('',(180.860140563953,-4.91824868670176,130.80795481517));
#203090=CARTESIAN_POINT('Ctrl Pts',(180.860140563953,-4.91824868670176,
130.80795481517));
#203091=CARTESIAN_POINT('Ctrl Pts',(180.851235208711,-4.91813337062327,
130.96575169062));
#203092=CARTESIAN_POINT('Ctrl Pts',(180.842329853469,-4.91041999025756,
131.123241678084));
#203093=CARTESIAN_POINT('Ctrl Pts',(180.833424498227,-4.89522072462637,
131.279752161126));
#203094=CARTESIAN_POINT('Ctrl Pts',(180.824474260165,-4.87994485498848,
131.437051453996));
#203095=CARTESIAN_POINT('Ctrl Pts',(180.815524022103,-4.85710756303225,
131.593361207987));
#203096=CARTESIAN_POINT('Ctrl Pts',(180.806573784042,-4.82687215032326,
131.74801749744));
#203097=CARTESIAN_POINT('Ctrl Pts',(180.79756682713,-4.79644513177894,131.903653864388));
#203098=CARTESIAN_POINT('Ctrl Pts',(180.788559870219,-4.75852601683665,
132.057615609648));
#203099=CARTESIAN_POINT('Ctrl Pts',(180.779552913307,-4.71332967202739,
132.209247255443));
#203100=CARTESIAN_POINT('Ctrl Pts',(180.774035108754,-4.68564167489048,
132.302139204833));
#203101=CARTESIAN_POINT('Ctrl Pts',(180.768517304201,-4.65522348627133,
132.394157094063));
#203102=CARTESIAN_POINT('Ctrl Pts',(180.762999499647,-4.6221331923805,132.485154422408));
#203103=CARTESIAN_POINT('Ctrl Pts',(180.755225165528,-4.57551048251068,
132.613365493978));
#203104=CARTESIAN_POINT('Ctrl Pts',(180.747450831409,-4.52347530734763,
132.739838306069));
#203105=CARTESIAN_POINT('Ctrl Pts',(180.73967649729,-4.46617630640889,132.864082021682));
#203106=CARTESIAN_POINT('Ctrl Pts',(180.731911744343,-4.4089479213679,132.988172618018));
#203107=CARTESIAN_POINT('Ctrl Pts',(180.724146991396,-4.34646878029648,
133.11003923229));
#203108=CARTESIAN_POINT('Ctrl Pts',(180.716382238449,-4.27893680000363,
133.229207607393));
#203109=CARTESIAN_POINT('Ctrl Pts',(180.708625197564,-4.21147189342562,
133.348257622787));
#203110=CARTESIAN_POINT('Ctrl Pts',(180.700868156679,-4.13896432627984,
133.464614394248));
#203111=CARTESIAN_POINT('Ctrl Pts',(180.693111115794,-4.06165931338313,
133.577825361259));
#203112=CARTESIAN_POINT('Ctrl Pts',(180.685359924554,-3.9844125967981,133.690950954998));
#203113=CARTESIAN_POINT('Ctrl Pts',(180.677608733314,-3.90237585503431,
133.800935144591));
#203114=CARTESIAN_POINT('Ctrl Pts',(180.669857542074,-3.81583908314369,
133.90735194112));
#203115=CARTESIAN_POINT('Ctrl Pts',(180.662109645297,-3.72933909168942,
134.013723507672));
#203116=CARTESIAN_POINT('Ctrl Pts',(180.65436174852,-3.6383431203381,134.116530394143));
#203117=CARTESIAN_POINT('Ctrl Pts',(180.646613851742,-3.54318300903784,
134.215377654604));
#203118=CARTESIAN_POINT('Ctrl Pts',(180.638867575658,-3.44804280318141,
134.314204238349));
#203119=CARTESIAN_POINT('Ctrl Pts',(180.631121299574,-3.34874046091821,
134.409072562077));
#203120=CARTESIAN_POINT('Ctrl Pts',(180.62337502349,-3.24564616409112,134.499622995263));
#203121=CARTESIAN_POINT('Ctrl Pts',(180.615628690225,-3.14255110624534,
134.590174096871));
#203122=CARTESIAN_POINT('Ctrl Pts',(180.60788235696,-3.03566433172752,134.676406986332));
#203123=CARTESIAN_POINT('Ctrl Pts',(180.600136023694,-2.92539041717838,
134.758001214482));
#203124=CARTESIAN_POINT('Ctrl Pts',(180.592387955691,-2.81509180755061,
134.839613715093));
#203125=CARTESIAN_POINT('Ctrl Pts',(180.584639887688,-2.70140486273715,
134.916585254807));
#203126=CARTESIAN_POINT('Ctrl Pts',(180.576891819685,-2.58476420983551,
134.988637979555));
#203127=CARTESIAN_POINT('Ctrl Pts',(180.569135516943,-2.46799958986003,
135.060767282796));
#203128=CARTESIAN_POINT('Ctrl Pts',(180.561379214202,-2.34827532398418,
135.12796712223));
#203129=CARTESIAN_POINT('Ctrl Pts',(180.55362291146,-2.22605226619562,135.190004740231));
#203130=CARTESIAN_POINT('Ctrl Pts',(180.545862468946,-2.10376397428102,
135.252075469577));
#203131=CARTESIAN_POINT('Ctrl Pts',(180.538102026431,-1.97897458853601,
135.308978325326));
#203132=CARTESIAN_POINT('Ctrl Pts',(180.530341583917,-1.85216521453456,
135.360528643503));
#203133=CARTESIAN_POINT('Ctrl Pts',(180.522568683652,-1.72515227486836,
135.412161714826));
#203134=CARTESIAN_POINT('Ctrl Pts',(180.514795783386,-1.59611323530802,
135.458424946265));
#203135=CARTESIAN_POINT('Ctrl Pts',(180.507022883121,-1.46554549602716,
135.499183240581));
#203136=CARTESIAN_POINT('Ctrl Pts',(180.499532547359,-1.33972422294845,
135.538459868235));
#203137=CARTESIAN_POINT('Ctrl Pts',(180.492042211597,-1.21248376217569,
135.572624766855));
#203138=CARTESIAN_POINT('Ctrl Pts',(180.484551875835,-1.08427646179028,
135.601602285119));
#203139=CARTESIAN_POINT('Ctrl Pts',(180.476777541716,-0.951208142644003,
135.631678494795));
#203140=CARTESIAN_POINT('Ctrl Pts',(180.469003207597,-0.81667670073027,
135.656261472423));
#203141=CARTESIAN_POINT('Ctrl Pts',(180.461228873478,-0.68117543440742,
135.675210963251));
#203142=CARTESIAN_POINT('Ctrl Pts',(180.45346412053,-0.545841161285354,
135.694137100525));
#203143=CARTESIAN_POINT('Ctrl Pts',(180.445699367583,-0.409539825369746,
135.707443511412));
#203144=CARTESIAN_POINT('Ctrl Pts',(180.437934614636,-0.272777411462797,
135.715040361379));
#203145=CARTESIAN_POINT('Ctrl Pts',(180.430177573751,-0.13615083191333,
135.722629666048));
#203146=CARTESIAN_POINT('Ctrl Pts',(180.422420532866,0.000935526450582369,
135.724520673434));
#203147=CARTESIAN_POINT('Ctrl Pts',(180.414663491981,0.137968367048358,
135.720675069693));
#203148=CARTESIAN_POINT('Ctrl Pts',(180.406912300741,0.274897870115078,
135.716832365952));
#203149=CARTESIAN_POINT('Ctrl Pts',(180.399161109501,0.411773546516112,
135.707261672693));
#203150=CARTESIAN_POINT('Ctrl Pts',(180.391409918261,0.548080250301332,
135.691976713551));
#203151=CARTESIAN_POINT('Ctrl Pts',(180.383662021484,0.684329020101435,
135.676698250924));
#203152=CARTESIAN_POINT('Ctrl Pts',(180.375914124707,0.820008910547644,
135.655710396422));
#203153=CARTESIAN_POINT('Ctrl Pts',(180.36816622793,0.9546082748462,135.629078858468));
#203154=CARTESIAN_POINT('Ctrl Pts',(180.360419951846,1.08917948385937,135.602452891258));
#203155=CARTESIAN_POINT('Ctrl Pts',(180.352673675761,1.22267023300946,135.570185664586));
#203156=CARTESIAN_POINT('Ctrl Pts',(180.344927399677,1.35457786262363,135.532394233837));
#203157=CARTESIAN_POINT('Ctrl Pts',(180.337181066412,1.4864864659498,135.494602524121));
#203158=CARTESIAN_POINT('Ctrl Pts',(180.329434733147,1.61681155057666,135.451286636637));
#203159=CARTESIAN_POINT('Ctrl Pts',(180.321688399881,1.74506482999139,135.402613742572));
#203160=CARTESIAN_POINT('Ctrl Pts',(180.313940331878,1.87334683083893,135.35392994855));
#203161=CARTESIAN_POINT('Ctrl Pts',(180.306192263875,1.99955573777708,135.299886899446));
#203162=CARTESIAN_POINT('Ctrl Pts',(180.298444195872,2.12322285774621,135.240700072437));
#203163=CARTESIAN_POINT('Ctrl Pts',(180.29068789313,2.24702141260209,135.181450340963));
#203164=CARTESIAN_POINT('Ctrl Pts',(180.282931590389,2.36827243084956,135.117046079976));
#203165=CARTESIAN_POINT('Ctrl Pts',(180.275175287647,2.48653098406956,135.047749207804));
#203166=CARTESIAN_POINT('Ctrl Pts',(180.267414845133,2.60485265544017,134.978415349805));
#203167=CARTESIAN_POINT('Ctrl Pts',(180.259654402618,2.72017835070013,134.904183888821));
#203168=CARTESIAN_POINT('Ctrl Pts',(180.251893960104,2.83209265750178,134.825359777206));
#203169=CARTESIAN_POINT('Ctrl Pts',(180.244121059839,2.94418661908395,134.746409130129));
#203170=CARTESIAN_POINT('Ctrl Pts',(180.236348159573,3.05285793877241,134.662851338207));
#203171=CARTESIAN_POINT('Ctrl Pts',(180.228575259308,3.15772409849079,134.575031854934));
#203172=CARTESIAN_POINT('Ctrl Pts',(180.221084923546,3.25877810916079,134.490404831082));
#203173=CARTESIAN_POINT('Ctrl Pts',(180.213594587784,3.35629858303754,134.401820790026));
#203174=CARTESIAN_POINT('Ctrl Pts',(180.206104252022,3.44997736733326,134.309619413631));
#203175=CARTESIAN_POINT('Ctrl Pts',(180.198329917903,3.54720801120912,134.213922194025));
#203176=CARTESIAN_POINT('Ctrl Pts',(180.190555583784,3.6406078969809,134.114024781695));
#203177=CARTESIAN_POINT('Ctrl Pts',(180.182781249665,3.72979238454181,134.010266391402));
#203178=CARTESIAN_POINT('Ctrl Pts',(180.175016496718,3.81886696019247,133.906635874052));
#203179=CARTESIAN_POINT('Ctrl Pts',(180.167251743771,3.90373622193616,133.799154140003));
#203180=CARTESIAN_POINT('Ctrl Pts',(180.159486990823,3.98405109229198,133.688198330841));
#203181=CARTESIAN_POINT('Ctrl Pts',(180.151729949938,4.06428619278623,133.577352724553));
#203182=CARTESIAN_POINT('Ctrl Pts',(180.143972909054,4.1399756760726,133.463040224457));
#203183=CARTESIAN_POINT('Ctrl Pts',(180.136215868169,4.21080985828836,133.345671971934));
#203184=CARTESIAN_POINT('Ctrl Pts',(180.128464676928,4.28159062389636,133.228392227724));
#203185=CARTESIAN_POINT('Ctrl Pts',(180.120713485688,4.3475231750704,133.108061651164));
#203186=CARTESIAN_POINT('Ctrl Pts',(180.112962294448,4.40834060892407,132.985121067091));
#203187=CARTESIAN_POINT('Ctrl Pts',(180.105214397671,4.46913219374597,132.862232736046));
#203188=CARTESIAN_POINT('Ctrl Pts',(180.097466500894,4.52481281229799,132.736736953544));
#203189=CARTESIAN_POINT('Ctrl Pts',(180.089718604117,4.57516118934884,132.609099699532));
#203190=CARTESIAN_POINT('Ctrl Pts',(180.081972328033,4.62549903460459,132.481489144482));
#203191=CARTESIAN_POINT('Ctrl Pts',(180.074226051949,4.6705067135582,132.351738372381));
#203192=CARTESIAN_POINT('Ctrl Pts',(180.066479775865,4.71001100838992,132.220333556342));
#203193=CARTESIAN_POINT('Ctrl Pts',(180.058733442599,4.74951559483336,132.088927770302));
#203194=CARTESIAN_POINT('Ctrl Pts',(180.050987109334,4.78351660353165,131.955868290373));
#203195=CARTESIAN_POINT('Ctrl Pts',(180.043240776069,4.811890749551,131.821656285937));
#203196=CARTESIAN_POINT('Ctrl Pts',(180.035492708066,4.84027124976361,131.687414225652));
#203197=CARTESIAN_POINT('Ctrl Pts',(180.027744640063,4.86302229899824,131.552019509708));
#203198=CARTESIAN_POINT('Ctrl Pts',(180.01999657206,4.880071844258,131.415982933526));
#203199=CARTESIAN_POINT('Ctrl Pts',(180.012240269318,4.89713950997736,131.279801776052));
#203200=CARTESIAN_POINT('Ctrl Pts',(180.004483966576,4.90849351826859,131.142977784168));
#203201=CARTESIAN_POINT('Ctrl Pts',(179.996727663834,4.9141137337624,131.006026862009));
#203202=CARTESIAN_POINT('Ctrl Pts',(179.98896722132,4.91973694893445,130.869002845019));
#203203=CARTESIAN_POINT('Ctrl Pts',(179.981206778806,4.91962027373891,130.731852153537));
#203204=CARTESIAN_POINT('Ctrl Pts',(179.973446336292,4.91379573270794,130.595089119934));
#203205=CARTESIAN_POINT('Ctrl Pts',(179.965673436026,4.90796184160662,130.458106542167));
#203206=CARTESIAN_POINT('Ctrl Pts',(179.957900535761,4.89640180751873,130.321513255635));
#203207=CARTESIAN_POINT('Ctrl Pts',(179.950127635495,4.87919950989027,130.185817809681));
#203208=CARTESIAN_POINT('Ctrl Pts',(179.942637299733,4.8626225591104,130.055055234982));
#203209=CARTESIAN_POINT('Ctrl Pts',(179.935146963971,4.84080649473996,129.925126660408));
#203210=CARTESIAN_POINT('Ctrl Pts',(179.927656628209,4.81387053664267,129.796474949971));
#203211=CARTESIAN_POINT('Ctrl Pts',(179.91988229409,4.7859132935074,129.662945370831));
#203212=CARTESIAN_POINT('Ctrl Pts',(179.912107959971,4.75235169095122,129.530368410215));
#203213=CARTESIAN_POINT('Ctrl Pts',(179.904333625852,4.71326321258631,129.399251030601));
#203214=CARTESIAN_POINT('Ctrl Pts',(179.896568872905,4.67422290727756,129.268295241439));
#203215=CARTESIAN_POINT('Ctrl Pts',(179.888804119958,4.62966938940084,129.138795825271));
#203216=CARTESIAN_POINT('Ctrl Pts',(179.88103936701,4.57973127394808,129.011250325107));
#203217=CARTESIAN_POINT('Ctrl Pts',(179.873282326125,4.52984275773558,128.883831504932));
#203218=CARTESIAN_POINT('Ctrl Pts',(179.86552528524,4.47458042844114,128.758363100465));
#203219=CARTESIAN_POINT('Ctrl Pts',(179.857768244355,4.41412279926086,128.635327889471));
#203220=CARTESIAN_POINT('Ctrl Pts',(179.850017053115,4.35371076164904,128.512385460287));
#203221=CARTESIAN_POINT('Ctrl Pts',(179.842265861875,4.28811139405136,128.391872921809));
#203222=CARTESIAN_POINT('Ctrl Pts',(179.834514670635,4.21755130735877,128.274253103586));
#203223=CARTESIAN_POINT('Ctrl Pts',(179.826766773858,4.14702121058527,128.156683276924));
#203224=CARTESIAN_POINT('Ctrl Pts',(179.819018877081,4.07153478894331,128.042004059732));
#203225=CARTESIAN_POINT('Ctrl Pts',(179.811270980304,3.99136447989174,127.930653490672));
#203226=CARTESIAN_POINT('Ctrl Pts',(179.80352470422,3.91121094074054,127.819326213751));
#203227=CARTESIAN_POINT('Ctrl Pts',(179.795778428136,3.82637569128667,127.711326517104));
#203228=CARTESIAN_POINT('Ctrl Pts',(179.788032152051,3.7371741342777,127.607062922232));
#203229=CARTESIAN_POINT('Ctrl Pts',(179.780285818786,3.64797191880316,127.50279855771));
#203230=CARTESIAN_POINT('Ctrl Pts',(179.772539485521,3.5544035856207,127.402270647074));
#203231=CARTESIAN_POINT('Ctrl Pts',(179.764793152255,3.4568241442069,127.305853807722));
#203232=CARTESIAN_POINT('Ctrl Pts',(179.757045084252,3.35922285055371,127.209415376487));
#203233=CARTESIAN_POINT('Ctrl Pts',(179.749297016249,3.25760893928871,127.117090123255));
#203234=CARTESIAN_POINT('Ctrl Pts',(179.741548948246,3.15237321066194,127.029214765655));
#203235=CARTESIAN_POINT('Ctrl Pts',(179.733792645505,3.04702563625045,126.94124601308));
#203236=CARTESIAN_POINT('Ctrl Pts',(179.726036342763,2.93804885563987,126.857736854617));
#203237=CARTESIAN_POINT('Ctrl Pts',(179.718280040021,2.82586602993138,126.77898308951));
#203238=CARTESIAN_POINT('Ctrl Pts',(179.710519597507,2.71362332887097,126.700187291147));
#203239=CARTESIAN_POINT('Ctrl Pts',(179.702759154993,2.59817150202462,126.626152154456));
#203240=CARTESIAN_POINT('Ctrl Pts',(179.694998712478,2.4799605818237,126.557128745499));
#203241=CARTESIAN_POINT('Ctrl Pts',(179.687225812213,2.36155989895946,126.487994534039));
#203242=CARTESIAN_POINT('Ctrl Pts',(179.679452911947,2.2403916176828,126.423888310267));
#203243=CARTESIAN_POINT('Ctrl Pts',(179.671680011682,2.11692893384896,126.365014387373));
#203244=CARTESIAN_POINT('Ctrl Pts',(179.66418967592,1.99795442955653,126.30828067987));
#203245=CARTESIAN_POINT('Ctrl Pts',(179.656699340158,1.87684972432121,126.256405584449));
#203246=CARTESIAN_POINT('Ctrl Pts',(179.649209004396,1.75405185342764,126.209528176879));
#203247=CARTESIAN_POINT('Ctrl Pts',(179.641434670277,1.6265980639352,126.160873398153));
#203248=CARTESIAN_POINT('Ctrl Pts',(179.633660336158,1.49691644622467,126.117448639312));
#203249=CARTESIAN_POINT('Ctrl Pts',(179.625886002039,1.36547540397288,126.079462736802));
#203250=CARTESIAN_POINT('Ctrl Pts',(179.618121249092,1.23419635105852,126.041523648523));
#203251=CARTESIAN_POINT('Ctrl Pts',(179.610356496145,1.10116255992973,126.009010187295));
#203252=CARTESIAN_POINT('Ctrl Pts',(179.602591743197,0.966862147156906,
125.982083079836));
#203253=CARTESIAN_POINT('Ctrl Pts',(179.594834702312,0.832695123447448,
125.955182716759));
#203254=CARTESIAN_POINT('Ctrl Pts',(179.587077661427,0.697264362478954,
125.933857742155));
#203255=CARTESIAN_POINT('Ctrl Pts',(179.579320620542,0.561072529599974,
125.918218920989));
#203256=CARTESIAN_POINT('Ctrl Pts',(179.571569429302,0.424983400041494,
125.90259189318));
#203257=CARTESIAN_POINT('Ctrl Pts',(179.563818238062,0.288134727787094,
125.89264252828));
#203258=CARTESIAN_POINT('Ctrl Pts',(179.556067046822,0.151038393166892,
125.888430342807));
#203259=CARTESIAN_POINT('Ctrl Pts',(179.548319150045,0.0140003281460682,
125.884219947625));
#203260=CARTESIAN_POINT('Ctrl Pts',(179.540571253268,-0.123284799917584,
125.885741893951));
#203261=CARTESIAN_POINT('Ctrl Pts',(179.532823356491,-0.260301197590463,
125.893003743032));
#203262=CARTESIAN_POINT('Ctrl Pts',(179.525077080407,-0.39728893438668,
125.90026407309));
#203263=CARTESIAN_POINT('Ctrl Pts',(179.517330804322,-0.534007662432173,
125.913261897038));
#203264=CARTESIAN_POINT('Ctrl Pts',(179.509584528238,-0.669943198128833,
125.931952673461));
#203265=CARTESIAN_POINT('Ctrl Pts',(179.501838194973,-0.805879737270736,
125.950643587855));
#203266=CARTESIAN_POINT('Ctrl Pts',(179.494091861708,-0.941032685206453,
125.975027485324));
#203267=CARTESIAN_POINT('Ctrl Pts',(179.486345528442,-1.07489497441483,
126.005008176197));
#203268=CARTESIAN_POINT('Ctrl Pts',(179.478597460439,-1.20878724115488,
126.034995581037));
#203269=CARTESIAN_POINT('Ctrl Pts',(179.470849392436,-1.34138789258256,
126.070582187898));
#203270=CARTESIAN_POINT('Ctrl Pts',(179.463101324433,-1.47220240153905,
126.111621209565));
#203271=CARTESIAN_POINT('Ctrl Pts',(179.455345021691,-1.60315594171228,
126.152703847993));
#203272=CARTESIAN_POINT('Ctrl Pts',(179.44758871895,-1.73231917365516,126.199250359929));
#203273=CARTESIAN_POINT('Ctrl Pts',(179.439832416208,-1.85921450417547,
126.251064614673));
#203274=CARTESIAN_POINT('Ctrl Pts',(179.432071973694,-1.98617756255448,
126.302906524244));
#203275=CARTESIAN_POINT('Ctrl Pts',(179.424311531179,-2.11086995231502,
126.360021616145));
#203276=CARTESIAN_POINT('Ctrl Pts',(179.416551088665,-2.23283719094561,
126.422166972686));
#203277=CARTESIAN_POINT('Ctrl Pts',(179.4087781884,-2.35500022221536,126.48441209047));
#203278=CARTESIAN_POINT('Ctrl Pts',(179.401005288134,-2.47442901958706,
126.551703417341));
#203279=CARTESIAN_POINT('Ctrl Pts',(179.393232387869,-2.59069591467029,
126.623753276496));
#203280=CARTESIAN_POINT('Ctrl Pts',(179.385742052107,-2.70273621525825,
126.693183941787));
#203281=CARTESIAN_POINT('Ctrl Pts',(179.378251716345,-2.81184025354116,
126.76703300397));
#203282=CARTESIAN_POINT('Ctrl Pts',(179.370761380583,-2.91765479288965,
126.845007946734));
#203283=CARTESIAN_POINT('Ctrl Pts',(179.362824623581,-3.02977583963157,
126.927630167234));
#203284=CARTESIAN_POINT('Ctrl Pts',(179.354887866579,-3.13858421238573,
127.015166053473));
#203285=CARTESIAN_POINT('Ctrl Pts',(179.346951109577,-3.24361582879236,
127.107315930562));
#203286=CARTESIAN_POINT('Ctrl Pts',(179.339259878588,-3.34539825992441,
127.196615122934));
#203287=CARTESIAN_POINT('Ctrl Pts',(179.331568647598,-3.44363378017725,
127.290246806879));
#203288=CARTESIAN_POINT('Ctrl Pts',(179.323877416609,-3.53792844756241,
127.387893822406));
#203289=CARTESIAN_POINT('Ctrl Pts',(179.316193156561,-3.63213765104985,
127.485452335638));
#203290=CARTESIAN_POINT('Ctrl Pts',(179.308508896513,-3.72241282922045,
127.587018658588));
#203291=CARTESIAN_POINT('Ctrl Pts',(179.300824636464,-3.80839397804645,
127.692236203202));
#203292=CARTESIAN_POINT('Ctrl Pts',(179.293145599922,-3.89431667973043,
127.797382224409));
#203293=CARTESIAN_POINT('Ctrl Pts',(179.28546656338,-3.97595090671817,127.906174222729));
#203294=CARTESIAN_POINT('Ctrl Pts',(179.277787526838,-4.05297468425983,
128.018220048383));
#203295=CARTESIAN_POINT('Ctrl Pts',(179.270111970762,-4.12996355134694,
128.130215090099));
#203296=CARTESIAN_POINT('Ctrl Pts',(179.262436414686,-4.20234590173357,
128.245460696354));
#203297=CARTESIAN_POINT('Ctrl Pts',(179.25476085861,-4.26984142786074,128.363533453791));
#203298=CARTESIAN_POINT('Ctrl Pts',(179.247085795211,-4.33733262159974,
128.481598632399));
#203299=CARTESIAN_POINT('Ctrl Pts',(179.239410731811,-4.39993741066976,
128.60249025877));
#203300=CARTESIAN_POINT('Ctrl Pts',(179.231735668412,-4.45742018209201,
128.725758110404));
#203301=CARTESIAN_POINT('Ctrl Pts',(179.224060790413,-4.51490156495416,
128.849022984367));
#203302=CARTESIAN_POINT('Ctrl Pts',(179.216385912414,-4.56726101346593,
128.974663605236));
#203303=CARTESIAN_POINT('Ctrl Pts',(179.208711034414,-4.61431036413111,
129.102208178455));
#203304=CARTESIAN_POINT('Ctrl Pts',(179.201032838487,-4.66138005470733,
129.229807890485));
#203305=CARTESIAN_POINT('Ctrl Pts',(179.19335464256,-4.70313493368093,129.359312821299));
#203306=CARTESIAN_POINT('Ctrl Pts',(179.185676446633,-4.73943621873225,
129.490234523514));
#203307=CARTESIAN_POINT('Ctrl Pts',(179.183877368601,-4.74794197257219,
129.520910786621));
#203308=CARTESIAN_POINT('Ctrl Pts',(179.182078290568,-4.75614853636364,
129.551664776996));
#203309=CARTESIAN_POINT('Ctrl Pts',(179.180279212536,-4.76405452823405,
129.582490119308));
#203310=CARTESIAN_POINT('Ctrl Pts',(180.930009319727,-4.76405452823405,
129.582490119308));
#203311=CARTESIAN_POINT('Ctrl Pts',(180.922246799312,-4.79822091605315,
129.715704346868));
#203312=CARTESIAN_POINT('Ctrl Pts',(180.914484278898,-4.82680923366528,
129.850405798733));
#203313=CARTESIAN_POINT('Ctrl Pts',(180.906721758483,-4.84970257641179,
129.986089279412));
#203314=CARTESIAN_POINT('Ctrl Pts',(180.89895822607,-4.87259890375656,130.121790449105));
#203315=CARTESIAN_POINT('Ctrl Pts',(180.891194693658,-4.88979869697442,
130.258473522519));
#203316=CARTESIAN_POINT('Ctrl Pts',(180.883431161245,-4.9012362819718,130.395623574));
#203317=CARTESIAN_POINT('Ctrl Pts',(180.875667628833,-4.91267386696918,
130.532773625481));
#203318=CARTESIAN_POINT('Ctrl Pts',(180.86790409642,-4.9183492172088,130.670390267495));
#203319=CARTESIAN_POINT('Ctrl Pts',(180.860140564008,-4.91824868670247,
130.8079548142));
#203320=CARTESIAN_POINT('Origin',(213.235140564004,0.,130.804360617566));
#203321=CARTESIAN_POINT('',(182.679902359578,-4.76405452823405,129.582490119308));
#203322=CARTESIAN_POINT('',(182.334764431275,-4.76405452823405,129.582490119308));
#203323=CARTESIAN_POINT('',(213.235140564004,-4.76405452823405,129.582490119308));
#203324=CARTESIAN_POINT('',(182.264859435942,-4.91824838731473,130.808343477848));
#203325=CARTESIAN_POINT('Ctrl Pts',(182.334764431275,-4.76405452823405,
129.582490119308));
#203326=CARTESIAN_POINT('Ctrl Pts',(182.327037589112,-4.79807206386625,
129.71512397445));
#203327=CARTESIAN_POINT('Ctrl Pts',(182.319310746949,-4.82655566072364,
129.849215252561));
#203328=CARTESIAN_POINT('Ctrl Pts',(182.311583904787,-4.84939387740225,
129.984261791623));
#203329=CARTESIAN_POINT('Ctrl Pts',(182.303796493321,-4.87241111868681,
130.120366935819));
#203330=CARTESIAN_POINT('Ctrl Pts',(182.296009081855,-4.88969399094239,
130.257441989725));
#203331=CARTESIAN_POINT('Ctrl Pts',(182.288221670389,-4.90118122870282,
130.394963956721));
#203332=CARTESIAN_POINT('Ctrl Pts',(182.280434258923,-4.91266846646326,
130.532485923717));
#203333=CARTESIAN_POINT('Ctrl Pts',(182.272646847457,-4.91836005162741,
130.670454396298));
#203334=CARTESIAN_POINT('Ctrl Pts',(182.264859435991,-4.91824838731544,
130.808343476974));
#203335=CARTESIAN_POINT('Ctrl Pts',(182.264859435942,-4.91824838731473,
130.808343477848));
#203336=CARTESIAN_POINT('Ctrl Pts',(182.255745689485,-4.91811770455124,
130.969717526973));
#203337=CARTESIAN_POINT('Ctrl Pts',(182.246631943028,-4.91004084791699,
131.130754613443));
#203338=CARTESIAN_POINT('Ctrl Pts',(182.237518196571,-4.89414028983605,
131.290749233699));
#203339=CARTESIAN_POINT('Ctrl Pts',(182.228343751195,-4.87813383165355,
131.451809442121));
#203340=CARTESIAN_POINT('Ctrl Pts',(182.21916930582,-4.85419921674639,131.611813182237));
#203341=CARTESIAN_POINT('Ctrl Pts',(182.209994860445,-4.82251028849471,
131.770061181852));
#203342=CARTESIAN_POINT('Ctrl Pts',(182.200752520834,-4.79058685063821,
131.929480274271));
#203343=CARTESIAN_POINT('Ctrl Pts',(182.191510181223,-4.75079397460461,
132.087117477438));
#203344=CARTESIAN_POINT('Ctrl Pts',(182.182267841612,-4.70335754186608,
132.242279563777));
#203345=CARTESIAN_POINT('Ctrl Pts',(182.179787432699,-4.69062680965446,
132.28392112189));
#203346=CARTESIAN_POINT('Ctrl Pts',(182.177307023785,-4.67734581439877,
132.325384532998));
#203347=CARTESIAN_POINT('Ctrl Pts',(182.174826614871,-4.66351949799474,
132.366656669639));
#203348=CARTESIAN_POINT('Ctrl Pts',(182.167052280752,-4.62018373880961,
132.496015735516));
#203349=CARTESIAN_POINT('Ctrl Pts',(182.159277946633,-4.57139291895546,
132.623775226555));
#203350=CARTESIAN_POINT('Ctrl Pts',(182.151503612514,-4.51728310406877,
132.749440672524));
#203351=CARTESIAN_POINT('Ctrl Pts',(182.143738859567,-4.46323997469291,
132.874951247062));
#203352=CARTESIAN_POINT('Ctrl Pts',(182.13597410662,-4.40389104628627,132.998372555757));
#203353=CARTESIAN_POINT('Ctrl Pts',(182.128209353673,-4.33942206882534,
133.119225445389));
#203354=CARTESIAN_POINT('Ctrl Pts',(182.120452312788,-4.27501712286173,
133.239958302227));
#203355=CARTESIAN_POINT('Ctrl Pts',(182.112695271903,-4.20550243065429,
133.358127473865));
#203356=CARTESIAN_POINT('Ctrl Pts',(182.104938231018,-4.13111157845121,
133.473274289622));
#203357=CARTESIAN_POINT('Ctrl Pts',(182.097187039777,-4.05677682496856,
133.588334272269));
#203358=CARTESIAN_POINT('Ctrl Pts',(182.089435848537,-3.97757344193555,
133.700376108544));
#203359=CARTESIAN_POINT('Ctrl Pts',(182.081684657297,-3.89378045932293,
133.808966547983));
#203360=CARTESIAN_POINT('Ctrl Pts',(182.07393676052,-3.81002309096304,133.917510833588));
#203361=CARTESIAN_POINT('Ctrl Pts',(182.066188863743,-3.72168024116592,
134.022606331103));
#203362=CARTESIAN_POINT('Ctrl Pts',(182.058440966966,-3.62907356334536,
134.123849755118));
#203363=CARTESIAN_POINT('Ctrl Pts',(182.050694690882,-3.53648625684542,
134.225072001192));
#203364=CARTESIAN_POINT('Ctrl Pts',(182.042948414798,-3.43963716006998,
134.322443488187));
#203365=CARTESIAN_POINT('Ctrl Pts',(182.035202138714,-3.33888715704143,
134.415595256169));
#203366=CARTESIAN_POINT('Ctrl Pts',(182.027455805448,-3.23813641029925,
134.508747711776));
#203367=CARTESIAN_POINT('Ctrl Pts',(182.019709472183,-3.1334849869114,134.597680120798));
#203368=CARTESIAN_POINT('Ctrl Pts',(182.011963138918,-3.02532915435104,
134.682061814194));
#203369=CARTESIAN_POINT('Ctrl Pts',(182.004215070915,-2.91714910104202,
134.766462404286));
#203370=CARTESIAN_POINT('Ctrl Pts',(181.996467002912,-2.8054633851131,134.846310010414));
#203371=CARTESIAN_POINT('Ctrl Pts',(181.988718934909,-2.69069940167571,
134.921315777915));
#203372=CARTESIAN_POINT('Ctrl Pts',(181.980962632167,-2.5758134457109,134.996401262438));
#203373=CARTESIAN_POINT('Ctrl Pts',(181.973206329425,-2.45784301461549,
135.066634414486));
#203374=CARTESIAN_POINT('Ctrl Pts',(181.965450026683,-2.33724287264859,
135.13177079188));
#203375=CARTESIAN_POINT('Ctrl Pts',(181.957689584169,-2.21657836275474,
135.196941934519));
#203376=CARTESIAN_POINT('Ctrl Pts',(181.949929141655,-2.09328169658598,
135.257010710924));
#203377=CARTESIAN_POINT('Ctrl Pts',(181.942168699141,-1.96782911067562,
135.311780240108));
#203378=CARTESIAN_POINT('Ctrl Pts',(181.934395798875,-1.8421751371371,135.366637690203));
#203379=CARTESIAN_POINT('Ctrl Pts',(181.92662289861,-1.71435869267866,135.416178752362));
#203380=CARTESIAN_POINT('Ctrl Pts',(181.918849998344,-1.58487356800099,
135.460255680382));
#203381=CARTESIAN_POINT('Ctrl Pts',(181.911359662582,-1.46009555375806,
135.502730301045));
#203382=CARTESIAN_POINT('Ctrl Pts',(181.90386932682,-1.33376836978196,135.540131073015));
#203383=CARTESIAN_POINT('Ctrl Pts',(181.896378991058,-1.20634228632941,
135.572370826313));
#203384=CARTESIAN_POINT('Ctrl Pts',(181.888604656939,-1.07408480419308,
135.605832959655));
#203385=CARTESIAN_POINT('Ctrl Pts',(181.88083032282,-0.940224496132468,
135.63384098669));
#203386=CARTESIAN_POINT('Ctrl Pts',(181.873055988701,-0.805250920756176,
135.656242110051));
#203387=CARTESIAN_POINT('Ctrl Pts',(181.865291235754,-0.670443688248645,
135.67861562603));
#203388=CARTESIAN_POINT('Ctrl Pts',(181.857526482807,-0.534526300288229,
135.695395923796));
#203389=CARTESIAN_POINT('Ctrl Pts',(181.849761729859,-0.398002284449767,
135.706480286043));
#203390=CARTESIAN_POINT('Ctrl Pts',(181.842004688974,-0.261613866188487,
135.717553639146));
#203391=CARTESIAN_POINT('Ctrl Pts',(181.834247648089,-0.124620406235299,
135.722942283547));
#203392=CARTESIAN_POINT('Ctrl Pts',(181.826490607204,0.0124659437015487,
135.722594819264));
#203393=CARTESIAN_POINT('Ctrl Pts',(181.818739415964,0.149448915755369,
135.722247617006));
#203394=CARTESIAN_POINT('Ctrl Pts',(181.810988224724,0.286524248982427,
135.716172916984));
#203395=CARTESIAN_POINT('Ctrl Pts',(181.803237033484,0.423176614983207,
135.704371292558));
#203396=CARTESIAN_POINT('Ctrl Pts',(181.795489136707,0.559770900083301,
135.692574684136));
#203397=CARTESIAN_POINT('Ctrl Pts',(181.78774123993,0.695942186810799,135.675056026109));
#203398=CARTESIAN_POINT('Ctrl Pts',(181.779993343153,0.831177318203662,
135.651867948989));
#203399=CARTESIAN_POINT('Ctrl Pts',(181.772247067069,0.966384161322348,
135.628684722316));
#203400=CARTESIAN_POINT('Ctrl Pts',(181.764500790985,1.10065485351256,135.599834501441));
#203401=CARTESIAN_POINT('Ctrl Pts',(181.756754514901,1.2334839117036,135.565421476457));
#203402=CARTESIAN_POINT('Ctrl Pts',(181.749008181635,1.36631395040857,135.531008197445));
#203403=CARTESIAN_POINT('Ctrl Pts',(181.74126184837,1.49770195540958,135.491032130437));
#203404=CARTESIAN_POINT('Ctrl Pts',(181.733515515104,1.62715553322994,135.44564793179));
#203405=CARTESIAN_POINT('Ctrl Pts',(181.725767447101,1.75663810128136,135.400253569667));
#203406=CARTESIAN_POINT('Ctrl Pts',(181.718019379098,1.88418501125313,135.34944879525));
#203407=CARTESIAN_POINT('Ctrl Pts',(181.710271311096,2.00932222403949,135.293437055151));
#203408=CARTESIAN_POINT('Ctrl Pts',(181.702515008354,2.13459243414487,135.237365785108));
#203409=CARTESIAN_POINT('Ctrl Pts',(181.694758705612,2.2574474736639,135.176076654553));
#203410=CARTESIAN_POINT('Ctrl Pts',(181.68700240287,2.37743587527888,135.109820142569));
#203411=CARTESIAN_POINT('Ctrl Pts',(181.679241960356,2.49748831831668,135.043528267489));
#203412=CARTESIAN_POINT('Ctrl Pts',(181.671481517842,2.61467074089446,134.972263931206));
#203413=CARTESIAN_POINT('Ctrl Pts',(181.663721075327,2.72856008398556,134.896321386022));
#203414=CARTESIAN_POINT('Ctrl Pts',(181.655948175062,2.84263225236077,134.820256931122));
#203415=CARTESIAN_POINT('Ctrl Pts',(181.648175274797,2.9534004613508,134.739499490654));
#203416=CARTESIAN_POINT('Ctrl Pts',(181.640402374531,3.06047350195551,134.654384644287));
#203417=CARTESIAN_POINT('Ctrl Pts',(181.632912038769,3.16365416783352,134.572363936976));
#203418=CARTESIAN_POINT('Ctrl Pts',(181.625421703007,3.26340342518855,134.486297330141));
#203419=CARTESIAN_POINT('Ctrl Pts',(181.617931367245,3.35940455337579,134.396516531395));
#203420=CARTESIAN_POINT('Ctrl Pts',(181.610157033126,3.45904559351708,134.303331666377));
#203421=CARTESIAN_POINT('Ctrl Pts',(181.602382699007,3.5549643061159,134.205850220831));
#203422=CARTESIAN_POINT('Ctrl Pts',(181.594608364888,3.64676752003656,134.104401483572));
#203423=CARTESIAN_POINT('Ctrl Pts',(181.586843611941,3.73845759470076,134.003077772814));
#203424=CARTESIAN_POINT('Ctrl Pts',(181.579078858994,3.82604200261285,133.897796785766));
#203425=CARTESIAN_POINT('Ctrl Pts',(181.571314106046,3.90916215584225,133.788926633226));
#203426=CARTESIAN_POINT('Ctrl Pts',(181.563557065161,3.99219975296364,133.680164612056));
#203427=CARTESIAN_POINT('Ctrl Pts',(181.555800024276,4.07078168346808,133.567820828264));
#203428=CARTESIAN_POINT('Ctrl Pts',(181.548042983391,4.14458787258715,133.452298386643));
#203429=CARTESIAN_POINT('Ctrl Pts',(181.540291792151,4.21833840388486,133.336863061394));
#203430=CARTESIAN_POINT('Ctrl Pts',(181.532540600911,4.28732015257257,133.21825417763));
#203431=CARTESIAN_POINT('Ctrl Pts',(181.524789409671,4.35125505344596,133.096905605644));
#203432=CARTESIAN_POINT('Ctrl Pts',(181.517041512894,4.41516278028099,132.975608610038));
#203433=CARTESIAN_POINT('Ctrl Pts',(181.509293616117,4.47402774377339,132.851574587362));
#203434=CARTESIAN_POINT('Ctrl Pts',(181.50154571934,4.52761684959189,132.72526371918));
#203435=CARTESIAN_POINT('Ctrl Pts',(181.493799443256,4.5811947457247,132.598979272509));
#203436=CARTESIAN_POINT('Ctrl Pts',(181.486053167172,4.62949882669481,132.470419287337));
#203437=CARTESIAN_POINT('Ctrl Pts',(181.478306891088,4.67234352463098,132.340065358178));
#203438=CARTESIAN_POINT('Ctrl Pts',(181.470560557822,4.71518853883696,132.209710466776));
#203439=CARTESIAN_POINT('Ctrl Pts',(181.462814224557,4.75257396751604,132.07756197638));
#203440=CARTESIAN_POINT('Ctrl Pts',(181.455067891292,4.78436377673831,131.944117747105));
#203441=CARTESIAN_POINT('Ctrl Pts',(181.447319823289,4.81616070506794,131.810643633919));
#203442=CARTESIAN_POINT('Ctrl Pts',(181.439571755286,4.84235942983139,131.675873584696));
#203443=CARTESIAN_POINT('Ctrl Pts',(181.431823687283,4.86287488670871,131.540316389823));
#203444=CARTESIAN_POINT('Ctrl Pts',(181.424067384541,4.88341214765773,131.404615123149));
#203445=CARTESIAN_POINT('Ctrl Pts',(181.416311081799,4.89825401608467,131.268125426831));
#203446=CARTESIAN_POINT('Ctrl Pts',(181.408554779057,4.90736719802281,131.131362523172));
#203447=CARTESIAN_POINT('Ctrl Pts',(181.400794336543,4.91648524394055,130.994526625032));
#203448=CARTESIAN_POINT('Ctrl Pts',(181.393033894029,4.91986850125779,130.85741761965));
#203449=CARTESIAN_POINT('Ctrl Pts',(181.385273451515,4.91753585903247,130.720550489122));
#203450=CARTESIAN_POINT('Ctrl Pts',(181.377500551249,4.91519947224276,130.583463647326));
#203451=CARTESIAN_POINT('Ctrl Pts',(181.369727650984,4.90712887303039,130.4466198468));
#203452=CARTESIAN_POINT('Ctrl Pts',(181.361954750718,4.89339493605524,130.310529611767));
#203453=CARTESIAN_POINT('Ctrl Pts',(181.354464414956,4.88016026228275,130.179386599566));
#203454=CARTESIAN_POINT('Ctrl Pts',(181.346974079194,4.86166689853009,130.048943621018));
#203455=CARTESIAN_POINT('Ctrl Pts',(181.339483743432,4.83802272456425,129.91964643824));
#203456=CARTESIAN_POINT('Ctrl Pts',(181.331709409313,4.81348207455615,129.785446913479));
#203457=CARTESIAN_POINT('Ctrl Pts',(181.323935075194,4.78331458070452,129.652056681576));
#203458=CARTESIAN_POINT('Ctrl Pts',(181.316160741075,4.74758476441283,129.519984517191));
#203459=CARTESIAN_POINT('Ctrl Pts',(181.308395988128,4.71189898192648,129.388075119944));
#203460=CARTESIAN_POINT('Ctrl Pts',(181.300631235181,4.67066461765525,129.257480931918));
#203461=CARTESIAN_POINT('Ctrl Pts',(181.292866482234,4.62399754810301,129.128702616172));
#203462=CARTESIAN_POINT('Ctrl Pts',(181.285109441349,4.57737682894217,129.000052204864));
#203463=CARTESIAN_POINT('Ctrl Pts',(181.277352400464,4.52533427480508,128.873214441886));
#203464=CARTESIAN_POINT('Ctrl Pts',(181.269595359579,4.46803602093881,128.748676503191));
#203465=CARTESIAN_POINT('Ctrl Pts',(181.261844168339,4.41078097613147,128.624232479525));
#203466=CARTESIAN_POINT('Ctrl Pts',(181.254092977099,4.3482782831815,128.502085181832));
#203467=CARTESIAN_POINT('Ctrl Pts',(181.246341785858,4.28074266841829,128.382703071734));
#203468=CARTESIAN_POINT('Ctrl Pts',(181.238593889081,4.2132357580929,128.263371702218));
#203469=CARTESIAN_POINT('Ctrl Pts',(181.230845992304,4.14070037261404,128.146803522334));
#203470=CARTESIAN_POINT('Ctrl Pts',(181.223098095527,4.06339768258434,128.03344338032));
#203471=CARTESIAN_POINT('Ctrl Pts',(181.215351819443,3.98611116261093,127.920106950803));
#203472=CARTESIAN_POINT('Ctrl Pts',(181.207605543359,3.90405954173491,127.809977547203));
#203473=CARTESIAN_POINT('Ctrl Pts',(181.199859267275,3.81754769509268,127.703471606622));
#203474=CARTESIAN_POINT('Ctrl Pts',(181.19211293401,3.7310352098397,127.596964879839));
#203475=CARTESIAN_POINT('Ctrl Pts',(181.184366600744,3.64006267962051,127.494081972915));
#203476=CARTESIAN_POINT('Ctrl Pts',(181.176620267479,3.54497543858795,127.395206440602));
#203477=CARTESIAN_POINT('Ctrl Pts',(181.168872199476,3.44986690342704,127.2963087658));
#203478=CARTESIAN_POINT('Ctrl Pts',(181.161124131473,3.35064209480331,127.201420533123));
#203479=CARTESIAN_POINT('Ctrl Pts',(181.15337606347,3.24768309313699,127.110888323227));
#203480=CARTESIAN_POINT('Ctrl Pts',(181.145619760728,3.14461466541844,127.02025989462));
#203481=CARTESIAN_POINT('Ctrl Pts',(181.137863457986,3.03780441073446,126.933996995563));
#203482=CARTESIAN_POINT('Ctrl Pts',(181.130107155245,2.92766780399824,126.852406127452));
#203483=CARTESIAN_POINT('Ctrl Pts',(181.12234671273,2.81747241403878,126.770771711838));
#203484=CARTESIAN_POINT('Ctrl Pts',(181.114586270216,2.7039474579022,126.693814515155));
#203485=CARTESIAN_POINT('Ctrl Pts',(181.106825827702,2.58753641460957,126.621797005908));
#203486=CARTESIAN_POINT('Ctrl Pts',(181.099052927437,2.4709384979758,126.54966388776));
#203487=CARTESIAN_POINT('Ctrl Pts',(181.091280027171,2.35144557696644,126.48248649467));
#203488=CARTESIAN_POINT('Ctrl Pts',(181.083507126906,2.22952547955141,126.420481148588));
#203489=CARTESIAN_POINT('Ctrl Pts',(181.076016791144,2.11203748477606,126.360729853018));
#203490=CARTESIAN_POINT('Ctrl Pts',(181.068526455382,1.99229599775392,126.305781227551));
#203491=CARTESIAN_POINT('Ctrl Pts',(181.06103611962,1.87073436242814,126.255785455196));
#203492=CARTESIAN_POINT('Ctrl Pts',(181.053261785501,1.74456368075061,126.203894077936));
#203493=CARTESIAN_POINT('Ctrl Pts',(181.045487451382,1.61603243353411,126.15717416632));
#203494=CARTESIAN_POINT('Ctrl Pts',(181.037713117262,1.48560354270351,126.115846441795));
#203495=CARTESIAN_POINT('Ctrl Pts',(181.029948364315,1.35533539382416,126.074569649997));
#203496=CARTESIAN_POINT('Ctrl Pts',(181.022183611368,1.22317462372418,126.038671939907));
#203497=CARTESIAN_POINT('Ctrl Pts',(181.014418858421,1.08960508849571,126.008326441955));
#203498=CARTESIAN_POINT('Ctrl Pts',(181.006661817536,0.956168216412676,
125.97801108358));
#203499=CARTESIAN_POINT('Ctrl Pts',(180.998904776651,0.821325742465903,
125.953237049223));
#203500=CARTESIAN_POINT('Ctrl Pts',(180.991147735766,0.685577341742052,
125.934127895099));
#203501=CARTESIAN_POINT('Ctrl Pts',(180.983396544526,0.549931309943087,
125.915033151336));
#203502=CARTESIAN_POINT('Ctrl Pts',(180.975645353286,0.413381096750075,
125.901594839067));
#203503=CARTESIAN_POINT('Ctrl Pts',(180.967894162046,0.276436897019386,
125.893885517897));
#203504=CARTESIAN_POINT('Ctrl Pts',(180.960146265269,0.139550902226688,
125.886179473395));
#203505=CARTESIAN_POINT('Ctrl Pts',(180.952398368492,0.00227164348105247,
125.884197598944));
#203506=CARTESIAN_POINT('Ctrl Pts',(180.944650471714,-0.134885446705906,
125.887960615657));
#203507=CARTESIAN_POINT('Ctrl Pts',(180.93690419563,-0.272013846586339,
125.891722845229));
#203508=CARTESIAN_POINT('Ctrl Pts',(180.929157919546,-0.409019738167906,
125.901227564989));
#203509=CARTESIAN_POINT('Ctrl Pts',(180.921411643462,-0.545387968662936,
125.916443369275));
#203510=CARTESIAN_POINT('Ctrl Pts',(180.913665310197,-0.681757205797242,
125.931659285882));
#203511=CARTESIAN_POINT('Ctrl Pts',(180.905918976931,-0.817488383898427,
125.952586327784));
#203512=CARTESIAN_POINT('Ctrl Pts',(180.898172643666,-0.95207214594684,
125.979141276291));
#203513=CARTESIAN_POINT('Ctrl Pts',(180.890424575663,-1.08668604709579,
126.005702171595));
#203514=CARTESIAN_POINT('Ctrl Pts',(180.88267650766,-1.22015163738299,126.037893405747));
#203515=CARTESIAN_POINT('Ctrl Pts',(180.874928439657,-1.35197080488857,
126.075580858978));
#203516=CARTESIAN_POINT('Ctrl Pts',(180.867172136915,-1.48393007137391,
126.113308366883));
#203517=CARTESIAN_POINT('Ctrl Pts',(180.859415834173,-1.61423904308519,
126.156543655144));
#203518=CARTESIAN_POINT('Ctrl Pts',(180.851659531431,-1.74241527737747,
126.20510284444));
#203519=CARTESIAN_POINT('Ctrl Pts',(180.843899088917,-1.87065992318532,
126.253687951238));
#203520=CARTESIAN_POINT('Ctrl Pts',(180.836138646403,-1.99676920408849,
126.307602467438));
#203521=CARTESIAN_POINT('Ctrl Pts',(180.828378203889,-2.12028258665798,
126.366615152218));
#203522=CARTESIAN_POINT('Ctrl Pts',(180.820605303623,-2.24399424387421,
126.425722569399));
#203523=CARTESIAN_POINT('Ctrl Pts',(180.812832403358,-2.3651013298266,126.489944326195));
#203524=CARTESIAN_POINT('Ctrl Pts',(180.805059503092,-2.48316897428491,
126.559003752985));
#203525=CARTESIAN_POINT('Ctrl Pts',(180.79756916733,-2.59694456247199,126.62555269566));
#203526=CARTESIAN_POINT('Ctrl Pts',(180.790078831568,-2.707897595887,126.696593525687));
#203527=CARTESIAN_POINT('Ctrl Pts',(180.782588495806,-2.81566748832438,
126.771842836118));
#203528=CARTESIAN_POINT('Ctrl Pts',(180.774860431703,-2.92685778253992,
126.849480409815));
#203529=CARTESIAN_POINT('Ctrl Pts',(180.7671323676,-3.03502137085671,126.931850825884));
#203530=CARTESIAN_POINT('Ctrl Pts',(180.759404303497,-3.13972510257354,
127.018689033452));
#203531=CARTESIAN_POINT('Ctrl Pts',(180.751688447729,-3.24426342957341,
127.105390059193));
#203532=CARTESIAN_POINT('Ctrl Pts',(180.743972591961,-3.3453524815515,127.196544571404));
#203533=CARTESIAN_POINT('Ctrl Pts',(180.736256736193,-3.44258800822052,
127.291844301852));
#203534=CARTESIAN_POINT('Ctrl Pts',(180.728547930298,-3.53973469210992,
127.387056958232));
#203535=CARTESIAN_POINT('Ctrl Pts',(180.720839124402,-3.63303457198762,
127.486407025166));
#203536=CARTESIAN_POINT('Ctrl Pts',(180.713130318507,-3.72211626851405,
127.589545918993));
#203537=CARTESIAN_POINT('Ctrl Pts',(180.705426833656,-3.81113647592418,
127.692613620647));
#203538=CARTESIAN_POINT('Ctrl Pts',(180.697723348805,-3.89594403403888,
127.799464648121));
#203539=CARTESIAN_POINT('Ctrl Pts',(180.690019863954,-3.97620460244335,
127.909713830476));
#203540=CARTESIAN_POINT('Ctrl Pts',(180.682319975564,-4.05642770026874,
128.01991154172));
#203541=CARTESIAN_POINT('Ctrl Pts',(180.674620087175,-4.13210780008793,
128.133503931074));
#203542=CARTESIAN_POINT('Ctrl Pts',(180.666920198785,-4.20295133298381,
128.250073406803));
#203543=CARTESIAN_POINT('Ctrl Pts',(180.659220735343,-4.27379095611665,
128.366636449212));
#203544=CARTESIAN_POINT('Ctrl Pts',(180.6515212719,-4.33979432957215,128.486175917609));
#203545=CARTESIAN_POINT('Ctrl Pts',(180.643821808457,-4.40071176989382,
128.608246098508));
#203546=CARTESIAN_POINT('Ctrl Pts',(180.636122680545,-4.46162655553023,
128.730310959782));
#203547=CARTESIAN_POINT('Ctrl Pts',(180.628423552633,-4.51745567719539,
128.854905956993));
#203548=CARTESIAN_POINT('Ctrl Pts',(180.620724424721,-4.56799625155725,
128.981562409245));
#203549=CARTESIAN_POINT('Ctrl Pts',(180.61302142386,-4.61856224971331,129.108282574417));
#203550=CARTESIAN_POINT('Ctrl Pts',(180.605318422999,-4.66383424513525,
129.237065895624));
#203551=CARTESIAN_POINT('Ctrl Pts',(180.597615422138,-4.70365818002023,
129.367425410944));
#203552=CARTESIAN_POINT('Ctrl Pts',(180.593405538846,-4.72542295989178,
129.438670157685));
#203553=CARTESIAN_POINT('Ctrl Pts',(180.589195655555,-4.74556133082426,
129.510385423281));
#203554=CARTESIAN_POINT('Ctrl Pts',(180.584985772263,-4.76405452823404,
129.582490119308));
#203555=CARTESIAN_POINT('',(182.610140564063,-4.91824890646276,130.801080895348));
#203556=CARTESIAN_POINT('Ctrl Pts',(182.610140564008,-4.91824890646341,
130.80108089632));
#203557=CARTESIAN_POINT('Ctrl Pts',(182.602350736543,-4.91834099197833,
130.939171742779));
#203558=CARTESIAN_POINT('Ctrl Pts',(182.594560909078,-4.91261293631802,
131.077296116385));
#203559=CARTESIAN_POINT('Ctrl Pts',(182.586771081613,-4.90108295938559,
131.214932033668));
#203560=CARTESIAN_POINT('Ctrl Pts',(182.578981013679,-4.88955262652708,
131.352572199721));
#203561=CARTESIAN_POINT('Ctrl Pts',(182.571190945745,-4.87222004712722,
131.48972349604));
#203562=CARTESIAN_POINT('Ctrl Pts',(182.563400877811,-4.84915540080159,
131.625868354217));
#203563=CARTESIAN_POINT('Ctrl Pts',(182.555608953444,-4.82608525799307,
131.762045656762));
#203564=CARTESIAN_POINT('Ctrl Pts',(182.547817029077,-4.79728039275426,
131.897215664416));
#203565=CARTESIAN_POINT('Ctrl Pts',(182.54002510471,-4.76286219548405,132.030870613175));
#203566=CARTESIAN_POINT('Ctrl Pts',(182.532229707094,-4.72842865631017,
132.164585138597));
#203567=CARTESIAN_POINT('Ctrl Pts',(182.524434309478,-4.68837689938111,
132.296782888428));
#203568=CARTESIAN_POINT('Ctrl Pts',(182.516638911862,-4.64287820456094,
132.42697118086));
#203569=CARTESIAN_POINT('Ctrl Pts',(182.508833566481,-4.59732144851264,
132.557325607555));
#203570=CARTESIAN_POINT('Ctrl Pts',(182.501028221099,-4.54630400030386,
132.685665092519));
#203571=CARTESIAN_POINT('Ctrl Pts',(182.493222875718,-4.49004557517999,
132.811516265568));
#203572=CARTESIAN_POINT('Ctrl Pts',(182.48541197276,-4.43374709282834,132.937457047402));
#203573=CARTESIAN_POINT('Ctrl Pts',(182.477601069802,-4.37220036926214,
133.060905643736));
#203574=CARTESIAN_POINT('Ctrl Pts',(182.469790166844,-4.30567070775944,
133.181414007552));
#203575=CARTESIAN_POINT('Ctrl Pts',(182.461966709995,-4.23903411801708,
133.302116055611));
#203576=CARTESIAN_POINT('Ctrl Pts',(182.454143253146,-4.16739879386563,
133.419868104856));
#203577=CARTESIAN_POINT('Ctrl Pts',(182.446319796298,-4.09107330250262,
133.534251145783));
#203578=CARTESIAN_POINT('Ctrl Pts',(182.442108278373,-4.04998581634815,
133.595825745913));
#203579=CARTESIAN_POINT('Ctrl Pts',(182.437896760449,-4.00753987680767,
133.656424612155));
#203580=CARTESIAN_POINT('Ctrl Pts',(182.433685242525,-3.96378825988816,
133.715986571097));
#203581=CARTESIAN_POINT('Ctrl Pts',(182.425910908406,-3.88302410446949,
133.825936137482));
#203582=CARTESIAN_POINT('Ctrl Pts',(182.418136574287,-3.7975538023016,133.932696893848));
#203583=CARTESIAN_POINT('Ctrl Pts',(182.410362240168,-3.70765790045001,
134.035839529106));
#203584=CARTESIAN_POINT('Ctrl Pts',(182.402597487221,-3.61787278726326,
134.138855050285));
#203585=CARTESIAN_POINT('Ctrl Pts',(182.394832734273,-3.52367318095091,
134.238261030556));
#203586=CARTESIAN_POINT('Ctrl Pts',(182.387067981326,-3.42538226341174,
134.333657914763));
#203587=CARTESIAN_POINT('Ctrl Pts',(182.379310940441,-3.32718896979766,
134.42896004944));
#203588=CARTESIAN_POINT('Ctrl Pts',(182.371553899556,-3.22491273033872,
134.520260741664));
#203589=CARTESIAN_POINT('Ctrl Pts',(182.363796858671,-3.11891602473428,
134.607194546777));
#203590=CARTESIAN_POINT('Ctrl Pts',(182.356045667431,-3.01299925206974,
134.694062794431));
#203591=CARTESIAN_POINT('Ctrl Pts',(182.348294476191,-2.90336789877549,
134.77657046277));
#203592=CARTESIAN_POINT('Ctrl Pts',(182.340543284951,-2.79041995640996,
134.854390188985));
#203593=CARTESIAN_POINT('Ctrl Pts',(182.332795388174,-2.67752001993321,
134.932176839741));
#203594=CARTESIAN_POINT('Ctrl Pts',(182.325047491397,-2.56130661932331,
135.005279289951));
#203595=CARTESIAN_POINT('Ctrl Pts',(182.31729959462,-2.44220918470204,135.073411725325));
#203596=CARTESIAN_POINT('Ctrl Pts',(182.309553318536,-2.32313666269663,
135.141529908862));
#203597=CARTESIAN_POINT('Ctrl Pts',(182.301807042451,-2.20118164577595,
135.204679951408));
#203598=CARTESIAN_POINT('Ctrl Pts',(182.294060766367,-2.07680044042566,
135.262620703423));
#203599=CARTESIAN_POINT('Ctrl Pts',(182.286314433102,-1.95241831692144,
135.320561883144));
#203600=CARTESIAN_POINT('Ctrl Pts',(182.278568099837,-1.82561032364971,
135.37329353051));
#203601=CARTESIAN_POINT('Ctrl Pts',(182.270821766571,-1.6968547692407,135.420621762108));
#203602=CARTESIAN_POINT('Ctrl Pts',(182.263073698568,-1.56807038091839,
135.467960592535));
#203603=CARTESIAN_POINT('Ctrl Pts',(182.255325630565,-1.43733793047416,
135.509893464457));
#203604=CARTESIAN_POINT('Ctrl Pts',(182.247577562562,-1.30515260026303,
135.546275816357));
#203605=CARTESIAN_POINT('Ctrl Pts',(182.239821259821,-1.17282678190962,
135.582696835854));
#203606=CARTESIAN_POINT('Ctrl Pts',(182.232064957079,-1.03904537675643,
135.613555447207));
#203607=CARTESIAN_POINT('Ctrl Pts',(182.224308654337,-0.904316068585796,
135.638757737228));
#203608=CARTESIAN_POINT('Ctrl Pts',(182.216548211823,-0.769514851326632,
135.663973478471));
#203609=CARTESIAN_POINT('Ctrl Pts',(182.208787769308,-0.633765109735002,
135.683526827158));
#203610=CARTESIAN_POINT('Ctrl Pts',(182.201027326794,-0.497580452340472,
135.69737571625));
#203611=CARTESIAN_POINT('Ctrl Pts',(182.193254426529,-0.361177179244034,
135.711246836808));
#203612=CARTESIAN_POINT('Ctrl Pts',(182.185481526263,-0.224337985686155,
135.719395175306));
#203613=CARTESIAN_POINT('Ctrl Pts',(182.177708625998,-0.0875781934747493,
135.721830812954));
#203614=CARTESIAN_POINT('Ctrl Pts',(182.170218290236,0.0442100358122264,
135.724177909039));
#203615=CARTESIAN_POINT('Ctrl Pts',(182.162727954474,0.175924228464083,
135.72122044237));
#203616=CARTESIAN_POINT('Ctrl Pts',(182.155237618712,0.307109000857396,
135.713012889228));
#203617=CARTESIAN_POINT('Ctrl Pts',(182.147463284593,0.443267683768998,
135.704494144214));
#203618=CARTESIAN_POINT('Ctrl Pts',(182.139688950474,0.579287317770908,
135.690292354947));
#203619=CARTESIAN_POINT('Ctrl Pts',(182.131914616355,0.714655068745021,
135.670411500491));
#203620=CARTESIAN_POINT('Ctrl Pts',(182.124149863408,0.849855991064199,
135.650555147412));
#203621=CARTESIAN_POINT('Ctrl Pts',(182.116385110461,0.984406245755034,
135.625033711212));
#203622=CARTESIAN_POINT('Ctrl Pts',(182.108620357513,1.11779498803749,135.593903124656));
#203623=CARTESIAN_POINT('Ctrl Pts',(182.100863316628,1.25105124674114,135.562803457436));
#203624=CARTESIAN_POINT('Ctrl Pts',(182.093106275743,1.38314791054298,135.526105814856));
#203625=CARTESIAN_POINT('Ctrl Pts',(182.085349234858,1.5135815913709,135.483917629588));
#203626=CARTESIAN_POINT('Ctrl Pts',(182.077598043618,1.64391691114509,135.441761258759));
#203627=CARTESIAN_POINT('Ctrl Pts',(182.069846852378,1.77259137360677,135.39412270641));
#203628=CARTESIAN_POINT('Ctrl Pts',(182.062095661138,1.8991144349961,135.341159866518));
#203629=CARTESIAN_POINT('Ctrl Pts',(182.054347764361,2.02558372070912,135.288219537246));
#203630=CARTESIAN_POINT('Ctrl Pts',(182.046599867584,2.14990306413975,135.229959571943));
#203631=CARTESIAN_POINT('Ctrl Pts',(182.038851970807,2.27159988415978,135.166586772729));
#203632=CARTESIAN_POINT('Ctrl Pts',(182.031105694723,2.39327124782866,135.103227229737));
#203633=CARTESIAN_POINT('Ctrl Pts',(182.023359418639,2.51232083268777,135.034757160578));
#203634=CARTESIAN_POINT('Ctrl Pts',(182.015613142554,2.62829910799688,134.961430121604));
#203635=CARTESIAN_POINT('Ctrl Pts',(182.007866809289,2.74427823943102,134.888102541346));
#203636=CARTESIAN_POINT('Ctrl Pts',(182.000120476024,2.85718568561855,134.809918128662));
#203637=CARTESIAN_POINT('Ctrl Pts',(181.992374142758,2.96659978945404,134.727174499426));
#203638=CARTESIAN_POINT('Ctrl Pts',(181.984626074756,3.07603839581934,134.644412340328));
#203639=CARTESIAN_POINT('Ctrl Pts',(181.976878006753,3.18198179135113,134.557089168775));
#203640=CARTESIAN_POINT('Ctrl Pts',(181.96912993875,3.28404069419147,134.465543456676));
#203641=CARTESIAN_POINT('Ctrl Pts',(181.961373636008,3.3862080664486,134.373900448704));
#203642=CARTESIAN_POINT('Ctrl Pts',(181.953617333266,3.48448240741909,134.278026196862));
#203643=CARTESIAN_POINT('Ctrl Pts',(181.945861030524,3.57851028979258,134.178297067523));
#203644=CARTESIAN_POINT('Ctrl Pts',(181.93810058801,3.67258835767799,134.078514709744));
#203645=CARTESIAN_POINT('Ctrl Pts',(181.930340145496,3.76241519491009,133.974873670094));
#203646=CARTESIAN_POINT('Ctrl Pts',(181.922579702982,3.84767779134117,133.86778332371));
#203647=CARTESIAN_POINT('Ctrl Pts',(181.914806802716,3.93307725886131,133.760521066396));
#203648=CARTESIAN_POINT('Ctrl Pts',(181.907033902451,4.01389761341318,133.64979875336));
#203649=CARTESIAN_POINT('Ctrl Pts',(181.899261002185,4.08986879258137,133.536055388577));
#203650=CARTESIAN_POINT('Ctrl Pts',(181.891770666423,4.16307822802756,133.426446881605));
#203651=CARTESIAN_POINT('Ctrl Pts',(181.884280330661,4.23178476598698,133.314033418012));
#203652=CARTESIAN_POINT('Ctrl Pts',(181.876789994899,4.29578809292371,133.199227570696));
#203653=CARTESIAN_POINT('Ctrl Pts',(181.86901566078,4.36221812545415,133.080068824786));
#203654=CARTESIAN_POINT('Ctrl Pts',(181.861241326661,4.42379169257108,132.957955240427));
#203655=CARTESIAN_POINT('Ctrl Pts',(181.853466992542,4.480234942605,132.833320430268));
#203656=CARTESIAN_POINT('Ctrl Pts',(181.845702239595,4.53660863137767,132.708839221374));
#203657=CARTESIAN_POINT('Ctrl Pts',(181.837937486648,4.5878644235316,132.58184332178));
#203658=CARTESIAN_POINT('Ctrl Pts',(181.8301727337,4.63377325280224,132.452792752692));
#203659=CARTESIAN_POINT('Ctrl Pts',(181.822415692815,4.67963648477647,132.323870358447));
#203660=CARTESIAN_POINT('Ctrl Pts',(181.81465865193,4.72016319216763,132.192897721815));
#203661=CARTESIAN_POINT('Ctrl Pts',(181.806901611045,4.75517166757724,132.06035642742));
#203662=CARTESIAN_POINT('Ctrl Pts',(181.799150419805,4.7901537428232,131.927915083446));
#203663=CARTESIAN_POINT('Ctrl Pts',(181.791399228565,4.81962576954726,131.793907812746));
#203664=CARTESIAN_POINT('Ctrl Pts',(181.783648037325,4.84345543753907,131.658832669229));
#203665=CARTESIAN_POINT('Ctrl Pts',(181.775900140548,4.86727497728632,131.523814936251));
#203666=CARTESIAN_POINT('Ctrl Pts',(181.768152243771,4.88545686026262,131.387730617391));
#203667=CARTESIAN_POINT('Ctrl Pts',(181.760404346994,4.8979196333033,131.251089090133));
#203668=CARTESIAN_POINT('Ctrl Pts',(181.75265807091,4.91037979940052,131.114476145337));
#203669=CARTESIAN_POINT('Ctrl Pts',(181.744911794826,4.91712319960808,130.97730661308));
#203670=CARTESIAN_POINT('Ctrl Pts',(181.737165518741,4.91812017572067,130.840095749709));
#203671=CARTESIAN_POINT('Ctrl Pts',(181.729419185476,4.91911715919271,130.702883873479));
#203672=CARTESIAN_POINT('Ctrl Pts',(181.721672852211,4.91436763108547,130.565631056479));
#203673=CARTESIAN_POINT('Ctrl Pts',(181.713926518945,4.90389406809912,130.428852919426));
#203674=CARTESIAN_POINT('Ctrl Pts',(181.706178450942,4.89341815963096,130.292044151858));
#203675=CARTESIAN_POINT('Ctrl Pts',(181.698430382939,4.87721569537927,130.155710665513));
#203676=CARTESIAN_POINT('Ctrl Pts',(181.690682314937,4.85536102499316,130.020362926576));
#203677=CARTESIAN_POINT('Ctrl Pts',(181.682926012195,4.83348312720327,129.884871338452));
#203678=CARTESIAN_POINT('Ctrl Pts',(181.675169709453,4.80594108560759,129.75036797714));
#203679=CARTESIAN_POINT('Ctrl Pts',(181.667413406711,4.77286051180006,129.617353626264));
#203680=CARTESIAN_POINT('Ctrl Pts',(181.659652964197,4.73976228189421,129.484268281624));
#203681=CARTESIAN_POINT('Ctrl Pts',(181.651892521683,4.70111973963549,129.352673905927));
#203682=CARTESIAN_POINT('Ctrl Pts',(181.644132079168,4.65710811429238,129.22305512074));
#203683=CARTESIAN_POINT('Ctrl Pts',(181.636359178903,4.61302583758112,129.093228259972));
#203684=CARTESIAN_POINT('Ctrl Pts',(181.628586278637,4.5635573955876,128.965383691997));
#203685=CARTESIAN_POINT('Ctrl Pts',(181.620813378372,4.5089261594554,128.839985920346));
#203686=CARTESIAN_POINT('Ctrl Pts',(181.61332304261,4.45628090636462,128.719146673552));
#203687=CARTESIAN_POINT('Ctrl Pts',(181.605832706848,4.39884183774708,128.600579694375));
#203688=CARTESIAN_POINT('Ctrl Pts',(181.598342371086,4.33684778850805,128.484676517993));
#203689=CARTESIAN_POINT('Ctrl Pts',(181.590568036967,4.27250321604925,128.36437883745));
#203690=CARTESIAN_POINT('Ctrl Pts',(181.582793702848,4.20304761613661,128.246569876445));
#203691=CARTESIAN_POINT('Ctrl Pts',(181.575019368729,4.12869777585513,128.13171441237));
#203692=CARTESIAN_POINT('Ctrl Pts',(181.567254615782,4.05443956510713,128.01700049739));
#203693=CARTESIAN_POINT('Ctrl Pts',(181.559489862835,3.97529932571951,127.905233162034));
#203694=CARTESIAN_POINT('Ctrl Pts',(181.551725109888,3.89154027064978,127.796853778935));
#203695=CARTESIAN_POINT('Ctrl Pts',(181.543968069003,3.80786440625398,127.688582039767));
#203696=CARTESIAN_POINT('Ctrl Pts',(181.536211028118,3.71957909298195,127.583691863779));
#203697=CARTESIAN_POINT('Ctrl Pts',(181.528453987233,3.62699128433114,127.482596434803));
#203698=CARTESIAN_POINT('Ctrl Pts',(181.520702795992,3.5344732968673,127.381577242677));
#203699=CARTESIAN_POINT('Ctrl Pts',(181.512951604752,3.43765953508295,127.28434738878));
#203700=CARTESIAN_POINT('Ctrl Pts',(181.505200413512,3.33689750893684,127.191287399743));
#203701=CARTESIAN_POINT('Ctrl Pts',(181.497452516735,3.23617830933978,127.098266963683));
#203702=CARTESIAN_POINT('Ctrl Pts',(181.489704619958,3.13151446964089,127.00941313221));
#203703=CARTESIAN_POINT('Ctrl Pts',(181.481956723181,3.02329051611814,126.925069765149));
#203704=CARTESIAN_POINT('Ctrl Pts',(181.474210447097,2.91508920071343,126.840744040902));
#203705=CARTESIAN_POINT('Ctrl Pts',(181.466464171013,2.80332956091226,126.760927144587));
#203706=CARTESIAN_POINT('Ctrl Pts',(181.458717894929,2.688429065486,126.685922537134));
#203707=CARTESIAN_POINT('Ctrl Pts',(181.450971561663,2.57352772189059,126.610917376014));
#203708=CARTESIAN_POINT('Ctrl Pts',(181.443225228398,2.45548580379192,126.54072478835));
#203709=CARTESIAN_POINT('Ctrl Pts',(181.435478895133,2.33474926670635,126.475604569448));
#203710=CARTESIAN_POINT('Ctrl Pts',(181.42773082713,2.21398569151045,126.410469767325));
#203711=CARTESIAN_POINT('Ctrl Pts',(181.419982759127,2.0905266405883,126.350409779878));
#203712=CARTESIAN_POINT('Ctrl Pts',(181.412234691124,1.96484177140072,126.295637974083));
#203713=CARTESIAN_POINT('Ctrl Pts',(181.404478388382,1.83902332283823,126.240807956161));
#203714=CARTESIAN_POINT('Ctrl Pts',(181.39672208564,1.71097468939951,126.19127750357));
#203715=CARTESIAN_POINT('Ctrl Pts',(181.388965782898,1.58118509066446,126.1472116215));
#203716=CARTESIAN_POINT('Ctrl Pts',(181.381205340384,1.45132621931234,126.103122220142));
#203717=CARTESIAN_POINT('Ctrl Pts',(181.37344489787,1.31972490610537,126.064503310922));
#203718=CARTESIAN_POINT('Ctrl Pts',(181.365684455356,1.18688359259093,126.031469418289));
#203719=CARTESIAN_POINT('Ctrl Pts',(181.35791155509,1.05382903040709,125.998382496718));
#203720=CARTESIAN_POINT('Ctrl Pts',(181.350138654825,0.919530873392618,
125.970898586219));
#203721=CARTESIAN_POINT('Ctrl Pts',(181.342365754559,0.784500659081397,
125.949080833825));
#203722=CARTESIAN_POINT('Ctrl Pts',(181.334875418797,0.65437913317976,125.928056211687));
#203723=CARTESIAN_POINT('Ctrl Pts',(181.327385083035,0.523578155989451,
125.912292978468));
#203724=CARTESIAN_POINT('Ctrl Pts',(181.319894747273,0.39255623324671,125.901801829929));
#203725=CARTESIAN_POINT('Ctrl Pts',(181.312120413154,0.256566574481517,
125.890912906304));
#203726=CARTESIAN_POINT('Ctrl Pts',(181.304346079035,0.119908110764656,
125.885669248528));
#203727=CARTESIAN_POINT('Ctrl Pts',(181.296571744916,-0.0169109488048534,
125.88613969102));
#203728=CARTESIAN_POINT('Ctrl Pts',(181.288806991969,-0.153561391111778,
125.886609553735));
#203729=CARTESIAN_POINT('Ctrl Pts',(181.281042239022,-0.290371648259795,
125.892779503671));
#203730=CARTESIAN_POINT('Ctrl Pts',(181.273277486075,-0.426828107918584,
125.904666665002));
#203731=CARTESIAN_POINT('Ctrl Pts',(181.26552044519,-0.563149037097825,
125.916542019838));
#203732=CARTESIAN_POINT('Ctrl Pts',(181.257763404305,-0.699116481113278,
125.934123252056));
#203733=CARTESIAN_POINT('Ctrl Pts',(181.25000636342,-0.834216900840216,
125.957375448943));
#203734=CARTESIAN_POINT('Ctrl Pts',(181.242255172179,-0.969215440289043,
125.980610111167));
#203735=CARTESIAN_POINT('Ctrl Pts',(181.234503980939,-1.1033478731167,126.009507159861));
#203736=CARTESIAN_POINT('Ctrl Pts',(181.226752789699,-1.23610621387061,
126.043979908995));
#203737=CARTESIAN_POINT('Ctrl Pts',(181.219004892922,-1.36880812878891,
126.078438006292));
#203738=CARTESIAN_POINT('Ctrl Pts',(181.211256996145,-1.50013673559273,
126.118466992577));
#203739=CARTESIAN_POINT('Ctrl Pts',(181.203509099368,-1.62959488942576,
126.16392921964));
#203740=CARTESIAN_POINT('Ctrl Pts',(181.195762823284,-1.75902596340384,
126.209381936985));
#203741=CARTESIAN_POINT('Ctrl Pts',(181.1880165472,-1.88658699399867,126.260265505053));
#203742=CARTESIAN_POINT('Ctrl Pts',(181.180270271116,-2.01179701886858,
126.316392723589));
#203743=CARTESIAN_POINT('Ctrl Pts',(181.17252393785,-2.13700796800998,126.372520356442));
#203744=CARTESIAN_POINT('Ctrl Pts',(181.164777604585,-2.25986752003577,
126.433891557078));
#203745=CARTESIAN_POINT('Ctrl Pts',(181.15703127132,-2.37991605194676,126.500271556198));
#203746=CARTESIAN_POINT('Ctrl Pts',(181.149283203317,-2.49999146789432,
126.566666420659));
#203747=CARTESIAN_POINT('Ctrl Pts',(181.141535135314,-2.61725426899975,
126.63807212648));
#203748=CARTESIAN_POINT('Ctrl Pts',(181.133787067311,-2.73127108225299,
126.7142088676));
#203749=CARTESIAN_POINT('Ctrl Pts',(181.126030764569,-2.8454090739322,126.790426527755));
#203750=CARTESIAN_POINT('Ctrl Pts',(181.118274461827,-2.95629386060742,
126.871385050119));
#203751=CARTESIAN_POINT('Ctrl Pts',(181.110518159085,-3.06352218360704,
126.956762029739));
#203752=CARTESIAN_POINT('Ctrl Pts',(181.102757716571,-3.17080773759117,
127.042184577624));
#203753=CARTESIAN_POINT('Ctrl Pts',(181.094997274057,-3.27443264399057,
127.132030025815));
#203754=CARTESIAN_POINT('Ctrl Pts',(181.087236831543,-3.37402896821536,
127.22593755927));
#203755=CARTESIAN_POINT('Ctrl Pts',(181.079463931278,-3.4737851733016,127.319995841434));
#203756=CARTESIAN_POINT('Ctrl Pts',(181.071691031012,-3.56949959987051,
127.418128959495));
#203757=CARTESIAN_POINT('Ctrl Pts',(181.063918130747,-3.66084262200152,
127.519940674953));
#203758=CARTESIAN_POINT('Ctrl Pts',(181.056427794985,-3.7488650952,127.618051278106));
#203759=CARTESIAN_POINT('Ctrl Pts',(181.048937459222,-3.83282827290767,
127.7195774321));
#203760=CARTESIAN_POINT('Ctrl Pts',(181.04144712346,-3.9124753229297,127.824139164391));
#203761=CARTESIAN_POINT('Ctrl Pts',(181.033651562904,-3.99536792231622,
127.932961698101));
#203762=CARTESIAN_POINT('Ctrl Pts',(181.025856002347,-4.07385081342254,
128.045421065337));
#203763=CARTESIAN_POINT('Ctrl Pts',(181.018060441791,-4.14758872176929,
128.161125694682));
#203764=CARTESIAN_POINT('Ctrl Pts',(181.01027762814,-4.22120605762,128.276641129674));
#203765=CARTESIAN_POINT('Ctrl Pts',(181.00249481449,-4.29009365664689,128.395390934063));
#203766=CARTESIAN_POINT('Ctrl Pts',(180.994712000839,-4.35395702277294,
128.516951317431));
#203767=CARTESIAN_POINT('Ctrl Pts',(180.986936519403,-4.41776022301778,
128.638397178372));
#203768=CARTESIAN_POINT('Ctrl Pts',(180.979161037966,-4.47654842553653,
128.762648010892));
#203769=CARTESIAN_POINT('Ctrl Pts',(180.971385556529,-4.53007071000093,
128.889251632445));
#203770=CARTESIAN_POINT('Ctrl Pts',(180.963616832862,-4.58354647756522,
129.015745221175));
#203771=CARTESIAN_POINT('Ctrl Pts',(180.955848109195,-4.63176528846851,
129.144587172));
#203772=CARTESIAN_POINT('Ctrl Pts',(180.948079385529,-4.67452267920003,
129.275301827282));
#203773=CARTESIAN_POINT('Ctrl Pts',(180.942056030262,-4.70767393617805,
129.376649338295));
#203774=CARTESIAN_POINT('Ctrl Pts',(180.936032674994,-4.73754299834085,
129.479122066623));
#203775=CARTESIAN_POINT('Ctrl Pts',(180.930009319727,-4.76405452823405,
129.582490119308));
#203776=CARTESIAN_POINT('Ctrl Pts',(182.679902359578,-4.76405452823405,
129.582490119308));
#203777=CARTESIAN_POINT('Ctrl Pts',(182.671073039678,-4.80263856972609,
129.732928711491));
#203778=CARTESIAN_POINT('Ctrl Pts',(182.662243719779,-4.83413672793406,
129.885367666505));
#203779=CARTESIAN_POINT('Ctrl Pts',(182.65341439988,-4.85836093134102,130.039172978278));
#203780=CARTESIAN_POINT('Ctrl Pts',(182.644641758985,-4.88242962971196,
130.19199095106));
#203781=CARTESIAN_POINT('Ctrl Pts',(182.635869118089,-4.89931737459966,
130.346157623678));
#203782=CARTESIAN_POINT('Ctrl Pts',(182.627096477193,-4.90888732968651,
130.501032005425));
#203783=CARTESIAN_POINT('Ctrl Pts',(182.62144450615,-4.91505298831555,130.600813306337));
#203784=CARTESIAN_POINT('Ctrl Pts',(182.615792535106,-4.91818209306794,
130.700887987475));
#203785=CARTESIAN_POINT('Ctrl Pts',(182.610140564063,-4.91824890646276,
130.801080895348));
#203786=CARTESIAN_POINT('Origin',(213.235140564004,0.,130.804360617566));
#203787=CARTESIAN_POINT('',(184.430229652623,-4.76405452823406,129.582490119308));
#203788=CARTESIAN_POINT('',(184.084599308536,-4.76405452823405,129.582490119308));
#203789=CARTESIAN_POINT('',(213.235140564004,-4.76405452823405,129.582490119308));
#203790=CARTESIAN_POINT('',(184.014859436043,-4.9182492280365,130.801605001777));
#203791=CARTESIAN_POINT('Ctrl Pts',(184.084599308536,-4.76405452823405,
129.582490119308));
#203792=CARTESIAN_POINT('Ctrl Pts',(184.075945911235,-4.8018983817438,129.730042729782));
#203793=CARTESIAN_POINT('Ctrl Pts',(184.067292513934,-4.83292755031847,
129.879527941908));
#203794=CARTESIAN_POINT('Ctrl Pts',(184.058639116632,-4.85696110866322,
130.030337458072));
#203795=CARTESIAN_POINT('Ctrl Pts',(184.050029728944,-4.88087243667851,
130.180379984322));
#203796=CARTESIAN_POINT('Ctrl Pts',(184.041420341256,-4.89785903432467,
130.331733166547));
#203797=CARTESIAN_POINT('Ctrl Pts',(184.032810953568,-4.90779083573385,
130.483779621269));
#203798=CARTESIAN_POINT('Ctrl Pts',(184.026827114393,-4.91469380078797,
130.589457465631));
#203799=CARTESIAN_POINT('Ctrl Pts',(184.020843275218,-4.91818976220946,
130.69546982899));
#203800=CARTESIAN_POINT('Ctrl Pts',(184.014859436043,-4.9182492280365,130.801605001777));
#203801=CARTESIAN_POINT('Ctrl Pts',(184.014859435991,-4.91824922803702,
130.801605002707));
#203802=CARTESIAN_POINT('Ctrl Pts',(184.0070245266,-4.91832708928895,130.94057255142));
#203803=CARTESIAN_POINT('Ctrl Pts',(183.999189617208,-4.91251071226177,
131.079545490942));
#203804=CARTESIAN_POINT('Ctrl Pts',(183.991354707817,-4.90082530395939,
131.217996209085));
#203805=CARTESIAN_POINT('Ctrl Pts',(183.983518210813,-4.88913752780615,
131.356474981931));
#203806=CARTESIAN_POINT('Ctrl Pts',(183.97568171381,-4.87157838318562,131.494430945472));
#203807=CARTESIAN_POINT('Ctrl Pts',(183.967845216806,-4.84822496807564,
131.631341706484));
#203808=CARTESIAN_POINT('Ctrl Pts',(183.960005585196,-4.82486221157711,
131.768307231932));
#203809=CARTESIAN_POINT('Ctrl Pts',(183.952165953587,-4.79570063209204,
131.904226349297));
#203810=CARTESIAN_POINT('Ctrl Pts',(183.944326321977,-4.76086839271114,
132.038587180959));
#203811=CARTESIAN_POINT('Ctrl Pts',(183.936091824958,-4.72428172823233,
132.179715479181));
#203812=CARTESIAN_POINT('Ctrl Pts',(183.927857327939,-4.68143846664776,
132.319123983606));
#203813=CARTESIAN_POINT('Ctrl Pts',(183.91962283092,-4.63254572439523,132.456239297702));
#203814=CARTESIAN_POINT('Ctrl Pts',(183.911767314248,-4.58590319711227,
132.58704408557));
#203815=CARTESIAN_POINT('Ctrl Pts',(183.903911797577,-4.53375578798978,
132.71576172528));
#203816=CARTESIAN_POINT('Ctrl Pts',(183.896056280906,-4.47633184758892,
132.84191705918));
#203817=CARTESIAN_POINT('Ctrl Pts',(183.888194193542,-4.41885987532938,
132.968177914837));
#203818=CARTESIAN_POINT('Ctrl Pts',(183.880332106178,-4.35610274681267,
133.09187185747));
#203819=CARTESIAN_POINT('Ctrl Pts',(183.872470018814,-4.28833398097888,
133.212549715225));
#203820=CARTESIAN_POINT('Ctrl Pts',(183.864595817316,-4.2204607950577,133.333413516936));
#203821=CARTESIAN_POINT('Ctrl Pts',(183.856721615819,-4.14756075301982,
133.451251635519));
#203822=CARTESIAN_POINT('Ctrl Pts',(183.848847414322,-4.06995003088787,
133.565644704468));
#203823=CARTESIAN_POINT('Ctrl Pts',(183.847735728798,-4.05899289239229,
133.58179480158));
#203824=CARTESIAN_POINT('Ctrl Pts',(183.846624043273,-4.04794192437879,
133.597876287981));
#203825=CARTESIAN_POINT('Ctrl Pts',(183.845512357748,-4.03679807846351,
133.613888039787));
#203826=CARTESIAN_POINT('Ctrl Pts',(183.837738023629,-3.95886598381865,
133.7258627895));
#203827=CARTESIAN_POINT('Ctrl Pts',(183.82996368951,-3.87614790100592,133.834769861943));
#203828=CARTESIAN_POINT('Ctrl Pts',(183.822189355391,-3.78891333030926,
133.940172926666));
#203829=CARTESIAN_POINT('Ctrl Pts',(183.814424602444,-3.70178626842471,
134.045446091532));
#203830=CARTESIAN_POINT('Ctrl Pts',(183.806659849497,-3.61015404055219,
134.147223542661));
#203831=CARTESIAN_POINT('Ctrl Pts',(183.79889509655,-3.51432952725466,134.245097607858));
#203832=CARTESIAN_POINT('Ctrl Pts',(183.791138055665,-3.41860018821441,
134.342874463155));
#203833=CARTESIAN_POINT('Ctrl Pts',(183.78338101478,-3.31868712171636,134.436755370167));
#203834=CARTESIAN_POINT('Ctrl Pts',(183.775623973895,-3.21494336377899,
134.526365753268));
#203835=CARTESIAN_POINT('Ctrl Pts',(183.767872782655,-3.11127783981671,
134.615908560482));
#203836=CARTESIAN_POINT('Ctrl Pts',(183.760121591415,-3.00378766898042,
134.701186999335));
#203837=CARTESIAN_POINT('Ctrl Pts',(183.752370400174,-2.89286235937896,
134.781863657438));
#203838=CARTESIAN_POINT('Ctrl Pts',(183.744622503397,-2.7819841959931,134.862506025808));
#203839=CARTESIAN_POINT('Ctrl Pts',(183.73687460662,-2.66767411324236,134.938550274043));
#203840=CARTESIAN_POINT('Ctrl Pts',(183.729126709843,-2.55035410782106,
135.009699722468));
#203841=CARTESIAN_POINT('Ctrl Pts',(183.721380433759,-2.43305864321574,
135.080834287963));
#203842=CARTESIAN_POINT('Ctrl Pts',(183.713634157675,-2.31275484235268,
135.147075887609));
#203843=CARTESIAN_POINT('Ctrl Pts',(183.705887881591,-2.18989270931988,
135.20817180609));
#203844=CARTESIAN_POINT('Ctrl Pts',(183.698141548325,-2.06702966934689,
135.269268175567));
#203845=CARTESIAN_POINT('Ctrl Pts',(183.69039521506,-1.94160860959151,135.325218614004));
#203846=CARTESIAN_POINT('Ctrl Pts',(183.682648881795,-1.81410273528698,
135.375817095356));
#203847=CARTESIAN_POINT('Ctrl Pts',(183.674900813792,-1.68656830692579,
135.426426907886));
#203848=CARTESIAN_POINT('Ctrl Pts',(183.667152745789,-1.55694849830684,
135.471682234208));
#203849=CARTESIAN_POINT('Ctrl Pts',(183.659404677786,-1.4257346415192,135.511425923515));
#203850=CARTESIAN_POINT('Ctrl Pts',(183.651648375044,-1.29438132908304,
135.551211852889));
#203851=CARTESIAN_POINT('Ctrl Pts',(183.643892072302,-1.1614309589586,135.585474330078));
#203852=CARTESIAN_POINT('Ctrl Pts',(183.63613576956,-1.02738865306596,135.614106517097));
#203853=CARTESIAN_POINT('Ctrl Pts',(183.628375327046,-0.893274804758753,
135.642753985975));
#203854=CARTESIAN_POINT('Ctrl Pts',(183.620614884532,-0.758068244641496,
135.665765111291));
#203855=CARTESIAN_POINT('Ctrl Pts',(183.612854442018,-0.622281340493539,
135.683084733129));
#203856=CARTESIAN_POINT('Ctrl Pts',(183.605081541752,-0.486276459152402,
135.700432157962));
#203857=CARTESIAN_POINT('Ctrl Pts',(183.597308641487,-0.349689761885385,
135.712069788455));
#203858=CARTESIAN_POINT('Ctrl Pts',(183.589535741221,-0.213036659942975,
135.717994552244));
#203859=CARTESIAN_POINT('Ctrl Pts',(183.582045405459,-0.0813512424637309,
135.723703935946));
#203860=CARTESIAN_POINT('Ctrl Pts',(183.574555069697,0.0503955275397817,
135.724108595028));
#203861=CARTESIAN_POINT('Ctrl Pts',(183.567064733935,0.181747024582314,
135.719251367273));
#203862=CARTESIAN_POINT('Ctrl Pts',(183.559290399816,0.318078753557754,
135.714209976251));
#203863=CARTESIAN_POINT('Ctrl Pts',(183.551516065697,0.45441650227473,135.703483843342));
#203864=CARTESIAN_POINT('Ctrl Pts',(183.543741731578,0.590247502080792,
135.687063859499));
#203865=CARTESIAN_POINT('Ctrl Pts',(183.535976978631,0.725911102318697,
135.67066411182));
#203866=CARTESIAN_POINT('Ctrl Pts',(183.528212225684,0.861068811846414,
135.648584521738));
#203867=CARTESIAN_POINT('Ctrl Pts',(183.520447472737,0.995208524915738,
135.620867967756));
#203868=CARTESIAN_POINT('Ctrl Pts',(183.512690431852,1.12921500853146,135.593178942246));
#203869=CARTESIAN_POINT('Ctrl Pts',(183.504933390967,1.26220512740057,135.559864173125));
#203870=CARTESIAN_POINT('Ctrl Pts',(183.497176350082,1.39367291584853,135.521018212318));
#203871=CARTESIAN_POINT('Ctrl Pts',(183.489425158842,1.52504156341419,135.482201545552));
#203872=CARTESIAN_POINT('Ctrl Pts',(183.481673967602,1.65488979216254,135.43786209979));
#203873=CARTESIAN_POINT('Ctrl Pts',(183.473922776362,1.78272318884635,135.388145199595));
#203874=CARTESIAN_POINT('Ctrl Pts',(183.466174879585,1.91050225292687,135.33844943041));
#203875=CARTESIAN_POINT('Ctrl Pts',(183.458426982807,2.0362678245576,135.283380894017));
#203876=CARTESIAN_POINT('Ctrl Pts',(183.45067908603,2.15954219920582,135.223134265576));
#203877=CARTESIAN_POINT('Ctrl Pts',(183.442932809946,2.28279078751236,135.162900239432));
#203878=CARTESIAN_POINT('Ctrl Pts',(183.435186533862,2.40354886430429,135.097490447235));
#203879=CARTESIAN_POINT('Ctrl Pts',(183.427440257778,2.52136057482751,135.027146891367));
#203880=CARTESIAN_POINT('Ctrl Pts',(183.419693924513,2.63917315501009,134.95680281624));
#203881=CARTESIAN_POINT('Ctrl Pts',(183.411947591247,2.7540389898437,134.881525105199));
#203882=CARTESIAN_POINT('Ctrl Pts',(183.404201257982,2.86552896479428,134.8016005171));
#203883=CARTESIAN_POINT('Ctrl Pts',(183.396453189979,2.97704390715139,134.721658030443));
#203884=CARTESIAN_POINT('Ctrl Pts',(183.388705121976,3.08518116758142,134.637066823728));
#203885=CARTESIAN_POINT('Ctrl Pts',(183.380957053973,3.18954295366573,134.548155324708));
#203886=CARTESIAN_POINT('Ctrl Pts',(183.373200751231,3.29401565669837,134.459149329488));
#203887=CARTESIAN_POINT('Ctrl Pts',(183.36544444849,3.3947045716674,134.36581412358));
#203888=CARTESIAN_POINT('Ctrl Pts',(183.357688145748,3.49124678201167,134.268516931821));
#203889=CARTESIAN_POINT('Ctrl Pts',(183.349927703234,3.58784051984049,134.171167809621));
#203890=CARTESIAN_POINT('Ctrl Pts',(183.342167260719,3.68028287962462,134.069852776656));
#203891=CARTESIAN_POINT('Ctrl Pts',(183.334406818205,3.76825050646584,133.964973087171));
#203892=CARTESIAN_POINT('Ctrl Pts',(183.32663391794,3.85635934675105,133.859925035496));
#203893=CARTESIAN_POINT('Ctrl Pts',(183.318861017674,3.93997886106847,133.751301202296));
#203894=CARTESIAN_POINT('Ctrl Pts',(183.311088117409,4.01882787217965,133.639533556964));
#203895=CARTESIAN_POINT('Ctrl Pts',(183.303597781647,4.094810523129,133.531828947063));
#203896=CARTESIAN_POINT('Ctrl Pts',(183.296107445885,4.16636332155617,133.421205386315));
#203897=CARTESIAN_POINT('Ctrl Pts',(183.288617110123,4.23327549087247,133.308070201539));
#203898=CARTESIAN_POINT('Ctrl Pts',(183.280842776004,4.3027246554253,133.190645461847));
#203899=CARTESIAN_POINT('Ctrl Pts',(183.273068441885,4.36739433944492,133.070142915728));
#203900=CARTESIAN_POINT('Ctrl Pts',(183.265294107765,4.42699971525186,132.94698904631));
#203901=CARTESIAN_POINT('Ctrl Pts',(183.257529354818,4.48653163276008,132.823986953029));
#203902=CARTESIAN_POINT('Ctrl Pts',(183.249764601871,4.5410114917085,132.698340386375));
#203903=CARTESIAN_POINT('Ctrl Pts',(183.241999848924,4.59019856132849,132.570503372294));
#203904=CARTESIAN_POINT('Ctrl Pts',(183.234242808039,4.63933677765773,132.442793327737));
#203905=CARTESIAN_POINT('Ctrl Pts',(183.226485767154,4.6831925265859,132.312897527787));
#203906=CARTESIAN_POINT('Ctrl Pts',(183.218728726269,4.72157187051949,132.181292763323));
#203907=CARTESIAN_POINT('Ctrl Pts',(183.210977535029,4.75992227229126,132.049787243035));
#203908=CARTESIAN_POINT('Ctrl Pts',(183.203226343789,4.79280438017088,131.91657569721));
#203909=CARTESIAN_POINT('Ctrl Pts',(183.195475152549,4.82007321739351,131.782152641192));
#203910=CARTESIAN_POINT('Ctrl Pts',(183.187727255772,4.84733046463286,131.647786718558));
#203911=CARTESIAN_POINT('Ctrl Pts',(183.179979358994,4.86897910880454,131.512210692235));
#203912=CARTESIAN_POINT('Ctrl Pts',(183.172231462217,4.88492472466578,131.375931695254));
#203913=CARTESIAN_POINT('Ctrl Pts',(183.164485186133,4.90086700504792,131.239681204901));
#203914=CARTESIAN_POINT('Ctrl Pts',(183.156738910049,4.91110858455677,131.102728424444));
#203915=CARTESIAN_POINT('Ctrl Pts',(183.148992633965,4.91560666602142,130.965587685597));
#203916=CARTESIAN_POINT('Ctrl Pts',(183.1412463007,4.92010478068989,130.828445934408));
#203917=CARTESIAN_POINT('Ctrl Pts',(183.133499967434,4.91885929989721,130.691116612814));
#203918=CARTESIAN_POINT('Ctrl Pts',(183.125753634169,4.91187953510186,130.554115747194));
#203919=CARTESIAN_POINT('Ctrl Pts',(183.118005566166,4.90489820723658,130.417084201179));
#203920=CARTESIAN_POINT('Ctrl Pts',(183.110257498163,4.89218005994142,130.280381647888));
#203921=CARTESIAN_POINT('Ctrl Pts',(183.10250943016,4.87378639226766,130.144520284571));
#203922=CARTESIAN_POINT('Ctrl Pts',(183.094753127418,4.85537317558499,130.00851452618));
#203923=CARTESIAN_POINT('Ctrl Pts',(183.086996824676,4.83127244146896,129.873352131727));
#203924=CARTESIAN_POINT('Ctrl Pts',(183.079240521934,4.80159698130756,129.739536927184));
#203925=CARTESIAN_POINT('Ctrl Pts',(183.07148007942,4.77190568245958,129.605650301438));
#203926=CARTESIAN_POINT('Ctrl Pts',(183.063719636906,4.73663382932912,129.473112675974));
#203927=CARTESIAN_POINT('Ctrl Pts',(183.055959194392,4.69594422725383,129.342412986144));
#203928=CARTESIAN_POINT('Ctrl Pts',(183.048186294126,4.65518930661703,129.211503485568));
#203929=CARTESIAN_POINT('Ctrl Pts',(183.040413393861,4.6089993893674,129.082438184816));
#203930=CARTESIAN_POINT('Ctrl Pts',(183.032640493595,4.55758592042437,128.955687136269));
#203931=CARTESIAN_POINT('Ctrl Pts',(183.025150157833,4.50804146058063,128.833543807605));
#203932=CARTESIAN_POINT('Ctrl Pts',(183.017659822071,4.453646761226,128.713549675095));
#203933=CARTESIAN_POINT('Ctrl Pts',(183.010169486309,4.39463058805635,128.596102241148));
#203934=CARTESIAN_POINT('Ctrl Pts',(183.00239515219,4.33337679874275,128.474201752045));
#203935=CARTESIAN_POINT('Ctrl Pts',(182.994620818071,4.26695013774061,128.354658745723));
#203936=CARTESIAN_POINT('Ctrl Pts',(182.986846483952,4.19555546106626,128.237943380323));
#203937=CARTESIAN_POINT('Ctrl Pts',(182.979081731005,4.1242487719503,128.121371856181));
#203938=CARTESIAN_POINT('Ctrl Pts',(182.971316978058,4.0479864514346,128.007621369533));
#203939=CARTESIAN_POINT('Ctrl Pts',(182.963552225111,3.96702036354612,127.897139866108));
#203940=CARTESIAN_POINT('Ctrl Pts',(182.955795184226,3.88613469231738,127.786768094469));
#203941=CARTESIAN_POINT('Ctrl Pts',(182.948038143341,3.80055478051184,127.679659158082));
#203942=CARTESIAN_POINT('Ctrl Pts',(182.940281102456,3.71057693779105,127.576233939253));
#203943=CARTESIAN_POINT('Ctrl Pts',(182.932529911216,3.62066694806208,127.472886714187));
#203944=CARTESIAN_POINT('Ctrl Pts',(182.924778719976,3.52636588431209,127.373217971168));
#203945=CARTESIAN_POINT('Ctrl Pts',(182.917027528736,3.42801143282299,127.277616980876));
#203946=CARTESIAN_POINT('Ctrl Pts',(182.909279631959,3.3296987845988,127.182056623554));
#203947=CARTESIAN_POINT('Ctrl Pts',(182.901531735182,3.22733645491275,127.090560852235));
#203948=CARTESIAN_POINT('Ctrl Pts',(182.893783838404,3.12130006999723,127.003483227339));
#203949=CARTESIAN_POINT('Ctrl Pts',(182.88603756232,3.01528586560767,126.916423817206));
#203950=CARTESIAN_POINT('Ctrl Pts',(182.878291286236,2.90559943659399,126.833780963214));
#203951=CARTESIAN_POINT('Ctrl Pts',(182.870545010152,2.79265037187774,126.75586868069));
#203952=CARTESIAN_POINT('Ctrl Pts',(182.862798676887,2.67970047339745,126.677955823035));
#203953=CARTESIAN_POINT('Ctrl Pts',(182.855052343622,2.5634882129824,126.604773828524));
#203954=CARTESIAN_POINT('Ctrl Pts',(182.847306010356,2.4444527713082,126.536593788023));
#203955=CARTESIAN_POINT('Ctrl Pts',(182.839557942353,2.32539067247181,126.468398479076));
#203956=CARTESIAN_POINT('Ctrl Pts',(182.83180987435,2.2035044734996,126.405207547392));
#203957=CARTESIAN_POINT('Ctrl Pts',(182.824061806347,2.07925823407926,126.34724627547));
#203958=CARTESIAN_POINT('Ctrl Pts',(182.816305503605,1.9548799442771,126.289223401619));
#203959=CARTESIAN_POINT('Ctrl Pts',(182.808549200864,1.82813695834241,126.236441456072));
#203960=CARTESIAN_POINT('Ctrl Pts',(182.800792898122,1.69951412583694,126.189077874485));
#203961=CARTESIAN_POINT('Ctrl Pts',(182.793032455608,1.57082264345299,126.141689013529));
#203962=CARTESIAN_POINT('Ctrl Pts',(182.785272013093,1.44024968730915,126.099724398543));
#203963=CARTESIAN_POINT('Ctrl Pts',(182.777511570579,1.3082946128271,126.063311338287));
#203964=CARTESIAN_POINT('Ctrl Pts',(182.769738670314,1.17612771234498,126.026839824555));
#203965=CARTESIAN_POINT('Ctrl Pts',(182.761965770048,1.04257464097785,125.995937762452));
#203966=CARTESIAN_POINT('Ctrl Pts',(182.754192869783,0.908145158251714,
125.970681332172));
#203967=CARTESIAN_POINT('Ctrl Pts',(182.746702534021,0.778602525828482,
125.94634303675));
#203968=CARTESIAN_POINT('Ctrl Pts',(182.739212198259,0.64824640006857,125.927247078214));
#203969=CARTESIAN_POINT('Ctrl Pts',(182.731721862497,0.517534864453755,
125.913415849265));
#203970=CARTESIAN_POINT('Ctrl Pts',(182.723947528378,0.381867361238935,
125.899060205066));
#203971=CARTESIAN_POINT('Ctrl Pts',(182.716173194259,0.245387211553195,
125.890330921351));
#203972=CARTESIAN_POINT('Ctrl Pts',(182.708398860139,0.108600702437423,
125.88730977891));
#203973=CARTESIAN_POINT('Ctrl Pts',(182.700634107192,-0.0280172295310573,
125.884292359757));
#203974=CARTESIAN_POINT('Ctrl Pts',(182.692869354245,-0.164940382578901,
125.886969093325));
#203975=CARTESIAN_POINT('Ctrl Pts',(182.685104601298,-0.301655748620083,
125.895370204882));
#203976=CARTESIAN_POINT('Ctrl Pts',(182.677347560413,-0.438235327031179,
125.903762972337));
#203977=CARTESIAN_POINT('Ctrl Pts',(182.669590519528,-0.57460714143116,
125.91786877949));
#203978=CARTESIAN_POINT('Ctrl Pts',(182.661833478643,-0.710256929006805,
125.937665829797));
#203979=CARTESIAN_POINT('Ctrl Pts',(182.654082287403,-0.845804422024122,
125.957447950995));
#203980=CARTESIAN_POINT('Ctrl Pts',(182.646331096163,-0.980630586681961,
125.982912716527));
#203981=CARTESIAN_POINT('Ctrl Pts',(182.638579904923,-1.11422539084784,
126.013986431671));
#203982=CARTESIAN_POINT('Ctrl Pts',(182.630832008146,-1.24776341365743,
126.045046939657));
#203983=CARTESIAN_POINT('Ctrl Pts',(182.623084111369,-1.38007073689753,
126.081711567367));
#203984=CARTESIAN_POINT('Ctrl Pts',(182.615336214591,-1.51064686501784,
126.123855397858));
#203985=CARTESIAN_POINT('Ctrl Pts',(182.607589938507,-1.64119567942685,
126.165990412768));
#203986=CARTESIAN_POINT('Ctrl Pts',(182.599843662423,-1.7700136471794,126.213602230732));
#203987=CARTESIAN_POINT('Ctrl Pts',(182.592097386339,-1.89661518547082,
126.266515985944));
#203988=CARTESIAN_POINT('Ctrl Pts',(182.584351053074,-2.02321765830595,
126.319430131753));
#203989=CARTESIAN_POINT('Ctrl Pts',(182.576604719809,-2.14760330830669,
126.37764614214));
#203990=CARTESIAN_POINT('Ctrl Pts',(182.568858386543,-2.26930667116602,
126.440941053199));
#203991=CARTESIAN_POINT('Ctrl Pts',(182.56111031854,-2.39103728865015,126.504250138715));
#203992=CARTESIAN_POINT('Ctrl Pts',(182.553362250537,-2.51008407691616,
126.572640207808));
#203993=CARTESIAN_POINT('Ctrl Pts',(182.545614182534,-2.62600666382235,
126.645842604612));
#203994=CARTESIAN_POINT('Ctrl Pts',(182.537857879792,-2.74205245463323,
126.719122801795));
#203995=CARTESIAN_POINT('Ctrl Pts',(182.53010157705,-2.85496708005182,126.797225334571));
#203996=CARTESIAN_POINT('Ctrl Pts',(182.522345274309,-2.96433918540366,
126.879838193579));
#203997=CARTESIAN_POINT('Ctrl Pts',(182.514584831794,-3.07376966594129,
126.962495145556));
#203998=CARTESIAN_POINT('Ctrl Pts',(182.50682438928,-3.17965355724597,127.049666972136));
#203999=CARTESIAN_POINT('Ctrl Pts',(182.499063946766,-3.28161383704965,
127.141002364953));
#204000=CARTESIAN_POINT('Ctrl Pts',(182.491291046501,-3.38373779254603,
127.232484377452));
#204001=CARTESIAN_POINT('Ctrl Pts',(182.483518146235,-3.4819252698745,127.328143039421));
#204002=CARTESIAN_POINT('Ctrl Pts',(182.47574524597,-3.57583663900372,127.427590652991));
#204003=CARTESIAN_POINT('Ctrl Pts',(182.468254910208,-3.66633409331571,
127.523423095313));
#204004=CARTESIAN_POINT('Ctrl Pts',(182.460764574446,-3.75286073415508,
127.622773563756));
#204005=CARTESIAN_POINT('Ctrl Pts',(182.453274238684,-3.83515011659531,
127.725268763516));
#204006=CARTESIAN_POINT('Ctrl Pts',(182.445516365561,-3.92037868426403,
127.831424853274));
#204007=CARTESIAN_POINT('Ctrl Pts',(182.437758492438,-4.00133819468862,
127.941298988973));
#204008=CARTESIAN_POINT('Ctrl Pts',(182.430000619315,-4.07768537362654,
128.054512429718));
#204009=CARTESIAN_POINT('Ctrl Pts',(182.422064270311,-4.15578897855251,
128.170330433359));
#204010=CARTESIAN_POINT('Ctrl Pts',(182.414127921308,-4.22906513008165,
128.289642999518));
#204011=CARTESIAN_POINT('Ctrl Pts',(182.406191572305,-4.29718794017761,
128.4120063651));
#204012=CARTESIAN_POINT('Ctrl Pts',(182.398453166183,-4.36361167865667,
128.53131782896));
#204013=CARTESIAN_POINT('Ctrl Pts',(182.390714760061,-4.42513586114829,
128.653529356966));
#204014=CARTESIAN_POINT('Ctrl Pts',(182.382976353939,-4.48150092218885,
128.778198593709));
#204015=CARTESIAN_POINT('Ctrl Pts',(182.374941033495,-4.54002865001674,
128.907651255019));
#204016=CARTESIAN_POINT('Ctrl Pts',(182.366905713051,-4.5929932099943,129.039753638606));
#204017=CARTESIAN_POINT('Ctrl Pts',(182.358870392607,-4.64015582391395,
129.173981216231));
#204018=CARTESIAN_POINT('Ctrl Pts',(182.350835072163,-4.68731843783359,
129.308208793856));
#204019=CARTESIAN_POINT('Ctrl Pts',(182.342799751719,-4.72867891245574,
129.444561130289));
#204020=CARTESIAN_POINT('Ctrl Pts',(182.334764431275,-4.76405452823405,
129.582490119308));
#204021=CARTESIAN_POINT('',(184.360140563971,-4.91824943376093,130.802000573005));
#204022=CARTESIAN_POINT('Ctrl Pts',(184.360140563971,-4.91824943376093,
130.802000573005));
#204023=CARTESIAN_POINT('Ctrl Pts',(184.352455145915,-4.9183142156431,130.937003725306));
#204024=CARTESIAN_POINT('Ctrl Pts',(184.344769727858,-4.9128161630471,131.072233610613));
#204025=CARTESIAN_POINT('Ctrl Pts',(184.337084309801,-4.90172557734377,
131.207187412745));
#204026=CARTESIAN_POINT('Ctrl Pts',(184.329407784764,-4.89064782487823,
131.341985055925));
#204027=CARTESIAN_POINT('Ctrl Pts',(184.321731259727,-4.87399044269163,
131.476506855924));
#204028=CARTESIAN_POINT('Ctrl Pts',(184.314054734689,-4.85177572413915,
131.610248565828));
#204029=CARTESIAN_POINT('Ctrl Pts',(184.306385156566,-4.82958110892026,
131.743869245425));
#204030=CARTESIAN_POINT('Ctrl Pts',(184.298715578444,-4.80183922716559,
131.876710846574));
#204031=CARTESIAN_POINT('Ctrl Pts',(184.291046000321,-4.76862425691908,
132.008273304941));
#204032=CARTESIAN_POINT('Ctrl Pts',(184.283267874699,-4.73493919537421,
132.141697766086));
#204033=CARTESIAN_POINT('Ctrl Pts',(184.275489749077,-4.69562496363401,
132.273806182506));
#204034=CARTESIAN_POINT('Ctrl Pts',(184.267711623456,-4.65081294627124,
132.404086219441));
#204035=CARTESIAN_POINT('Ctrl Pts',(184.260049224998,-4.606667666365,132.532427879451));
#204036=CARTESIAN_POINT('Ctrl Pts',(184.252386826541,-4.55718721851533,
132.658994805512));
#204037=CARTESIAN_POINT('Ctrl Pts',(184.244724428084,-4.50254756195381,
132.783311985044));
#204038=CARTESIAN_POINT('Ctrl Pts',(184.237062723623,-4.44791285419833,
132.90761790496));
#204039=CARTESIAN_POINT('Ctrl Pts',(184.229401019162,-4.38812002801154,
133.029674116977));
#204040=CARTESIAN_POINT('Ctrl Pts',(184.221739314701,-4.32339297491415,
133.149026104787));
#204041=CARTESIAN_POINT('Ctrl Pts',(184.214076556531,-4.25865701995485,
133.268394506983));
#204042=CARTESIAN_POINT('Ctrl Pts',(184.206413798362,-4.18898567966582,
133.385057593469));
#204043=CARTESIAN_POINT('Ctrl Pts',(184.198751040193,-4.11464827331411,
133.498586415344));
#204044=CARTESIAN_POINT('Ctrl Pts',(184.190886035627,-4.0383488485568,133.615111651125));
#204045=CARTESIAN_POINT('Ctrl Pts',(184.183021031061,-3.95713386805491,
133.728334497134));
#204046=CARTESIAN_POINT('Ctrl Pts',(184.175156026495,-3.87134055205237,
133.837824873583));
#204047=CARTESIAN_POINT('Ctrl Pts',(184.167481864777,-3.78762899462731,
133.944658486767));
#204048=CARTESIAN_POINT('Ctrl Pts',(184.159807703058,-3.69955904336469,
134.047938419428));
#204049=CARTESIAN_POINT('Ctrl Pts',(184.15213354134,-3.60748270613891,134.147301177523));
#204050=CARTESIAN_POINT('Ctrl Pts',(184.14417311535,-3.51197170509786,134.25037040006));
#204051=CARTESIAN_POINT('Ctrl Pts',(184.136212689361,-3.41214997576047,
134.34922420526));
#204052=CARTESIAN_POINT('Ctrl Pts',(184.128252263371,-3.30844873692504,
134.443502002239));
#204053=CARTESIAN_POINT('Ctrl Pts',(184.120291837381,-3.2047474980896,134.537779799218));
#204054=CARTESIAN_POINT('Ctrl Pts',(184.112331411392,-3.09716715988707,
134.627481342045));
#204055=CARTESIAN_POINT('Ctrl Pts',(184.104370985402,-2.98617212354664,
134.712296020186));
#204056=CARTESIAN_POINT('Ctrl Pts',(184.096596651283,-2.87777183200501,
134.795127975026));
#204057=CARTESIAN_POINT('Ctrl Pts',(184.088822317164,-2.76575077820207,
134.873577418346));
#204058=CARTESIAN_POINT('Ctrl Pts',(184.081047983045,-2.65049881953031,
134.947311144687));
#204059=CARTESIAN_POINT('Ctrl Pts',(184.073283230098,-2.53538889859732,
135.020954000799));
#204060=CARTESIAN_POINT('Ctrl Pts',(184.065518477151,-2.41705632156664,
135.089892494809));
#204061=CARTESIAN_POINT('Ctrl Pts',(184.057753724204,-2.29592350409848,
135.153833956469));
#204062=CARTESIAN_POINT('Ctrl Pts',(184.049996683319,-2.17491099745172,
135.217711910569));
#204063=CARTESIAN_POINT('Ctrl Pts',(184.042239642434,-2.05110412867136,
135.27660252783));
#204064=CARTESIAN_POINT('Ctrl Pts',(184.034482601549,-1.92495344569139,
135.330256914922));
#204065=CARTESIAN_POINT('Ctrl Pts',(184.026731410308,-1.79889789392326,
135.383870840824));
#204066=CARTESIAN_POINT('Ctrl Pts',(184.018980219068,-1.67050240435444,
135.432256243768));
#204067=CARTESIAN_POINT('Ctrl Pts',(184.011229027828,-1.54024090802878,
135.475210755146));
#204068=CARTESIAN_POINT('Ctrl Pts',(184.003481131051,-1.41003477631391,
135.518147009712));
#204069=CARTESIAN_POINT('Ctrl Pts',(183.995733234274,-1.27796458578426,
135.55565684151));
#204070=CARTESIAN_POINT('Ctrl Pts',(183.987985337497,-1.14452276743259,
135.587586589369));
#204071=CARTESIAN_POINT('Ctrl Pts',(183.980239061413,-1.01110886223263,
135.619509658213));
#204072=CARTESIAN_POINT('Ctrl Pts',(183.972492785329,-0.876324279891128,
135.645854873884));
#204073=CARTESIAN_POINT('Ctrl Pts',(183.964746509245,-0.740674697423658,
135.666518991693));
#204074=CARTESIAN_POINT('Ctrl Pts',(183.957000175979,-0.605024113621508,
135.68718326204));
#204075=CARTESIAN_POINT('Ctrl Pts',(183.949253842714,-0.468508903458449,
135.702166291965));
#204076=CARTESIAN_POINT('Ctrl Pts',(183.941507509448,-0.331642581234947,
135.711416380527));
#204077=CARTESIAN_POINT('Ctrl Pts',(183.933759441445,-0.194745608747665,
135.720668540583));
#204078=CARTESIAN_POINT('Ctrl Pts',(183.926011373442,-0.0574977577378105,
135.724185178199));
#204079=CARTESIAN_POINT('Ctrl Pts',(183.918263305439,0.0795851196291304,
135.721966668403));
#204080=CARTESIAN_POINT('Ctrl Pts',(183.910507002698,0.216813690309234,
135.719745800749));
#204081=CARTESIAN_POINT('Ctrl Pts',(183.902750699956,0.353876545556638,
135.711777615836));
#204082=CARTESIAN_POINT('Ctrl Pts',(183.894994397214,0.490260064193617,
135.698114609335));
#204083=CARTESIAN_POINT('Ctrl Pts',(183.8872339547,0.626716374821129,135.684444310477));
#204084=CARTESIAN_POINT('Ctrl Pts',(183.879473512186,0.762492239505508,
135.665073188767));
#204085=CARTESIAN_POINT('Ctrl Pts',(183.871713069671,0.89708291638147,135.640105162477));
#204086=CARTESIAN_POINT('Ctrl Pts',(183.863940169406,1.03188965016026,135.615097055295));
#204087=CARTESIAN_POINT('Ctrl Pts',(183.856167269141,1.16550701288779,135.58447417673));
#204088=CARTESIAN_POINT('Ctrl Pts',(183.848394368875,1.29744326874112,135.548390974435));
#204089=CARTESIAN_POINT('Ctrl Pts',(183.840904033113,1.42458330936598,135.513619487432));
#204090=CARTESIAN_POINT('Ctrl Pts',(183.833413697351,1.55016205245454,135.473777870507));
#204091=CARTESIAN_POINT('Ctrl Pts',(183.825923361589,1.67375775862039,135.42904633964));
#204092=CARTESIAN_POINT('Ctrl Pts',(183.81814902747,1.80203963355247,135.382618799184));
#204093=CARTESIAN_POINT('Ctrl Pts',(183.810374693351,1.92859148786851,135.330776154368));
#204094=CARTESIAN_POINT('Ctrl Pts',(183.802600359232,2.05292225893399,135.273666297565));
#204095=CARTESIAN_POINT('Ctrl Pts',(183.794835606285,2.17709980343563,135.216626823557));
#204096=CARTESIAN_POINT('Ctrl Pts',(183.787070853338,2.29906135920444,135.154333215077));
#204097=CARTESIAN_POINT('Ctrl Pts',(183.779306100391,2.41833236849072,135.086982666966));
#204098=CARTESIAN_POINT('Ctrl Pts',(183.771549059506,2.53748491612928,135.019699012369));
#204099=CARTESIAN_POINT('Ctrl Pts',(183.763792018621,2.65395189702597,134.947368604385));
#204100=CARTESIAN_POINT('Ctrl Pts',(183.756034977736,2.76728037800997,134.870235968826));
#204101=CARTESIAN_POINT('Ctrl Pts',(183.748283786496,2.88052339710438,134.793161499588));
#204102=CARTESIAN_POINT('Ctrl Pts',(183.740532595256,2.99063230529288,134.711292230035));
#204103=CARTESIAN_POINT('Ctrl Pts',(183.732781404016,3.09718067282804,134.624917506602));
#204104=CARTESIAN_POINT('Ctrl Pts',(183.725033507239,3.20368375446525,134.53857949473));
#204105=CARTESIAN_POINT('Ctrl Pts',(183.717285610461,3.30662900226592,134.447740083331));
#204106=CARTESIAN_POINT('Ctrl Pts',(183.709537713684,3.4056209657537,134.352730510928));
#204107=CARTESIAN_POINT('Ctrl Pts',(183.7017914376,3.50459222225675,134.25774081248));
#204108=CARTESIAN_POINT('Ctrl Pts',(183.694045161516,3.59961155738863,134.158582958646));
#204109=CARTESIAN_POINT('Ctrl Pts',(183.686298885432,3.6903187776887,134.055626583546));
#204110=CARTESIAN_POINT('Ctrl Pts',(183.678552552167,3.78102666756886,133.952669448445));
#204111=CARTESIAN_POINT('Ctrl Pts',(183.670806218901,3.86742212064859,133.845914029478));
#204112=CARTESIAN_POINT('Ctrl Pts',(183.663059885636,3.94918407243948,133.73576441515));
#204113=CARTESIAN_POINT('Ctrl Pts',(183.655311817633,4.03096433425261,133.625590133579));
#204114=CARTESIAN_POINT('Ctrl Pts',(183.64756374963,4.10810879701171,133.512020457994));
#204115=CARTESIAN_POINT('Ctrl Pts',(183.639815681627,4.18033894554159,133.395489592142));
#204116=CARTESIAN_POINT('Ctrl Pts',(183.632059378885,4.25264586113286,133.278834875899));
#204117=CARTESIAN_POINT('Ctrl Pts',(183.624303076144,4.32002782270208,133.159213015378));
#204118=CARTESIAN_POINT('Ctrl Pts',(183.616546773402,4.38225137155276,133.037084509816));
#204119=CARTESIAN_POINT('Ctrl Pts',(183.608786330888,4.444508130985,132.914890820593));
#204120=CARTESIAN_POINT('Ctrl Pts',(183.601025888373,4.50160082904401,132.790188175812));
#204121=CARTESIAN_POINT('Ctrl Pts',(183.593265445859,4.55334406980649,132.663457399463));
#204122=CARTESIAN_POINT('Ctrl Pts',(183.585492545594,4.60517037341259,132.53652318362));
#204123=CARTESIAN_POINT('Ctrl Pts',(183.577719645328,4.65162992673136,132.407554698248));
#204124=CARTESIAN_POINT('Ctrl Pts',(183.569946745063,4.69258687572239,132.277049137348));
#204125=CARTESIAN_POINT('Ctrl Pts',(183.562456409301,4.73205493645361,132.15128778231));
#204126=CARTESIAN_POINT('Ctrl Pts',(183.554966073539,4.7664134338327,132.024099462039));
#204127=CARTESIAN_POINT('Ctrl Pts',(183.547475737777,4.79558602822751,131.895936408965));
#204128=CARTESIAN_POINT('Ctrl Pts',(183.539701403658,4.82586471040535,131.762914014781));
#204129=CARTESIAN_POINT('Ctrl Pts',(183.531927069538,4.85065239351974,131.62842013976));
#204130=CARTESIAN_POINT('Ctrl Pts',(183.524152735419,4.86980807226552,131.492947868245));
#204131=CARTESIAN_POINT('Ctrl Pts',(183.516387982472,4.88894014334924,131.357642554197));
#204132=CARTESIAN_POINT('Ctrl Pts',(183.508623229525,4.90245396625799,131.221361626208));
#204133=CARTESIAN_POINT('Ctrl Pts',(183.500858476578,4.91025893654111,131.084610931782));
#204134=CARTESIAN_POINT('Ctrl Pts',(183.493101435693,4.91805615481771,130.947996060074));
#204135=CARTESIAN_POINT('Ctrl Pts',(183.485344394808,4.92015578211555,130.810912738245));
#204136=CARTESIAN_POINT('Ctrl Pts',(183.477587353923,4.91651872348393,130.673874203975));
#204137=CARTESIAN_POINT('Ctrl Pts',(183.469836162683,4.9128844075865,130.536939011528));
#204138=CARTESIAN_POINT('Ctrl Pts',(183.462084971443,4.90352202688916,130.40004892866));
#204139=CARTESIAN_POINT('Ctrl Pts',(183.454333780202,4.88844452104653,130.263719121609));
#204140=CARTESIAN_POINT('Ctrl Pts',(183.446585883425,4.87337342354616,130.127447258364));
#204141=CARTESIAN_POINT('Ctrl Pts',(183.438837986648,4.85259207504386,129.991735585091));
#204142=CARTESIAN_POINT('Ctrl Pts',(183.431090089871,4.82616540524861,129.857095847989));
#204143=CARTESIAN_POINT('Ctrl Pts',(183.423343813787,4.79974426334297,129.722484274618));
#204144=CARTESIAN_POINT('Ctrl Pts',(183.415597537703,4.76768022423145,129.588944574821));
#204145=CARTESIAN_POINT('Ctrl Pts',(183.407851261619,4.73008957820223,129.45697958583));
#204146=CARTESIAN_POINT('Ctrl Pts',(183.400104928353,4.69249865468751,129.325013622703));
#204147=CARTESIAN_POINT('Ctrl Pts',(183.392358595088,4.64938114995637,129.194622769583));
#204148=CARTESIAN_POINT('Ctrl Pts',(183.384612261823,4.60090349191246,129.066295566825));
#204149=CARTESIAN_POINT('Ctrl Pts',(183.37686419382,4.55241497763291,128.937939626078));
#204150=CARTESIAN_POINT('Ctrl Pts',(183.369116125817,4.49856405958199,128.811648620967));
#204151=CARTESIAN_POINT('Ctrl Pts',(183.361368057814,4.43956550141456,128.687891571927));
#204152=CARTESIAN_POINT('Ctrl Pts',(183.353611755072,4.38050423887763,128.564002992422));
#204153=CARTESIAN_POINT('Ctrl Pts',(183.34585545233,4.31628457587822,128.44265410226));
#204154=CARTESIAN_POINT('Ctrl Pts',(183.338099149588,4.24716775333799,128.324290227939));
#204155=CARTESIAN_POINT('Ctrl Pts',(183.330338707074,4.17801404106853,128.205863179254));
#204156=CARTESIAN_POINT('Ctrl Pts',(183.32257826456,4.10395817211934,128.090424649892));
#204157=CARTESIAN_POINT('Ctrl Pts',(183.314817822046,4.02530446630552,127.978390515806));
#204158=CARTESIAN_POINT('Ctrl Pts',(183.30704492178,3.94652449858048,127.866176534582));
#204159=CARTESIAN_POINT('Ctrl Pts',(183.299272021515,3.86313218266577,127.757378179998));
#204160=CARTESIAN_POINT('Ctrl Pts',(183.291499121249,3.77547238952982,127.652378495409));
#204161=CARTESIAN_POINT('Ctrl Pts',(183.284008785487,3.69099925067666,127.551195813834));
#204162=CARTESIAN_POINT('Ctrl Pts',(183.276518449725,3.60256372176028,127.453540643053));
#204163=CARTESIAN_POINT('Ctrl Pts',(183.269028113963,3.51050501529534,127.359721652437));
#204164=CARTESIAN_POINT('Ctrl Pts',(183.261253779844,3.41495587499346,127.262345486275));
#204165=CARTESIAN_POINT('Ctrl Pts',(183.253479445725,3.31520071706981,127.168793681802));
#204166=CARTESIAN_POINT('Ctrl Pts',(183.245705111606,3.21157817053554,127.079451394908));
#204167=CARTESIAN_POINT('Ctrl Pts',(183.237940358659,3.10808332952903,126.990219214398));
#204168=CARTESIAN_POINT('Ctrl Pts',(183.230175605712,3.00073087651156,126.905186482029));
#204169=CARTESIAN_POINT('Ctrl Pts',(183.222410852765,2.88989742139538,126.824702848824));
#204170=CARTESIAN_POINT('Ctrl Pts',(183.21465381188,2.77917404762878,126.744299153096));
#204171=CARTESIAN_POINT('Ctrl Pts',(183.206896770995,2.66497686641319,126.668435793291));
#204172=CARTESIAN_POINT('Ctrl Pts',(183.19913973011,2.54771654736785,126.597423078599));
#204173=CARTESIAN_POINT('Ctrl Pts',(183.19138853887,2.43054465524129,126.526463915148));
#204174=CARTESIAN_POINT('Ctrl Pts',(183.18363734763,2.31031455614051,126.460348317669));
#204175=CARTESIAN_POINT('Ctrl Pts',(183.175886156389,2.18746666821171,126.3993438596));
#204176=CARTESIAN_POINT('Ctrl Pts',(183.168138259612,2.0646709939127,126.338365330053));
#204177=CARTESIAN_POINT('Ctrl Pts',(183.160390362835,1.93926009315588,126.282493792761));
#204178=CARTESIAN_POINT('Ctrl Pts',(183.152642466058,1.811699608605,126.231951231839));
#204179=CARTESIAN_POINT('Ctrl Pts',(183.144896189974,1.68416580695755,126.181419243332));
#204180=CARTESIAN_POINT('Ctrl Pts',(183.13714991389,1.55448367913088,126.136214157909));
#204181=CARTESIAN_POINT('Ctrl Pts',(183.129403637806,1.42313913406825,126.096509933062));
#204182=CARTESIAN_POINT('Ctrl Pts',(183.121657304541,1.29179361945,126.056805415127));
#204183=CARTESIAN_POINT('Ctrl Pts',(183.113910971275,1.15878603734873,126.022601951924));
#204184=CARTESIAN_POINT('Ctrl Pts',(183.10616463801,1.02461736894711,125.994023590938));
#204185=CARTESIAN_POINT('Ctrl Pts',(183.098416570007,0.890418654402585,
125.965438830026));
#204186=CARTESIAN_POINT('Ctrl Pts',(183.090668502004,0.755058718467256,
125.942481759427));
#204187=CARTESIAN_POINT('Ctrl Pts',(183.082920434001,0.619048246319054,
125.925225209399));
#204188=CARTESIAN_POINT('Ctrl Pts',(183.075164131259,0.482893220622485,
125.907950318904));
#204189=CARTESIAN_POINT('Ctrl Pts',(183.067407828517,0.346086666046123,
125.896388100937));
#204190=CARTESIAN_POINT('Ctrl Pts',(183.059651525776,0.209144455485154,
125.890559475961));
#204191=CARTESIAN_POINT('Ctrl Pts',(183.051891083261,0.0721291547430187,
125.884727740072));
#204192=CARTESIAN_POINT('Ctrl Pts',(183.044130640747,-0.065021555480375,
125.884635695128));
#204193=CARTESIAN_POINT('Ctrl Pts',(183.036370198233,-0.201793294674736,
125.890252099358));
#204194=CARTESIAN_POINT('Ctrl Pts',(183.028597297968,-0.338784592006899,
125.895877519539));
#204195=CARTESIAN_POINT('Ctrl Pts',(183.020824397702,-0.475395312770501,
125.907229668511));
#204196=CARTESIAN_POINT('Ctrl Pts',(183.013051497437,-0.611116780560397,
125.92422544085));
#204197=CARTESIAN_POINT('Ctrl Pts',(183.005561161675,-0.74190443113344,
125.940603374055));
#204198=CARTESIAN_POINT('Ctrl Pts',(182.998070825913,-0.87186605558637,
125.96222168399));
#204199=CARTESIAN_POINT('Ctrl Pts',(182.990580490151,-1.00055860898726,
125.988961824892));
#204200=CARTESIAN_POINT('Ctrl Pts',(182.982806156032,-1.13413057966649,
126.016715826365));
#204201=CARTESIAN_POINT('Ctrl Pts',(182.975031821913,-1.26675846180681,
126.050075630492));
#204202=CARTESIAN_POINT('Ctrl Pts',(182.967257487794,-1.39793517559902,
126.088964525261));
#204203=CARTESIAN_POINT('Ctrl Pts',(182.959492734846,-1.52895022581513,
126.127805492943));
#204204=CARTESIAN_POINT('Ctrl Pts',(182.951727981899,-1.65851729489495,
126.172161883161));
#204205=CARTESIAN_POINT('Ctrl Pts',(182.943963228952,-1.78613864467428,
126.221905838247));
#204206=CARTESIAN_POINT('Ctrl Pts',(182.936206188067,-1.91363323913031,
126.271600386936));
#204207=CARTESIAN_POINT('Ctrl Pts',(182.928449147182,-2.03918559816484,
126.326671710685));
#204208=CARTESIAN_POINT('Ctrl Pts',(182.920692106297,-2.16231267290643,
126.386942031209));
#204209=CARTESIAN_POINT('Ctrl Pts',(182.912940915057,-2.28534689656263,
126.447166901416));
#204210=CARTESIAN_POINT('Ctrl Pts',(182.905189723817,-2.40595912655983,
126.512582793482));
#204211=CARTESIAN_POINT('Ctrl Pts',(182.897438532577,-2.52368618902095,
126.582963801127));
#204212=CARTESIAN_POINT('Ctrl Pts',(182.8896906358,-2.64136321434017,126.653314894965));
#204213=CARTESIAN_POINT('Ctrl Pts',(182.881942739023,-2.75615717621927,
126.728626706948));
#204214=CARTESIAN_POINT('Ctrl Pts',(182.874194842245,-2.86762962189981,
126.808627466553));
#204215=CARTESIAN_POINT('Ctrl Pts',(182.866448566161,-2.97907874994782,
126.888611491724));
#204216=CARTESIAN_POINT('Ctrl Pts',(182.858702290077,-3.08720742634127,
126.973282285786));
#204217=CARTESIAN_POINT('Ctrl Pts',(182.850956013993,-3.1916066500627,127.062325068059));
#204218=CARTESIAN_POINT('Ctrl Pts',(182.843209680728,-3.29600664443559,
127.151368507625));
#204219=CARTESIAN_POINT('Ctrl Pts',(182.835463347462,-3.39667683373769,
127.24478374609));
#204220=CARTESIAN_POINT('Ctrl Pts',(182.827717014197,-3.49324206073987,
127.342216344492));
#204221=CARTESIAN_POINT('Ctrl Pts',(182.819968946194,-3.58982891285543,
127.43967076225));
#204222=CARTESIAN_POINT('Ctrl Pts',(182.812220878191,-3.68230869825185,
127.541144052529));
#204223=CARTESIAN_POINT('Ctrl Pts',(182.804472810188,-3.77034410495834,
127.64624592796));
#204224=CARTESIAN_POINT('Ctrl Pts',(182.796716507446,-3.85847307674226,
127.751459506914));
#204225=CARTESIAN_POINT('Ctrl Pts',(182.788960204704,-3.94214798261169,
127.860309074608));
#204226=CARTESIAN_POINT('Ctrl Pts',(182.781203901962,-4.02107237968682,
127.972371920586));
#204227=CARTESIAN_POINT('Ctrl Pts',(182.773443459448,-4.10003890108901,
128.08449457788));
#204228=CARTESIAN_POINT('Ctrl Pts',(182.765683016934,-4.17424965007582,
128.19983360216));
#204229=CARTESIAN_POINT('Ctrl Pts',(182.75792257442,-4.24345287600184,128.317939343596));
#204230=CARTESIAN_POINT('Ctrl Pts',(182.750149674154,-4.31276719308979,
128.436234678853));
#204231=CARTESIAN_POINT('Ctrl Pts',(182.742376773889,-4.37705774012523,
128.557305261059));
#204232=CARTESIAN_POINT('Ctrl Pts',(182.734603873624,-4.43611948403242,
128.680678205837));
#204233=CARTESIAN_POINT('Ctrl Pts',(182.727113537862,-4.49303418478051,
128.799566233313));
#204234=CARTESIAN_POINT('Ctrl Pts',(182.7196232021,-4.54509352087592,128.920591853246));
#204235=CARTESIAN_POINT('Ctrl Pts',(182.712132866338,-4.59215775161795,
129.043318242507));
#204236=CARTESIAN_POINT('Ctrl Pts',(182.703253522123,-4.64794957700628,
129.188803023033));
#204237=CARTESIAN_POINT('Ctrl Pts',(182.694374177909,-4.69687000701748,
129.337061417581));
#204238=CARTESIAN_POINT('Ctrl Pts',(182.685494833695,-4.73867041310273,
129.487475740865));
#204239=CARTESIAN_POINT('Ctrl Pts',(182.683630675656,-4.74744612459306,
129.519054206932));
#204240=CARTESIAN_POINT('Ctrl Pts',(182.681766517617,-4.75590817585868,
129.550727615035));
#204241=CARTESIAN_POINT('Ctrl Pts',(182.679902359578,-4.76405452823405,
129.582490119308));
#204242=CARTESIAN_POINT('Ctrl Pts',(184.430229652623,-4.76405452823406,
129.582490119308));
#204243=CARTESIAN_POINT('Ctrl Pts',(184.422327812055,-4.7986868585295,129.717521049511));
#204244=CARTESIAN_POINT('Ctrl Pts',(184.414425971487,-4.82753715525285,
129.853882584735));
#204245=CARTESIAN_POINT('Ctrl Pts',(184.406524130919,-4.85053490297993,
129.991037669732));
#204246=CARTESIAN_POINT('Ctrl Pts',(184.398622290351,-4.873532650707,130.128192754729));
#204247=CARTESIAN_POINT('Ctrl Pts',(184.390720449783,-4.89067785997628,
130.266140963835));
#204248=CARTESIAN_POINT('Ctrl Pts',(184.382818609216,-4.90195570679255,
130.404343978982));
#204249=CARTESIAN_POINT('Ctrl Pts',(184.375259260813,-4.91274473405513,
130.536556813798));
#204250=CARTESIAN_POINT('Ctrl Pts',(184.367699912411,-4.91818571452675,
130.669211977639));
#204251=CARTESIAN_POINT('Ctrl Pts',(184.360140564008,-4.91824943376062,
130.802000572364));
#204252=CARTESIAN_POINT('Origin',(213.235140564004,0.,130.804360617566));
#204253=CARTESIAN_POINT('',(186.18020938313,-4.76405452823405,129.582490119308));
#204254=CARTESIAN_POINT('',(185.834939443695,-4.76405452823405,129.582490119308));
#204255=CARTESIAN_POINT('',(213.235140564004,-4.76405452823405,129.582490119308));
#204256=CARTESIAN_POINT('',(185.764859435953,-4.91824909926408,130.801384027568));
#204257=CARTESIAN_POINT('Ctrl Pts',(185.834939443695,-4.76405452823405,
129.582490119308));
#204258=CARTESIAN_POINT('Ctrl Pts',(185.82716587756,-4.79810227029313,129.71524174885));
#204259=CARTESIAN_POINT('Ctrl Pts',(185.819392311426,-4.82655888961819,
129.849268541578));
#204260=CARTESIAN_POINT('Ctrl Pts',(185.811618745292,-4.84935969226982,
129.984059674321));
#204261=CARTESIAN_POINT('Ctrl Pts',(185.805961071674,-4.8659543281669,130.082161912396));
#204262=CARTESIAN_POINT('Ctrl Pts',(185.800303398056,-4.87955412703471,
130.180668865511));
#204263=CARTESIAN_POINT('Ctrl Pts',(185.794645724439,-4.8901515047038,130.279383167057));
#204264=CARTESIAN_POINT('Ctrl Pts',(185.784716961623,-4.90874905140923,
130.45261883826));
#204265=CARTESIAN_POINT('Ctrl Pts',(185.774788198807,-4.91814347496568,
130.626859993452));
#204266=CARTESIAN_POINT('Ctrl Pts',(185.764859435991,-4.91824909926368,
130.801384026903));
#204267=CARTESIAN_POINT('Ctrl Pts',(185.764859435953,-4.91824909926409,
130.801384027568));
#204268=CARTESIAN_POINT('Ctrl Pts',(185.757191235898,-4.9183306751947,130.936172744721));
#204269=CARTESIAN_POINT('Ctrl Pts',(185.749523035843,-4.91286708241096,
131.071183771682));
#204270=CARTESIAN_POINT('Ctrl Pts',(185.741854835789,-4.901829924088,131.205915667111));
#204271=CARTESIAN_POINT('Ctrl Pts',(185.734195115826,-4.89080497151269,
131.340498565537));
#204272=CARTESIAN_POINT('Ctrl Pts',(185.726535395862,-4.87421874451201,
131.474802549089));
#204273=CARTESIAN_POINT('Ctrl Pts',(185.718875675899,-4.85209485286721,
131.608324921052));
#204274=CARTESIAN_POINT('Ctrl Pts',(185.711222480037,-4.82998980505673,
131.741733566484));
#204275=CARTESIAN_POINT('Ctrl Pts',(185.703569284174,-4.80235654064527,
131.874361530089));
#204276=CARTESIAN_POINT('Ctrl Pts',(185.695916088312,-4.76927054522506,
132.00571049539));
#204277=CARTESIAN_POINT('Ctrl Pts',(185.688267001704,-4.73620231477376,
132.136988935073));
#204278=CARTESIAN_POINT('Ctrl Pts',(185.680617915096,-4.69768727340913,
132.266989353296));
#204279=CARTESIAN_POINT('Ctrl Pts',(185.672968828489,-4.65385205465889,
132.395223313039));
#204280=CARTESIAN_POINT('Ctrl Pts',(185.665321809995,-4.61002868781017,
132.523422601658));
#204281=CARTESIAN_POINT('Ctrl Pts',(185.657674791501,-4.56088813315632,
132.649856001177));
#204282=CARTESIAN_POINT('Ctrl Pts',(185.650027773007,-4.50660683515309,
132.774050414425));
#204283=CARTESIAN_POINT('Ctrl Pts',(185.642381064432,-4.4523277370657,132.898239794315));
#204284=CARTESIAN_POINT('Ctrl Pts',(185.634734355857,-4.39290847102935,
133.020189999991));
#204285=CARTESIAN_POINT('Ctrl Pts',(185.627087647282,-4.3285733387234,133.139448606014));
#204286=CARTESIAN_POINT('Ctrl Pts',(185.619439490905,-4.26422602542105,
133.258729792058));
#204287=CARTESIAN_POINT('Ctrl Pts',(185.611791334528,-4.19496118620005,
133.37531801141));
#204288=CARTESIAN_POINT('Ctrl Pts',(185.604143178151,-4.12104844176228,
133.488786590311));
#204289=CARTESIAN_POINT('Ctrl Pts',(185.596487235631,-4.04706045105567,
133.602370684977));
#204290=CARTESIAN_POINT('Ctrl Pts',(185.58883129311,-3.96841532550673,133.71282845947));
#204291=CARTESIAN_POINT('Ctrl Pts',(185.58117535059,-3.88542548694373,133.819763053048));
#204292=CARTESIAN_POINT('Ctrl Pts',(185.573515374056,-3.80239191997511,
133.926753991828));
#204293=CARTESIAN_POINT('Ctrl Pts',(185.565855397521,-3.71500934088863,
134.03021774658));
#204294=CARTESIAN_POINT('Ctrl Pts',(185.558195420987,-3.62362875719401,
134.129792573348));
#204295=CARTESIAN_POINT('Ctrl Pts',(185.550523572136,-3.5321065413066,134.229521732694));
#204296=CARTESIAN_POINT('Ctrl Pts',(185.542851723284,-3.43657422762343,
134.325349640552));
#204297=CARTESIAN_POINT('Ctrl Pts',(185.535179874433,-3.33741822988249,
134.416952847717));
#204298=CARTESIAN_POINT('Ctrl Pts',(185.528852616497,-3.25564060551483,
134.492501405919));
#204299=CARTESIAN_POINT('Ctrl Pts',(185.522525358561,-3.17139888835135,
134.56517703643));
#204300=CARTESIAN_POINT('Ctrl Pts',(185.516198100626,-3.08492473413098,
134.634820439473));
#204301=CARTESIAN_POINT('Ctrl Pts',(185.508423766507,-2.97867349948799,
134.720391644243));
#204302=CARTESIAN_POINT('Ctrl Pts',(185.500649432388,-2.86869084610792,
134.801674161477));
#204303=CARTESIAN_POINT('Ctrl Pts',(185.492875098269,-2.75535800148616,
134.878324945606));
#204304=CARTESIAN_POINT('Ctrl Pts',(185.485110345321,-2.64216482946666,
134.954881264495));
#204305=CARTESIAN_POINT('Ctrl Pts',(185.477345592374,-2.52563000205102,
135.026816990961));
#204306=CARTESIAN_POINT('Ctrl Pts',(185.469580839427,-2.4061683288018,135.093828770609));
#204307=CARTESIAN_POINT('Ctrl Pts',(185.461823798542,-2.28682530657056,
135.160773993213));
#204308=CARTESIAN_POINT('Ctrl Pts',(185.454066757657,-2.16456156231129,
135.222804811345));
#204309=CARTESIAN_POINT('Ctrl Pts',(185.446309716772,-2.03982114582494,
135.279660915372));
#204310=CARTESIAN_POINT('Ctrl Pts',(185.438558525532,-1.91517479705691,
135.33647414377));
#204311=CARTESIAN_POINT('Ctrl Pts',(185.430807334292,-1.78805584787562,
135.388120263844));
#204312=CARTESIAN_POINT('Ctrl Pts',(185.423056143052,-1.65893291082312,
135.434384878829));
#204313=CARTESIAN_POINT('Ctrl Pts',(185.415308246275,-1.52986485446345,
135.480629830119));
#204314=CARTESIAN_POINT('Ctrl Pts',(185.407560349498,-1.39879487157781,
135.521497693954));
#204315=CARTESIAN_POINT('Ctrl Pts',(185.399812452721,-1.2662113115785,135.556822293049));
#204316=CARTESIAN_POINT('Ctrl Pts',(185.392066176637,-1.13365548520171,
135.592139502999));
#204317=CARTESIAN_POINT('Ctrl Pts',(185.384319900553,-0.999587089008202,
135.62191565399));
#204318=CARTESIAN_POINT('Ctrl Pts',(185.376573624468,-0.864509000677892,
135.646034630782));
#204319=CARTESIAN_POINT('Ctrl Pts',(185.368827291203,-0.729429915231751,
135.670153785614));
#204320=CARTESIAN_POINT('Ctrl Pts',(185.361080957938,-0.593341507654216,
135.688615614195));
#204321=CARTESIAN_POINT('Ctrl Pts',(185.353334624672,-0.456755805682509,
135.701355328251));
#204322=CARTESIAN_POINT('Ctrl Pts',(185.345586556669,-0.320139516289562,
135.714097895278));
#204323=CARTESIAN_POINT('Ctrl Pts',(185.337838488666,-0.183026100098795,
135.721115761585));
#204324=CARTESIAN_POINT('Ctrl Pts',(185.330090420663,-0.0459312508572161,
135.722396138248));
#204325=CARTESIAN_POINT('Ctrl Pts',(185.322334117922,0.0913093044211189,
135.723677875712));
#204326=CARTESIAN_POINT('Ctrl Pts',(185.31457781518,0.228530861759579,135.719209938718));
#204327=CARTESIAN_POINT('Ctrl Pts',(185.306821512438,0.365218627626155,
135.709031698947));
#204328=CARTESIAN_POINT('Ctrl Pts',(185.299061069924,0.501979347869056,
135.698848026743));
#204329=CARTESIAN_POINT('Ctrl Pts',(185.29130062741,0.638205320812515,135.682948024144));
#204330=CARTESIAN_POINT('Ctrl Pts',(185.283540184895,0.773389317112324,
135.661422695271));
#204331=CARTESIAN_POINT('Ctrl Pts',(185.27576728463,0.908790322764111,135.639862812028));
#204332=CARTESIAN_POINT('Ctrl Pts',(185.267994384365,1.04314562582757,135.612659634777));
#204333=CARTESIAN_POINT('Ctrl Pts',(185.260221484099,1.175959709326,135.57995501246));
#204334=CARTESIAN_POINT('Ctrl Pts',(185.252731148337,1.30394566635063,135.548439285542));
#204335=CARTESIAN_POINT('Ctrl Pts',(185.245240812575,1.43050021692963,135.511815237666));
#204336=CARTESIAN_POINT('Ctrl Pts',(185.237750476813,1.55519716015653,135.470252263923));
#204337=CARTESIAN_POINT('Ctrl Pts',(185.229976142694,1.68462202588672,135.427113417397));
#204338=CARTESIAN_POINT('Ctrl Pts',(185.222201808575,1.81245562030366,135.378517082239));
#204339=CARTESIAN_POINT('Ctrl Pts',(185.214427474456,1.93820326668134,135.324598571427));
#204340=CARTESIAN_POINT('Ctrl Pts',(185.206662721509,2.06379594032369,135.270746510361));
#204341=CARTESIAN_POINT('Ctrl Pts',(185.198897968562,2.18730742506553,135.211585476901));
#204342=CARTESIAN_POINT('Ctrl Pts',(185.191133215614,2.30825828556062,135.147300491619));
#204343=CARTESIAN_POINT('Ctrl Pts',(185.183376174729,2.42908901595603,135.083079355091));
#204344=CARTESIAN_POINT('Ctrl Pts',(185.175619133844,2.54736384028493,135.013744576743));
#204345=CARTESIAN_POINT('Ctrl Pts',(185.167862092959,2.66262373291742,134.939529044535));
#204346=CARTESIAN_POINT('Ctrl Pts',(185.160110901719,2.77779670716764,134.865369478838));
#204347=CARTESIAN_POINT('Ctrl Pts',(185.152359710479,2.8899589477656,134.786336696123));
#204348=CARTESIAN_POINT('Ctrl Pts',(185.144608519239,2.99867678011411,134.702709066705));
#204349=CARTESIAN_POINT('Ctrl Pts',(185.136860622462,3.107348404484,134.61911698126));
#204350=CARTESIAN_POINT('Ctrl Pts',(185.129112725685,3.21257822307831,134.530934171219));
#204351=CARTESIAN_POINT('Ctrl Pts',(185.121364828908,3.31396246145469,134.438481675892));
#204352=CARTESIAN_POINT('Ctrl Pts',(185.113618552824,3.41532549243393,134.346048519634));
#204353=CARTESIAN_POINT('Ctrl Pts',(185.10587227674,3.51284425451252,134.249347717836));
#204354=CARTESIAN_POINT('Ctrl Pts',(185.098126000655,3.60614923898019,134.148739592608));
#204355=CARTESIAN_POINT('Ctrl Pts',(185.09037966739,3.69945491220408,134.048130724714));
#204356=CARTESIAN_POINT('Ctrl Pts',(185.082633334125,3.78854647989511,133.943614762498));
#204357=CARTESIAN_POINT('Ctrl Pts',(185.074887000859,3.87309267034491,133.835587469753));
#204358=CARTESIAN_POINT('Ctrl Pts',(185.067138932856,3.95765779432756,133.727535985046));
#204359=CARTESIAN_POINT('Ctrl Pts',(185.059390864854,4.03767527464004,133.615971912911));
#204360=CARTESIAN_POINT('Ctrl Pts',(185.051642796851,4.11285560653182,133.501322208379));
#204361=CARTESIAN_POINT('Ctrl Pts',(185.043886494109,4.18811584097532,133.386550652776));
#204362=CARTESIAN_POINT('Ctrl Pts',(185.036130191367,4.2585284426082,133.268687241189));
#204363=CARTESIAN_POINT('Ctrl Pts',(185.028373888625,4.32384827746161,133.148186365354));
#204364=CARTESIAN_POINT('Ctrl Pts',(185.020613446111,4.38920297547765,133.027621174572));
#204365=CARTESIAN_POINT('Ctrl Pts',(185.012853003597,4.44945931886022,132.904416065631));
#204366=CARTESIAN_POINT('Ctrl Pts',(185.005092561082,4.50441970210254,132.779046974892));
#204367=CARTESIAN_POINT('Ctrl Pts',(184.997319660817,4.55946831263118,132.65347663056));
#204368=CARTESIAN_POINT('Ctrl Pts',(184.989546760552,4.6092038322925,132.525735727174));
#204369=CARTESIAN_POINT('Ctrl Pts',(184.981773860286,4.65347776358927,132.396317830019));
#204370=CARTESIAN_POINT('Ctrl Pts',(184.974283524524,4.69614222596426,132.271604599409));
#204371=CARTESIAN_POINT('Ctrl Pts',(184.966793188762,4.7337352030942,132.145334479326));
#204372=CARTESIAN_POINT('Ctrl Pts',(184.959302853,4.7661688398658,132.017957606847));
#204373=CARTESIAN_POINT('Ctrl Pts',(184.951528518881,4.79983220783342,131.885751201534));
#204374=CARTESIAN_POINT('Ctrl Pts',(184.943754184762,4.8280439150364,131.751933671931));
#204375=CARTESIAN_POINT('Ctrl Pts',(184.935979850643,4.85065041926304,131.616994343548));
#204376=CARTESIAN_POINT('Ctrl Pts',(184.928215097696,4.87322906299363,131.482221315828));
#204377=CARTESIAN_POINT('Ctrl Pts',(184.920450344748,4.8902161844549,131.346329622014));
#204378=CARTESIAN_POINT('Ctrl Pts',(184.912685591801,4.90150830017843,131.209822632781));
#204379=CARTESIAN_POINT('Ctrl Pts',(184.904928550916,4.91278920041345,131.073451224213));
#204380=CARTESIAN_POINT('Ctrl Pts',(184.897171510031,4.91838631929962,130.936466123495));
#204381=CARTESIAN_POINT('Ctrl Pts',(184.889414469146,4.91824747750727,130.799379403521));
#204382=CARTESIAN_POINT('Ctrl Pts',(184.881663277906,4.9181087404166,130.662396061707));
#204383=CARTESIAN_POINT('Ctrl Pts',(184.873912086666,4.91224265275202,130.525311642551));
#204384=CARTESIAN_POINT('Ctrl Pts',(184.866160895426,4.9006490036298,130.388641474728));
#204385=CARTESIAN_POINT('Ctrl Pts',(184.858412998649,4.88906028211778,130.252029395372));
#204386=CARTESIAN_POINT('Ctrl Pts',(184.850665101872,4.87174887389483,130.115831605913));
#204387=CARTESIAN_POINT('Ctrl Pts',(184.842917205095,4.84876662847558,129.980561342814));
#204388=CARTESIAN_POINT('Ctrl Pts',(184.835170929011,4.82578919044663,129.845319375338));
#204389=CARTESIAN_POINT('Ctrl Pts',(184.827424652926,4.7971433401164,129.711004933506));
#204390=CARTESIAN_POINT('Ctrl Pts',(184.819678376842,4.76293249819749,129.578123658363));
#204391=CARTESIAN_POINT('Ctrl Pts',(184.811932043577,4.72872140374189,129.445241402321));
#204392=CARTESIAN_POINT('Ctrl Pts',(184.804185710312,4.68894533320337,129.313792712696));
#204393=CARTESIAN_POINT('Ctrl Pts',(184.796439377046,4.64375819341888,129.184270217756));
#204394=CARTESIAN_POINT('Ctrl Pts',(184.788691309043,4.59856093428778,129.054718717152));
#204395=CARTESIAN_POINT('Ctrl Pts',(184.78094324104,4.54795032338664,128.927094638659));
#204396=CARTESIAN_POINT('Ctrl Pts',(184.773195173037,4.49212908568403,128.801872330446));
#204397=CARTESIAN_POINT('Ctrl Pts',(184.765438870295,4.43624852050568,128.676516934474));
#204398=CARTESIAN_POINT('Ctrl Pts',(184.757682567554,4.37514642537891,128.553568765596));
#204399=CARTESIAN_POINT('Ctrl Pts',(184.749926264812,4.30907259203993,128.433479671793));
#204400=CARTESIAN_POINT('Ctrl Pts',(184.742165822298,4.24296349310673,128.313326482825));
#204401=CARTESIAN_POINT('Ctrl Pts',(184.734405379783,4.17187757104574,128.196035743754));
#204402=CARTESIAN_POINT('Ctrl Pts',(184.726644937269,4.09610843399477,128.08203096092));
#204403=CARTESIAN_POINT('Ctrl Pts',(184.718872037004,4.02021766559842,127.967843167486));
#204404=CARTESIAN_POINT('Ctrl Pts',(184.711099136738,3.93962888900392,127.856952187687));
#204405=CARTESIAN_POINT('Ctrl Pts',(184.703326236473,3.85467708813893,127.749749740764));
#204406=CARTESIAN_POINT('Ctrl Pts',(184.695835900711,3.77281349921669,127.646444372814));
#204407=CARTESIAN_POINT('Ctrl Pts',(184.688345564949,3.68689879343445,127.546564252244));
#204408=CARTESIAN_POINT('Ctrl Pts',(184.680855229187,3.59726419602927,127.450426604133));
#204409=CARTESIAN_POINT('Ctrl Pts',(184.673080895068,3.50423107561896,127.350643867872));
#204410=CARTESIAN_POINT('Ctrl Pts',(184.665306560949,3.4068957149069,127.25457691618));
#204411=CARTESIAN_POINT('Ctrl Pts',(184.65753222683,3.30558680398728,127.162619420857));
#204412=CARTESIAN_POINT('Ctrl Pts',(184.649767473883,3.20440274724626,127.070775254929));
#204413=CARTESIAN_POINT('Ctrl Pts',(184.642002720936,3.09925517067157,126.983030728698));
#204414=CARTESIAN_POINT('Ctrl Pts',(184.634237967988,2.99051163892463,126.899744989882));
#204415=CARTESIAN_POINT('Ctrl Pts',(184.626480927103,2.88187611278586,126.816541971634));
#204416=CARTESIAN_POINT('Ctrl Pts',(184.618723886218,2.7696520474073,126.737789164012));
#204417=CARTESIAN_POINT('Ctrl Pts',(184.610966845333,2.65424206001439,126.663807254868));
#204418=CARTESIAN_POINT('Ctrl Pts',(184.603215654093,2.53891910419166,126.589881136058));
#204419=CARTESIAN_POINT('Ctrl Pts',(184.595464462853,2.42041533625422,126.52071896472));
#204420=CARTESIAN_POINT('Ctrl Pts',(184.587713271613,2.29916420282371,126.456599466013));
#204421=CARTESIAN_POINT('Ctrl Pts',(184.579965374836,2.17796460435902,126.392507219803));
#204422=CARTESIAN_POINT('Ctrl Pts',(184.572217478059,2.0540203077666,126.333453565807));
#204423=CARTESIAN_POINT('Ctrl Pts',(184.564469581282,1.92779113934713,126.279672298405));
#204424=CARTESIAN_POINT('Ctrl Pts',(184.556723305198,1.80158837534844,126.225902280884));
#204425=CARTESIAN_POINT('Ctrl Pts',(184.548977029114,1.67310204963539,126.177402609436));
#204426=CARTESIAN_POINT('Ctrl Pts',(184.54123075303,1.54281347376092,126.134359584624));
#204427=CARTESIAN_POINT('Ctrl Pts',(184.533484419764,1.41252393612583,126.091316242077));
#204428=CARTESIAN_POINT('Ctrl Pts',(184.525738086499,1.28043249301377,126.053729749183));
#204429=CARTESIAN_POINT('Ctrl Pts',(184.517991753233,1.14703679694263,126.021736897372));
#204430=CARTESIAN_POINT('Ctrl Pts',(184.51024368523,1.01361122783021,125.989736880984));
#204431=CARTESIAN_POINT('Ctrl Pts',(184.502495617228,0.878881204667642,
125.963333089485));
#204432=CARTESIAN_POINT('Ctrl Pts',(184.494747549225,0.743355387800147,
125.94261136139));
#204433=CARTESIAN_POINT('Ctrl Pts',(184.486991246483,0.607685532481822,
125.921867609995));
#204434=CARTESIAN_POINT('Ctrl Pts',(184.479234943741,0.471218581013933,
125.906818044672));
#204435=CARTESIAN_POINT('Ctrl Pts',(184.471478640999,0.334469704435209,
125.897496743429));
#204436=CARTESIAN_POINT('Ctrl Pts',(184.463718198485,0.197647840863254,
125.888170467126));
#204437=CARTESIAN_POINT('Ctrl Pts',(184.455957755971,0.0605441429922865,
125.88457855716));
#204438=CARTESIAN_POINT('Ctrl Pts',(184.448197313456,-0.0763263789303934,
125.886702908211));
#204439=CARTESIAN_POINT('Ctrl Pts',(184.440424413191,-0.213416617565448,
125.888830669458));
#204440=CARTESIAN_POINT('Ctrl Pts',(184.432651512926,-0.350272541705855,
125.896693006356));
#204441=CARTESIAN_POINT('Ctrl Pts',(184.42487861266,-0.486383519863692,
125.910219821256));
#204442=CARTESIAN_POINT('Ctrl Pts',(184.417388276898,-0.617546521122763,
125.923254902363));
#204443=CARTESIAN_POINT('Ctrl Pts',(184.409897941136,-0.748017492370623,
125.941549732693));
#204444=CARTESIAN_POINT('Ctrl Pts',(184.402407605374,-0.877350507831442,
125.964997110977));
#204445=CARTESIAN_POINT('Ctrl Pts',(184.394633271255,-1.01158722388324,
125.989333503735));
#204446=CARTESIAN_POINT('Ctrl Pts',(184.386858937136,-1.14502321111271,
126.019297965427));
#204447=CARTESIAN_POINT('Ctrl Pts',(184.379084603017,-1.27714959725893,
126.054826748993));
#204448=CARTESIAN_POINT('Ctrl Pts',(184.37131985007,-1.40911314944234,126.090311746508));
#204449=CARTESIAN_POINT('Ctrl Pts',(184.363555097123,-1.53976993792535,
126.131347320907));
#204450=CARTESIAN_POINT('Ctrl Pts',(184.355790344176,-1.66861912388403,
126.177818357745));
#204451=CARTESIAN_POINT('Ctrl Pts',(184.348033303291,-1.79734033501496,
126.224243238894));
#204452=CARTESIAN_POINT('Ctrl Pts',(184.340276262406,-1.92425715102514,
126.276092707283));
#204453=CARTESIAN_POINT('Ctrl Pts',(184.332519221521,-2.04888214369525,
126.333201369256));
#204454=CARTESIAN_POINT('Ctrl Pts',(184.32476803028,-2.17341315568864,126.390266965143));
#204455=CARTESIAN_POINT('Ctrl Pts',(184.31701683904,-2.29565543039551,126.452583698322));
#204456=CARTESIAN_POINT('Ctrl Pts',(184.3092656478,-2.41514017995914,126.51993755563));
#204457=CARTESIAN_POINT('Ctrl Pts',(184.301517751023,-2.5345741453172,126.587262785753));
#204458=CARTESIAN_POINT('Ctrl Pts',(184.293769854246,-2.65125257672636,
126.659620690311));
#204459=CARTESIAN_POINT('Ctrl Pts',(184.286021957469,-2.76473022900649,
126.736750775986));
#204460=CARTESIAN_POINT('Ctrl Pts',(184.278275681385,-2.87818414420808,
126.81386472771));
#204461=CARTESIAN_POINT('Ctrl Pts',(184.270529405301,-2.98843828887982,
126.895748655367));
#204462=CARTESIAN_POINT('Ctrl Pts',(184.262783129217,-3.09507576243218,
126.982098317919));
#204463=CARTESIAN_POINT('Ctrl Pts',(184.255036795951,-3.20171402315806,
127.068448617884));
#204464=CARTESIAN_POINT('Ctrl Pts',(184.247290462686,-3.30473525564962,
127.159264472488));
#204465=CARTESIAN_POINT('Ctrl Pts',(184.239544129421,-3.40375538006029,
127.254201131682));
#204466=CARTESIAN_POINT('Ctrl Pts',(184.231796061418,-3.50279767934135,
127.349159051283));
#204467=CARTESIAN_POINT('Ctrl Pts',(184.224047993415,-3.59783680540671,
127.448239341269));
#204468=CARTESIAN_POINT('Ctrl Pts',(184.216299925412,-3.6885255965423,127.551060449098));
#204469=CARTESIAN_POINT('Ctrl Pts',(184.20854362267,-3.77931077280425,127.653990836424));
#204470=CARTESIAN_POINT('Ctrl Pts',(184.200787319928,-3.86573611899577,
127.760669689976));
#204471=CARTESIAN_POINT('Ctrl Pts',(184.193031017186,-3.94749450179272,
127.870682001764));
#204472=CARTESIAN_POINT('Ctrl Pts',(184.185270574672,-4.02929652150032,
127.980753030435));
#204473=CARTESIAN_POINT('Ctrl Pts',(184.177510132158,-4.10642639472572,
128.094160739358));
#204474=CARTESIAN_POINT('Ctrl Pts',(184.169749689644,-4.17862097836977,
128.210462049459));
#204475=CARTESIAN_POINT('Ctrl Pts',(184.161976789378,-4.25093145516856,
128.326950056747));
#204476=CARTESIAN_POINT('Ctrl Pts',(184.154203889113,-4.31829061835359,
128.446340606829));
#204477=CARTESIAN_POINT('Ctrl Pts',(184.146430988847,-4.38048143426836,
128.568166201481));
#204478=CARTESIAN_POINT('Ctrl Pts',(184.138940653085,-4.44041145737599,
128.685563128908));
#204479=CARTESIAN_POINT('Ctrl Pts',(184.131450317323,-4.49554224537381,
128.805220854819));
#204480=CARTESIAN_POINT('Ctrl Pts',(184.123959981561,-4.54572295595053,
128.926706264325));
#204481=CARTESIAN_POINT('Ctrl Pts',(184.115260747627,-4.60400255170544,
129.067798737404));
#204482=CARTESIAN_POINT('Ctrl Pts',(184.106561513693,-4.65576212734771,
129.211734291794));
#204483=CARTESIAN_POINT('Ctrl Pts',(184.097862279759,-4.70074664434197,
129.357929130005));
#204484=CARTESIAN_POINT('Ctrl Pts',(184.093441289351,-4.72360798128571,
129.432226014336));
#204485=CARTESIAN_POINT('Ctrl Pts',(184.089020298944,-4.74472023587179,
129.507106006827));
#204486=CARTESIAN_POINT('Ctrl Pts',(184.084599308536,-4.76405452823405,
129.582490119308));
#204487=CARTESIAN_POINT('',(186.110140564058,-4.91824801325411,130.808781321355));
#204488=CARTESIAN_POINT('Ctrl Pts',(186.110140564008,-4.91824801325332,
130.808781322232));
#204489=CARTESIAN_POINT('Ctrl Pts',(186.099074116598,-4.91807260824191,
131.003927891408));
#204490=CARTESIAN_POINT('Ctrl Pts',(186.088007669188,-4.90627932088814,
131.198573828951));
#204491=CARTESIAN_POINT('Ctrl Pts',(186.076941221778,-4.88306599966,131.391599500359));
#204492=CARTESIAN_POINT('Ctrl Pts',(186.069128931883,-4.86667869954997,
131.527864775596));
#204493=CARTESIAN_POINT('Ctrl Pts',(186.061316641987,-4.84460109965971,
131.663323468629));
#204494=CARTESIAN_POINT('Ctrl Pts',(186.053504352092,-4.81691589639799,
131.797589850688));
#204495=CARTESIAN_POINT('Ctrl Pts',(186.045730017973,-4.78936520086549,
131.931203903559));
#204496=CARTESIAN_POINT('Ctrl Pts',(186.037955683854,-4.75620727242799,
132.063882400062));
#204497=CARTESIAN_POINT('Ctrl Pts',(186.030181349735,-4.71751805131938,
132.195118144231));
#204498=CARTESIAN_POINT('Ctrl Pts',(186.022416596788,-4.67887651121803,
132.326192152075));
#204499=CARTESIAN_POINT('Ctrl Pts',(186.014651843841,-4.63471735138709,
132.455826573993));
#204500=CARTESIAN_POINT('Ctrl Pts',(186.006887090894,-4.58516767187299,
132.583523477821));
#204501=CARTESIAN_POINT('Ctrl Pts',(185.999130050009,-4.53566720579912,
132.711093551284));
#204502=CARTESIAN_POINT('Ctrl Pts',(185.991373009124,-4.48078701513992,
132.83672957411));
#204503=CARTESIAN_POINT('Ctrl Pts',(185.983615968239,-4.42070414285521,
132.95994822744));
#204504=CARTESIAN_POINT('Ctrl Pts',(185.975864776998,-4.36066657953178,
133.083073960625));
#204505=CARTESIAN_POINT('Ctrl Pts',(185.968113585758,-4.29543431449837,
133.203785602808));
#204506=CARTESIAN_POINT('Ctrl Pts',(185.960362394518,-4.22523254890233,
133.321619636856));
#204507=CARTESIAN_POINT('Ctrl Pts',(185.952614497741,-4.15506062092945,
133.439403588296));
#204508=CARTESIAN_POINT('Ctrl Pts',(185.944866600964,-4.07992359302457,
133.554312029003));
#204509=CARTESIAN_POINT('Ctrl Pts',(185.937118704187,-4.0000925681456,133.665906093138));
#204510=CARTESIAN_POINT('Ctrl Pts',(185.929372428103,-3.92027824219608,
133.7774768142));
#204511=CARTESIAN_POINT('Ctrl Pts',(185.921626152019,-3.83577209961954,
133.885734219918));
#204512=CARTESIAN_POINT('Ctrl Pts',(185.913879875934,-3.74688829830369,
133.990268830703));
#204513=CARTESIAN_POINT('Ctrl Pts',(185.906133542669,-3.65800384086778,
134.09480421314));
#204514=CARTESIAN_POINT('Ctrl Pts',(185.898387209404,-3.56474191346714,
134.195616447958));
#204515=CARTESIAN_POINT('Ctrl Pts',(185.890640876138,-3.4674563837275,134.292329838968));
#204516=CARTESIAN_POINT('Ctrl Pts',(185.882892808135,-3.37014906756808,
134.389064888271));
#204517=CARTESIAN_POINT('Ctrl Pts',(185.875144740132,-3.26881663328405,
134.481698991651));
#204518=CARTESIAN_POINT('Ctrl Pts',(185.867396672129,-3.16384885446265,
134.569894243576));
#204519=CARTESIAN_POINT('Ctrl Pts',(185.859640369388,-3.05876951463674,
134.658183230465));
#204520=CARTESIAN_POINT('Ctrl Pts',(185.851884066646,-2.95004741195152,
134.742023689953));
#204521=CARTESIAN_POINT('Ctrl Pts',(185.844127763904,-2.83810480523698,
134.82111853621));
#204522=CARTESIAN_POINT('Ctrl Pts',(185.83636732139,-2.72610245138265,134.900255597768));
#204523=CARTESIAN_POINT('Ctrl Pts',(185.828606878875,-2.6108764967903,134.974641787181));
#204524=CARTESIAN_POINT('Ctrl Pts',(185.820846436361,-2.49287620764804,
135.044024669804));
#204525=CARTESIAN_POINT('Ctrl Pts',(185.813073536096,-2.3746864939661,135.11351893199));
#204526=CARTESIAN_POINT('Ctrl Pts',(185.80530063583,-2.25371389122609,135.177993653395));
#204527=CARTESIAN_POINT('Ctrl Pts',(185.797527735565,-2.13043097123238,
135.237243081529));
#204528=CARTESIAN_POINT('Ctrl Pts',(185.790037399803,-2.01162969591266,
135.294338643711));
#204529=CARTESIAN_POINT('Ctrl Pts',(185.782547064041,-1.89068344157314,
135.346582099913));
#204530=CARTESIAN_POINT('Ctrl Pts',(185.775056728279,-1.76802881817535,
135.393833044828));
#204531=CARTESIAN_POINT('Ctrl Pts',(185.76728239416,-1.64072370745012,135.442875523682));
#204532=CARTESIAN_POINT('Ctrl Pts',(185.759508060041,-1.51117486044447,
135.486694787618));
#204533=CARTESIAN_POINT('Ctrl Pts',(185.751733725922,-1.37985004303931,
135.525080575499));
#204534=CARTESIAN_POINT('Ctrl Pts',(185.743968972975,-1.24868707173481,
135.563419056326));
#204535=CARTESIAN_POINT('Ctrl Pts',(185.736204220028,-1.11575285660129,
135.596337276052));
#204536=CARTESIAN_POINT('Ctrl Pts',(185.728439467081,-0.981535022751411,
135.623673023046));
#204537=CARTESIAN_POINT('Ctrl Pts',(185.720682426196,-0.847450495946294,
135.650981619791));
#204538=CARTESIAN_POINT('Ctrl Pts',(185.712925385311,-0.712085268171024,
135.672718700269));
#204539=CARTESIAN_POINT('Ctrl Pts',(185.705168344426,-0.575941665315386,
135.688771970089));
#204540=CARTESIAN_POINT('Ctrl Pts',(185.697417153186,-0.439900729409612,
135.704813134013));
#204541=CARTESIAN_POINT('Ctrl Pts',(185.689665961946,-0.303082973473198,
135.715178973112));
#204542=CARTESIAN_POINT('Ctrl Pts',(185.681914770705,-0.166000094317469,
135.719808413158));
#204543=CARTESIAN_POINT('Ctrl Pts',(185.674166873928,-0.0289754790421877,
135.724435885568));
#204544=CARTESIAN_POINT('Ctrl Pts',(185.666418977151,0.108313645407252,
135.723331794998));
#204545=CARTESIAN_POINT('Ctrl Pts',(185.658671080374,0.245351511000205,
135.716487010336));
#204546=CARTESIAN_POINT('Ctrl Pts',(185.65092480429,0.382360711225824,135.709643657456));
#204547=CARTESIAN_POINT('Ctrl Pts',(185.643178528206,0.519118366904536,
135.697062018493));
#204548=CARTESIAN_POINT('Ctrl Pts',(185.635432252122,0.655110161251152,
135.678785069655));
#204549=CARTESIAN_POINT('Ctrl Pts',(185.627685918857,0.791102959458301,
135.660507985901));
#204550=CARTESIAN_POINT('Ctrl Pts',(185.619939585591,0.926329497570983,
135.636535560459));
#204551=CARTESIAN_POINT('Ctrl Pts',(185.612193252326,1.06028241764848,135.606962439217));
#204552=CARTESIAN_POINT('Ctrl Pts',(185.604445184323,1.19426533555364,135.577382695279));
#204553=CARTESIAN_POINT('Ctrl Pts',(185.59669711632,1.32697368617402,135.542199844023));
#204554=CARTESIAN_POINT('Ctrl Pts',(185.588949048317,1.45791249787162,135.501559166813));
#204555=CARTESIAN_POINT('Ctrl Pts',(185.581192745575,1.58899047289653,135.460875296208));
#204556=CARTESIAN_POINT('Ctrl Pts',(185.573436442833,1.71829477813514,135.414722128319));
#204557=CARTESIAN_POINT('Ctrl Pts',(185.565680140092,1.84534722565303,135.363294339312));
#204558=CARTESIAN_POINT('Ctrl Pts',(185.557919697577,1.97246748488773,135.311839101746));
#204559=CARTESIAN_POINT('Ctrl Pts',(185.550159255063,2.09733313577467,135.25510379514));
#204560=CARTESIAN_POINT('Ctrl Pts',(185.542398812549,2.21948895854959,135.193329952772));
#204561=CARTESIAN_POINT('Ctrl Pts',(185.534625912284,2.34184087669565,135.131456945548));
#204562=CARTESIAN_POINT('Ctrl Pts',(185.526853012018,2.46147393253308,135.064529430542));
#204563=CARTESIAN_POINT('Ctrl Pts',(185.519080111753,2.57795958406316,134.992833781553));
#204564=CARTESIAN_POINT('Ctrl Pts',(185.511589775991,2.69021068875094,134.923744449994));
#204565=CARTESIAN_POINT('Ctrl Pts',(185.504099440229,2.79953899281448,134.850227805036));
#204566=CARTESIAN_POINT('Ctrl Pts',(185.496609104467,2.90559037094153,134.772575286506));
#204567=CARTESIAN_POINT('Ctrl Pts',(185.488834770348,3.01566271930338,134.691978549134));
#204568=CARTESIAN_POINT('Ctrl Pts',(185.481060436228,3.12255342329199,134.606670817637));
#204569=CARTESIAN_POINT('Ctrl Pts',(185.473286102109,3.22583274537233,134.516931985417));
#204570=CARTESIAN_POINT('Ctrl Pts',(185.465521349162,3.32898478491854,134.427303748286));
#204571=CARTESIAN_POINT('Ctrl Pts',(185.457756596215,3.42853400584439,134.333255530036));
#204572=CARTESIAN_POINT('Ctrl Pts',(185.449991843268,3.52408036162776,134.235109904134));
#204573=CARTESIAN_POINT('Ctrl Pts',(185.442234802383,3.61953181942352,134.137061757852));
#204574=CARTESIAN_POINT('Ctrl Pts',(185.434477761498,3.71098805294843,134.034924580939));
#204575=CARTESIAN_POINT('Ctrl Pts',(185.426720720613,3.79808306633545,133.92906029653));
#204576=CARTESIAN_POINT('Ctrl Pts',(185.418969529373,3.88511240069542,133.823275845201));
#204577=CARTESIAN_POINT('Ctrl Pts',(185.411218338133,3.96778681374832,133.713770181484));
#204578=CARTESIAN_POINT('Ctrl Pts',(185.403467146893,4.0457783373907,133.600940798287));
#204579=CARTESIAN_POINT('Ctrl Pts',(185.395719250116,4.12373671255506,133.488159370587));
#204580=CARTESIAN_POINT('Ctrl Pts',(185.387971353338,4.19701593512668,133.372057354035));
#204581=CARTESIAN_POINT('Ctrl Pts',(185.380223456561,4.2653295376257,133.253063743296));
#204582=CARTESIAN_POINT('Ctrl Pts',(185.372477180477,4.33362885039174,133.134095023454));
#204583=CARTESIAN_POINT('Ctrl Pts',(185.364730904393,4.39696441458693,133.01223625137));
#204584=CARTESIAN_POINT('Ctrl Pts',(185.356984628309,4.45509438652842,132.887943366012));
#204585=CARTESIAN_POINT('Ctrl Pts',(185.349238295044,4.51322478757213,132.763649563153));
#204586=CARTESIAN_POINT('Ctrl Pts',(185.341491961778,4.56614935405513,132.636921965314));
#204587=CARTESIAN_POINT('Ctrl Pts',(185.333745628513,4.61367347488339,132.508238585514));
#204588=CARTESIAN_POINT('Ctrl Pts',(185.32599756051,4.661208238409,132.379526387963));
#204589=CARTESIAN_POINT('Ctrl Pts',(185.318249492507,4.70334001430907,132.248857903597));
#204590=CARTESIAN_POINT('Ctrl Pts',(185.310501424504,4.73992348764949,132.116728094201));
#204591=CARTESIAN_POINT('Ctrl Pts',(185.302745121762,4.77654584234074,131.98445785567));
#204592=CARTESIAN_POINT('Ctrl Pts',(185.29498881902,4.80760801048513,131.850723566987));
#204593=CARTESIAN_POINT('Ctrl Pts',(185.287232516278,4.83301530639473,131.716032768426));
#204594=CARTESIAN_POINT('Ctrl Pts',(185.279472073764,4.85843616294317,131.581270081331));
#204595=CARTESIAN_POINT('Ctrl Pts',(185.27171163125,4.87819607698591,131.445550253803));
#204596=CARTESIAN_POINT('Ctrl Pts',(185.263951188736,4.8922521999072,131.30938682976));
#204597=CARTESIAN_POINT('Ctrl Pts',(185.25617828847,4.90633088696485,131.173004824101));
#204598=CARTESIAN_POINT('Ctrl Pts',(185.248405388205,4.91468746198499,131.036178189385));
#204599=CARTESIAN_POINT('Ctrl Pts',(185.24063248794,4.91733122193595,130.899422262165));
#204600=CARTESIAN_POINT('Ctrl Pts',(185.233142152178,4.91987887455347,130.767637757367));
#204601=CARTESIAN_POINT('Ctrl Pts',(185.225651816415,4.91712185788959,130.635919216476));
#204602=CARTESIAN_POINT('Ctrl Pts',(185.218161480653,4.90911395514333,130.504722105494));
#204603=CARTESIAN_POINT('Ctrl Pts',(185.210387146534,4.90080243033051,130.368550616171));
#204604=CARTESIAN_POINT('Ctrl Pts',(185.202612812415,4.8868076562378,130.232509526972));
#204605=CARTESIAN_POINT('Ctrl Pts',(185.194838478296,4.86713283147692,130.097111677475));
#204606=CARTESIAN_POINT('Ctrl Pts',(185.187073725349,4.84748225417918,129.961880693727));
#204607=CARTESIAN_POINT('Ctrl Pts',(185.179308972402,4.82216561011635,129.827291755562));
#204608=CARTESIAN_POINT('Ctrl Pts',(185.171544219455,4.79123805456728,129.693855792288));
#204609=CARTESIAN_POINT('Ctrl Pts',(185.16378717857,4.76034121670238,129.560552359494));
#204610=CARTESIAN_POINT('Ctrl Pts',(185.156030137685,4.72384464525298,129.428400001093));
#204611=CARTESIAN_POINT('Ctrl Pts',(185.1482730968,4.68185500669668,129.297902268069));
#204612=CARTESIAN_POINT('Ctrl Pts',(185.14052190556,4.63989703285347,129.167502944401));
#204613=CARTESIAN_POINT('Ctrl Pts',(185.13277071432,4.59245435629693,129.038756133175));
#204614=CARTESIAN_POINT('Ctrl Pts',(185.12501952308,4.53968412429643,128.912152617871));
#204615=CARTESIAN_POINT('Ctrl Pts',(185.117271626302,4.48693632105218,128.785602912438));
#204616=CARTESIAN_POINT('Ctrl Pts',(185.109523729525,4.42886561609171,128.661195051217));
#204617=CARTESIAN_POINT('Ctrl Pts',(185.101775832748,4.36567809210519,128.539401929507));
#204618=CARTESIAN_POINT('Ctrl Pts',(185.094029556664,4.30250378558652,128.417634284293));
#204619=CARTESIAN_POINT('Ctrl Pts',(185.08628328058,4.23421496891706,128.298480637502));
#204620=CARTESIAN_POINT('Ctrl Pts',(185.078537004496,4.16106451404611,128.182390905223));
#204621=CARTESIAN_POINT('Ctrl Pts',(185.070790671231,4.08791351919513,128.066300315995));
#204622=CARTESIAN_POINT('Ctrl Pts',(185.063044337965,4.00990102295931,127.953274017186));
#204623=CARTESIAN_POINT('Ctrl Pts',(185.0552980047,3.92732399917947,127.843734118332));
#204624=CARTESIAN_POINT('Ctrl Pts',(185.047549936697,3.84472848284773,127.734169688777));
#204625=CARTESIAN_POINT('Ctrl Pts',(185.039801868694,3.75756664022695,127.628093524923));
#204626=CARTESIAN_POINT('Ctrl Pts',(185.032053800691,3.66617635041229,127.525895423275));
#204627=CARTESIAN_POINT('Ctrl Pts',(185.024297497949,3.57468892991002,127.423588704268));
#204628=CARTESIAN_POINT('Ctrl Pts',(185.016541195207,3.47896434590667,127.325168572807));
#204629=CARTESIAN_POINT('Ctrl Pts',(185.008784892466,3.37937842648236,127.230989028559));
#204630=CARTESIAN_POINT('Ctrl Pts',(185.001024449951,3.27973935505435,127.136759217851));
#204631=CARTESIAN_POINT('Ctrl Pts',(184.993264007437,3.17623513657302,127.046774760618));
#204632=CARTESIAN_POINT('Ctrl Pts',(184.985503564923,3.06927466935573,126.961349289642));
#204633=CARTESIAN_POINT('Ctrl Pts',(184.977730664658,2.96214249970095,126.875786686117));
#204634=CARTESIAN_POINT('Ctrl Pts',(184.969957764392,2.85154330970152,126.794797924641));
#204635=CARTESIAN_POINT('Ctrl Pts',(184.962184864127,2.73791569183312,126.718653735408));
#204636=CARTESIAN_POINT('Ctrl Pts',(184.954694528365,2.62841872408481,126.645277579249));
#204637=CARTESIAN_POINT('Ctrl Pts',(184.947204192603,2.51610995032003,126.576400046695));
#204638=CARTESIAN_POINT('Ctrl Pts',(184.939713856841,2.40140163811663,126.512222078918));
#204639=CARTESIAN_POINT('Ctrl Pts',(184.931939522722,2.28234412539138,126.445610783985));
#204640=CARTESIAN_POINT('Ctrl Pts',(184.924165188603,2.16032438692566,126.383851452082));
#204641=CARTESIAN_POINT('Ctrl Pts',(184.916390854484,2.03577561811003,126.327218594444));
#204642=CARTESIAN_POINT('Ctrl Pts',(184.908626101536,1.91138034452076,126.270655531741));
#204643=CARTESIAN_POINT('Ctrl Pts',(184.900861348589,1.78446259457604,126.2192065328));
#204644=CARTESIAN_POINT('Ctrl Pts',(184.893096595642,1.65548204034892,126.173101363693));
#204645=CARTESIAN_POINT('Ctrl Pts',(184.885339554757,1.5266295914267,126.12704198689));
#204646=CARTESIAN_POINT('Ctrl Pts',(184.877582513872,1.3957187812083,126.086316008371));
#204647=CARTESIAN_POINT('Ctrl Pts',(184.869825472987,1.26323091723401,126.051105868213));
#204648=CARTESIAN_POINT('Ctrl Pts',(184.862074281747,1.13084296338832,126.015922280296));
#204649=CARTESIAN_POINT('Ctrl Pts',(184.854323090507,0.996880699273993,
125.986246351446));
#204650=CARTESIAN_POINT('Ctrl Pts',(184.846571899267,0.861841976869711,
125.962211149674));
#204651=CARTESIAN_POINT('Ctrl Pts',(184.83882400249,0.726860649524842,125.938186163504));
#204652=CARTESIAN_POINT('Ctrl Pts',(184.831076105713,0.590804157979271,
125.919797204415));
#204653=CARTESIAN_POINT('Ctrl Pts',(184.823328208936,0.454181755168668,
125.907126500662));
#204654=CARTESIAN_POINT('Ctrl Pts',(184.815581932852,0.317587930819519,
125.894458447347));
#204655=CARTESIAN_POINT('Ctrl Pts',(184.807835656767,0.180428819710515,
125.88750630627));
#204656=CARTESIAN_POINT('Ctrl Pts',(184.800089380683,0.0432196324551924,
125.886300519736));
#204657=CARTESIAN_POINT('Ctrl Pts',(184.792343047418,-0.0939905676472747,
125.8850947243));
#204658=CARTESIAN_POINT('Ctrl Pts',(184.784596714153,-0.231250453683563,
125.889635371485));
#204659=CARTESIAN_POINT('Ctrl Pts',(184.776850380887,-0.368044371329767,
125.899900769302));
#204660=CARTESIAN_POINT('Ctrl Pts',(184.769102312884,-0.504868923025204,
125.910168465984));
#204661=CARTESIAN_POINT('Ctrl Pts',(184.761354244881,-0.641226908890993,
125.926163435116));
#204662=CARTESIAN_POINT('Ctrl Pts',(184.753606176878,-0.77660775018482,
125.947812103976));
#204663=CARTESIAN_POINT('Ctrl Pts',(184.745849874136,-0.912132475847942,
125.969483781299));
#204664=CARTESIAN_POINT('Ctrl Pts',(184.738093571395,-1.04667759570581,
125.996821099783));
#204665=CARTESIAN_POINT('Ctrl Pts',(184.730337268653,-1.17974213555564,
126.029699210084));
#204666=CARTESIAN_POINT('Ctrl Pts',(184.722576826139,-1.312877695957,126.062594868424));
#204667=CARTESIAN_POINT('Ctrl Pts',(184.714816383624,-1.44453072664021,
126.101037101697));
#204668=CARTESIAN_POINT('Ctrl Pts',(184.70705594111,-1.57421633993268,126.144851418349));
#204669=CARTESIAN_POINT('Ctrl Pts',(184.699283040845,-1.70411013608448,
126.188736069632));
#204670=CARTESIAN_POINT('Ctrl Pts',(184.691510140579,-1.83202983856468,
126.238009896672));
#204671=CARTESIAN_POINT('Ctrl Pts',(184.683737240314,-1.95751060444897,
126.292450235481));
#204672=CARTESIAN_POINT('Ctrl Pts',(184.676246904552,-2.07842982842536,
126.344911530846));
#204673=CARTESIAN_POINT('Ctrl Pts',(184.66875656879,-2.19708408278854,126.402170094191));
#204674=CARTESIAN_POINT('Ctrl Pts',(184.661266233028,-2.31308146934551,
126.463987686737));
#204675=CARTESIAN_POINT('Ctrl Pts',(184.653490953882,-2.43349156701393,
126.528156911382));
#204676=CARTESIAN_POINT('Ctrl Pts',(184.645715674736,-2.55142012255629,
126.597442189508));
#204677=CARTESIAN_POINT('Ctrl Pts',(184.63794039559,-2.66640186075916,126.671627359849));
#204678=CARTESIAN_POINT('Ctrl Pts',(184.630174906103,-2.78123882835338,
126.745719125512));
#204679=CARTESIAN_POINT('Ctrl Pts',(184.622409416615,-2.89313603609128,
126.824698297011));
#204680=CARTESIAN_POINT('Ctrl Pts',(184.614643927127,-3.00165158969343,
126.908302250884));
#204681=CARTESIAN_POINT('Ctrl Pts',(184.606887744613,-3.11003708692624,
126.99180600505));
#204682=CARTESIAN_POINT('Ctrl Pts',(184.599131562098,-3.21504869422354,
127.079923265202));
#204683=CARTESIAN_POINT('Ctrl Pts',(184.591375379584,-3.31627290310998,
127.172347801702));
#204684=CARTESIAN_POINT('Ctrl Pts',(184.583624474521,-3.41742823714848,
127.264709450816));
#204685=CARTESIAN_POINT('Ctrl Pts',(184.575873569458,-3.51480101205282,
127.361372283403));
#204686=CARTESIAN_POINT('Ctrl Pts',(184.568122664396,-3.60801021796009,
127.461989403952));
#204687=CARTESIAN_POINT('Ctrl Pts',(184.560375354587,-3.70117618882434,
127.562559853301));
#204688=CARTESIAN_POINT('Ctrl Pts',(184.552628044778,-3.79018216867158,
127.66708065461));
#204689=CARTESIAN_POINT('Ctrl Pts',(184.544880734968,-3.87468379235378,
127.77516789148));
#204690=CARTESIAN_POINT('Ctrl Pts',(184.537135340988,-3.9591645196716,127.883228399511));
#204691=CARTESIAN_POINT('Ctrl Pts',(184.529389947007,-4.03914286792834,
127.994853279576));
#204692=CARTESIAN_POINT('Ctrl Pts',(184.521644553026,-4.11431484242556,
128.10962566958));
#204693=CARTESIAN_POINT('Ctrl Pts',(184.513896696704,-4.18951071487447,
128.22443454692));
#204694=CARTESIAN_POINT('Ctrl Pts',(184.506148840382,-4.25989694066962,
128.342392609911));
#204695=CARTESIAN_POINT('Ctrl Pts',(184.49840098406,-4.32521289149947,128.463054036679));
#204696=CARTESIAN_POINT('Ctrl Pts',(184.49065211975,-4.39053733987044,128.583731161379));
#204697=CARTESIAN_POINT('Ctrl Pts',(184.482903255439,-4.45079002018339,
128.707112002701));
#204698=CARTESIAN_POINT('Ctrl Pts',(184.475154391129,-4.50575679107406,
128.832727081082));
#204699=CARTESIAN_POINT('Ctrl Pts',(184.467398393862,-4.56077415977317,
128.958457790189));
#204700=CARTESIAN_POINT('Ctrl Pts',(184.459642396596,-4.61049574662458,
129.086426484169));
#204701=CARTESIAN_POINT('Ctrl Pts',(184.451886399329,-4.65475582965104,
129.216144250433));
#204702=CARTESIAN_POINT('Ctrl Pts',(184.44466748376,-4.6959510224118,129.336879414498));
#204703=CARTESIAN_POINT('Ctrl Pts',(184.437448568192,-4.73241533402233,
129.459129381269));
#204704=CARTESIAN_POINT('Ctrl Pts',(184.430229652623,-4.76405452823406,
129.582490119308));
#204705=CARTESIAN_POINT('Ctrl Pts',(186.18020938313,-4.76405452823405,129.582490119308));
#204706=CARTESIAN_POINT('Ctrl Pts',(186.17256993295,-4.79768574483935,129.713617722427));
#204707=CARTESIAN_POINT('Ctrl Pts',(186.164930482769,-4.82588839263014,
129.846093738758));
#204708=CARTESIAN_POINT('Ctrl Pts',(186.157291032589,-4.84857298836732,
129.979422414441));
#204709=CARTESIAN_POINT('Ctrl Pts',(186.149432621167,-4.87190776796963,
130.116572544767));
#204710=CARTESIAN_POINT('Ctrl Pts',(186.141574209745,-4.88940334476083,
130.254624496003));
#204711=CARTESIAN_POINT('Ctrl Pts',(186.133715798323,-4.90101953991361,
130.393032850591));
#204712=CARTESIAN_POINT('Ctrl Pts',(186.125857386902,-4.9126357350664,130.531441205178));
#204713=CARTESIAN_POINT('Ctrl Pts',(186.11799897548,-4.91837257034282,130.67020550101));
#204714=CARTESIAN_POINT('Ctrl Pts',(186.110140564058,-4.91824801325411,
130.808781321355));
#204715=CARTESIAN_POINT('Origin',(213.235140564004,0.,130.804360617566));
#204716=CARTESIAN_POINT('',(187.929867347344,-4.76405452823404,129.582490119308));
#204717=CARTESIAN_POINT('',(187.584954980304,-4.76405452823404,129.582490119308));
#204718=CARTESIAN_POINT('',(213.235140564004,-4.76405452823405,129.582490119308));
#204719=CARTESIAN_POINT('',(187.514859436036,-4.91824821531416,130.808550493347));
#204720=CARTESIAN_POINT('Ctrl Pts',(187.584954980304,-4.76405452823404,
129.582490119308));
#204721=CARTESIAN_POINT('Ctrl Pts',(187.577318467045,-4.79766509150003,
129.713537195371));
#204722=CARTESIAN_POINT('Ctrl Pts',(187.569681953786,-4.82585013568644,
129.845916938469));
#204723=CARTESIAN_POINT('Ctrl Pts',(187.562045440527,-4.84852382797168,
129.979133526341));
#204724=CARTESIAN_POINT('Ctrl Pts',(187.554181106445,-4.87187394666516,
130.116324377291));
#204725=CARTESIAN_POINT('Ctrl Pts',(187.546316772363,-4.88937865955207,
130.254402327779));
#204726=CARTESIAN_POINT('Ctrl Pts',(187.538452438282,-4.90100172800805,
130.392820674715));
#204727=CARTESIAN_POINT('Ctrl Pts',(187.5305881042,-4.91262479646404,130.53123902165));
#204728=CARTESIAN_POINT('Ctrl Pts',(187.522723770118,-4.91836624934627,
130.669997300341));
#204729=CARTESIAN_POINT('Ctrl Pts',(187.514859436036,-4.91824821531416,
130.808550493347));
#204730=CARTESIAN_POINT('Ctrl Pts',(187.514859435991,-4.91824821531348,
130.808550494141));
#204731=CARTESIAN_POINT('Ctrl Pts',(187.50296817185,-4.91806974195455,131.018049810722));
#204732=CARTESIAN_POINT('Ctrl Pts',(187.49107690771,-4.90450242768287,131.226999653672));
#204733=CARTESIAN_POINT('Ctrl Pts',(187.47918564357,-4.87777335736303,131.434051126228));
#204734=CARTESIAN_POINT('Ctrl Pts',(187.474567584818,-4.86739292886978,
131.514461068646));
#204735=CARTESIAN_POINT('Ctrl Pts',(187.469949526067,-4.85502785952663,
131.594585104556));
#204736=CARTESIAN_POINT('Ctrl Pts',(187.465331467316,-4.84069308080701,
131.674345421989));
#204737=CARTESIAN_POINT('Ctrl Pts',(187.457557133197,-4.8165610016603,131.808619018444));
#204738=CARTESIAN_POINT('Ctrl Pts',(187.449782799078,-4.78679964152417,
131.942100451967));
#204739=CARTESIAN_POINT('Ctrl Pts',(187.442008464958,-4.75147197296815,
132.074280753873));
#204740=CARTESIAN_POINT('Ctrl Pts',(187.434243712011,-4.71618784260629,
132.206298155371));
#204741=CARTESIAN_POINT('Ctrl Pts',(187.426478959064,-4.67535115311574,
132.337017241715));
#204742=CARTESIAN_POINT('Ctrl Pts',(187.418714206117,-4.62907625661752,
132.465936999476));
#204743=CARTESIAN_POINT('Ctrl Pts',(187.410957165232,-4.58284732099878,
132.594728712316));
#204744=CARTESIAN_POINT('Ctrl Pts',(187.403200124347,-4.53119105843935,
132.721724287424));
#204745=CARTESIAN_POINT('Ctrl Pts',(187.395443083462,-4.47427212062073,
132.846436045442));
#204746=CARTESIAN_POINT('Ctrl Pts',(187.387691892222,-4.41739610581604,
132.971053757354));
#204747=CARTESIAN_POINT('Ctrl Pts',(187.379940700982,-4.35526547673165,
133.093390725966));
#204748=CARTESIAN_POINT('Ctrl Pts',(187.372189509742,-4.28809353286631,
133.212977838274));
#204749=CARTESIAN_POINT('Ctrl Pts',(187.364441612965,-4.22095013886891,
133.332514122869));
#204750=CARTESIAN_POINT('Ctrl Pts',(187.356693716188,-4.14876988281084,
133.44930253558));
#204751=CARTESIAN_POINT('Ctrl Pts',(187.348945819411,-4.07181258012,133.562897435315));
#204752=CARTESIAN_POINT('Ctrl Pts',(187.341199543326,-3.99487137523789,
133.676468573446));
#204753=CARTESIAN_POINT('Ctrl Pts',(187.333453267242,-3.91315533044107,
133.786847203844));
#204754=CARTESIAN_POINT('Ctrl Pts',(187.325706991158,-3.82696805196249,
133.893615963399));
#204755=CARTESIAN_POINT('Ctrl Pts',(187.317960657893,-3.74078013726901,
134.000385511097));
#204756=CARTESIAN_POINT('Ctrl Pts',(187.310214324628,-3.65012116860682,
134.103544830563));
#204757=CARTESIAN_POINT('Ctrl Pts',(187.302467991362,-3.55533531112048,
134.202709317744));
#204758=CARTESIAN_POINT('Ctrl Pts',(187.294719923359,-3.46052822699846,
134.301896012124));
#204759=CARTESIAN_POINT('Ctrl Pts',(187.286971855356,-3.36159268511726,
134.397085811471));
#204760=CARTESIAN_POINT('Ctrl Pts',(187.279223787353,-3.25890970925504,
134.487930973813));
#204761=CARTESIAN_POINT('Ctrl Pts',(187.271467484611,-3.15611760070424,
134.578872687475));
#204762=CARTESIAN_POINT('Ctrl Pts',(187.263711181869,-3.04957039534964,
134.665460280642));
#204763=CARTESIAN_POINT('Ctrl Pts',(187.255954879128,-2.93968263329513,
134.747385988776));
#204764=CARTESIAN_POINT('Ctrl Pts',(187.248194436613,-2.82973622083337,
134.829355423126));
#204765=CARTESIAN_POINT('Ctrl Pts',(187.240433994099,-2.71644602177129,
134.906657794264));
#204766=CARTESIAN_POINT('Ctrl Pts',(187.232673551585,-2.60025471421194,
134.979029285103));
#204767=CARTESIAN_POINT('Ctrl Pts',(187.22490065132,-2.48387688605068,135.051516953085));
#204768=CARTESIAN_POINT('Ctrl Pts',(187.217127751054,-2.36458898340092,
135.119057730363));
#204769=CARTESIAN_POINT('Ctrl Pts',(187.209354850789,-2.24285817365602,
135.181433872078));
#204770=CARTESIAN_POINT('Ctrl Pts',(187.201864515027,-2.12555258546736,
135.241542483926));
#204771=CARTESIAN_POINT('Ctrl Pts',(187.194374179265,-2.0059788977942,135.296855306772));
#204772=CARTESIAN_POINT('Ctrl Pts',(187.186883843503,-1.88456999546703,
135.347220839352));
#204773=CARTESIAN_POINT('Ctrl Pts',(187.179109509384,-1.75855783770604,
135.399495996409));
#204774=CARTESIAN_POINT('Ctrl Pts',(187.171335175265,-1.63016938517756,
135.446606896525));
#204775=CARTESIAN_POINT('Ctrl Pts',(187.163560841146,-1.49986688586205,
135.488331410301));
#204776=CARTESIAN_POINT('Ctrl Pts',(187.155796088199,-1.36972497273157,
135.530004502343));
#204777=CARTESIAN_POINT('Ctrl Pts',(187.148031335251,-1.23767407507255,
135.566304298079));
#204778=CARTESIAN_POINT('Ctrl Pts',(187.140266582304,-1.10419751978648,
135.597056195192));
#204779=CARTESIAN_POINT('Ctrl Pts',(187.132509541419,-0.970853535296745,
135.627777549087));
#204780=CARTESIAN_POINT('Ctrl Pts',(187.124752500534,-0.836087089569735,
135.6529618828));
#204781=CARTESIAN_POINT('Ctrl Pts',(187.116995459649,-0.700397479315045,
135.672484119848));
#204782=CARTESIAN_POINT('Ctrl Pts',(187.109244268409,-0.564810193650936,
135.691991635025));
#204783=CARTESIAN_POINT('Ctrl Pts',(187.101493077169,-0.42830151454915,
135.705845496927));
#204784=CARTESIAN_POINT('Ctrl Pts',(187.093741885929,-0.291381413656383,
135.713971593425));
#204785=CARTESIAN_POINT('Ctrl Pts',(187.085993989152,-0.154519507459005,
135.722094236115));
#204786=CARTESIAN_POINT('Ctrl Pts',(187.078246092375,-0.017246916725652,
135.724493932228));
#204787=CARTESIAN_POINT('Ctrl Pts',(187.070498195598,0.119920991487449,
135.721148391947));
#204788=CARTESIAN_POINT('Ctrl Pts',(187.062751919514,0.257060207131151,
135.717803551481));
#204789=CARTESIAN_POINT('Ctrl Pts',(187.05500564343,0.394094393208233,135.708715874552));
#204790=CARTESIAN_POINT('Ctrl Pts',(187.047259367345,0.53050830372916,135.693915198729));
#204791=CARTESIAN_POINT('Ctrl Pts',(187.03951303408,0.66692322122647,135.679114413651));
#204792=CARTESIAN_POINT('Ctrl Pts',(187.031766700815,0.802717465346965,
135.658600587698));
#204793=CARTESIAN_POINT('Ctrl Pts',(187.024020367549,0.937381428141232,
135.632455388868));
#204794=CARTESIAN_POINT('Ctrl Pts',(187.016272299546,1.07207554799625,135.606304335003));
#204795=CARTESIAN_POINT('Ctrl Pts',(187.008524231543,1.20563849912314,135.574519473305));
#204796=CARTESIAN_POINT('Ctrl Pts',(187.000776163541,1.33757176369478,135.537233406842));
#204797=CARTESIAN_POINT('Ctrl Pts',(186.993019860799,1.46964524851015,135.499907712303));
#204798=CARTESIAN_POINT('Ctrl Pts',(186.985263558057,1.60008520998432,135.457069239991));
#204799=CARTESIAN_POINT('Ctrl Pts',(186.977507255315,1.7284086480416,135.408900399985));
#204800=CARTESIAN_POINT('Ctrl Pts',(186.969746812801,1.85680057618161,135.360705850817));
#204801=CARTESIAN_POINT('Ctrl Pts',(186.961986370287,1.98307337019677,135.307175417617));
#204802=CARTESIAN_POINT('Ctrl Pts',(186.954225927772,2.10676579497374,135.248538938429));
#204803=CARTESIAN_POINT('Ctrl Pts',(186.946453027507,2.23065678181183,135.189808330759));
#204804=CARTESIAN_POINT('Ctrl Pts',(186.938680127242,2.3519587757408,135.125955479745));
#204805=CARTESIAN_POINT('Ctrl Pts',(186.930907226976,2.47023606645755,135.05725573013));
#204806=CARTESIAN_POINT('Ctrl Pts',(186.923416891214,2.58421367973449,134.991053389458));
#204807=CARTESIAN_POINT('Ctrl Pts',(186.915926555452,2.69538242307315,134.920350591354));
#204808=CARTESIAN_POINT('Ctrl Pts',(186.90843621969,2.80338084934492,134.845429643953));
#204809=CARTESIAN_POINT('Ctrl Pts',(186.900661885571,2.91547406877391,134.76766804606));
#204810=CARTESIAN_POINT('Ctrl Pts',(186.892887551452,3.02450689794558,134.685115797058));
#204811=CARTESIAN_POINT('Ctrl Pts',(186.885113217333,3.13004259678052,134.5980417329));
#204812=CARTESIAN_POINT('Ctrl Pts',(186.877348464386,3.23544823229863,134.511074979743));
#204813=CARTESIAN_POINT('Ctrl Pts',(186.869583711439,3.3373650142225,134.419597745934));
#204814=CARTESIAN_POINT('Ctrl Pts',(186.861818958491,3.43538479468078,134.323922291266));
#204815=CARTESIAN_POINT('Ctrl Pts',(186.854061917606,3.53330722051126,134.228341862808));
#204816=CARTESIAN_POINT('Ctrl Pts',(186.846304876721,3.62734006948965,134.128571782767));
#204817=CARTESIAN_POINT('Ctrl Pts',(186.838547835836,3.7171082291624,134.024964516712));
#204818=CARTESIAN_POINT('Ctrl Pts',(186.830796644596,3.8068086939677,133.921435381702));
#204819=CARTESIAN_POINT('Ctrl Pts',(186.823045453356,3.89225061581199,133.814075114605));
#204820=CARTESIAN_POINT('Ctrl Pts',(186.815294262116,3.97309598993045,133.703272709593));
#204821=CARTESIAN_POINT('Ctrl Pts',(186.807546365339,4.05390700260826,133.592517398559));
#204822=CARTESIAN_POINT('Ctrl Pts',(186.799798468562,4.13012512327185,133.478323174578));
#204823=CARTESIAN_POINT('Ctrl Pts',(186.792050571785,4.20145303038427,133.36111158236));
#204824=CARTESIAN_POINT('Ctrl Pts',(186.784304295701,4.27276601723617,133.24392450828));
#204825=CARTESIAN_POINT('Ctrl Pts',(186.776558019617,4.33919062208088,133.123721655165));
#204826=CARTESIAN_POINT('Ctrl Pts',(186.768811743533,4.40047344506548,133.000952641992));
#204827=CARTESIAN_POINT('Ctrl Pts',(186.761065410267,4.46175672042594,132.878182722566));
#204828=CARTESIAN_POINT('Ctrl Pts',(186.753319077002,4.51789796357578,132.752846955089));
#204829=CARTESIAN_POINT('Ctrl Pts',(186.745572743736,4.56869042857052,132.62541823071));
#204830=CARTESIAN_POINT('Ctrl Pts',(186.737824675734,4.61949426818561,132.497960969551));
#204831=CARTESIAN_POINT('Ctrl Pts',(186.730076607731,4.66494680138576,132.368410181932));
#204832=CARTESIAN_POINT('Ctrl Pts',(186.722328539728,4.70489012982407,132.237256960218));
#204833=CARTESIAN_POINT('Ctrl Pts',(186.714572236986,4.74487591050721,132.105964347298));
#204834=CARTESIAN_POINT('Ctrl Pts',(186.706815934244,4.77934067585266,131.973066272786));
#204835=CARTESIAN_POINT('Ctrl Pts',(186.699059631502,4.80817681928663,131.839067695427));
#204836=CARTESIAN_POINT('Ctrl Pts',(186.691299188988,4.83702835343861,131.704997598992));
#204837=CARTESIAN_POINT('Ctrl Pts',(186.683538746474,4.86024521347585,131.569826214457));
#204838=CARTESIAN_POINT('Ctrl Pts',(186.675778303959,4.8777714598113,131.434065825064));
#204839=CARTESIAN_POINT('Ctrl Pts',(186.668005403694,4.89532584083327,131.298087501042));
#204840=CARTESIAN_POINT('Ctrl Pts',(186.660232503429,4.90717131955267,131.161518672433));
#204841=CARTESIAN_POINT('Ctrl Pts',(186.652459603163,4.91330403923953,131.024874745214));
#204842=CARTESIAN_POINT('Ctrl Pts',(186.644969267401,4.91921381911843,130.893198168935));
#204843=CARTESIAN_POINT('Ctrl Pts',(186.637478931639,4.91981897388855,130.761452167314));
#204844=CARTESIAN_POINT('Ctrl Pts',(186.629988595877,4.91516164637668,130.630093430501));
#204845=CARTESIAN_POINT('Ctrl Pts',(186.622214261758,4.91032773487667,130.493754187256));
#204846=CARTESIAN_POINT('Ctrl Pts',(186.614439927639,4.89980909723262,130.357400273068));
#204847=CARTESIAN_POINT('Ctrl Pts',(186.60666559352,4.88359584406322,130.221544442131));
#204848=CARTESIAN_POINT('Ctrl Pts',(186.598900840573,4.86740257227934,130.085856041365));
#204849=CARTESIAN_POINT('Ctrl Pts',(186.591136087626,4.84552869479156,129.95066488697));
#204850=CARTESIAN_POINT('Ctrl Pts',(186.583371334678,4.81801631071333,129.816483149354));
#204851=CARTESIAN_POINT('Ctrl Pts',(186.575614293793,4.79053125232284,129.682434682933));
#204852=CARTESIAN_POINT('Ctrl Pts',(186.567857252908,4.75741891010157,129.549394018657));
#204853=CARTESIAN_POINT('Ctrl Pts',(186.560100212023,4.71877306587156,129.417867265507));
#204854=CARTESIAN_POINT('Ctrl Pts',(186.552349020783,4.68015636477332,129.286439697704));
#204855=CARTESIAN_POINT('Ctrl Pts',(186.544597829543,4.63601457725516,129.156524142229));
#204856=CARTESIAN_POINT('Ctrl Pts',(186.536846638303,4.58649227530057,129.028615232915));
#204857=CARTESIAN_POINT('Ctrl Pts',(186.529098741526,4.53699102164532,128.9007606883));
#204858=CARTESIAN_POINT('Ctrl Pts',(186.521350844749,4.48211394281148,128.774911457366));
#204859=CARTESIAN_POINT('Ctrl Pts',(186.513602947972,4.42205498674884,128.651545540354));
#204860=CARTESIAN_POINT('Ctrl Pts',(186.505856671888,4.3620085937251,128.528205428834));
#204861=CARTESIAN_POINT('Ctrl Pts',(186.498110395804,4.29678265050747,128.407347949309));
#204862=CARTESIAN_POINT('Ctrl Pts',(186.490364119719,4.2266184654652,128.289429324292));
#204863=CARTESIAN_POINT('Ctrl Pts',(186.482617786454,4.15645376248687,128.171509828827));
#204864=CARTESIAN_POINT('Ctrl Pts',(186.474871453189,4.08135094486343,128.056529567145));
#204865=CARTESIAN_POINT('Ctrl Pts',(186.467125119923,4.00159611807821,127.94491808968));
#204866=CARTESIAN_POINT('Ctrl Pts',(186.45937705192,3.92182343075255,127.833281617599));
#204867=CARTESIAN_POINT('Ctrl Pts',(186.451628983917,3.83739688849461,127.725015748974));
#204868=CARTESIAN_POINT('Ctrl Pts',(186.443880915914,3.74864431330477,127.620518775573));
#204869=CARTESIAN_POINT('Ctrl Pts',(186.436124613173,3.65979741082176,127.515910741544));
#204870=CARTESIAN_POINT('Ctrl Pts',(186.428368310431,3.56661554438332,127.415079902877));
#204871=CARTESIAN_POINT('Ctrl Pts',(186.420612007689,3.46946538610199,127.318389734564));
#204872=CARTESIAN_POINT('Ctrl Pts',(186.412851565175,3.37226337585601,127.221647959797));
#204873=CARTESIAN_POINT('Ctrl Pts',(186.405091122661,3.2710891417477,127.129051522826));
#204874=CARTESIAN_POINT('Ctrl Pts',(186.397330680146,3.166343445464,127.040924388816));
#204875=CARTESIAN_POINT('Ctrl Pts',(186.389557779881,3.06142960208977,126.952655785307));
#204876=CARTESIAN_POINT('Ctrl Pts',(186.381784879615,2.95293314934019,126.868871060837));
#204877=CARTESIAN_POINT('Ctrl Pts',(186.37401197935,2.84128562820487,126.789852049702));
#204878=CARTESIAN_POINT('Ctrl Pts',(186.366521643588,2.73369677568628,126.713705578658));
#204879=CARTESIAN_POINT('Ctrl Pts',(186.359031307826,2.6231822342181,126.641984512861));
#204880=CARTESIAN_POINT('Ctrl Pts',(186.351540972064,2.51014900938351,126.574900248537));
#204881=CARTESIAN_POINT('Ctrl Pts',(186.343766637945,2.39283009547328,126.50527246394));
#204882=CARTESIAN_POINT('Ctrl Pts',(186.335992303826,2.27242610514435,126.440419470445));
#204883=CARTESIAN_POINT('Ctrl Pts',(186.328217969707,2.14936308757183,126.380626744435));
#204884=CARTESIAN_POINT('Ctrl Pts',(186.32045321676,2.02645173417003,126.320907707617));
#204885=CARTESIAN_POINT('Ctrl Pts',(186.312688463813,1.90088822208354,126.266236699069));
#204886=CARTESIAN_POINT('Ctrl Pts',(186.304923710865,1.773126210382,126.216855140233));
#204887=CARTESIAN_POINT('Ctrl Pts',(186.29716666998,1.64549109371175,126.167522627858));
#204888=CARTESIAN_POINT('Ctrl Pts',(186.289409629095,1.51566218516442,126.123469250419));
#204889=CARTESIAN_POINT('Ctrl Pts',(186.28165258821,1.38411597992469,126.08488967088));
#204890=CARTESIAN_POINT('Ctrl Pts',(186.27390139697,1.25266897470157,126.046339184501));
#204891=CARTESIAN_POINT('Ctrl Pts',(186.26615020573,1.11950762410406,126.013254389403));
#204892=CARTESIAN_POINT('Ctrl Pts',(186.25839901449,0.985126222273834,125.985781014749));
#204893=CARTESIAN_POINT('Ctrl Pts',(186.250651117713,0.850801936124037,
125.958319317012));
#204894=CARTESIAN_POINT('Ctrl Pts',(186.242903220936,0.715259012346737,
125.936464374276));
#204895=CARTESIAN_POINT('Ctrl Pts',(186.235155324159,0.579004439687522,
125.920311383445));
#204896=CARTESIAN_POINT('Ctrl Pts',(186.227409048075,0.442778368547621,
125.904161771471));
#204897=CARTESIAN_POINT('Ctrl Pts',(186.219662771991,0.305841332620214,
125.893711785003));
#204898=CARTESIAN_POINT('Ctrl Pts',(186.211916495907,0.168707597893969,
125.889005003888));
#204899=CARTESIAN_POINT('Ctrl Pts',(186.204170162641,0.0315728508776698,
125.884298188029));
#204900=CARTESIAN_POINT('Ctrl Pts',(186.196423829376,-0.10575820709968,
125.885334675529));
#204901=CARTESIAN_POINT('Ctrl Pts',(186.18867749611,-0.242769536089092,
125.892105940247));
#204902=CARTESIAN_POINT('Ctrl Pts',(186.180929428107,-0.379811547815777,
125.898878721341));
#204903=CARTESIAN_POINT('Ctrl Pts',(186.173181360104,-0.516533297662758,
125.911388815894));
#204904=CARTESIAN_POINT('Ctrl Pts',(186.165433292102,-0.652422495685759,
125.929575704401));
#204905=CARTESIAN_POINT('Ctrl Pts',(186.15767698936,-0.788456118365381,
125.947781922149));
#204906=CARTESIAN_POINT('Ctrl Pts',(186.149920686618,-0.923655033517907,
125.971676934201));
#204907=CARTESIAN_POINT('Ctrl Pts',(186.142164383876,-1.05751524410295,
126.001148716037));
#204908=CARTESIAN_POINT('Ctrl Pts',(186.134403941362,-1.19144689991294,
126.03063622785));
#204909=CARTESIAN_POINT('Ctrl Pts',(186.126643498848,-1.3240380496573,126.065706340432));
#204910=CARTESIAN_POINT('Ctrl Pts',(186.118883056333,-1.45479951078708,
126.106196992711));
#204911=CARTESIAN_POINT('Ctrl Pts',(186.111110156068,-1.5857708818227,126.146752644179));
#204912=CARTESIAN_POINT('Ctrl Pts',(186.103337255803,-1.7149063263107,126.192746092524));
#204913=CARTESIAN_POINT('Ctrl Pts',(186.095564355537,-1.8417354706294,126.243966608412));
#204914=CARTESIAN_POINT('Ctrl Pts',(186.088074019775,-1.96395405608863,
126.293325129531));
#204915=CARTESIAN_POINT('Ctrl Pts',(186.080583684013,-2.08403082912152,
126.347537155255));
#204916=CARTESIAN_POINT('Ctrl Pts',(186.073093348251,-2.20156793963613,
126.406374525084));
#204917=CARTESIAN_POINT('Ctrl Pts',(186.065318218632,-2.32357398828093,
126.467448980412));
#204918=CARTESIAN_POINT('Ctrl Pts',(186.057543089012,-2.44322994792608,
126.533700949362));
#204919=CARTESIAN_POINT('Ctrl Pts',(186.049767959393,-2.56006520571822,
126.604926226488));
#204920=CARTESIAN_POINT('Ctrl Pts',(186.042002588127,-2.67675382676365,
126.67606211071));
#204921=CARTESIAN_POINT('Ctrl Pts',(186.03423721686,-2.79062845967751,126.75215868097));
#204922=CARTESIAN_POINT('Ctrl Pts',(186.026471845594,-2.90124067215559,
126.832964688585));
#204923=CARTESIAN_POINT('Ctrl Pts',(186.018491328848,-3.01491747957512,
126.916009487709));
#204924=CARTESIAN_POINT('Ctrl Pts',(186.010510812103,-3.12514807592882,
127.004028321582));
#204925=CARTESIAN_POINT('Ctrl Pts',(186.002530295357,-3.2314741111118,127.096698533218));
#204926=CARTESIAN_POINT('Ctrl Pts',(185.994779503498,-3.33473947526146,
127.186701166476));
#204927=CARTESIAN_POINT('Ctrl Pts',(185.987028711639,-3.43432165183175,
127.28109080366));
#204928=CARTESIAN_POINT('Ctrl Pts',(185.979277919781,-3.52983187439647,
127.37952923471));
#204929=CARTESIAN_POINT('Ctrl Pts',(185.971530630239,-3.62529893917089,
127.477923184813));
#204930=CARTESIAN_POINT('Ctrl Pts',(185.963783340697,-3.71669743948121,
127.580362008493));
#204931=CARTESIAN_POINT('Ctrl Pts',(185.956036051155,-3.80367440789667,
127.686469653916));
#204932=CARTESIAN_POINT('Ctrl Pts',(185.948290584601,-3.89063091006273,
127.792552331516));
#204933=CARTESIAN_POINT('Ctrl Pts',(185.940545118047,-3.97316770391064,
127.902301810235));
#204934=CARTESIAN_POINT('Ctrl Pts',(185.932799651493,-4.05097143863642,
128.015308186031));
#204935=CARTESIAN_POINT('Ctrl Pts',(185.925054330194,-4.12877371426179,
128.12831244255));
#204936=CARTESIAN_POINT('Ctrl Pts',(185.917309008896,-4.20184288741614,
128.244573151684));
#204937=CARTESIAN_POINT('Ctrl Pts',(185.909563687597,-4.26990858509716,
128.363650938515));
#204938=CARTESIAN_POINT('Ctrl Pts',(185.901814172698,-4.33801113604076,
128.482793198423));
#204939=CARTESIAN_POINT('Ctrl Pts',(185.894064657798,-4.40110460739271,
128.604755242451));
#204940=CARTESIAN_POINT('Ctrl Pts',(185.886315142899,-4.45896424491958,
128.729072462868));
#204941=CARTESIAN_POINT('Ctrl Pts',(185.878563054062,-4.51684310004943,
128.853430974228));
#204942=CARTESIAN_POINT('Ctrl Pts',(185.870810965225,-4.56948450454414,
128.980145861196));
#204943=CARTESIAN_POINT('Ctrl Pts',(185.863058876388,-4.61671198790392,
129.108732862649));
#204944=CARTESIAN_POINT('Ctrl Pts',(185.855299774332,-4.66398219738179,
129.237436195167));
#204945=CARTESIAN_POINT('Ctrl Pts',(185.847540672277,-4.70582858667214,
129.368014652284));
#204946=CARTESIAN_POINT('Ctrl Pts',(185.839781570221,-4.74212459112503,
129.49996902577));
#204947=CARTESIAN_POINT('Ctrl Pts',(185.838167528046,-4.74967485680883,
129.527418068522));
#204948=CARTESIAN_POINT('Ctrl Pts',(185.83655348587,-4.75698512267265,129.554926614318));
#204949=CARTESIAN_POINT('Ctrl Pts',(185.834939443695,-4.76405452823405,
129.582490119308));
#204950=CARTESIAN_POINT('',(187.860140563976,-4.91824998954374,130.80468132454));
#204951=CARTESIAN_POINT('Ctrl Pts',(187.860140563976,-4.91824998954374,
130.80468132454));
#204952=CARTESIAN_POINT('Ctrl Pts',(187.851985238763,-4.91824054696515,
130.949489407629));
#204953=CARTESIAN_POINT('Ctrl Pts',(187.84382991355,-4.91183143561811,131.094160796668));
#204954=CARTESIAN_POINT('Ctrl Pts',(187.835674588336,-4.89908446976143,
131.238128321115));
#204955=CARTESIAN_POINT('Ctrl Pts',(187.827507043422,-4.8863184042239,131.382311562291));
#204956=CARTESIAN_POINT('Ctrl Pts',(187.819339498508,-4.86719555824919,
131.525788509872));
#204957=CARTESIAN_POINT('Ctrl Pts',(187.811171953594,-4.84182909625093,
131.668000626596));
#204958=CARTESIAN_POINT('Ctrl Pts',(187.802983701521,-4.81639832271632,
131.810573293393));
#204959=CARTESIAN_POINT('Ctrl Pts',(187.794795449448,-4.78469233773483,
131.951874395443));
#204960=CARTESIAN_POINT('Ctrl Pts',(187.786607197375,-4.74687508460216,
132.091357118604));
#204961=CARTESIAN_POINT('Ctrl Pts',(187.778407825462,-4.70900647474592,
132.2310292626));
#204962=CARTESIAN_POINT('Ctrl Pts',(187.770208453549,-4.66501012991102,
132.368877788919));
#204963=CARTESIAN_POINT('Ctrl Pts',(187.762009081637,-4.61509878206581,
132.504374233475));
#204964=CARTESIAN_POINT('Ctrl Pts',(187.7537907155,-4.56507181227561,132.640184561809));
#204965=CARTESIAN_POINT('Ctrl Pts',(187.745572349363,-4.5091025670614,132.773631612781));
#204966=CARTESIAN_POINT('Ctrl Pts',(187.737353983226,-4.44745127249184,
132.904208288544));
#204967=CARTESIAN_POINT('Ctrl Pts',(187.732966020474,-4.4145343179928,132.973925989116));
#204968=CARTESIAN_POINT('Ctrl Pts',(187.728578057722,-4.37999833546582,
133.042825876845));
#204969=CARTESIAN_POINT('Ctrl Pts',(187.724190094969,-4.34388802098799,
133.110834099663));
#204970=CARTESIAN_POINT('Ctrl Pts',(187.71641576085,-4.27990989132784,133.23132706574));
#204971=CARTESIAN_POINT('Ctrl Pts',(187.708641426731,-4.21081318308159,
133.349346880017));
#204972=CARTESIAN_POINT('Ctrl Pts',(187.700867092612,-4.13681326770758,
133.464428107428));
#204973=CARTESIAN_POINT('Ctrl Pts',(187.693102339665,-4.06290455061579,
133.57936750751));
#204974=CARTESIAN_POINT('Ctrl Pts',(187.685337586718,-3.98410485912279,
133.691375200834));
#204975=CARTESIAN_POINT('Ctrl Pts',(187.677572833771,-3.90067606158043,
133.800009015678));
#204976=CARTESIAN_POINT('Ctrl Pts',(187.669815792886,-3.81733012669587,
133.908534933887));
#204977=CARTESIAN_POINT('Ctrl Pts',(187.662058752001,-3.72936447197065,
134.013693334156));
#204978=CARTESIAN_POINT('Ctrl Pts',(187.654301711116,-3.63708479189096,
134.115070100305));
#204979=CARTESIAN_POINT('Ctrl Pts',(187.646550519876,-3.54487470063586,
134.216370417446));
#204980=CARTESIAN_POINT('Ctrl Pts',(187.638799328636,-3.44835732151588,
134.313894488769));
#204981=CARTESIAN_POINT('Ctrl Pts',(187.631048137396,-3.34787900468798,
134.407260731706));
#204982=CARTESIAN_POINT('Ctrl Pts',(187.623300240619,-3.24744339382506,
134.500587291499));
#204983=CARTESIAN_POINT('Ctrl Pts',(187.615552343842,-3.14305047942049,
134.589759272133));
#204984=CARTESIAN_POINT('Ctrl Pts',(187.607804447065,-3.03508373938013,
134.674431645009));
#204985=CARTESIAN_POINT('Ctrl Pts',(187.60005817098,-2.92713958365424,134.759086306249));
#204986=CARTESIAN_POINT('Ctrl Pts',(187.592311894896,-2.81562339669253,
134.839242990757));
#204987=CARTESIAN_POINT('Ctrl Pts',(187.584565618812,-2.70095172170201,
134.914596968378));
#204988=CARTESIAN_POINT('Ctrl Pts',(187.576819285547,-2.58627920023135,
134.989951502245));
#204989=CARTESIAN_POINT('Ctrl Pts',(187.569072952282,-2.4684514709862,135.060503043776));
#204990=CARTESIAN_POINT('Ctrl Pts',(187.561326619016,-2.34791369668973,
135.125990441533));
#204991=CARTESIAN_POINT('Ctrl Pts',(187.553578551013,-2.22734892879446,
135.191492504738));
#204992=CARTESIAN_POINT('Ctrl Pts',(187.54583048301,-2.10407325166797,135.251927980875));
#204993=CARTESIAN_POINT('Ctrl Pts',(187.538082415007,-1.97855567117998,
135.307082074479));
#204994=CARTESIAN_POINT('Ctrl Pts',(187.530326112265,-1.8529046891137,135.36229478651));
#204995=CARTESIAN_POINT('Ctrl Pts',(187.522569809524,-1.72500740244735,
135.412214745672));
#204996=CARTESIAN_POINT('Ctrl Pts',(187.514813506782,-1.59535252627577,
135.456675458525));
#204997=CARTESIAN_POINT('Ctrl Pts',(187.507053064268,-1.46562844939287,
135.501159901399));
#204998=CARTESIAN_POINT('Ctrl Pts',(187.499292621754,-1.33414528842969,
135.540179180866));
#204999=CARTESIAN_POINT('Ctrl Pts',(187.491532179239,-1.20140513403331,
135.573617243752));
#205000=CARTESIAN_POINT('Ctrl Pts',(187.483759278974,-1.06845189335697,
135.607108984385));
#205001=CARTESIAN_POINT('Ctrl Pts',(187.475986378709,-0.934238009971892,
135.635001524974));
#205002=CARTESIAN_POINT('Ctrl Pts',(187.468213478443,-0.799274826844706,
135.657230161833));
#205003=CARTESIAN_POINT('Ctrl Pts',(187.460723142681,-0.669217895375251,
135.678650731752));
#205004=CARTESIAN_POINT('Ctrl Pts',(187.453232806919,-0.538465501906267,
135.694812005137));
#205005=CARTESIAN_POINT('Ctrl Pts',(187.445742471157,-0.40747611749601,
135.705701890745));
#205006=CARTESIAN_POINT('Ctrl Pts',(187.437968137038,-0.271520230763168,
135.717004669676));
#205007=CARTESIAN_POINT('Ctrl Pts',(187.430193802919,-0.134878359929164,
135.722664244519));
#205008=CARTESIAN_POINT('Ctrl Pts',(187.4224194688,0.0019414977692763,135.722610234359));
#205009=CARTESIAN_POINT('Ctrl Pts',(187.414654715853,0.138592737221022,
135.722556290762));
#205010=CARTESIAN_POINT('Ctrl Pts',(187.406889962905,0.275421139878357,
135.716802772767));
#205011=CARTESIAN_POINT('Ctrl Pts',(187.399125209958,0.411913147910088,
135.70533099302));
#205012=CARTESIAN_POINT('Ctrl Pts',(187.391368169073,0.548269590155265,
135.693870607207));
#205013=CARTESIAN_POINT('Ctrl Pts',(187.383611128188,0.684289915601994,
135.676703294552));
#205014=CARTESIAN_POINT('Ctrl Pts',(187.375854087303,0.819460481241922,
135.653862404573));
#205015=CARTESIAN_POINT('Ctrl Pts',(187.368102896063,0.954529113706643,
135.631038739087));
#205016=CARTESIAN_POINT('Ctrl Pts',(187.360351704823,1.08874887791857,135.602550077227));
#205017=CARTESIAN_POINT('Ctrl Pts',(187.352600513583,1.22161152693562,135.568481558491));
#205018=CARTESIAN_POINT('Ctrl Pts',(187.344852616806,1.35441770578278,135.534427519784));
#205019=CARTESIAN_POINT('Ctrl Pts',(187.337104720029,1.4858675387463,135.494798438013));
#205020=CARTESIAN_POINT('Ctrl Pts',(187.329356823252,1.6154634643188,135.449730447617));
#205021=CARTESIAN_POINT('Ctrl Pts',(187.321610547168,1.74503228121749,135.404671884473));
#205022=CARTESIAN_POINT('Ctrl Pts',(187.313864271084,1.87274759303631,135.354176803992));
#205023=CARTESIAN_POINT('Ctrl Pts',(187.306117994999,1.99812786988819,135.298430941679));
#205024=CARTESIAN_POINT('Ctrl Pts',(187.298371661734,2.12350907226879,135.242684667863));
#205025=CARTESIAN_POINT('Ctrl Pts',(187.290625328469,2.24655484804188,135.181687693709));
#205026=CARTESIAN_POINT('Ctrl Pts',(187.282878995203,2.36680486178025,135.115673388492));
#205027=CARTESIAN_POINT('Ctrl Pts',(187.2751309272,2.48708180467538,135.04964429983));
#205028=CARTESIAN_POINT('Ctrl Pts',(187.267382859197,2.60456139703364,134.978595832385));
#205029=CARTESIAN_POINT('Ctrl Pts',(187.259634791194,2.71880941621897,134.902806471884));
#205030=CARTESIAN_POINT('Ctrl Pts',(187.251878488453,2.83317885955863,134.826936561549));
#205031=CARTESIAN_POINT('Ctrl Pts',(187.244122185711,2.9443095425167,134.746315909328));
#205032=CARTESIAN_POINT('Ctrl Pts',(187.236365882969,3.05179722699965,134.661265691298));
#205033=CARTESIAN_POINT('Ctrl Pts',(187.228605440455,3.15934228089629,134.576170079406));
#205034=CARTESIAN_POINT('Ctrl Pts',(187.220844997941,3.26324016595116,134.486640445942));
#205035=CARTESIAN_POINT('Ctrl Pts',(187.213084555426,3.36312185108178,134.393036484411));
#205036=CARTESIAN_POINT('Ctrl Pts',(187.205311655161,3.46316387516043,134.299282261492));
#205037=CARTESIAN_POINT('Ctrl Pts',(187.197538754896,3.55917654184175,134.201440919767));
#205038=CARTESIAN_POINT('Ctrl Pts',(187.18976585463,3.65082902071832,134.099907692633));
#205039=CARTESIAN_POINT('Ctrl Pts',(187.182275518868,3.73914970112908,134.002065454052));
#205040=CARTESIAN_POINT('Ctrl Pts',(187.174785183106,3.82342150061338,133.900795325352));
#205041=CARTESIAN_POINT('Ctrl Pts',(187.167294847344,3.90338643166027,133.796476495608));
#205042=CARTESIAN_POINT('Ctrl Pts',(187.159520513225,3.98638325737254,133.688202385727));
#205043=CARTESIAN_POINT('Ctrl Pts',(187.151746179106,4.06500308682427,133.576300848341));
#205044=CARTESIAN_POINT('Ctrl Pts',(187.143971844987,4.13891212164383,133.461161233309));
#205045=CARTESIAN_POINT('Ctrl Pts',(187.13620709204,4.2127300701834,133.346163517562));
#205046=CARTESIAN_POINT('Ctrl Pts',(187.128442339093,4.28184856640189,133.227935990211));
#205047=CARTESIAN_POINT('Ctrl Pts',(187.120677586145,4.34597429754696,133.106900621032));
#205048=CARTESIAN_POINT('Ctrl Pts',(187.11292054526,4.41003633811182,132.985985465888));
#205049=CARTESIAN_POINT('Ctrl Pts',(187.105163504375,4.46911530015668,132.862268361969));
#205050=CARTESIAN_POINT('Ctrl Pts',(187.09740646349,4.52296160498285,132.736199477914));
#205051=CARTESIAN_POINT('Ctrl Pts',(187.08965527225,4.5767673038917,132.610225663385));
#205052=CARTESIAN_POINT('Ctrl Pts',(187.08190408101,4.62534804688488,132.481903956843));
#205053=CARTESIAN_POINT('Ctrl Pts',(187.07415288977,4.6685007443457,132.351707980812));
#205054=CARTESIAN_POINT('Ctrl Pts',(187.066404992993,4.71163510075898,132.221567341544));
#205055=CARTESIAN_POINT('Ctrl Pts',(187.058657096216,4.74934587746924,132.089554387528));
#205056=CARTESIAN_POINT('Ctrl Pts',(187.050909199439,4.7814786640856,131.956161315341));
#205057=CARTESIAN_POINT('Ctrl Pts',(187.043162923355,4.8136047292157,131.822796146108));
#205058=CARTESIAN_POINT('Ctrl Pts',(187.035416647271,4.84015503356989,131.688051812779));
#205059=CARTESIAN_POINT('Ctrl Pts',(187.027670371187,4.86102556302323,131.552433834661));
#205060=CARTESIAN_POINT('Ctrl Pts',(187.019924037921,4.88189624653807,131.416814855442));
#205061=CARTESIAN_POINT('Ctrl Pts',(187.012177704656,4.89708701202375,131.280322604983));
#205062=CARTESIAN_POINT('Ctrl Pts',(187.00443137139,4.90654537711804,131.143470518309));
#205063=CARTESIAN_POINT('Ctrl Pts',(186.996683303387,4.9160058603476,131.006587784559));
#205064=CARTESIAN_POINT('Ctrl Pts',(186.988935235385,4.91973136175744,130.869345444204));
#205065=CARTESIAN_POINT('Ctrl Pts',(186.981187167382,4.9177214713347,130.732259349382));
#205066=CARTESIAN_POINT('Ctrl Pts',(186.97343086464,4.91570944477649,130.595027557828));
#205067=CARTESIAN_POINT('Ctrl Pts',(186.965674561898,4.90794985542348,130.457952735076));
#205068=CARTESIAN_POINT('Ctrl Pts',(186.957918259156,4.89449441724326,130.321548581599));
#205069=CARTESIAN_POINT('Ctrl Pts',(186.950157816642,4.88103179749054,130.185071625118));
#205070=CARTESIAN_POINT('Ctrl Pts',(186.942397374128,4.8618673259655,130.04926643811));
#205071=CARTESIAN_POINT('Ctrl Pts',(186.934636931613,4.83710415268687,129.914637920003));
#205072=CARTESIAN_POINT('Ctrl Pts',(186.926864031348,4.81230122736411,129.779793284246));
#205073=CARTESIAN_POINT('Ctrl Pts',(186.919091131083,4.78188172714106,129.646129473437));
#205074=CARTESIAN_POINT('Ctrl Pts',(186.911318230817,4.74599935115195,129.514138457872));
#205075=CARTESIAN_POINT('Ctrl Pts',(186.903827895055,4.71142138991215,129.386945648188));
#205076=CARTESIAN_POINT('Ctrl Pts',(186.896337559293,4.67177092859245,129.261306418357));
#205077=CARTESIAN_POINT('Ctrl Pts',(186.888847223531,4.62722754114839,129.137642781537));
#205078=CARTESIAN_POINT('Ctrl Pts',(186.881072889412,4.58099527763089,129.00929040034));
#205079=CARTESIAN_POINT('Ctrl Pts',(186.873298555293,4.52934528322642,128.882659796889));
#205080=CARTESIAN_POINT('Ctrl Pts',(186.865524221174,4.47242470282503,128.758242258316));
#205081=CARTESIAN_POINT('Ctrl Pts',(186.857759468227,4.41557427195186,128.63397805324));
#205082=CARTESIAN_POINT('Ctrl Pts',(186.84999471528,4.35346634033301,128.511921838433));
#205083=CARTESIAN_POINT('Ctrl Pts',(186.842229962332,4.28629738038526,128.392548471191));
#205084=CARTESIAN_POINT('Ctrl Pts',(186.834472921447,4.21919513359548,128.27329366726));
#205085=CARTESIAN_POINT('Ctrl Pts',(186.826715880562,4.14704205228711,128.156716746663));
#205086=CARTESIAN_POINT('Ctrl Pts',(186.818958839677,4.07008197270261,128.04327101417));
#205087=CARTESIAN_POINT('Ctrl Pts',(186.811207648437,3.99317992931273,127.929910831987));
#205088=CARTESIAN_POINT('Ctrl Pts',(186.803456457197,3.91147832157752,127.81967746021));
#205089=CARTESIAN_POINT('Ctrl Pts',(186.795705265957,3.82526584664194,127.712997768431));
#205090=CARTESIAN_POINT('Ctrl Pts',(186.78795736918,3.739090014308,127.606363418365));
#205091=CARTESIAN_POINT('Ctrl Pts',(186.780209472403,3.64840737324212,127.503280047653));
#205092=CARTESIAN_POINT('Ctrl Pts',(186.772461575626,3.55354855977579,127.404143610401));
#205093=CARTESIAN_POINT('Ctrl Pts',(186.764715299542,3.45870958872832,127.305027910354));
#205094=CARTESIAN_POINT('Ctrl Pts',(186.756969023458,3.35969645297088,127.209857783879));
#205095=CARTESIAN_POINT('Ctrl Pts',(186.749222747373,3.25687823804013,127.11899398654));
#205096=CARTESIAN_POINT('Ctrl Pts',(186.741476414108,3.15405926412871,127.028129518465));
#205097=CARTESIAN_POINT('Ctrl Pts',(186.733730080843,3.04743544795587,126.941571701855));
#205098=CARTESIAN_POINT('Ctrl Pts',(186.725983747577,2.9374103889513,126.859642215781));
#205099=CARTESIAN_POINT('Ctrl Pts',(186.718235679574,2.82736069059759,126.777694382167));
#205100=CARTESIAN_POINT('Ctrl Pts',(186.710487611571,2.71390854726417,126.700377175026));
#205101=CARTESIAN_POINT('Ctrl Pts',(186.702739543568,2.5974877383432,126.627969769997));
#205102=CARTESIAN_POINT('Ctrl Pts',(186.694983240827,2.48094319600109,126.555485409516));
#205103=CARTESIAN_POINT('Ctrl Pts',(186.687226938085,2.36142401787533,126.487921481866));
#205104=CARTESIAN_POINT('Ctrl Pts',(186.679470635343,2.23939034738478,126.425512146274));
#205105=CARTESIAN_POINT('Ctrl Pts',(186.671710192829,2.11729154384987,126.36306950094));
#205106=CARTESIAN_POINT('Ctrl Pts',(186.663949750315,1.99267592883989,126.305787092796));
#205107=CARTESIAN_POINT('Ctrl Pts',(186.6561893078,1.86602404364675,126.253851049283));
#205108=CARTESIAN_POINT('Ctrl Pts',(186.648416407535,1.73916884560389,126.201831633423));
#205109=CARTESIAN_POINT('Ctrl Pts',(186.64064350727,1.6102712131062,126.155175865823));
#205110=CARTESIAN_POINT('Ctrl Pts',(186.632870607004,1.47982813283383,126.114020357012));
#205111=CARTESIAN_POINT('Ctrl Pts',(186.625380271242,1.35412698709598,126.074360954611));
#205112=CARTESIAN_POINT('Ctrl Pts',(186.61788993548,1.22699110189288,126.039808938046));
#205113=CARTESIAN_POINT('Ctrl Pts',(186.610399599718,1.09887259295406,126.010441335084));
#205114=CARTESIAN_POINT('Ctrl Pts',(186.602625265599,0.965896431807742,
125.979960250529));
#205115=CARTESIAN_POINT('Ctrl Pts',(186.59485093148,0.831440435162286,125.954967919335));
#205116=CARTESIAN_POINT('Ctrl Pts',(186.587076597361,0.695997472203889,
125.935606097036));
#205117=CARTESIAN_POINT('Ctrl Pts',(186.579311844414,0.560721430592498,
125.916268136452));
#205118=CARTESIAN_POINT('Ctrl Pts',(186.571547091467,0.424461226152909,
125.902546932818));
#205119=CARTESIAN_POINT('Ctrl Pts',(186.56378233852,0.287722567918223,125.894533860295));
#205120=CARTESIAN_POINT('Ctrl Pts',(186.556025297635,0.151119720446433,
125.886528746469));
#205121=CARTESIAN_POINT('Ctrl Pts',(186.54826825675,0.014039752633058,125.884220504122));
#205122=CARTESIAN_POINT('Ctrl Pts',(186.540511215865,-0.123004157933034,
125.887649009221));
#205123=CARTESIAN_POINT('Ctrl Pts',(186.532760024625,-0.259944722620193,
125.891074928858));
#205124=CARTESIAN_POINT('Ctrl Pts',(186.525008833384,-0.396848894920734,
125.90022897531));
#205125=CARTESIAN_POINT('Ctrl Pts',(186.517257642144,-0.533201489500632,
125.915098992935));
#205126=CARTESIAN_POINT('Ctrl Pts',(186.509509745367,-0.669496130590324,
125.929962690404));
#205127=CARTESIAN_POINT('Ctrl Pts',(186.50176184859,-0.805239272386058,
125.950537484778));
#205128=CARTESIAN_POINT('Ctrl Pts',(186.494013951813,-0.939919070470149,
125.976759225211));
#205129=CARTESIAN_POINT('Ctrl Pts',(186.486267675729,-1.07457069644382,
126.002975480622));
#205130=CARTESIAN_POINT('Ctrl Pts',(186.478521399645,-1.20815903761232,
126.034836257913));
#205131=CARTESIAN_POINT('Ctrl Pts',(186.470775123561,-1.34018108035477,
126.072226032164));
#205132=CARTESIAN_POINT('Ctrl Pts',(186.463028790295,-1.47220409765393,
126.109616082418));
#205133=CARTESIAN_POINT('Ctrl Pts',(186.45528245703,-1.60266041728542,126.152535104537));
#205134=CARTESIAN_POINT('Ctrl Pts',(186.447536123765,-1.73106124618654,
126.200817414288));
#205135=CARTESIAN_POINT('Ctrl Pts',(186.439788055762,-1.85949082956307,
126.249110536526));
#205136=CARTESIAN_POINT('Ctrl Pts',(186.432039987759,-1.98586364036161,
126.302769198807));
#205137=CARTESIAN_POINT('Ctrl Pts',(186.424291919756,-2.10971033185508,
126.361579351494));
#205138=CARTESIAN_POINT('Ctrl Pts',(186.416535617014,-2.23368864908604,
126.42045200831));
#205139=CARTESIAN_POINT('Ctrl Pts',(186.408779314272,-2.35513513012335,
126.484486924591));
#205140=CARTESIAN_POINT('Ctrl Pts',(186.40102301153,-2.47360405141956,126.553423537427));
#205141=CARTESIAN_POINT('Ctrl Pts',(186.393262569016,-2.59213620314615,
126.622396943809));
#205142=CARTESIAN_POINT('Ctrl Pts',(186.385502126502,-2.70768729925805,
126.696277049213));
#205143=CARTESIAN_POINT('Ctrl Pts',(186.377741683988,-2.81984100116167,
126.774760167066));
#205144=CARTESIAN_POINT('Ctrl Pts',(186.369968783722,-2.93217474214415,
126.853369272988));
#205145=CARTESIAN_POINT('Ctrl Pts',(186.362195883457,-3.04109987965048,
126.936595919761));
#205146=CARTESIAN_POINT('Ctrl Pts',(186.354422983192,-3.14623284593448,
127.024095819743));
#205147=CARTESIAN_POINT('Ctrl Pts',(186.346932647429,-3.24754396407987,
127.108414877961));
#205148=CARTESIAN_POINT('Ctrl Pts',(186.339442311667,-3.34533360559828,
127.196701689925));
#205149=CARTESIAN_POINT('Ctrl Pts',(186.331951975905,-3.43929258525454,
127.288617513255));
#205150=CARTESIAN_POINT('Ctrl Pts',(186.324290294265,-3.53540093236302,
127.382635965623));
#205151=CARTESIAN_POINT('Ctrl Pts',(186.316628612625,-3.62782449528663,
127.480768053431));
#205152=CARTESIAN_POINT('Ctrl Pts',(186.308966930984,-3.7161827594279,127.582688883663));
#205153=CARTESIAN_POINT('Ctrl Pts',(186.301314183386,-3.80443799181967,
127.68449086727));
#205154=CARTESIAN_POINT('Ctrl Pts',(186.293661435788,-3.88863708801042,
127.790072509402));
#205155=CARTESIAN_POINT('Ctrl Pts',(186.28600868819,-3.96843439155349,127.899070349377));
#205156=CARTESIAN_POINT('Ctrl Pts',(186.278363092695,-4.04815711815039,
128.007966322175));
#205157=CARTESIAN_POINT('Ctrl Pts',(186.2707174972,-4.12348599584845,128.120271821147));
#205158=CARTESIAN_POINT('Ctrl Pts',(186.263071901705,-4.19411426884116,
128.235588817191));
#205159=CARTESIAN_POINT('Ctrl Pts',(186.255431906839,-4.26469080449765,
128.350821340064));
#205160=CARTESIAN_POINT('Ctrl Pts',(186.247791911973,-4.33057337660585,
128.469060628456));
#205161=CARTESIAN_POINT('Ctrl Pts',(186.240151917107,-4.39149772261774,
128.589878552896));
#205162=CARTESIAN_POINT('Ctrl Pts',(186.232515226792,-4.45239571683195,
128.710644219582));
#205163=CARTESIAN_POINT('Ctrl Pts',(186.224878536477,-4.50833957015994,
128.833985944203));
#205164=CARTESIAN_POINT('Ctrl Pts',(186.217241846161,-4.5591105114303,128.959450211322));
#205165=CARTESIAN_POINT('Ctrl Pts',(186.209605532488,-4.60987894867488,
129.084908290537));
#205166=CARTESIAN_POINT('Ctrl Pts',(186.201969218815,-4.65547482316395,
129.212488333294));
#205167=CARTESIAN_POINT('Ctrl Pts',(186.194332905142,-4.695727286753,129.341716330344));
#205168=CARTESIAN_POINT('Ctrl Pts',(186.189625064471,-4.72054321146236,
129.421386292359));
#205169=CARTESIAN_POINT('Ctrl Pts',(186.184917223801,-4.74332916114695,
129.501682227587));
#205170=CARTESIAN_POINT('Ctrl Pts',(186.18020938313,-4.76405452823405,129.582490119308));
#205171=CARTESIAN_POINT('Ctrl Pts',(187.929867347344,-4.76405452823405,
129.582490119308));
#205172=CARTESIAN_POINT('Ctrl Pts',(187.921775086847,-4.79957275528882,
129.72097514753));
#205173=CARTESIAN_POINT('Ctrl Pts',(187.913682826349,-4.82908397265096,
129.861148571076));
#205174=CARTESIAN_POINT('Ctrl Pts',(187.905590565851,-4.85243842824599,
130.00247261879));
#205175=CARTESIAN_POINT('Ctrl Pts',(187.897511509163,-4.87575477733303,
130.143566073847));
#205176=CARTESIAN_POINT('Ctrl Pts',(187.889432452475,-4.8929343404035,130.285806076163));
#205177=CARTESIAN_POINT('Ctrl Pts',(187.881353395787,-4.90387800511191,
130.428643205833));
#205178=CARTESIAN_POINT('Ctrl Pts',(187.87428245186,-4.91345610840887,130.553656975815));
#205179=CARTESIAN_POINT('Ctrl Pts',(187.867211507934,-4.91825817656564,
130.679127798048));
#205180=CARTESIAN_POINT('Ctrl Pts',(187.860140564008,-4.91824998954378,
130.804681323973));
#205181=CARTESIAN_POINT('Origin',(213.235140564004,0.,130.804360617566));
#205182=CARTESIAN_POINT('',(189.680106903305,-4.76405452823404,129.582490119308));
#205183=CARTESIAN_POINT('',(189.334601801321,-4.76405452823404,129.582490119308));
#205184=CARTESIAN_POINT('',(213.235140564004,-4.76405452823405,129.582490119308));
#205185=CARTESIAN_POINT('',(189.264859435947,-4.91824989634823,130.805370355446));
#205186=CARTESIAN_POINT('Ctrl Pts',(189.334601801321,-4.76405452823404,
129.582490119308));
#205187=CARTESIAN_POINT('Ctrl Pts',(189.326589951379,-4.79924357938049,
129.71969169566));
#205188=CARTESIAN_POINT('Ctrl Pts',(189.318578101437,-4.82853357011572,
129.858539643826));
#205189=CARTESIAN_POINT('Ctrl Pts',(189.310566251495,-4.85178106031378,
129.99850479592));
#205190=CARTESIAN_POINT('Ctrl Pts',(189.302564129565,-4.8750003233392,130.138300001905));
#205191=CARTESIAN_POINT('Ctrl Pts',(189.294562007635,-4.89219165463957,
130.279209361064));
#205192=CARTESIAN_POINT('Ctrl Pts',(189.286559885705,-4.90326234654455,
130.420692240633));
#205193=CARTESIAN_POINT('Ctrl Pts',(189.279326402467,-4.91326965023596,
130.548585072909));
#205194=CARTESIAN_POINT('Ctrl Pts',(189.272092919229,-4.91827626236202,
130.676946189752));
#205195=CARTESIAN_POINT('Ctrl Pts',(189.264859435991,-4.91824989634839,
130.805370354665));
#205196=CARTESIAN_POINT('Ctrl Pts',(189.264859435947,-4.91824989634823,
130.805370355446));
#205197=CARTESIAN_POINT('Ctrl Pts',(189.256607171556,-4.91821981685867,
130.951882088204));
#205198=CARTESIAN_POINT('Ctrl Pts',(189.248354907165,-4.91163874752937,
131.098225889341));
#205199=CARTESIAN_POINT('Ctrl Pts',(189.240102642774,-4.89857698727829,
131.243822290761));
#205200=CARTESIAN_POINT('Ctrl Pts',(189.231428856725,-4.88484803865739,
131.396855685653));
#205201=CARTESIAN_POINT('Ctrl Pts',(189.222755070677,-4.86395906746465,
131.549062909309));
#205202=CARTESIAN_POINT('Ctrl Pts',(189.214081284629,-4.83605175230801,
131.699785941922));
#205203=CARTESIAN_POINT('Ctrl Pts',(189.205787676123,-4.80936763247221,
131.843902688434));
#205204=CARTESIAN_POINT('Ctrl Pts',(189.197494067618,-4.77626745182874,
131.986662328151));
#205205=CARTESIAN_POINT('Ctrl Pts',(189.189200459113,-4.73692581437122,
132.127507204926));
#205206=CARTESIAN_POINT('Ctrl Pts',(189.180893279678,-4.69751980172804,
132.268582547836));
#205207=CARTESIAN_POINT('Ctrl Pts',(189.172586100243,-4.65185203318383,
132.407736580464));
#205208=CARTESIAN_POINT('Ctrl Pts',(189.164278920808,-4.60014566525104,
132.544430421043));
#205209=CARTESIAN_POINT('Ctrl Pts',(189.155952232729,-4.54831786968213,
132.681445274498));
#205210=CARTESIAN_POINT('Ctrl Pts',(189.147625544649,-4.49042324122083,
132.815988102357));
#205211=CARTESIAN_POINT('Ctrl Pts',(189.139298856569,-4.42673210121107,
132.947541890022));
#205212=CARTESIAN_POINT('Ctrl Pts',(189.138204974444,-4.41836495704328,
132.964824191878));
#205213=CARTESIAN_POINT('Ctrl Pts',(189.137111092319,-4.40989783749088,
132.982054947649));
#205214=CARTESIAN_POINT('Ctrl Pts',(189.136017210193,-4.40133141131699,
132.99923302166));
#205215=CARTESIAN_POINT('Ctrl Pts',(189.128242876074,-4.34044892888366,
133.121319381593));
#205216=CARTESIAN_POINT('Ctrl Pts',(189.120468541955,-4.27438642335554,
133.241064014106));
#205217=CARTESIAN_POINT('Ctrl Pts',(189.112694207836,-4.20334731880043,
133.357996139725));
#205218=CARTESIAN_POINT('Ctrl Pts',(189.104929454889,-4.13239576359281,
133.47478415695));
#205219=CARTESIAN_POINT('Ctrl Pts',(189.097164701942,-4.05648001367186,
133.588766232983));
#205220=CARTESIAN_POINT('Ctrl Pts',(189.089399948995,-3.97585056850522,
133.699493657586));
#205221=CARTESIAN_POINT('Ctrl Pts',(189.08164290811,-3.8953012056402,133.81011110615));
#205222=CARTESIAN_POINT('Ctrl Pts',(189.073885867225,-3.81004769299365,
133.917480022228));
#205223=CARTESIAN_POINT('Ctrl Pts',(189.06612882634,-3.7203850578337,134.0211786236));
#205224=CARTESIAN_POINT('Ctrl Pts',(189.0583776351,-3.63079003796426,134.124799025051));
#205225=CARTESIAN_POINT('Ctrl Pts',(189.050626443859,-3.53679276837891,
134.224754326412));
#205226=CARTESIAN_POINT('Ctrl Pts',(189.042875252619,-3.43872974898933,
134.320654231006));
#205227=CARTESIAN_POINT('Ctrl Pts',(189.035127355842,-3.34070840899898,
134.416513375581));
#205228=CARTESIAN_POINT('Ctrl Pts',(189.027379459065,-3.23862503510299,
134.508320278819));
#205229=CARTESIAN_POINT('Ctrl Pts',(189.019631562288,-3.13285417567755,
134.595720238657));
#205230=CARTESIAN_POINT('Ctrl Pts',(189.011885286204,-3.02710544123581,
134.683101916308));
#205231=CARTESIAN_POINT('Ctrl Pts',(189.00413901012,-2.91767105670176,134.766078235263));
#205232=CARTESIAN_POINT('Ctrl Pts',(188.996392734036,-2.80495965334516,
134.844333935003));
#205233=CARTESIAN_POINT('Ctrl Pts',(188.98864640077,-2.69224741797864,134.922590212409));
#205234=CARTESIAN_POINT('Ctrl Pts',(188.980900067505,-2.57625843666835,
134.996125578092));
#205235=CARTESIAN_POINT('Ctrl Pts',(188.97315373424,-2.45743106294825,135.064667605725));
#205236=CARTESIAN_POINT('Ctrl Pts',(188.965405666237,-2.33857707866192,
135.13322498287));
#205237=CARTESIAN_POINT('Ctrl Pts',(188.957657598234,-2.21688377571787,
135.19678660152));
#205238=CARTESIAN_POINT('Ctrl Pts',(188.949909530231,-2.09281452597186,
135.255125767782));
#205239=CARTESIAN_POINT('Ctrl Pts',(188.942153227489,-1.96861341395046,
135.313526937605));
#205240=CARTESIAN_POINT('Ctrl Pts',(188.934396924747,-1.84203166516669,
135.366694400722));
#205241=CARTESIAN_POINT('Ctrl Pts',(188.926640622005,-1.71355358688341,
135.414449246582));
#205242=CARTESIAN_POINT('Ctrl Pts',(188.918880179491,-1.5850069359812,135.46222958064));
#205243=CARTESIAN_POINT('Ctrl Pts',(188.911119736977,-1.45456231049509,
135.504591420412));
#205244=CARTESIAN_POINT('Ctrl Pts',(188.903359294463,-1.3227186760497,135.541405937861));
#205245=CARTESIAN_POINT('Ctrl Pts',(188.895586394197,-1.19066339449785,
135.578279553241));
#205246=CARTESIAN_POINT('Ctrl Pts',(188.887813493932,-1.05720499698669,
135.609587961818));
#205247=CARTESIAN_POINT('Ctrl Pts',(188.880040593666,-0.922853008814749,
135.635253432214));
#205248=CARTESIAN_POINT('Ctrl Pts',(188.872550257904,-0.793385053824595,
135.659985898115));
#205249=CARTESIAN_POINT('Ctrl Pts',(188.865059922142,-0.663087653395633,
135.679478527407));
#205250=CARTESIAN_POINT('Ctrl Pts',(188.85756958638,-0.532418820732127,
135.693707533242));
#205251=CARTESIAN_POINT('Ctrl Pts',(188.849795252261,-0.396795639562776,
135.708476036158));
#205252=CARTESIAN_POINT('Ctrl Pts',(188.842020918142,-0.260342690980689,
135.717620678069));
#205253=CARTESIAN_POINT('Ctrl Pts',(188.834246584023,-0.123566010769087,
135.721058137597));
#205254=CARTESIAN_POINT('Ctrl Pts',(188.826481831076,0.0130421044082147,
135.724491360764));
#205255=CARTESIAN_POINT('Ctrl Pts',(188.818717078129,0.149972770293301,
135.722231386573));
#205256=CARTESIAN_POINT('Ctrl Pts',(188.810952325181,0.28671307317168,135.714246428476));
#205257=CARTESIAN_POINT('Ctrl Pts',(188.803195284296,0.423317563653494,
135.706269401151));
#205258=CARTESIAN_POINT('Ctrl Pts',(188.795438243411,0.559731679614168,
135.692578728228));
#205259=CARTESIAN_POINT('Ctrl Pts',(188.787681202526,0.695441094281352,
135.673194640911));
#205260=CARTESIAN_POINT('Ctrl Pts',(188.779930011286,0.8310481694232,135.653825171285));
#205261=CARTESIAN_POINT('Ctrl Pts',(188.772178820046,0.965951215561337,
135.628770888172));
#205262=CARTESIAN_POINT('Ctrl Pts',(188.764427628806,1.09963997862434,135.598103933589));
#205263=CARTESIAN_POINT('Ctrl Pts',(188.756679732029,1.23327192039691,135.567450013279));
#205264=CARTESIAN_POINT('Ctrl Pts',(188.748931835252,1.36569022531323,135.531188253377));
#205265=CARTESIAN_POINT('Ctrl Pts',(188.741183938475,1.49639401993704,135.489442046911));
#205266=CARTESIAN_POINT('Ctrl Pts',(188.733437662391,1.62707047414466,135.447704572852));
#205267=CARTESIAN_POINT('Ctrl Pts',(188.725691386307,1.75603275921754,135.400485053005));
#205268=CARTESIAN_POINT('Ctrl Pts',(188.717945110223,1.88279476236884,135.34795687442));
#205269=CARTESIAN_POINT('Ctrl Pts',(188.710198776957,2.00955770124844,135.295428308083));
#205270=CARTESIAN_POINT('Ctrl Pts',(188.702452443692,2.13411996461381,135.237591154481));
#205271=CARTESIAN_POINT('Ctrl Pts',(188.694706110426,2.25601541168853,135.174666959772));
#205272=CARTESIAN_POINT('Ctrl Pts',(188.686958042423,2.3779381564034,135.111728673626));
#205273=CARTESIAN_POINT('Ctrl Pts',(188.679209974421,2.4971925490977,135.043701258784));
#205274=CARTESIAN_POINT('Ctrl Pts',(188.671461906418,2.61333740197348,134.970852029527));
#205275=CARTESIAN_POINT('Ctrl Pts',(188.663705603676,2.72960569498105,134.897925375242));
#205276=CARTESIAN_POINT('Ctrl Pts',(188.655949300934,2.84275751463042,134.820166877511));
#205277=CARTESIAN_POINT('Ctrl Pts',(188.648192998192,2.95238055850332,134.737887292227));
#205278=CARTESIAN_POINT('Ctrl Pts',(188.640432555678,3.06206211149548,134.655563791851));
#205279=CARTESIAN_POINT('Ctrl Pts',(188.632672113164,3.1682108334075,134.568714643188));
#205280=CARTESIAN_POINT('Ctrl Pts',(188.62491167065,3.27044863445584,134.477690005449));
#205281=CARTESIAN_POINT('Ctrl Pts',(188.617138770384,3.37285055669868,134.386519246881));
#205282=CARTESIAN_POINT('Ctrl Pts',(188.609365870119,3.47132873129138,134.291159876902));
#205283=CARTESIAN_POINT('Ctrl Pts',(188.601592969853,3.5655423497568,134.191998557871));
#205284=CARTESIAN_POINT('Ctrl Pts',(188.594102634091,3.65633106588129,134.096442002558));
#205285=CARTESIAN_POINT('Ctrl Pts',(188.586612298329,3.74315969458697,133.997355351629));
#205286=CARTESIAN_POINT('Ctrl Pts',(188.579121962567,3.82576065600049,133.895111087193));
#205287=CARTESIAN_POINT('Ctrl Pts',(188.571347628448,3.91149345797192,133.788990200394));
#205288=CARTESIAN_POINT('Ctrl Pts',(188.563573294329,3.99294325595813,133.679131372527));
#205289=CARTESIAN_POINT('Ctrl Pts',(188.55579896021,4.06976642462402,133.565915308588));
#205290=CARTESIAN_POINT('Ctrl Pts',(188.548034207263,4.14649491560041,133.452838773329));
#205291=CARTESIAN_POINT('Ctrl Pts',(188.540269454316,4.21860790493604,133.336413554789));
#205292=CARTESIAN_POINT('Ctrl Pts',(188.532504701369,4.28580140731598,133.217054000395));
#205293=CARTESIAN_POINT('Ctrl Pts',(188.524747660484,4.35292817216208,133.097812995594));
#205294=CARTESIAN_POINT('Ctrl Pts',(188.516990619599,4.41514498306898,132.97564379326));
#205295=CARTESIAN_POINT('Ctrl Pts',(188.509233578714,4.47219085493765,132.850990046533));
#205296=CARTESIAN_POINT('Ctrl Pts',(188.501482387474,4.52919370807062,132.726430302165));
#205297=CARTESIAN_POINT('Ctrl Pts',(188.493731196234,4.58103322174094,132.599390096789));
#205298=CARTESIAN_POINT('Ctrl Pts',(188.485980004993,4.6274942862818,132.470337716127));
#205299=CARTESIAN_POINT('Ctrl Pts',(188.478232108216,4.67393560363083,132.341340186169));
#205300=CARTESIAN_POINT('Ctrl Pts',(188.470484211439,4.71500288634316,132.210332548992));
#205301=CARTESIAN_POINT('Ctrl Pts',(188.462736314662,4.75052921414137,132.077802900549));
#205302=CARTESIAN_POINT('Ctrl Pts',(188.454990038578,4.78604811059766,131.945300974451));
#205303=CARTESIAN_POINT('Ctrl Pts',(188.447243762494,4.81602825638518,131.81127804774));
#205304=CARTESIAN_POINT('Ctrl Pts',(188.43949748641,4.84035277110316,131.676236820805));
#205305=CARTESIAN_POINT('Ctrl Pts',(188.431751153145,4.86467746537918,131.541194597026));
#205306=CARTESIAN_POINT('Ctrl Pts',(188.424004819879,4.88334637597157,131.405134442797));
#205307=CARTESIAN_POINT('Ctrl Pts',(188.416258486614,4.89629393546274,131.268568286666));
#205308=CARTESIAN_POINT('Ctrl Pts',(188.408510418611,4.90924439447009,131.13197154749));
#205309=CARTESIAN_POINT('Ctrl Pts',(188.400762350608,4.91647091592922,130.994868970073));
#205310=CARTESIAN_POINT('Ctrl Pts',(188.393014282605,4.91795992613311,130.857776228101));
#205311=CARTESIAN_POINT('Ctrl Pts',(188.385257979863,4.91945051887476,130.720537782331));
#205312=CARTESIAN_POINT('Ctrl Pts',(188.377501677121,4.91519141490565,130.583309584453));
#205313=CARTESIAN_POINT('Ctrl Pts',(188.36974537438,4.90522120243238,130.44660648732));
#205314=CARTESIAN_POINT('Ctrl Pts',(188.361984931865,4.89524566855652,130.309830427629));
#205315=CARTESIAN_POINT('Ctrl Pts',(188.354224489351,4.87955299711073,130.173580415335));
#205316=CARTESIAN_POINT('Ctrl Pts',(188.346464046837,4.85823342019293,130.03836381769));
#205317=CARTESIAN_POINT('Ctrl Pts',(188.338691146572,4.8368796191976,129.902930158358));
#205318=CARTESIAN_POINT('Ctrl Pts',(188.330918246306,4.80988093934744,129.768533612271));
#205319=CARTESIAN_POINT('Ctrl Pts',(188.323145346041,4.77737847532777,129.635669911701));
#205320=CARTESIAN_POINT('Ctrl Pts',(188.315655010279,4.74605755774389,129.50763614131));
#205321=CARTESIAN_POINT('Ctrl Pts',(188.308164674517,4.70962614676043,129.381026001712));
#205322=CARTESIAN_POINT('Ctrl Pts',(188.300674338755,4.66825298866656,129.256265951111));
#205323=CARTESIAN_POINT('Ctrl Pts',(188.292900004636,4.62531115470858,129.126775585272));
#205324=CARTESIAN_POINT('Ctrl Pts',(188.285125670517,4.57690941679345,128.998868183534));
#205325=CARTESIAN_POINT('Ctrl Pts',(188.277351336398,4.52318233493014,128.873038627975));
#205326=CARTESIAN_POINT('Ctrl Pts',(188.269586583451,4.46952146689349,128.747364146098));
#205327=CARTESIAN_POINT('Ctrl Pts',(188.261821830503,4.41054846539562,128.623762771359));
#205328=CARTESIAN_POINT('Ctrl Pts',(188.254057077556,4.34644762117504,128.502714220119));
#205329=CARTESIAN_POINT('Ctrl Pts',(188.246300036671,4.28241044281667,128.381785896006));
#205330=CARTESIAN_POINT('Ctrl Pts',(188.238542995786,4.21325573890659,128.263405692909));
#205331=CARTESIAN_POINT('Ctrl Pts',(188.230785954901,4.13921569857526,128.148032990339));
#205332=CARTESIAN_POINT('Ctrl Pts',(188.223034763661,4.06523149241429,128.032747291222));
#205333=CARTESIAN_POINT('Ctrl Pts',(188.215283572421,3.98636949305475,127.920464906065));
#205334=CARTESIAN_POINT('Ctrl Pts',(188.207532381181,3.90290741050956,127.811619932594));
#205335=CARTESIAN_POINT('Ctrl Pts',(188.199784484404,3.81948080157582,127.702821221139));
#205336=CARTESIAN_POINT('Ctrl Pts',(188.192036587627,3.73145823551986,127.597457325174));
#205337=CARTESIAN_POINT('Ctrl Pts',(188.18428869085,3.63916013680356,127.495932507239));
#205338=CARTESIAN_POINT('Ctrl Pts',(188.176542414766,3.54688134485975,127.394428926108));
#205339=CARTESIAN_POINT('Ctrl Pts',(188.168796138682,3.45032906199472,127.296763114795));
#205340=CARTESIAN_POINT('Ctrl Pts',(188.161049862597,3.34986304757216,127.203305129933));
#205341=CARTESIAN_POINT('Ctrl Pts',(188.153303529332,3.24939629153235,127.109846455185));
#205342=CARTESIAN_POINT('Ctrl Pts',(188.145557196067,3.14501603254435,127.020595935158));
#205343=CARTESIAN_POINT('Ctrl Pts',(188.137810862801,3.03711752980305,126.935885443461));
#205344=CARTESIAN_POINT('Ctrl Pts',(188.130062794798,2.92919486394014,126.851155981437));
#205345=CARTESIAN_POINT('Ctrl Pts',(188.122314726795,2.81775269397828,126.770968812257));
#205346=CARTESIAN_POINT('Ctrl Pts',(188.114566658792,2.703217533875,126.695614090089));
#205347=CARTESIAN_POINT('Ctrl Pts',(188.106810356051,2.58856064444062,126.620179280026));
#205348=CARTESIAN_POINT('Ctrl Pts',(188.099054053309,2.47080452533179,126.549587391881));
#205349=CARTESIAN_POINT('Ctrl Pts',(188.091297750567,2.35040319470329,126.484084250847));
#205350=CARTESIAN_POINT('Ctrl Pts',(188.083537308053,2.22993760225931,126.418546148814));
#205351=CARTESIAN_POINT('Ctrl Pts',(188.075776865539,2.10682433588469,126.358102378005));
#205352=CARTESIAN_POINT('Ctrl Pts',(188.068016423024,1.98153903066888,126.302951267992));
#205353=CARTESIAN_POINT('Ctrl Pts',(188.060243522759,1.85605260635887,126.24771162452));
#205354=CARTESIAN_POINT('Ctrl Pts',(188.052470622493,1.72838753988925,126.197781762542));
#205355=CARTESIAN_POINT('Ctrl Pts',(188.044697722228,1.59903716998487,126.153310930505));
#205356=CARTESIAN_POINT('Ctrl Pts',(188.037207386466,1.47438901184074,126.110456725228));
#205357=CARTESIAN_POINT('Ctrl Pts',(188.029717050704,1.34817624808902,126.072671630003));
#205358=CARTESIAN_POINT('Ctrl Pts',(188.022226714942,1.22084888158536,126.040044184873));
#205359=CARTESIAN_POINT('Ctrl Pts',(188.014452380823,1.08869385928014,126.006179660243));
#205360=CARTESIAN_POINT('Ctrl Pts',(188.006678046704,0.954919418051348,
125.977764338209));
#205361=CARTESIAN_POINT('Ctrl Pts',(187.998903712585,0.820014649177363,
125.954952505473));
#205362=CARTESIAN_POINT('Ctrl Pts',(187.991138959638,0.685276138374253,
125.932168786282));
#205363=CARTESIAN_POINT('Ctrl Pts',(187.98337420669,0.54941045342816,125.914974880467));
#205364=CARTESIAN_POINT('Ctrl Pts',(187.975609453743,0.412920806945482,
125.903475037419));
#205365=CARTESIAN_POINT('Ctrl Pts',(187.967852412858,0.276566723903787,
125.891986616178));
#205366=CARTESIAN_POINT('Ctrl Pts',(187.960095371973,0.139590299674858,
125.886181035769));
#205367=CARTESIAN_POINT('Ctrl Pts',(187.952338331088,0.00250352715083474,
125.886111254749));
#205368=CARTESIAN_POINT('Ctrl Pts',(187.944587139848,-0.134479867171555,
125.886041526351));
#205369=CARTESIAN_POINT('Ctrl Pts',(187.936835948608,-0.271573054772387,
125.891698988073));
#205370=CARTESIAN_POINT('Ctrl Pts',(187.929084757368,-0.408260707894014,
125.90308463504));
#205371=CARTESIAN_POINT('Ctrl Pts',(187.921336860591,-0.544890265116803,
125.914465442803));
#205372=CARTESIAN_POINT('Ctrl Pts',(187.913588963814,-0.681114241876996,
125.931569561129));
#205373=CARTESIAN_POINT('Ctrl Pts',(187.905841067037,-0.816419323400283,
125.954345921621));
#205374=CARTESIAN_POINT('Ctrl Pts',(187.898094790952,-0.951696102017355,
125.977117517791));
#205375=CARTESIAN_POINT('Ctrl Pts',(187.890348514868,-1.08605398242313,
126.005558931233));
#205376=CARTESIAN_POINT('Ctrl Pts',(187.882602238784,-1.21898716676947,
126.039567510856));
#205377=CARTESIAN_POINT('Ctrl Pts',(187.874855905519,-1.35192133239828,
126.073576341522));
#205378=CARTESIAN_POINT('Ctrl Pts',(187.867109572253,-1.48343040221569,
126.113152323472));
#205379=CARTESIAN_POINT('Ctrl Pts',(187.859363238988,-1.61302151430496,
126.158142299741));
#205380=CARTESIAN_POINT('Ctrl Pts',(187.851615170985,-1.74264164742518,
126.203142351204));
#205381=CARTESIAN_POINT('Ctrl Pts',(187.843867102982,-1.87034259886549,
126.253558681377));
#205382=CARTESIAN_POINT('Ctrl Pts',(187.836119034979,-1.99564971249439,
126.309189287403));
#205383=CARTESIAN_POINT('Ctrl Pts',(187.828362732237,-2.12109000401499,
126.364879018299));
#205384=CARTESIAN_POINT('Ctrl Pts',(187.820606429495,-2.24413101750869,
126.425793936487));
#205385=CARTESIAN_POINT('Ctrl Pts',(187.812850126754,-2.36432052537678,
126.491684938155));
#205386=CARTESIAN_POINT('Ctrl Pts',(187.805089684239,-2.48457418200409,
126.557611107835));
#205387=CARTESIAN_POINT('Ctrl Pts',(187.797329241725,-2.60197296592657,
126.628518451041));
#205388=CARTESIAN_POINT('Ctrl Pts',(187.789568799211,-2.71609292447437,
126.70411400448));
#205389=CARTESIAN_POINT('Ctrl Pts',(187.781795898946,-2.83039607851072,
126.779830910613));
#205390=CARTESIAN_POINT('Ctrl Pts',(187.77402299868,-2.94140957229936,126.860250836692));
#205391=CARTESIAN_POINT('Ctrl Pts',(187.766250098415,-3.04874117726313,
126.945039395309));
#205392=CARTESIAN_POINT('Ctrl Pts',(187.758759762653,-3.15217100803496,
127.026745676251));
#205393=CARTESIAN_POINT('Ctrl Pts',(187.751269426891,-3.25218176050425,
127.112508282006));
#205394=CARTESIAN_POINT('Ctrl Pts',(187.743779091128,-3.34845570588935,
127.201996470482));
#205395=CARTESIAN_POINT('Ctrl Pts',(187.736122099101,-3.44687169893981,
127.293475726888));
#205396=CARTESIAN_POINT('Ctrl Pts',(187.728465107073,-3.54171430929935,
127.389156956171));
#205397=CARTESIAN_POINT('Ctrl Pts',(187.720808115045,-3.63259513007057,
127.488725582842));
#205398=CARTESIAN_POINT('Ctrl Pts',(187.713159991201,-3.72337069438334,
127.588178891002));
#205399=CARTESIAN_POINT('Ctrl Pts',(187.705511867358,-3.81019332122524,
127.691510351903));
#205400=CARTESIAN_POINT('Ctrl Pts',(187.697863743514,-3.8927084393723,127.798365928858));
#205401=CARTESIAN_POINT('Ctrl Pts',(187.690222703422,-3.97514713137943,
127.905122535353));
#205402=CARTESIAN_POINT('Ctrl Pts',(187.68258166333,-4.05328600255709,128.015396450587));
#205403=CARTESIAN_POINT('Ctrl Pts',(187.674940623237,-4.12680846773921,
128.1287980724));
#205404=CARTESIAN_POINT('Ctrl Pts',(187.667304890307,-4.2002798671441,128.242120929961));
#205405=CARTESIAN_POINT('Ctrl Pts',(187.659669157377,-4.26914101941565,
128.358566835824));
#205406=CARTESIAN_POINT('Ctrl Pts',(187.652033424447,-4.33311701410075,
128.47771496242));
#205407=CARTESIAN_POINT('Ctrl Pts',(187.6444009553,-4.39706566317769,128.596812160883));
#205408=CARTESIAN_POINT('Ctrl Pts',(187.636768486153,-4.45613311784616,
128.718608927462));
#205409=CARTESIAN_POINT('Ctrl Pts',(187.629136017006,-4.5100892971886,128.842657889351));
#205410=CARTESIAN_POINT('Ctrl Pts',(187.621503159863,-4.56404821939219,
128.966713157266));
#205411=CARTESIAN_POINT('Ctrl Pts',(187.613870302719,-4.61289517533641,
129.093020483825));
#205412=CARTESIAN_POINT('Ctrl Pts',(187.606237445576,-4.65644742360532,
129.221110651926));
#205413=CARTESIAN_POINT('Ctrl Pts',(187.599143290485,-4.69692589686468,
129.340160635574));
#205414=CARTESIAN_POINT('Ctrl Pts',(187.592049135395,-4.73283104437265,
129.460750229615));
#205415=CARTESIAN_POINT('Ctrl Pts',(187.584954980304,-4.76405452823404,
129.582490119308));
#205416=CARTESIAN_POINT('',(189.610140563969,-4.91824791299378,130.799829742121));
#205417=CARTESIAN_POINT('Ctrl Pts',(189.610140563969,-4.91824791299378,
130.799829742121));
#205418=CARTESIAN_POINT('Ctrl Pts',(189.602485915437,-4.91837237034752,
130.934927722133));
#205419=CARTESIAN_POINT('Ctrl Pts',(189.594831266904,-4.91292619023357,
131.070187999666));
#205420=CARTESIAN_POINT('Ctrl Pts',(189.587176618372,-4.90189607666226,
131.205107315747));
#205421=CARTESIAN_POINT('Ctrl Pts',(189.57916408585,-4.89035026324752,131.346334624011));
#205422=CARTESIAN_POINT('Ctrl Pts',(189.571151553328,-4.87268569848204,
131.487187873076));
#205423=CARTESIAN_POINT('Ctrl Pts',(189.563139020806,-4.84894837207892,
131.627089459538));
#205424=CARTESIAN_POINT('Ctrl Pts',(189.555493068658,-4.82629704912697,
131.760590426017));
#205425=CARTESIAN_POINT('Ctrl Pts',(189.547847116509,-4.79811638583712,
131.893224434576));
#205426=CARTESIAN_POINT('Ctrl Pts',(189.54020116436,-4.76449933419752,132.02449551049));
#205427=CARTESIAN_POINT('Ctrl Pts',(189.532556401308,-4.73088751067271,
132.155746171162));
#205428=CARTESIAN_POINT('Ctrl Pts',(189.524911638256,-4.69184107950793,
132.285633931062));
#205429=CARTESIAN_POINT('Ctrl Pts',(189.517266875204,-4.64750370934258,
132.413674861009));
#205430=CARTESIAN_POINT('Ctrl Pts',(189.509621542448,-4.60316303506545,
132.541725332827));
#205431=CARTESIAN_POINT('Ctrl Pts',(189.501976209692,-4.55353076963928,
132.667928320977));
#205432=CARTESIAN_POINT('Ctrl Pts',(189.494330876936,-4.49879968865441,
132.791817390395));
#205433=CARTESIAN_POINT('Ctrl Pts',(189.486683215447,-4.44405193682891,
132.915744195865));
#205434=CARTESIAN_POINT('Ctrl Pts',(189.479035553957,-4.38420244384357,
133.037355313473));
#205435=CARTESIAN_POINT('Ctrl Pts',(189.471387892468,-4.31949088284538,
133.156207035918));
#205436=CARTESIAN_POINT('Ctrl Pts',(189.46373199972,-4.25470967211568,133.275186679718));
#205437=CARTESIAN_POINT('Ctrl Pts',(189.456076106972,-4.18505614095032,
133.39140064717));
#205438=CARTESIAN_POINT('Ctrl Pts',(189.448420214224,-4.11081455193053,
133.504432242937));
#205439=CARTESIAN_POINT('Ctrl Pts',(189.440759493914,-4.0365261485234,133.617535112838));
#205440=CARTESIAN_POINT('Ctrl Pts',(189.433098773603,-3.95764416228724,
133.727451290957));
#205441=CARTESIAN_POINT('Ctrl Pts',(189.425438053292,-3.87449360985302,
133.833796593075));
#205442=CARTESIAN_POINT('Ctrl Pts',(189.417766480026,-3.79122525788974,
133.940292554763));
#205443=CARTESIAN_POINT('Ctrl Pts',(189.41009490676,-3.70367653135893,134.043207240323));
#205444=CARTESIAN_POINT('Ctrl Pts',(189.402423333494,-3.61220996172295,
134.142192586813));
#205445=CARTESIAN_POINT('Ctrl Pts',(189.399907501612,-3.58221422237703,
134.174654049665));
#205446=CARTESIAN_POINT('Ctrl Pts',(189.397391669729,-3.55179740394281,
134.206693246693));
#205447=CARTESIAN_POINT('Ctrl Pts',(189.394875837847,-3.52097305098158,
134.238298857657));
#205448=CARTESIAN_POINT('Ctrl Pts',(189.387101503728,-3.42572073281059,
134.335965391495));
#205449=CARTESIAN_POINT('Ctrl Pts',(189.379327169609,-3.32625077645834,
134.429820383029));
#205450=CARTESIAN_POINT('Ctrl Pts',(189.37155283549,-3.22290063708545,134.519477647482));
#205451=CARTESIAN_POINT('Ctrl Pts',(189.363788082543,-3.11967786752259,
134.609024417371));
#205452=CARTESIAN_POINT('Ctrl Pts',(189.356023329596,-3.01258472214135,
134.694383499813));
#205453=CARTESIAN_POINT('Ctrl Pts',(189.348258576648,-2.90199674489212,
134.775204099137));
#205454=CARTESIAN_POINT('Ctrl Pts',(189.340501535763,-2.79151860518099,
134.855944426302));
#205455=CARTESIAN_POINT('Ctrl Pts',(189.332744494878,-2.67755285489058,
134.932155011651));
#205456=CARTESIAN_POINT('Ctrl Pts',(189.324987453993,-2.56050921726351,
135.003524297492));
#205457=CARTESIAN_POINT('Ctrl Pts',(189.317236262753,-2.44355384315431,
135.074839763199));
#205458=CARTESIAN_POINT('Ctrl Pts',(189.309485071513,-2.32352553408762,
135.141320993499));
#205459=CARTESIAN_POINT('Ctrl Pts',(189.301733880273,-2.20086389176815,
135.202699075713));
#205460=CARTESIAN_POINT('Ctrl Pts',(189.293985983496,-2.07825438391844,
135.264051070604));
#205461=CARTESIAN_POINT('Ctrl Pts',(189.286238086719,-1.95301411779677,
135.320304056746));
#205462=CARTESIAN_POINT('Ctrl Pts',(189.278490189942,-1.82560805826677,
135.371234633793));
#205463=CARTESIAN_POINT('Ctrl Pts',(189.270743913858,-1.69822864933794,
135.422154557262));
#205464=CARTESIAN_POINT('Ctrl Pts',(189.262997637774,-1.56868471092015,
135.467754141087));
#205465=CARTESIAN_POINT('Ctrl Pts',(189.255251361689,-1.43746162023923,
135.507857949641));
#205466=CARTESIAN_POINT('Ctrl Pts',(189.247505028424,-1.3062375608992,135.547962054233));
#205467=CARTESIAN_POINT('Ctrl Pts',(189.239758695159,-1.1733346984564,135.582570188336));
#205468=CARTESIAN_POINT('Ctrl Pts',(189.232012361893,-1.03925363421513,
135.611556780224));
#205469=CARTESIAN_POINT('Ctrl Pts',(189.22426429389,-0.905142543449059,
135.640549863458));
#205470=CARTESIAN_POINT('Ctrl Pts',(189.216516225887,-0.76985310791742,
135.663918816804));
#205471=CARTESIAN_POINT('Ctrl Pts',(189.208768157884,-0.633895788762408,
135.681589255993));
#205472=CARTESIAN_POINT('Ctrl Pts',(189.201011855143,-0.497793972550918,
135.699278475534));
#205473=CARTESIAN_POINT('Ctrl Pts',(189.193255552401,-0.361023243067375,
135.711257032039));
#205474=CARTESIAN_POINT('Ctrl Pts',(189.185499249659,-0.224099407142775,
135.717502435));
#205475=CARTESIAN_POINT('Ctrl Pts',(189.177738807145,-0.0871024908441983,
135.723751171321));
#205476=CARTESIAN_POINT('Ctrl Pts',(189.16997836463,0.0500473039532961,
135.724260655423));
#205477=CARTESIAN_POINT('Ctrl Pts',(189.162217922116,0.186835504032796,
135.719060563334));
#205478=CARTESIAN_POINT('Ctrl Pts',(189.154445021851,0.323843288674548,
135.713852123596));
#205479=CARTESIAN_POINT('Ctrl Pts',(189.146672121585,0.46048792870308,135.702915823248));
#205480=CARTESIAN_POINT('Ctrl Pts',(189.13889922132,0.596260497125072,135.686333219094));
#205481=CARTESIAN_POINT('Ctrl Pts',(189.131408885558,0.727097390693978,
135.67035343437));
#205482=CARTESIAN_POINT('Ctrl Pts',(189.123918549796,0.857124211873021,
135.649130783049));
#205483=CARTESIAN_POINT('Ctrl Pts',(189.116428214034,0.985897556969896,
135.622782461869));
#205484=CARTESIAN_POINT('Ctrl Pts',(189.108653879915,1.11955338258629,135.595435136084));
#205485=CARTESIAN_POINT('Ctrl Pts',(189.100879545796,1.25228218617169,135.562479160128));
#205486=CARTESIAN_POINT('Ctrl Pts',(189.093105211677,1.38357665678069,135.523989702284));
#205487=CARTESIAN_POINT('Ctrl Pts',(189.08534045873,1.51470931868909,135.485547679256));
#205488=CARTESIAN_POINT('Ctrl Pts',(189.077575705783,1.64441079321712,135.441585852083));
#205489=CARTESIAN_POINT('Ctrl Pts',(189.069810952835,1.7721829553513,135.392230562896));
#205490=CARTESIAN_POINT('Ctrl Pts',(189.06205391195,1.89982821237275,135.342924294078));
#205491=CARTESIAN_POINT('Ctrl Pts',(189.054296871065,2.02554760802274,135.288235363609));
#205492=CARTESIAN_POINT('Ctrl Pts',(189.04653983018,2.14885755457138,135.228340078714));
#205493=CARTESIAN_POINT('Ctrl Pts',(189.03878863894,2.2720745121302,135.16848996132));
#205494=CARTESIAN_POINT('Ctrl Pts',(189.0310374477,2.39288528693343,135.103441474395));
#205495=CARTESIAN_POINT('Ctrl Pts',(189.02328625646,2.51082601966835,135.033419113432));
#205496=CARTESIAN_POINT('Ctrl Pts',(189.015538359683,2.62871662444556,134.963426513841));
#205497=CARTESIAN_POINT('Ctrl Pts',(189.007790462906,2.7437392778564,134.888464444029));
#205498=CARTESIAN_POINT('Ctrl Pts',(189.000042566129,2.85545470199736,134.808803338762));
#205499=CARTESIAN_POINT('Ctrl Pts',(188.992296290045,2.96714675767976,134.729158896881));
#205500=CARTESIAN_POINT('Ctrl Pts',(188.984550013961,3.07553264200004,134.644817601504));
#205501=CARTESIAN_POINT('Ctrl Pts',(188.976803737876,3.18020239775109,134.556092986997));
#205502=CARTESIAN_POINT('Ctrl Pts',(188.969057404611,3.28487292615045,134.467367717545));
#205503=CARTESIAN_POINT('Ctrl Pts',(188.961311071346,3.38582697300727,134.374259317201));
#205504=CARTESIAN_POINT('Ctrl Pts',(188.95356473808,3.48268830403982,134.277121081434));
#205505=CARTESIAN_POINT('Ctrl Pts',(188.945816670077,3.57957132649582,134.179961092233));
#205506=CARTESIAN_POINT('Ctrl Pts',(188.938068602074,3.67235953332192,134.078769748627));
#205507=CARTESIAN_POINT('Ctrl Pts',(188.930320534071,3.76071442620922,133.973936309516));
#205508=CARTESIAN_POINT('Ctrl Pts',(188.92256423133,3.8491632237282,133.868991452179));
#205509=CARTESIAN_POINT('Ctrl Pts',(188.914807928588,3.93316904266262,133.7603970663));
#205510=CARTESIAN_POINT('Ctrl Pts',(188.907051625846,4.01243415492057,133.648574958105));
#205511=CARTESIAN_POINT('Ctrl Pts',(188.899291183332,4.09174157335567,133.536693167084));
#205512=CARTESIAN_POINT('Ctrl Pts',(188.891530740818,4.16630303091852,133.421580549039));
#205513=CARTESIAN_POINT('Ctrl Pts',(188.883770298303,4.23586540955038,133.303685985475));
#205514=CARTESIAN_POINT('Ctrl Pts',(188.875997398038,4.30553945588784,133.185602167092));
#205515=CARTESIAN_POINT('Ctrl Pts',(188.868224497773,4.37019820233963,133.064727823987));
#205516=CARTESIAN_POINT('Ctrl Pts',(188.860451597507,4.42963517748233,132.941535214297));
#205517=CARTESIAN_POINT('Ctrl Pts',(188.852961261745,4.48691146886592,132.822820966272));
#205518=CARTESIAN_POINT('Ctrl Pts',(188.845470925983,4.53933892418261,132.701954357632));
#205519=CARTESIAN_POINT('Ctrl Pts',(188.837980590221,4.58677647383961,132.579371784159));
#205520=CARTESIAN_POINT('Ctrl Pts',(188.830206256102,4.63601263261018,132.452141455156));
#205521=CARTESIAN_POINT('Ctrl Pts',(188.822431921983,4.68002899709644,132.322659443626));
#205522=CARTESIAN_POINT('Ctrl Pts',(188.814657587864,4.7186145945435,132.191393194927));
#205523=CARTESIAN_POINT('Ctrl Pts',(188.806892834917,4.75715263869014,132.060288720149));
#205524=CARTESIAN_POINT('Ctrl Pts',(188.79912808197,4.79027312354286,131.927404754878));
#205525=CARTESIAN_POINT('Ctrl Pts',(188.791363329022,4.8178130955777,131.793228676803));
#205526=CARTESIAN_POINT('Ctrl Pts',(188.783606288137,4.84532571452407,131.659185864302));
#205527=CARTESIAN_POINT('Ctrl Pts',(188.775849247252,4.86726877266508,131.523853873413));
#205528=CARTESIAN_POINT('Ctrl Pts',(188.768092206367,4.88352921128275,131.387734858554));
#205529=CARTESIAN_POINT('Ctrl Pts',(188.760341015127,4.89977738777712,131.251718492103));
#205530=CARTESIAN_POINT('Ctrl Pts',(188.752589823887,4.91035142820668,131.114916669642));
#205531=CARTESIAN_POINT('Ctrl Pts',(188.744838632647,4.91518947969835,130.977840994447));
#205532=CARTESIAN_POINT('Ctrl Pts',(188.73709073587,4.9200254748891,130.840823580069));
#205533=CARTESIAN_POINT('Ctrl Pts',(188.729342839093,4.91913031627366,130.70353293436));
#205534=CARTESIAN_POINT('Ctrl Pts',(188.721594942316,4.91249408784202,130.566484810858));
#205535=CARTESIAN_POINT('Ctrl Pts',(188.713848666232,4.90585924756631,130.429465354868));
#205536=CARTESIAN_POINT('Ctrl Pts',(188.706102390148,4.89348574504375,130.29268871044));
#205537=CARTESIAN_POINT('Ctrl Pts',(188.698356114064,4.87541577373173,130.156669259165));
#205538=CARTESIAN_POINT('Ctrl Pts',(188.690609780798,4.85734566903134,130.020648803825));
#205539=CARTESIAN_POINT('Ctrl Pts',(188.682863447533,4.8335790631205,129.885385940352));
#205540=CARTESIAN_POINT('Ctrl Pts',(188.675117114268,4.8042098296649,129.751388170134));
#205541=CARTESIAN_POINT('Ctrl Pts',(188.667369046265,4.77483401917306,129.617360392044));
#205542=CARTESIAN_POINT('Ctrl Pts',(188.659620978262,4.73985316817686,129.484598652787));
#205543=CARTESIAN_POINT('Ctrl Pts',(188.651872910259,4.69941180461004,129.353598144522));
#205544=CARTESIAN_POINT('Ctrl Pts',(188.644116607517,4.65892745948071,129.222458407358));
#205545=CARTESIAN_POINT('Ctrl Pts',(188.636360304775,4.61297112417784,129.093084014587));
#205546=CARTESIAN_POINT('Ctrl Pts',(188.628604002033,4.56173674692024,128.965953449853));
#205547=CARTESIAN_POINT('Ctrl Pts',(188.620843559519,4.51047502433273,128.838755031709));
#205548=CARTESIAN_POINT('Ctrl Pts',(188.613083117005,4.4539298076903,128.713803183936));
#205549=CARTESIAN_POINT('Ctrl Pts',(188.605322674491,4.39234193722288,128.591553493343));
#205550=CARTESIAN_POINT('Ctrl Pts',(188.597549774225,4.33065520043842,128.469107556694));
#205551=CARTESIAN_POINT('Ctrl Pts',(188.58977687396,4.26390982407976,128.349372787105));
#205552=CARTESIAN_POINT('Ctrl Pts',(188.582003973694,4.1923915294448,128.23277816189));
#205553=CARTESIAN_POINT('Ctrl Pts',(188.574513637932,4.12347310496294,128.120422044985));
#205554=CARTESIAN_POINT('Ctrl Pts',(188.56702330217,4.05012292420374,128.010981987703));
#205555=CARTESIAN_POINT('Ctrl Pts',(188.559532966408,3.9726318877381,127.904812558467));
#205556=CARTESIAN_POINT('Ctrl Pts',(188.551758632289,3.89220275507264,127.794617683053));
#205557=CARTESIAN_POINT('Ctrl Pts',(188.54398429817,3.80705779181573,127.687597278996));
#205558=CARTESIAN_POINT('Ctrl Pts',(188.536209964051,3.71747623705813,127.584181509285));
#205559=CARTESIAN_POINT('Ctrl Pts',(188.528445211104,3.62800508356063,127.480893190268));
#205560=CARTESIAN_POINT('Ctrl Pts',(188.520680458157,3.53410847118426,127.38120095924));
#205561=CARTESIAN_POINT('Ctrl Pts',(188.512915705209,3.4361083642224,127.285505353162));
#205562=CARTESIAN_POINT('Ctrl Pts',(188.505158664324,3.33820559234877,127.18990479331));
#205563=CARTESIAN_POINT('Ctrl Pts',(188.49740162344,3.23620771452785,127.098293230294));
#205564=CARTESIAN_POINT('Ctrl Pts',(188.489644582555,3.13047609649216,127.011037210342));
#205565=CARTESIAN_POINT('Ctrl Pts',(188.481893391314,3.02482421149156,126.923846990833));
#205566=CARTESIAN_POINT('Ctrl Pts',(188.474142200074,2.91544449096346,126.841006024537));
#205567=CARTESIAN_POINT('Ctrl Pts',(188.466391008834,2.80273392824307,126.762842884093));
#205568=CARTESIAN_POINT('Ctrl Pts',(188.458643112057,2.69007127051854,126.684712965069));
#205569=CARTESIAN_POINT('Ctrl Pts',(188.45089521528,2.57408090691345,126.611257139848));
#205570=CARTESIAN_POINT('Ctrl Pts',(188.443147318503,2.45519139564007,126.542762528436));
#205571=CARTESIAN_POINT('Ctrl Pts',(188.435401042419,2.33632675348964,126.47428224462));
#205572=CARTESIAN_POINT('Ctrl Pts',(188.427654766335,2.21456450846326,126.410761305459));
#205573=CARTESIAN_POINT('Ctrl Pts',(188.419908490251,2.09036023095675,126.352442248218));
#205574=CARTESIAN_POINT('Ctrl Pts',(188.412162156985,1.96615503660239,126.294122760479));
#205575=CARTESIAN_POINT('Ctrl Pts',(188.40441582372,1.83950812769249,126.241005397451));
#205576=CARTESIAN_POINT('Ctrl Pts',(188.396669490455,1.71089722052739,126.193285497457));
#205577=CARTESIAN_POINT('Ctrl Pts',(188.388921422452,1.58225751184136,126.145554910922));
#205578=CARTESIAN_POINT('Ctrl Pts',(188.381173354449,1.45165329617858,126.10322432862));
#205579=CARTESIAN_POINT('Ctrl Pts',(188.373425286446,1.31957931360486,126.066439818565));
#205580=CARTESIAN_POINT('Ctrl Pts',(188.365668983704,1.18736496123061,126.029616213495));
#205581=CARTESIAN_POINT('Ctrl Pts',(188.357912680962,1.05367809874174,125.998350560498));
#205582=CARTESIAN_POINT('Ctrl Pts',(188.35015637822,0.919026121729599,125.972738317543));
#205583=CARTESIAN_POINT('Ctrl Pts',(188.342395935706,0.78430227690315,125.947112404563));
#205584=CARTESIAN_POINT('Ctrl Pts',(188.334635493192,0.648612677762575,
125.927145970928));
#205585=CARTESIAN_POINT('Ctrl Pts',(188.326875050678,0.512470802420838,
125.912882646731));
#205586=CARTESIAN_POINT('Ctrl Pts',(188.319102150412,0.376110380054625,
125.89859642578));
#205587=CARTESIAN_POINT('Ctrl Pts',(188.311329250147,0.239296621066078,
125.89003163359));
#205588=CARTESIAN_POINT('Ctrl Pts',(188.303556349881,0.102544875559919,
125.88717975746));
#205589=CARTESIAN_POINT('Ctrl Pts',(188.296066014119,-0.0292355995406955,
125.88443155421));
#205590=CARTESIAN_POINT('Ctrl Pts',(188.288575678357,-0.160958183613458,
125.886988114484));
#205591=CARTESIAN_POINT('Ctrl Pts',(188.281085342595,-0.292167329337183,
125.894796348288));
#205592=CARTESIAN_POINT('Ctrl Pts',(188.273311008476,-0.428351309700771,
125.90290063365));
#205593=CARTESIAN_POINT('Ctrl Pts',(188.265536674357,-0.564413539030559,
125.916688360158));
#205594=CARTESIAN_POINT('Ctrl Pts',(188.257762340238,-0.699841173472941,
125.936157109658));
#205595=CARTESIAN_POINT('Ctrl Pts',(188.249997587291,-0.835101905459319,
125.955601865663));
#205596=CARTESIAN_POINT('Ctrl Pts',(188.242232834344,-0.9697292153955,125.980713658957));
#205597=CARTESIAN_POINT('Ctrl Pts',(188.234468081397,-1.10321209062758,
126.011438111871));
#205598=CARTESIAN_POINT('Ctrl Pts',(188.226711040512,-1.23656238878648,
126.042132048826));
#205599=CARTESIAN_POINT('Ctrl Pts',(188.218953999627,-1.36877013572612,
126.07842746462));
#205600=CARTESIAN_POINT('Ctrl Pts',(188.211196958742,-1.49933161871793,
126.120218459218));
#205601=CARTESIAN_POINT('Ctrl Pts',(188.203445767502,-1.62979464427913,
126.161977938902));
#205602=CARTESIAN_POINT('Ctrl Pts',(188.195694576262,-1.75861350609556,
126.20922462979));
#205603=CARTESIAN_POINT('Ctrl Pts',(188.187943385022,-1.88529718210462,
126.261802131685));
#205604=CARTESIAN_POINT('Ctrl Pts',(188.180195488244,-2.01192701417225,
126.314357286739));
#205605=CARTESIAN_POINT('Ctrl Pts',(188.172447591467,-2.13642310505805,
126.372238596868));
#205606=CARTESIAN_POINT('Ctrl Pts',(188.16469969469,-2.25831224638831,126.435240699286));
#205607=CARTESIAN_POINT('Ctrl Pts',(188.156953418606,-2.38017589113758,
126.498229623022));
#205608=CARTESIAN_POINT('Ctrl Pts',(188.149207142522,-2.49943332390471,
126.566337029047));
#205609=CARTESIAN_POINT('Ctrl Pts',(188.141460866438,-2.61563424429333,
126.6393107304));
#205610=CARTESIAN_POINT('Ctrl Pts',(188.133714533173,-2.73183602245093,
126.712284970429));
#205611=CARTESIAN_POINT('Ctrl Pts',(188.125968199908,-2.84498091211698,
126.790125369541));
#205612=CARTESIAN_POINT('Ctrl Pts',(188.118221866642,-2.95464635229878,
126.872535596619));
#205613=CARTESIAN_POINT('Ctrl Pts',(188.110473798639,-3.06433635129529,
126.954964278895));
#205614=CARTESIAN_POINT('Ctrl Pts',(188.102725730636,-3.17054503780084,
127.04196459072));
#205615=CARTESIAN_POINT('Ctrl Pts',(188.094977662633,-3.27288210156859,
127.133199246592));
#205616=CARTESIAN_POINT('Ctrl Pts',(188.087221359892,-3.37532793038579,
127.224530867742));
#205617=CARTESIAN_POINT('Ctrl Pts',(188.07946505715,-3.47389362439947,127.320105562212));
#205618=CARTESIAN_POINT('Ctrl Pts',(188.071708754408,-3.56822461240654,
127.419548041083));
#205619=CARTESIAN_POINT('Ctrl Pts',(188.063948311894,-3.66260594770211,
127.519043595399));
#205620=CARTESIAN_POINT('Ctrl Pts',(188.05618786938,-3.75274781653608,127.622410752998));
#205621=CARTESIAN_POINT('Ctrl Pts',(188.048427426866,-3.83833596421348,
127.729241093332));
#205622=CARTESIAN_POINT('Ctrl Pts',(188.0406545266,-3.92406150558378,127.836242927212));
#205623=CARTESIAN_POINT('Ctrl Pts',(188.032881626335,-4.00521848641537,
127.946718738031));
#205624=CARTESIAN_POINT('Ctrl Pts',(188.025108726069,-4.08153550936666,
128.060230345826));
#205625=CARTESIAN_POINT('Ctrl Pts',(188.017618390307,-4.15507821630353,
128.169615520761));
#205626=CARTESIAN_POINT('Ctrl Pts',(188.010128054545,-4.22412658393381,
128.281819344595));
#205627=CARTESIAN_POINT('Ctrl Pts',(188.002637718783,-4.28847904391944,
128.396429856027));
#205628=CARTESIAN_POINT('Ctrl Pts',(187.994504561361,-4.35835424099316,
128.52087625753));
#205629=CARTESIAN_POINT('Ctrl Pts',(187.98637140394,-4.42289737344505,128.648524117943));
#205630=CARTESIAN_POINT('Ctrl Pts',(187.978238246518,-4.48181742515692,
128.778898786264));
#205631=CARTESIAN_POINT('Ctrl Pts',(187.970122616113,-4.54061050370865,
128.908992496183));
#205632=CARTESIAN_POINT('Ctrl Pts',(187.962006985708,-4.59380452073732,
129.041800991969));
#205633=CARTESIAN_POINT('Ctrl Pts',(187.953891355302,-4.6411539136234,129.176824623322));
#205634=CARTESIAN_POINT('Ctrl Pts',(187.94588335265,-4.68787536899956,129.310057600188));
#205635=CARTESIAN_POINT('Ctrl Pts',(187.937875349997,-4.72890612235297,
129.445447018229));
#205636=CARTESIAN_POINT('Ctrl Pts',(187.929867347344,-4.76405452823405,
129.582490119308));
#205637=CARTESIAN_POINT('Ctrl Pts',(189.680106903305,-4.76405452823404,
129.582490119308));
#205638=CARTESIAN_POINT('Ctrl Pts',(189.67784575609,-4.77392102796961,129.620959452032));
#205639=CARTESIAN_POINT('Ctrl Pts',(189.675584608875,-4.78331723303707,
129.659531493429));
#205640=CARTESIAN_POINT('Ctrl Pts',(189.67332346166,-4.79224143417708,129.69819376801));
#205641=CARTESIAN_POINT('Ctrl Pts',(189.662792978718,-4.83380270327263,
129.87824945843));
#205642=CARTESIAN_POINT('Ctrl Pts',(189.652262495776,-4.86523011335524,
130.060725185327));
#205643=CARTESIAN_POINT('Ctrl Pts',(189.641732012834,-4.88629864809003,
130.244656602775));
#205644=CARTESIAN_POINT('Ctrl Pts',(189.631201529892,-4.90736718282481,
130.428588020222));
#205645=CARTESIAN_POINT('Ctrl Pts',(189.62067104695,-4.91807669726267,130.613975751142));
#205646=CARTESIAN_POINT('Ctrl Pts',(189.610140564008,-4.91824791299315,
130.799829741432));
#205647=CARTESIAN_POINT('Origin',(213.235140564004,0.,130.804360617566));
#205648=CARTESIAN_POINT('',(191.430300680169,-4.76051597898721,129.583432241588));
#205649=CARTESIAN_POINT('',(191.084784152919,-4.76405452823405,129.582490119308));
#205650=CARTESIAN_POINT('',(213.235140564004,-4.76405452823405,129.582490119308));
#205651=CARTESIAN_POINT('',(191.014859436046,-4.91824790535574,130.799821458629));
#205652=CARTESIAN_POINT('Ctrl Pts',(191.084784152919,-4.76405452823405,
129.582490119308));
#205653=CARTESIAN_POINT('Ctrl Pts',(191.074632403862,-4.8083124628535,129.755051134682));
#205654=CARTESIAN_POINT('Ctrl Pts',(191.064480654806,-4.84321315731302,
129.930105519379));
#205655=CARTESIAN_POINT('Ctrl Pts',(191.054328905749,-4.86852710622365,
130.106774150907));
#205656=CARTESIAN_POINT('Ctrl Pts',(191.04439137085,-4.89330690026231,130.279714861098));
#205657=CARTESIAN_POINT('Ctrl Pts',(191.03445383595,-4.90890030782398,130.45420266127));
#205658=CARTESIAN_POINT('Ctrl Pts',(191.02451630105,-4.91513668305779,130.629390764849));
#205659=CARTESIAN_POINT('Ctrl Pts',(191.021297346049,-4.91715676263013,
130.686137496098));
#205660=CARTESIAN_POINT('Ctrl Pts',(191.018078391047,-4.91819542437289,
130.74295751366));
#205661=CARTESIAN_POINT('Ctrl Pts',(191.014859436046,-4.91824790535574,
130.799821458629));
#205662=CARTESIAN_POINT('Ctrl Pts',(191.014859435991,-4.91824790535664,
130.799821459599));
#205663=CARTESIAN_POINT('Ctrl Pts',(191.007192991401,-4.9183728969955,130.93525183469));
#205664=CARTESIAN_POINT('Ctrl Pts',(190.999526546812,-4.91289980315623,
131.070824814365));
#205665=CARTESIAN_POINT('Ctrl Pts',(190.991860102222,-4.90182013838234,
131.206035104495));
#205666=CARTESIAN_POINT('Ctrl Pts',(190.984145221007,-4.8906704722459,131.342099653731));
#205667=CARTESIAN_POINT('Ctrl Pts',(190.976430339793,-4.87384310420628,
131.477796505531));
#205668=CARTESIAN_POINT('Ctrl Pts',(190.968715458578,-4.85138271638349,
131.612611074835));
#205669=CARTESIAN_POINT('Ctrl Pts',(190.961055815356,-4.82908314331645,
131.746460381553));
#205670=CARTESIAN_POINT('Ctrl Pts',(190.953396172134,-4.80123103213926,
131.879439600074));
#205671=CARTESIAN_POINT('Ctrl Pts',(190.945736528912,-4.76792200125562,
132.011051486199));
#205672=CARTESIAN_POINT('Ctrl Pts',(190.938077448338,-4.7346154171254,132.142653704621));
#205673=CARTESIAN_POINT('Ctrl Pts',(190.930418367764,-4.69585280864405,
132.27288840198));
#205674=CARTESIAN_POINT('Ctrl Pts',(190.92275928719,-4.65178043486449,132.401270711564));
#205675=CARTESIAN_POINT('Ctrl Pts',(190.91509902035,-4.60770123499393,132.529672905471));
#205676=CARTESIAN_POINT('Ctrl Pts',(190.907438753509,-4.55831076464351,
132.65622176218));
#205677=CARTESIAN_POINT('Ctrl Pts',(190.899778486669,-4.50380428023245,
132.780450207605));
#205678=CARTESIAN_POINT('Ctrl Pts',(190.892022192202,-4.44861451305745,
132.906235956834));
#205679=CARTESIAN_POINT('Ctrl Pts',(190.884265897736,-4.38817975595761,
133.029642333155));
#205680=CARTESIAN_POINT('Ctrl Pts',(190.876509603269,-4.32275123572271,
133.150209039045));
#205681=CARTESIAN_POINT('Ctrl Pts',(190.868837761032,-4.25803511551729,
133.269462988289));
#205682=CARTESIAN_POINT('Ctrl Pts',(190.861165918795,-4.18843370140229,
133.385938486624));
#205683=CARTESIAN_POINT('Ctrl Pts',(190.853494076558,-4.11423393107197,
133.499219096766));
#205684=CARTESIAN_POINT('Ctrl Pts',(190.845695555977,-4.03880896557229,
133.614370209414));
#205685=CARTESIAN_POINT('Ctrl Pts',(190.837897035395,-3.95863270394605,
133.726219643716));
#205686=CARTESIAN_POINT('Ctrl Pts',(190.830098514814,-3.87404868695243,
133.834365540602));
#205687=CARTESIAN_POINT('Ctrl Pts',(190.822299994233,-3.78946466995879,
133.942511437488));
#205688=CARTESIAN_POINT('Ctrl Pts',(190.814501473652,-3.70047322628425,
134.046953515992));
#205689=CARTESIAN_POINT('Ctrl Pts',(190.80670295307,-3.60745575518182,134.147330260998));
#205690=CARTESIAN_POINT('Ctrl Pts',(190.798928618951,-3.51472677001999,
134.247395695888));
#205691=CARTESIAN_POINT('Ctrl Pts',(190.791154284832,-3.41768425491403,
134.343758457961));
#205692=CARTESIAN_POINT('Ctrl Pts',(190.783379950713,-3.31665570023412,
134.436023876818));
#205693=CARTESIAN_POINT('Ctrl Pts',(190.775615197766,-3.21575165421878,
134.528175586793));
#205694=CARTESIAN_POINT('Ctrl Pts',(190.767850444819,-3.11087162883549,
134.616239739652));
#205695=CARTESIAN_POINT('Ctrl Pts',(190.760085691872,-3.00238209392103,
134.699856070599));
#205696=CARTESIAN_POINT('Ctrl Pts',(190.752328650987,-2.89400031234197,
134.783389352628));
#205697=CARTESIAN_POINT('Ctrl Pts',(190.744571610102,-2.78201646323467,
134.862483366925));
#205698=CARTESIAN_POINT('Ctrl Pts',(190.736814569217,-2.66683218589617,
134.936816201691));
#205699=CARTESIAN_POINT('Ctrl Pts',(190.729063377977,-2.55173476991692,
135.011092981489));
#205700=CARTESIAN_POINT('Ctrl Pts',(190.721312186737,-2.43344205673886,
135.080615517179));
#205701=CARTESIAN_POINT('Ctrl Pts',(190.713560995496,-2.3123866426324,135.145103765631));
#205702=CARTESIAN_POINT('Ctrl Pts',(190.705813098719,-2.19138268030653,
135.209564604857));
#205703=CARTESIAN_POINT('Ctrl Pts',(190.698065201942,-2.06761869682469,
135.268995229124));
#205704=CARTESIAN_POINT('Ctrl Pts',(190.690317305165,-1.94155380476799,
135.323160445584));
#205705=CARTESIAN_POINT('Ctrl Pts',(190.682571029081,-1.81551528276903,
135.377314331847));
#205706=CARTESIAN_POINT('Ctrl Pts',(190.674824752997,-1.68717716851246,
135.426204846825));
#205707=CARTESIAN_POINT('Ctrl Pts',(190.667078476913,-1.55702020428703,
135.469644225873));
#205708=CARTESIAN_POINT('Ctrl Pts',(190.659332143647,-1.42686227927271,
135.513083925581));
#205709=CARTESIAN_POINT('Ctrl Pts',(190.651585810382,-1.29488584835446,
135.551072285292));
#205710=CARTESIAN_POINT('Ctrl Pts',(190.643839477117,-1.16158814539901,
135.583470999527));
#205711=CARTESIAN_POINT('Ctrl Pts',(190.636091409114,-1.02826059134723,
135.615876969229));
#205712=CARTESIAN_POINT('Ctrl Pts',(190.628343341111,-0.893611556303883,
135.642690710273));
#205713=CARTESIAN_POINT('Ctrl Pts',(190.620595273108,-0.758149436995237,
135.663824836354));
#205714=CARTESIAN_POINT('Ctrl Pts',(190.612838970366,-0.622543346934008,
135.684981424036));
#205715=CARTESIAN_POINT('Ctrl Pts',(190.605082667624,-0.486122833271634,
135.700446278109));
#205716=CARTESIAN_POINT('Ctrl Pts',(190.597326364882,-0.349402960938852,
135.710183752717));
#205717=CARTESIAN_POINT('Ctrl Pts',(190.589565922368,-0.21261011709358,
135.719926424509));
#205718=CARTESIAN_POINT('Ctrl Pts',(190.581805479854,-0.0755179868161497,
135.723935614332));
#205719=CARTESIAN_POINT('Ctrl Pts',(190.57404503734,0.0613583669252786,
135.722227859909));
#205720=CARTESIAN_POINT('Ctrl Pts',(190.566272137074,0.198454446740975,
135.720517364047));
#205721=CARTESIAN_POINT('Ctrl Pts',(190.558499236809,0.335333667223026,
135.713071605924));
#205722=CARTESIAN_POINT('Ctrl Pts',(190.550726336543,0.471485185895587,
135.699959128676));
#205723=CARTESIAN_POINT('Ctrl Pts',(190.543236000781,0.602687253919808,
135.687323323004));
#205724=CARTESIAN_POINT('Ctrl Pts',(190.535745665019,0.7332133040056,135.669425686172));
#205725=CARTESIAN_POINT('Ctrl Pts',(190.528255329257,0.862617086158864,
135.646372061704));
#205726=CARTESIAN_POINT('Ctrl Pts',(190.520480995138,0.996927252043568,
135.622444352059));
#205727=CARTESIAN_POINT('Ctrl Pts',(190.512706661019,1.13045382272073,135.592886162405));
#205728=CARTESIAN_POINT('Ctrl Pts',(190.5049323269,1.26268773426236,135.557759690676));
#205729=CARTESIAN_POINT('Ctrl Pts',(190.497167573953,1.3947586793262,135.522676509184));
#205730=CARTESIAN_POINT('Ctrl Pts',(190.489402821006,1.5255397607892,135.482038799179));
#205731=CARTESIAN_POINT('Ctrl Pts',(190.481638068059,1.65452979177848,135.435960150192));
#205732=CARTESIAN_POINT('Ctrl Pts',(190.473881027174,1.78339170804989,135.389927267168));
#205733=CARTESIAN_POINT('Ctrl Pts',(190.466123986289,1.91046574813598,135.338464330073));
#205734=CARTESIAN_POINT('Ctrl Pts',(190.458366945404,2.03526398267376,135.281735248232));
#205735=CARTESIAN_POINT('Ctrl Pts',(190.450615754164,2.15996810589255,135.225048946233));
#205736=CARTESIAN_POINT('Ctrl Pts',(190.442864562924,2.28239948508168,135.163104565135));
#205737=CARTESIAN_POINT('Ctrl Pts',(190.435113371684,2.40208868317336,135.096114690282));
#205738=CARTESIAN_POINT('Ctrl Pts',(190.427365474906,2.52172701016312,135.029153287912));
#205739=CARTESIAN_POINT('Ctrl Pts',(190.419617578129,2.63862513369723,134.95715084752));
#205740=CARTESIAN_POINT('Ctrl Pts',(190.411869681352,2.75233701780585,134.880366506045));
#205741=CARTESIAN_POINT('Ctrl Pts',(190.404123405268,2.86602511583959,134.803598226199));
#205742=CARTESIAN_POINT('Ctrl Pts',(190.396377129184,2.97652797633052,134.722050253513));
#205743=CARTESIAN_POINT('Ctrl Pts',(190.3886308531,3.08342777461511,134.636025558715));
#205744=CARTESIAN_POINT('Ctrl Pts',(190.380884519835,3.1903283620097,134.550000228902));
#205745=CARTESIAN_POINT('Ctrl Pts',(190.373138186569,3.29362552953602,134.459498356145));
#205746=CARTESIAN_POINT('Ctrl Pts',(190.365391853304,3.39293414982598,134.364863519888));
#205747=CARTESIAN_POINT('Ctrl Pts',(190.357643785301,3.49226500959297,134.270207490816));
#205748=CARTESIAN_POINT('Ctrl Pts',(190.349895717298,3.58760526176411,134.171416926171));
#205749=CARTESIAN_POINT('Ctrl Pts',(190.342147649295,3.67860658491866,134.068872320086));
#205750=CARTESIAN_POINT('Ctrl Pts',(190.334391346553,3.76970462536241,133.966218728374));
#205751=CARTESIAN_POINT('Ctrl Pts',(190.326635043811,3.85645426497193,133.859803417977));
#205752=CARTESIAN_POINT('Ctrl Pts',(190.31887874107,3.93854710870415,133.750040460152));
#205753=CARTESIAN_POINT('Ctrl Pts',(190.311118298555,4.02068376785884,133.640218918532));
#205754=CARTESIAN_POINT('Ctrl Pts',(190.303357856041,4.09815845787932,133.527046491708));
#205755=CARTESIAN_POINT('Ctrl Pts',(190.295597413527,4.17070668830499,133.410965455785));
#205756=CARTESIAN_POINT('Ctrl Pts',(190.287824513262,4.24337137959067,133.294698076279));
#205757=CARTESIAN_POINT('Ctrl Pts',(190.280051612996,4.31109361453856,133.175513097328));
#205758=CARTESIAN_POINT('Ctrl Pts',(190.272278712731,4.37365493759366,133.053877354415));
#205759=CARTESIAN_POINT('Ctrl Pts',(190.264788376969,4.43394199897344,132.936663377138));
#205760=CARTESIAN_POINT('Ctrl Pts',(190.257298041207,4.4894367285661,132.817174004629));
#205761=CARTESIAN_POINT('Ctrl Pts',(190.249807705445,4.53998696650629,132.695841890657));
#205762=CARTESIAN_POINT('Ctrl Pts',(190.242033371326,4.59245383208216,132.569909432706));
#205763=CARTESIAN_POINT('Ctrl Pts',(190.234259037206,4.63976006301382,132.44159282362));
#205764=CARTESIAN_POINT('Ctrl Pts',(190.226484703087,4.68168282669612,132.3113539728));
#205765=CARTESIAN_POINT('Ctrl Pts',(190.21871995014,4.72355392431904,132.181275629723));
#205766=CARTESIAN_POINT('Ctrl Pts',(190.210955197193,4.76005463700814,132.049280127086));
#205767=CARTESIAN_POINT('Ctrl Pts',(190.203190444246,4.79100962710627,131.915850525516));
#205768=CARTESIAN_POINT('Ctrl Pts',(190.195433403361,4.82193387227178,131.782553448108));
#205769=CARTESIAN_POINT('Ctrl Pts',(190.187676362476,4.84732326841009,131.647825484707));
#205770=CARTESIAN_POINT('Ctrl Pts',(190.179919321591,4.8670519793402,131.5121657411));
#205771=CARTESIAN_POINT('Ctrl Pts',(190.172168130351,4.8867658126959,131.376608299561));
#205772=CARTESIAN_POINT('Ctrl Pts',(190.164416939111,4.90082740152704,131.240120861754));
#205773=CARTESIAN_POINT('Ctrl Pts',(190.156665747871,4.90916185770046,131.103213285948));
#205774=CARTESIAN_POINT('Ctrl Pts',(190.148917851094,4.91749277150769,130.966363899514));
#205775=CARTESIAN_POINT('Ctrl Pts',(190.141169954316,4.92010137035702,130.829095119669));
#205776=CARTESIAN_POINT('Ctrl Pts',(190.133422057539,4.91696458015609,130.691922278951));
#205777=CARTESIAN_POINT('Ctrl Pts',(190.125675781455,4.91382844610404,130.554778131835));
#205778=CARTESIAN_POINT('Ctrl Pts',(190.117929505371,4.90494932240312,130.417730274544));
#205779=CARTESIAN_POINT('Ctrl Pts',(190.110183229287,4.8903562624689,130.281293997879));
#205780=CARTESIAN_POINT('Ctrl Pts',(190.102436896022,4.87576309481204,130.144856714072));
#205781=CARTESIAN_POINT('Ctrl Pts',(190.094690562756,4.85545594833678,130.009031408648));
#205782=CARTESIAN_POINT('Ctrl Pts',(190.086944229491,4.82951571541046,129.87432781325));
#205783=CARTESIAN_POINT('Ctrl Pts',(190.079196161488,4.80356967334887,129.739594051917));
#205784=CARTESIAN_POINT('Ctrl Pts',(190.071448093485,4.77198810853258,129.605982884305));
#205785=CARTESIAN_POINT('Ctrl Pts',(190.063700025482,4.73490286521561,129.473993029464));
#205786=CARTESIAN_POINT('Ctrl Pts',(190.05594372274,4.69777820726065,129.341862894234));
#205787=CARTESIAN_POINT('Ctrl Pts',(190.048187419998,4.65513829197155,129.211357890945));
#205788=CARTESIAN_POINT('Ctrl Pts',(190.040431117256,4.60716479417153,129.082961296709));
#205789=CARTESIAN_POINT('Ctrl Pts',(190.032670674742,4.55916569147128,128.954496173345));
#205790=CARTESIAN_POINT('Ctrl Pts',(190.024910232228,4.50582748595494,128.828142061345));
#205791=CARTESIAN_POINT('Ctrl Pts',(190.017149789714,4.44737931348167,128.704360545062));
#205792=CARTESIAN_POINT('Ctrl Pts',(190.009376889448,4.38883731481318,128.580380323701));
#205793=CARTESIAN_POINT('Ctrl Pts',(190.001603989183,4.32516913872479,128.458981297068));
#205794=CARTESIAN_POINT('Ctrl Pts',(189.993831088917,4.25664946656522,128.34059959399));
#205795=CARTESIAN_POINT('Ctrl Pts',(189.986340753155,4.19062065707926,128.226521364005));
#205796=CARTESIAN_POINT('Ctrl Pts',(189.978850417393,4.12008712075145,128.115245151775));
#205797=CARTESIAN_POINT('Ctrl Pts',(189.971360081631,4.04533061532805,128.007132833636));
#205798=CARTESIAN_POINT('Ctrl Pts',(189.963585747512,3.96773969427981,127.894921404095));
#205799=CARTESIAN_POINT('Ctrl Pts',(189.955811413393,3.88535347027769,127.785763070711));
#205800=CARTESIAN_POINT('Ctrl Pts',(189.948037079274,3.79844011431754,127.680094982182));
#205801=CARTESIAN_POINT('Ctrl Pts',(189.940272326327,3.71163387130119,127.574557120128));
#205802=CARTESIAN_POINT('Ctrl Pts',(189.93250757338,3.62031184341438,127.472501243445));
#205803=CARTESIAN_POINT('Ctrl Pts',(189.924742820433,3.52478566895689,127.374335974737));
#205804=CARTESIAN_POINT('Ctrl Pts',(189.916985779548,3.42935437244241,127.276268205157));
#205805=CARTESIAN_POINT('Ctrl Pts',(189.909228738663,3.32972750992248,127.18208363199));
#205806=CARTESIAN_POINT('Ctrl Pts',(189.901471697778,3.22625697570096,127.092157903645));
#205807=CARTESIAN_POINT('Ctrl Pts',(189.893720506538,3.12286446941407,127.002299988992));
#205808=CARTESIAN_POINT('Ctrl Pts',(189.885969315298,3.01563435469827,126.916694782037));
#205809=CARTESIAN_POINT('Ctrl Pts',(189.878218124058,2.90495511089095,126.835680879138));
#205810=CARTESIAN_POINT('Ctrl Pts',(189.87047022728,2.79432290871461,126.754701409308));
#205811=CARTESIAN_POINT('Ctrl Pts',(189.862722330503,2.68024480797378,126.678309592735));
#205812=CARTESIAN_POINT('Ctrl Pts',(189.854974433726,2.56314190041725,126.606803392128));
#205813=CARTESIAN_POINT('Ctrl Pts',(189.847228157642,2.44606348826436,126.535312149077));
#205814=CARTESIAN_POINT('Ctrl Pts',(189.839481881558,2.32596186128318,126.468704692871));
#205815=CARTESIAN_POINT('Ctrl Pts',(189.831735605474,2.20328625229884,126.407235107311));
#205816=CARTESIAN_POINT('Ctrl Pts',(189.823989272209,2.0806097377515,126.345765067998));
#205817=CARTESIAN_POINT('Ctrl Pts',(189.816242938943,1.9553595528264,126.289433150157));
#205818=CARTESIAN_POINT('Ctrl Pts',(189.808496605678,1.82800827349247,126.238446819152));
#205819=CARTESIAN_POINT('Ctrl Pts',(189.800748537675,1.70062847472297,126.187449070113));
#205820=CARTESIAN_POINT('Ctrl Pts',(189.793000469672,1.57114700814089,126.141799435301));
#205821=CARTESIAN_POINT('Ctrl Pts',(189.785252401669,1.44005472524652,126.10165656024));
#205822=CARTESIAN_POINT('Ctrl Pts',(189.777496098927,1.30882311591319,126.061471020852));
#205823=CARTESIAN_POINT('Ctrl Pts',(189.769739796186,1.17597764480057,126.02680404717));
#205824=CARTESIAN_POINT('Ctrl Pts',(189.761983493444,1.04202310631098,125.997764014104));
#205825=CARTESIAN_POINT('Ctrl Pts',(189.75422305093,0.907997072250902,125.968708481497));
#205826=CARTESIAN_POINT('Ctrl Pts',(189.746462608415,0.772861176351149,
125.945285940508));
#205827=CARTESIAN_POINT('Ctrl Pts',(189.738702165901,0.637127616130016,
125.927553110265));
#205828=CARTESIAN_POINT('Ctrl Pts',(189.730929265636,0.501176164348156,
125.909791813709));
#205829=CARTESIAN_POINT('Ctrl Pts',(189.723156365371,0.36462552068547,125.897738514198));
#205830=CARTESIAN_POINT('Ctrl Pts',(189.715383465105,0.227991084653854,
125.891397852816));
#205831=CARTESIAN_POINT('Ctrl Pts',(189.707893129343,0.0963236545319259,
125.885287690447));
#205832=CARTESIAN_POINT('Ctrl Pts',(189.700402793581,-0.035421273587108,
125.88448204139));
#205833=CARTESIAN_POINT('Ctrl Pts',(189.692912457819,-0.166786945949541,
125.888939457873));
#205834=CARTESIAN_POINT('Ctrl Pts',(189.6851381237,-0.303133387705632,125.893565878656));
#205835=CARTESIAN_POINT('Ctrl Pts',(189.677363789581,-0.439503151574217,
125.903876996674));
#205836=CARTESIAN_POINT('Ctrl Pts',(189.669589455462,-0.575383499002755,
125.91988348162));
#205837=CARTESIAN_POINT('Ctrl Pts',(189.661824702515,-0.711096386047016,
125.935870240005));
#205838=CARTESIAN_POINT('Ctrl Pts',(189.654059949567,-0.846320672210825,
125.95753835424));
#205839=CARTESIAN_POINT('Ctrl Pts',(189.64629519662,-0.980544123610611,
125.984846504696));
#205840=CARTESIAN_POINT('Ctrl Pts',(189.638538155735,-1.11463426238657,
126.012127532312));
#205841=CARTESIAN_POINT('Ctrl Pts',(189.63078111485,-1.24772516395203,126.045037370947));
#205842=CARTESIAN_POINT('Ctrl Pts',(189.623024073965,-1.37931057719251,
126.083483009097));
#205843=CARTESIAN_POINT('Ctrl Pts',(189.615272882725,-1.51079676084857,
126.121899655092));
#205844=CARTESIAN_POINT('Ctrl Pts',(189.607521691485,-1.64077934216929,
126.165843682135));
#205845=CARTESIAN_POINT('Ctrl Pts',(189.599770500245,-1.76876346787959,
126.215171271157));
#205846=CARTESIAN_POINT('Ctrl Pts',(189.592022603468,-1.89669319692298,
126.264477894638));
#205847=CARTESIAN_POINT('Ctrl Pts',(189.584274706691,-2.02262579569819,
126.319163388819));
#205848=CARTESIAN_POINT('Ctrl Pts',(189.576526809914,-2.14608296936092,
126.379034533409));
#205849=CARTESIAN_POINT('Ctrl Pts',(189.56878053383,-2.26951431844442,126.438893154247));
#205850=CARTESIAN_POINT('Ctrl Pts',(189.561034257746,-2.39047092080065,
126.503935097423));
#205851=CARTESIAN_POINT('Ctrl Pts',(189.553287981662,-2.50849618721501,
126.573919749143));
#205852=CARTESIAN_POINT('Ctrl Pts',(189.545541648396,-2.62652232486488,
126.643904917472));
#205853=CARTESIAN_POINT('Ctrl Pts',(189.537795315131,-2.74161674710555,
126.718832667743));
#205854=CARTESIAN_POINT('Ctrl Pts',(189.530048981866,-2.85334946859526,
126.798417548504));
#205855=CARTESIAN_POINT('Ctrl Pts',(189.522300913863,-2.96510721185335,
126.878020251747));
#205856=CARTESIAN_POINT('Ctrl Pts',(189.51455284586,-3.0735014379343,126.962281934019));
#205857=CARTESIAN_POINT('Ctrl Pts',(189.506804777857,-3.17813335664093,
127.050875379829));
#205858=CARTESIAN_POINT('Ctrl Pts',(189.499048475115,-3.28287647939589,
127.139562983809));
#205859=CARTESIAN_POINT('Ctrl Pts',(189.491292172373,-3.38384900824164,
127.232591294972));
#205860=CARTESIAN_POINT('Ctrl Pts',(189.483535869631,-3.48068691059195,
127.329594194778));
#205861=CARTESIAN_POINT('Ctrl Pts',(189.475775427117,-3.5775764982465,127.426648867953));
#205862=CARTESIAN_POINT('Ctrl Pts',(189.468014984603,-3.67032679795341,
127.527682068888));
#205863=CARTESIAN_POINT('Ctrl Pts',(189.460254542089,-3.75861323503234,
127.632293529382));
#205864=CARTESIAN_POINT('Ctrl Pts',(189.452481641823,-3.84704139733793,
127.737072921479));
#205865=CARTESIAN_POINT('Ctrl Pts',(189.444708741558,-3.93099113791891,
127.845441742504));
#205866=CARTESIAN_POINT('Ctrl Pts',(189.436935841292,-4.01017996607299,
127.95696888087));
#205867=CARTESIAN_POINT('Ctrl Pts',(189.42944550553,-4.08649008085959,128.064441726837));
#205868=CARTESIAN_POINT('Ctrl Pts',(189.421955169768,-4.15837924792512,
128.174846993079));
#205869=CARTESIAN_POINT('Ctrl Pts',(189.414464834006,-4.22563545189443,
128.287777996194));
#205870=CARTESIAN_POINT('Ctrl Pts',(189.406414631678,-4.29791873357895,
128.409150048544));
#205871=CARTESIAN_POINT('Ctrl Pts',(189.398364429349,-4.36506593948658,
128.533801166826));
#205872=CARTESIAN_POINT('Ctrl Pts',(189.39031422702,-4.42677811181953,128.661274382433));
#205873=CARTESIAN_POINT('Ctrl Pts',(189.382275040237,-4.48840583991566,
128.788573169269));
#205874=CARTESIAN_POINT('Ctrl Pts',(189.374235853453,-4.54461318938345,
128.918686050171));
#205875=CARTESIAN_POINT('Ctrl Pts',(189.366196666669,-4.59514535868655,
129.051128689086));
#205876=CARTESIAN_POINT('Ctrl Pts',(189.358170521655,-4.64559555092435,
129.183356469644));
#205877=CARTESIAN_POINT('Ctrl Pts',(189.350144376642,-4.69038878678416,
129.317906148175));
#205878=CARTESIAN_POINT('Ctrl Pts',(189.342118231628,-4.72931719504994,
129.454271016427));
#205879=CARTESIAN_POINT('Ctrl Pts',(189.339612754859,-4.74146925838755,
129.496839274155));
#205880=CARTESIAN_POINT('Ctrl Pts',(189.33710727809,-4.7530501596044,129.539584253036));
#205881=CARTESIAN_POINT('Ctrl Pts',(189.334601801321,-4.76405452823404,
129.582490119308));
#205882=CARTESIAN_POINT('',(191.360141504983,-4.9217530988948,130.806072159341));
#205883=CARTESIAN_POINT('Ctrl Pts',(191.360140564008,-4.9182496968395,130.806087475454));
#205884=CARTESIAN_POINT('Ctrl Pts',(191.354763444185,-4.91821654842555,
130.90049719961));
#205885=CARTESIAN_POINT('Ctrl Pts',(191.349386324361,-4.91546519350092,
130.994855987655));
#205886=CARTESIAN_POINT('Ctrl Pts',(191.344009204538,-4.91000321302235,
131.089056087516));
#205887=CARTESIAN_POINT('Ctrl Pts',(191.336234870419,-4.90210618588047,
131.225252243524));
#205888=CARTESIAN_POINT('Ctrl Pts',(191.3284605363,-4.88852553889003,131.361335297868));
#205889=CARTESIAN_POINT('Ctrl Pts',(191.32068620218,-4.86926290974064,131.49679240361));
#205890=CARTESIAN_POINT('Ctrl Pts',(191.312921449233,-4.85002402006014,
131.632082570575));
#205891=CARTESIAN_POINT('Ctrl Pts',(191.305156696286,-4.82511713569348,
131.76674794049));
#205892=CARTESIAN_POINT('Ctrl Pts',(191.297391943339,-4.79459585657098,
131.900277418538));
#205893=CARTESIAN_POINT('Ctrl Pts',(191.289634902454,-4.76410489161315,
132.033674273226));
#205894=CARTESIAN_POINT('Ctrl Pts',(191.281877861569,-4.72801071553388,
132.165937102515));
#205895=CARTESIAN_POINT('Ctrl Pts',(191.274120820684,-4.68641846168075,
132.296562033099));
#205896=CARTESIAN_POINT('Ctrl Pts',(191.266369629444,-4.64485757286983,
132.427088458406));
#205897=CARTESIAN_POINT('Ctrl Pts',(191.258618438204,-4.59780697707092,
132.555979072473));
#205898=CARTESIAN_POINT('Ctrl Pts',(191.250867246964,-4.5454223270494,132.682742615792));
#205899=CARTESIAN_POINT('Ctrl Pts',(191.243119350187,-4.49305994190156,
132.809452281224));
#205900=CARTESIAN_POINT('Ctrl Pts',(191.235371453409,-4.4353681606558,132.934036313446));
#205901=CARTESIAN_POINT('Ctrl Pts',(191.227623556632,-4.37255162571712,
133.056021192106));
#205902=CARTESIAN_POINT('Ctrl Pts',(191.219877280548,-4.3097482306434,133.177980554159));
#205903=CARTESIAN_POINT('Ctrl Pts',(191.212131004464,-4.24182239299693,
133.297341496706));
#205904=CARTESIAN_POINT('Ctrl Pts',(191.20438472838,-4.16902561416592,133.413653336087));
#205905=CARTESIAN_POINT('Ctrl Pts',(191.196638395115,-4.09622829796563,
133.529966034056));
#205906=CARTESIAN_POINT('Ctrl Pts',(191.188892061849,-4.01856017625269,
133.643229252539));
#205907=CARTESIAN_POINT('Ctrl Pts',(191.181145728584,-3.93631693673612,
133.753019980067));
#205908=CARTESIAN_POINT('Ctrl Pts',(191.173397660581,-3.85405527941647,
133.862835294467));
#205909=CARTESIAN_POINT('Ctrl Pts',(191.165649592578,-3.76721669987783,
133.969176257649));
#205910=CARTESIAN_POINT('Ctrl Pts',(191.157901524575,-3.67613788924386,
134.071652046528));
#205911=CARTESIAN_POINT('Ctrl Pts',(191.150145221833,-3.58496227896587,
134.174236747894));
#205912=CARTESIAN_POINT('Ctrl Pts',(191.142388919091,-3.48953769537748,
134.272947776186));
#205913=CARTESIAN_POINT('Ctrl Pts',(191.134632616349,-3.3902388873648,134.367429989484));
#205914=CARTESIAN_POINT('Ctrl Pts',(191.126872173835,-3.29088708058837,
134.461962630784));
#205915=CARTESIAN_POINT('Ctrl Pts',(191.119111731321,-3.18765722326609,
134.552261702453));
#205916=CARTESIAN_POINT('Ctrl Pts',(191.111351288807,-3.08095725723101,
134.638012328613));
#205917=CARTESIAN_POINT('Ctrl Pts',(191.103578388541,-2.97408600693812,
134.723900609291));
#205918=CARTESIAN_POINT('Ctrl Pts',(191.095805488276,-2.86373383115774,
134.805225621522));
#205919=CARTESIAN_POINT('Ctrl Pts',(191.088032588011,-2.7503384963244,134.881715301443));
#205920=CARTESIAN_POINT('Ctrl Pts',(191.080542252248,-2.64106536753748,
134.955424388834));
#205921=CARTESIAN_POINT('Ctrl Pts',(191.073051916486,-2.52896675349539,
135.024643431626));
#205922=CARTESIAN_POINT('Ctrl Pts',(191.065561580724,-2.41445430827056,
135.08917023478));
#205923=CARTESIAN_POINT('Ctrl Pts',(191.057787246605,-2.29560008888017,
135.156143591289));
#205924=CARTESIAN_POINT('Ctrl Pts',(191.050012912486,-2.17376888976368,
135.218274023238));
#205925=CARTESIAN_POINT('Ctrl Pts',(191.042238578367,-2.04939306878735,
135.275285702166));
#205926=CARTESIAN_POINT('Ctrl Pts',(191.03447382542,-1.92517052989461,135.332227119295));
#205927=CARTESIAN_POINT('Ctrl Pts',(191.026709072473,-1.79840996087941,
135.384062173901));
#205928=CARTESIAN_POINT('Ctrl Pts',(191.018944319526,-1.66957033235678,
135.430559701891));
#205929=CARTESIAN_POINT('Ctrl Pts',(191.011187278641,-1.54085866916962,
135.477011047882));
#205930=CARTESIAN_POINT('Ctrl Pts',(191.003430237756,-1.41007242119069,
135.518135285236));
#205931=CARTESIAN_POINT('Ctrl Pts',(190.995673196871,-1.27769233844608,
135.553748509787));
#205932=CARTESIAN_POINT('Ctrl Pts',(190.987922005631,-1.14541208455148,
135.589334878129));
#205933=CARTESIAN_POINT('Ctrl Pts',(190.980170814391,-1.01154076426068,
135.619418404572));
#205934=CARTESIAN_POINT('Ctrl Pts',(190.972419623151,-0.876575822233106,
135.643864506435));
#205935=CARTESIAN_POINT('Ctrl Pts',(190.964671726373,-0.741668243906204,
135.668300218052));
#205936=CARTESIAN_POINT('Ctrl Pts',(190.956923829596,-0.605668352230964,
135.687103201124));
#205937=CARTESIAN_POINT('Ctrl Pts',(190.949175932819,-0.469085147509697,
135.700189677785));
#205938=CARTESIAN_POINT('Ctrl Pts',(190.941429656735,-0.332530513050464,
135.713273417038));
#205939=CARTESIAN_POINT('Ctrl Pts',(190.933683380651,-0.195393197179081,
135.720642991066));
#205940=CARTESIAN_POINT('Ctrl Pts',(190.925937104567,-0.0581883154667574,
135.722266389584));
#205941=CARTESIAN_POINT('Ctrl Pts',(190.918190771302,0.0790175790607411,
135.723889800085));
#205942=CARTESIAN_POINT('Ctrl Pts',(190.910444438036,0.216290649486569,
135.71976694581));
#205943=CARTESIAN_POINT('Ctrl Pts',(190.902698104771,0.353115177852348,
135.709917949172));
#205944=CARTESIAN_POINT('Ctrl Pts',(190.894950036768,0.489970347122603,
135.700066746919));
#205945=CARTESIAN_POINT('Ctrl Pts',(190.887201968765,0.626376384571554,
135.684486878679));
#205946=CARTESIAN_POINT('Ctrl Pts',(190.879453900762,0.7618224898918,135.663250362806));
#205947=CARTESIAN_POINT('Ctrl Pts',(190.87169759802,0.897412548944634,135.641991276511));
#205948=CARTESIAN_POINT('Ctrl Pts',(190.863941295278,1.03204025099248,135.615063593716));
#205949=CARTESIAN_POINT('Ctrl Pts',(190.856184992537,1.16520424415458,135.58259063839));
#205950=CARTESIAN_POINT('Ctrl Pts',(190.848424550022,1.29843931094942,135.550100351271));
#205951=CARTESIAN_POINT('Ctrl Pts',(190.840664107508,1.43020873675926,135.512059002598));
#205952=CARTESIAN_POINT('Ctrl Pts',(190.832903664994,1.56002710506518,135.468639607288));
#205953=CARTESIAN_POINT('Ctrl Pts',(190.825130764729,1.69005386934062,135.42515051131));
#205954=CARTESIAN_POINT('Ctrl Pts',(190.817357864463,1.81812295188554,135.376266256074));
#205955=CARTESIAN_POINT('Ctrl Pts',(190.809584964198,1.94376883421616,135.322208089718));
#205956=CARTESIAN_POINT('Ctrl Pts',(190.802094628436,2.06484717224159,135.270115073873));
#205957=CARTESIAN_POINT('Ctrl Pts',(190.794604292674,2.1836751523785,135.21321791848));
#205958=CARTESIAN_POINT('Ctrl Pts',(190.787113956912,2.29986015313222,135.151753668411));
#205959=CARTESIAN_POINT('Ctrl Pts',(190.779339622793,2.42045034350282,135.087958982619));
#205960=CARTESIAN_POINT('Ctrl Pts',(190.771565288673,2.5385751745423,135.019041960452));
#205961=CARTESIAN_POINT('Ctrl Pts',(190.763790954554,2.65376888396502,134.945217264807));
#205962=CARTESIAN_POINT('Ctrl Pts',(190.756026201607,2.768820627436,134.871483551501));
#205963=CARTESIAN_POINT('Ctrl Pts',(190.74826144866,2.88094811077286,134.792854407899));
#205964=CARTESIAN_POINT('Ctrl Pts',(190.740496695713,2.98970876424912,134.709591029139));
#205965=CARTESIAN_POINT('Ctrl Pts',(190.732739654828,3.09836139511106,134.62641034874));
#205966=CARTESIAN_POINT('Ctrl Pts',(190.724982613943,3.20365354236057,134.538604829062));
#205967=CARTESIAN_POINT('Ctrl Pts',(190.717225573058,3.3051706250811,134.446479534021));
#205968=CARTESIAN_POINT('Ctrl Pts',(190.709474381818,3.40661115297993,134.354423711382));
#205969=CARTESIAN_POINT('Ctrl Pts',(190.701723190578,3.50428199439297,134.258054859062));
#205970=CARTESIAN_POINT('Ctrl Pts',(190.693971999338,3.59780104010722,134.157718746115));
#205971=CARTESIAN_POINT('Ctrl Pts',(190.68622410256,3.69128033773231,134.057425278691));
#205972=CARTESIAN_POINT('Ctrl Pts',(190.678476205783,3.78061108335151,133.953168189747));
#205973=CARTESIAN_POINT('Ctrl Pts',(190.670728309006,3.86544766517695,133.845330431668));
#205974=CARTESIAN_POINT('Ctrl Pts',(190.662982032922,3.95026650101836,133.737515230923));
#205975=CARTESIAN_POINT('Ctrl Pts',(190.655235756838,4.03059280135912,133.626121157924));
#205976=CARTESIAN_POINT('Ctrl Pts',(190.647489480754,4.10612120249017,133.511564291648));
#205977=CARTESIAN_POINT('Ctrl Pts',(190.639743147489,4.18165016115467,133.397006579739));
#205978=CARTESIAN_POINT('Ctrl Pts',(190.631996814223,4.25238093473435,133.279286354372));
#205979=CARTESIAN_POINT('Ctrl Pts',(190.624250480958,4.31805169463097,133.158848380328));
#205980=CARTESIAN_POINT('Ctrl Pts',(190.616502412955,4.38373716103891,133.038383435034));
#205981=CARTESIAN_POINT('Ctrl Pts',(190.608754344952,4.44436017178771,132.915199873166));
#205982=CARTESIAN_POINT('Ctrl Pts',(190.601006276949,4.49970521791473,132.789766373166));
#205983=CARTESIAN_POINT('Ctrl Pts',(190.593249974207,4.55510908541542,132.664199560951));
#205984=CARTESIAN_POINT('Ctrl Pts',(190.585493671465,4.60522362466958,132.536378392067));
#205985=CARTESIAN_POINT('Ctrl Pts',(190.577737368723,4.64988159868781,132.40679132767));
#205986=CARTESIAN_POINT('Ctrl Pts',(190.569976926209,4.69456340801143,132.277135098755));
#205987=CARTESIAN_POINT('Ctrl Pts',(190.562216483695,4.73378273728387,132.145711470748));
#205988=CARTESIAN_POINT('Ctrl Pts',(190.554456041181,4.76742276936732,132.013022357102));
#205989=CARTESIAN_POINT('Ctrl Pts',(190.546683140915,4.80111680341668,131.880120239111));
#205990=CARTESIAN_POINT('Ctrl Pts',(190.53891024065,4.82921356238978,131.745948958842));
#205991=CARTESIAN_POINT('Ctrl Pts',(190.531137340384,4.85164756449836,131.611019760201));
#205992=CARTESIAN_POINT('Ctrl Pts',(190.523647004622,4.8732660341224,131.480995577798));
#205993=CARTESIAN_POINT('Ctrl Pts',(190.51615666886,4.88962627167772,131.350267930446));
#205994=CARTESIAN_POINT('Ctrl Pts',(190.508666333098,4.90071548822044,131.219295270272));
#205995=CARTESIAN_POINT('Ctrl Pts',(190.500891998979,4.91222515577889,131.083356741879));
#205996=CARTESIAN_POINT('Ctrl Pts',(190.49311766486,4.91809266973481,130.946723642184));
#205997=CARTESIAN_POINT('Ctrl Pts',(190.485343330741,4.91824687616993,130.809903860727));
#205998=CARTESIAN_POINT('Ctrl Pts',(190.477578577794,4.91840089255939,130.673252697422));
#205999=CARTESIAN_POINT('Ctrl Pts',(190.469813824847,4.91285561076338,130.536415697335));
#206000=CARTESIAN_POINT('Ctrl Pts',(190.4620490719,4.90159156190185,130.399906389262));
#206001=CARTESIAN_POINT('Ctrl Pts',(190.454292031015,4.89033870065244,130.26353266416));
#206002=CARTESIAN_POINT('Ctrl Pts',(190.44653499013,4.8733784076575,130.127486370495));
#206003=CARTESIAN_POINT('Ctrl Pts',(190.438777949245,4.85074325071888,129.992281201434));
#206004=CARTESIAN_POINT('Ctrl Pts',(190.431026758005,4.82812516312819,129.857177991643));
#206005=CARTESIAN_POINT('Ctrl Pts',(190.423275566765,4.79984079389075,129.722915027962));
#206006=CARTESIAN_POINT('Ctrl Pts',(190.415524375525,4.76597450893968,129.590000686311));
#206007=CARTESIAN_POINT('Ctrl Pts',(190.407776478747,4.73212261806311,129.457142836802));
#206008=CARTESIAN_POINT('Ctrl Pts',(190.40002858197,4.6926936264518,129.325632847339));
#206009=CARTESIAN_POINT('Ctrl Pts',(190.392280685193,4.64782291118133,129.195968486027));
#206010=CARTESIAN_POINT('Ctrl Pts',(190.384534409109,4.60296158189719,129.066331247704));
#206011=CARTESIAN_POINT('Ctrl Pts',(190.376788133025,4.55266092085215,128.938539238861));
#206012=CARTESIAN_POINT('Ctrl Pts',(190.369041856941,4.49710593053007,128.813074271484));
#206013=CARTESIAN_POINT('Ctrl Pts',(190.361295523676,4.44155053011368,128.687608377954));
#206014=CARTESIAN_POINT('Ctrl Pts',(190.35354919041,4.38074088131789,128.564469917655));
#206015=CARTESIAN_POINT('Ctrl Pts',(190.345802857145,4.31490965259537,128.444119580629));
#206016=CARTESIAN_POINT('Ctrl Pts',(190.338054789142,4.24906368142562,128.32374229198));
#206017=CARTESIAN_POINT('Ctrl Pts',(190.330306721139,4.17819408019494,128.206154711989));
#206018=CARTESIAN_POINT('Ctrl Pts',(190.322558653136,4.10257867349393,128.091791486596));
#206019=CARTESIAN_POINT('Ctrl Pts',(190.314802350394,4.02688290183881,127.977306714606));
#206020=CARTESIAN_POINT('Ctrl Pts',(190.307046047653,3.94643146495612,127.866053469427));
#206021=CARTESIAN_POINT('Ctrl Pts',(190.299289744911,3.86154492337111,127.758436477459));
#206022=CARTESIAN_POINT('Ctrl Pts',(190.291529302397,3.77661307528294,127.650762047062));
#206023=CARTESIAN_POINT('Ctrl Pts',(190.283768859882,3.68724166038745,127.546728033458));
#206024=CARTESIAN_POINT('Ctrl Pts',(190.276008417368,3.59378981017076,127.446704014694));
#206025=CARTESIAN_POINT('Ctrl Pts',(190.268235517103,3.50018794274785,127.346519428494));
#206026=CARTESIAN_POINT('Ctrl Pts',(190.260462616837,3.40249282925593,127.250357975128));
#206027=CARTESIAN_POINT('Ctrl Pts',(190.252689716572,3.30109919916671,127.158551086096));
#206028=CARTESIAN_POINT('Ctrl Pts',(190.24519938081,3.2033914829259,127.070081608727));
#206029=CARTESIAN_POINT('Ctrl Pts',(190.237709045048,3.10224971882835,126.985655790931));
#206030=CARTESIAN_POINT('Ctrl Pts',(190.230218709286,2.99805270289559,126.905532196981));
#206031=CARTESIAN_POINT('Ctrl Pts',(190.222444375167,2.88990502543422,126.822370692614));
#206032=CARTESIAN_POINT('Ctrl Pts',(190.214670041048,2.7781232636251,126.743580659112));
#206033=CARTESIAN_POINT('Ctrl Pts',(190.206895706929,2.66309625889214,126.669496486984));
#206034=CARTESIAN_POINT('Ctrl Pts',(190.199130953982,2.54821101466232,126.595503616977));
#206035=CARTESIAN_POINT('Ctrl Pts',(190.191366201034,2.43008881080192,126.526205278626));
#206036=CARTESIAN_POINT('Ctrl Pts',(190.183601448087,2.30915117022697,126.461895426509));
#206037=CARTESIAN_POINT('Ctrl Pts',(190.175844407202,2.18833364662157,126.397649447844));
#206038=CARTESIAN_POINT('Ctrl Pts',(190.168087366317,2.06470659408811,126.33838227784));
#206039=CARTESIAN_POINT('Ctrl Pts',(190.160330325432,1.938719800928,126.284344179986));
#206040=CARTESIAN_POINT('Ctrl Pts',(190.152579134192,1.81282801538859,126.230346832682));
#206041=CARTESIAN_POINT('Ctrl Pts',(190.144827942952,1.68458038906157,126.181570862152));
#206042=CARTESIAN_POINT('Ctrl Pts',(190.137076751712,1.55445023485514,126.138220078549));
#206043=CARTESIAN_POINT('Ctrl Pts',(190.129328854935,1.42437538943564,126.094887720185));
#206044=CARTESIAN_POINT('Ctrl Pts',(190.121580958158,1.29241997767127,126.0569760859));
#206045=CARTESIAN_POINT('Ctrl Pts',(190.113833061381,1.1590759605821,126.024640334945));
#206046=CARTESIAN_POINT('Ctrl Pts',(190.106086785297,1.02575983618676,125.992311347931));
#206047=CARTESIAN_POINT('Ctrl Pts',(190.098340509213,0.891056063932395,
125.965556016384));
#206048=CARTESIAN_POINT('Ctrl Pts',(190.090594233128,0.755470004251004,
125.944479123622));
#206049=CARTESIAN_POINT('Ctrl Pts',(190.082847899863,0.619882943704145,
125.923402075275));
#206050=CARTESIAN_POINT('Ctrl Pts',(190.075101566598,0.483413969059678,
125.90800360941));
#206051=CARTESIAN_POINT('Ctrl Pts',(190.067355233332,0.346576434879642,
125.898336989689));
#206052=CARTESIAN_POINT('Ctrl Pts',(190.059607165329,0.20970825688259,125.888668205195));
#206053=CARTESIAN_POINT('Ctrl Pts',(190.051859097326,0.0724717450308378,
125.884733848621));
#206054=CARTESIAN_POINT('Ctrl Pts',(190.044111029323,-0.0646172497580651,
125.886535115016));
#206055=CARTESIAN_POINT('Ctrl Pts',(190.036354726582,-0.201851944362056,
125.888338295818));
#206056=CARTESIAN_POINT('Ctrl Pts',(190.02859842384,-0.33893841715767,125.89588927164));
#206057=CARTESIAN_POINT('Ctrl Pts',(190.020842121098,-0.475362889567487,
125.909137110338));
#206058=CARTESIAN_POINT('Ctrl Pts',(190.013081678584,-0.611860175825985,
125.922392019806));
#206059=CARTESIAN_POINT('Ctrl Pts',(190.00532123607,-0.747694370636893,
125.941349796762));
#206060=CARTESIAN_POINT('Ctrl Pts',(189.997560793555,-0.882360418181386,
125.965908059679));
#206061=CARTESIAN_POINT('Ctrl Pts',(189.98978789329,-1.01724264362044,125.990505745699));
#206062=CARTESIAN_POINT('Ctrl Pts',(189.982014993024,-1.15095259295001,
126.02072179713));
#206063=CARTESIAN_POINT('Ctrl Pts',(189.974242092759,-1.28299806253933,
126.056403263712));
#206064=CARTESIAN_POINT('Ctrl Pts',(189.966751756997,-1.4102433467065,126.090787619106));
#206065=CARTESIAN_POINT('Ctrl Pts',(189.959261421235,-1.53594277230061,
126.130246832991));
#206066=CARTESIAN_POINT('Ctrl Pts',(189.951771085473,-1.65967405337326,
126.17460197385));
#206067=CARTESIAN_POINT('Ctrl Pts',(189.943996623503,-1.78809875550871,
126.220639610442));
#206068=CARTESIAN_POINT('Ctrl Pts',(189.936222161534,-1.91480987036354,
126.272097770317));
#206069=CARTESIAN_POINT('Ctrl Pts',(189.928447699565,-2.03931586329617,
126.328830048772));
#206070=CARTESIAN_POINT('Ctrl Pts',(189.92068284859,-2.16366793863765,126.385492193289));
#206071=CARTESIAN_POINT('Ctrl Pts',(189.912917997615,-2.28581996373698,
126.447415322767));
#206072=CARTESIAN_POINT('Ctrl Pts',(189.905153146641,-2.40529676525213,
126.514403679138));
#206073=CARTESIAN_POINT('Ctrl Pts',(189.897396037425,-2.5246544452745,126.581325246367));
#206074=CARTESIAN_POINT('Ctrl Pts',(189.88963892821,-2.6413418709589,126.653301800276));
#206075=CARTESIAN_POINT('Ctrl Pts',(189.881881818995,-2.75490535575686,
126.730090186762));
#206076=CARTESIAN_POINT('Ctrl Pts',(189.874130589026,-2.86838276883409,
126.806820374008));
#206077=CARTESIAN_POINT('Ctrl Pts',(189.866379359057,-2.97874063130287,
126.888354916463));
#206078=CARTESIAN_POINT('Ctrl Pts',(189.858628129089,-3.08555162944487,
126.974405760844));
#206079=CARTESIAN_POINT('Ctrl Pts',(189.850880345889,-3.19231513152848,
127.060418340663));
#206080=CARTESIAN_POINT('Ctrl Pts',(189.84313256269,-3.29553460322023,127.150942982288));
#206081=CARTESIAN_POINT('Ctrl Pts',(189.835384779491,-3.39481360629566,
127.245649665408));
#206082=CARTESIAN_POINT('Ctrl Pts',(189.827638659146,-3.49407130178288,
127.340336022266));
#206083=CARTESIAN_POINT('Ctrl Pts',(189.819892538802,-3.58938992840192,
127.439202365372));
#206084=CARTESIAN_POINT('Ctrl Pts',(189.812146418457,-3.68040819178631,
127.541880180179));
#206085=CARTESIAN_POINT('Ctrl Pts',(189.804400283122,-3.77142663131764,
127.644558193698));
#206086=CARTESIAN_POINT('Ctrl Pts',(189.796654147786,-3.85814443183768,
127.751047400979));
#206087=CARTESIAN_POINT('Ctrl Pts',(189.788908012451,-3.94023932495192,
127.860944723642));
#206088=CARTESIAN_POINT('Ctrl Pts',(189.781160184633,-4.02235215528922,
127.970866058186));
#206089=CARTESIAN_POINT('Ctrl Pts',(189.773412356815,-4.0998398346877,128.084196676547));
#206090=CARTESIAN_POINT('Ctrl Pts',(189.765664528998,-4.17242255225989,
128.200503265887));
#206091=CARTESIAN_POINT('Ctrl Pts',(189.757909049044,-4.24507695609062,
128.31692472533));
#206092=CARTESIAN_POINT('Ctrl Pts',(189.750153569091,-4.31281651589305,
128.436327693783));
#206093=CARTESIAN_POINT('Ctrl Pts',(189.742398089138,-4.37540644239081,
128.55825253326));
#206094=CARTESIAN_POINT('Ctrl Pts',(189.734638486836,-4.43802963794533,
128.68024218068));
#206095=CARTESIAN_POINT('Ctrl Pts',(189.726878884534,-4.49549758245539,
128.804756015469));
#206096=CARTESIAN_POINT('Ctrl Pts',(189.719119282232,-4.54762346778534,
128.931313939624));
#206097=CARTESIAN_POINT('Ctrl Pts',(189.711348586192,-4.59982387637704,
129.058052800933));
#206098=CARTESIAN_POINT('Ctrl Pts',(189.703577890153,-4.64666683607839,
129.186841222174));
#206099=CARTESIAN_POINT('Ctrl Pts',(189.695807194114,-4.68801507639694,
129.317182852141));
#206100=CARTESIAN_POINT('Ctrl Pts',(189.690573763844,-4.71586240582347,
129.404965700449));
#206101=CARTESIAN_POINT('Ctrl Pts',(189.685340333575,-4.74121849260404,
129.493452762972));
#206102=CARTESIAN_POINT('Ctrl Pts',(189.680106903305,-4.76405452823404,
129.582490119308));
#206103=CARTESIAN_POINT('Ctrl Pts',(191.430300680169,-4.76051597898714,
129.583432241587));
#206104=CARTESIAN_POINT('Ctrl Pts',(191.406914637273,-4.86678982625872,
129.983174630901));
#206105=CARTESIAN_POINT('Ctrl Pts',(191.383528594377,-4.92378206388031,
130.394832064542));
#206106=CARTESIAN_POINT('Ctrl Pts',(191.360142551482,-4.9256493795537,130.806055125649));
#206107=CARTESIAN_POINT('Origin',(213.235140564004,0.,130.804360617566));
#206108=CARTESIAN_POINT('',(193.179932595466,-4.75726252818781,129.584191622251));
#206109=CARTESIAN_POINT('',(192.834981455508,-4.76405452823404,129.582490119308));
#206110=CARTESIAN_POINT('',(213.235140564004,-4.76405452823405,129.582490119308));
#206111=CARTESIAN_POINT('',(192.764859436031,-4.9182499011834,130.805346522958));
#206112=CARTESIAN_POINT('Ctrl Pts',(192.834981455508,-4.76405452823404,
129.582490119308));
#206113=CARTESIAN_POINT('Ctrl Pts',(192.827262795634,-4.79795815032377,
129.714679827277));
#206114=CARTESIAN_POINT('Ctrl Pts',(192.819544135761,-4.82632919785479,
129.848178265195));
#206115=CARTESIAN_POINT('Ctrl Pts',(192.811825475887,-4.84909224210237,
129.982480157838));
#206116=CARTESIAN_POINT('Ctrl Pts',(192.803997802578,-4.87217677708874,
130.118678844873));
#206117=CARTESIAN_POINT('Ctrl Pts',(192.796170129268,-4.88949364919261,
130.255703433094));
#206118=CARTESIAN_POINT('Ctrl Pts',(192.788342455959,-4.90101880375934,
130.393024079319));
#206119=CARTESIAN_POINT('Ctrl Pts',(192.78051478265,-4.91254395832607,130.530344725543));
#206120=CARTESIAN_POINT('Ctrl Pts',(192.77268710934,-4.91827744128822,130.667961010208));
#206121=CARTESIAN_POINT('Ctrl Pts',(192.764859436031,-4.9182499011834,130.805346522958));
#206122=CARTESIAN_POINT('Ctrl Pts',(192.764859435991,-4.91824990118326,
130.805346523653));
#206123=CARTESIAN_POINT('Ctrl Pts',(192.761851730581,-4.91823931916517,
130.85813553689));
#206124=CARTESIAN_POINT('Ctrl Pts',(192.758844025171,-4.91737886410589,
130.910915070119));
#206125=CARTESIAN_POINT('Ctrl Pts',(192.755836319761,-4.91566928905583,
130.963666936127));
#206126=CARTESIAN_POINT('Ctrl Pts',(192.748061985642,-4.91125036970399,
131.100020260621));
#206127=CARTESIAN_POINT('Ctrl Pts',(192.740287651523,-4.90114679519269,
131.236405558342));
#206128=CARTESIAN_POINT('Ctrl Pts',(192.732513317404,-4.88534711553905,
131.372310107569));
#206129=CARTESIAN_POINT('Ctrl Pts',(192.724748564456,-4.86956690757853,
131.508047166585));
#206130=CARTESIAN_POINT('Ctrl Pts',(192.716983811509,-4.84810460677939,
131.643304271342));
#206131=CARTESIAN_POINT('Ctrl Pts',(192.709219058562,-4.82100075318953,
131.77756912567));
#206132=CARTESIAN_POINT('Ctrl Pts',(192.701462017677,-4.79392381952918,
131.911700626251));
#206133=CARTESIAN_POINT('Ctrl Pts',(192.693704976792,-4.76121656070021,
132.044841456872));
#206134=CARTESIAN_POINT('Ctrl Pts',(192.685947935907,-4.72297121766863,
132.176485225455));
#206135=CARTESIAN_POINT('Ctrl Pts',(192.678196744667,-4.68475471574775,
132.308029720448));
#206136=CARTESIAN_POINT('Ctrl Pts',(192.670445553427,-4.6410085509534,132.43807902658));
#206137=CARTESIAN_POINT('Ctrl Pts',(192.662694362187,-4.59187578910414,
132.56613807228));
#206138=CARTESIAN_POINT('Ctrl Pts',(192.65494646541,-4.54276390998926,132.69414268947));
#206139=CARTESIAN_POINT('Ctrl Pts',(192.647198568633,-4.48827012711119,
132.820158364431));
#206140=CARTESIAN_POINT('Ctrl Pts',(192.639450671856,-4.42858693265309,
132.943706508822));
#206141=CARTESIAN_POINT('Ctrl Pts',(192.631704395771,-4.36891622263265,
133.067228809605));
#206142=CARTESIAN_POINT('Ctrl Pts',(192.623958119687,-4.30405843013184,
133.188284254661));
#206143=CARTESIAN_POINT('Ctrl Pts',(192.616211843603,-4.23425347381781,
133.30641588913));
#206144=CARTESIAN_POINT('Ctrl Pts',(192.608465510338,-4.16444800221951,
133.42454839562));
#206145=CARTESIAN_POINT('Ctrl Pts',(192.600719177073,-4.08969549283255,
133.539756711864));
#206146=CARTESIAN_POINT('Ctrl Pts',(192.592972843807,-4.01028074241126,
133.65161041861));
#206147=CARTESIAN_POINT('Ctrl Pts',(192.585224775804,-3.93084820760729,
133.763489174218));
#206148=CARTESIAN_POINT('Ctrl Pts',(192.577476707801,-3.84675158046991,
133.872011506716));
#206149=CARTESIAN_POINT('Ctrl Pts',(192.569728639798,-3.7583174692179,133.976778128404));
#206150=CARTESIAN_POINT('Ctrl Pts',(192.561972337057,-3.66978936913993,
134.081656097304));
#206151=CARTESIAN_POINT('Ctrl Pts',(192.554216034315,-3.57691482870239,
134.182770082479));
#206152=CARTESIAN_POINT('Ctrl Pts',(192.546459731573,-3.4800594120266,134.279755494593));
#206153=CARTESIAN_POINT('Ctrl Pts',(192.538699289059,-3.38315230069857,
134.376792670742));
#206154=CARTESIAN_POINT('Ctrl Pts',(192.530938846545,-3.28226036692496,
134.469696618379));
#206155=CARTESIAN_POINT('Ctrl Pts',(192.523178404031,-3.17778338449789,
134.558142154058));
#206156=CARTESIAN_POINT('Ctrl Pts',(192.515405503765,-3.07313868634362,
134.646729670363));
#206157=CARTESIAN_POINT('Ctrl Pts',(192.5076326035,-2.96489774802298,134.73084423263));
#206158=CARTESIAN_POINT('Ctrl Pts',(192.499859703234,-2.85349125072007,
134.810202694404));
#206159=CARTESIAN_POINT('Ctrl Pts',(192.492369367472,-2.74613466020842,
134.886676276202));
#206160=CARTESIAN_POINT('Ctrl Pts',(192.48487903171,-2.63583892488735,134.958733378042));
#206161=CARTESIAN_POINT('Ctrl Pts',(192.477388695948,-2.52301040503746,
135.026161365893));
#206162=CARTESIAN_POINT('Ctrl Pts',(192.469614361829,-2.40590395756583,
135.096145906396));
#206163=CARTESIAN_POINT('Ctrl Pts',(192.46184002771,-2.28569791514371,135.161365067826));
#206164=CARTESIAN_POINT('Ctrl Pts',(192.454065693591,-2.16281745608086,
135.221532078373));
#206165=CARTESIAN_POINT('Ctrl Pts',(192.446300940644,-2.04008843620172,
135.281624938458));
#206166=CARTESIAN_POINT('Ctrl Pts',(192.438536187696,-1.91469190546091,
135.336677865911));
#206167=CARTESIAN_POINT('Ctrl Pts',(192.430771434749,-1.78708078602292,
135.386448059631));
#206168=CARTESIAN_POINT('Ctrl Pts',(192.423014393864,-1.65959641174775,
135.436168820892));
#206169=CARTESIAN_POINT('Ctrl Pts',(192.415257352979,-1.52990218788621,
135.480617148817));
#206170=CARTESIAN_POINT('Ctrl Pts',(192.407500312094,-1.39847401492876,
135.519596931058));
#206171=CARTESIAN_POINT('Ctrl Pts',(192.399749120854,-1.26714495297885,
135.558547318341));
#206172=CARTESIAN_POINT('Ctrl Pts',(192.391997929614,-1.13408491791114,
135.592037257539));
#206173=CARTESIAN_POINT('Ctrl Pts',(192.384246738374,-0.999787758028332,
135.6199195157));
#206174=CARTESIAN_POINT('Ctrl Pts',(192.376498841597,-0.865547678020963,
135.647789923158));
#206175=CARTESIAN_POINT('Ctrl Pts',(192.36875094482,-0.730071900997154,
135.670057310698));
#206176=CARTESIAN_POINT('Ctrl Pts',(192.361003048043,-0.593867123607528,
135.686624938759));
#206177=CARTESIAN_POINT('Ctrl Pts',(192.353256771959,-0.457690837321097,
135.70318910123));
#206178=CARTESIAN_POINT('Ctrl Pts',(192.345510495875,-0.320786241840849,
135.714055828527));
#206179=CARTESIAN_POINT('Ctrl Pts',(192.337764219791,-0.18366746813134,
135.719179975757));
#206180=CARTESIAN_POINT('Ctrl Pts',(192.330017886525,-0.0465476822422854,
135.724304160812));
#206181=CARTESIAN_POINT('Ctrl Pts',(192.32227155326,0.0907858943383346,
135.723685666614));
#206182=CARTESIAN_POINT('Ctrl Pts',(192.314525219994,0.227817198101151,
135.717331448616));
#206183=CARTESIAN_POINT('Ctrl Pts',(192.306777151991,0.364879189074196,
135.710975807636));
#206184=CARTESIAN_POINT('Ctrl Pts',(192.299029083989,0.501638382059588,
135.698881905005));
#206185=CARTESIAN_POINT('Ctrl Pts',(192.291281015986,0.637582305285388,
135.681108700714));
#206186=CARTESIAN_POINT('Ctrl Pts',(192.283524713244,0.773670711330755,
135.663316606849));
#206187=CARTESIAN_POINT('Ctrl Pts',(192.275768410502,0.908941728448333,
135.639833204469));
#206188=CARTESIAN_POINT('Ctrl Pts',(192.26801210776,1.04289102096811,135.610768983579));
#206189=CARTESIAN_POINT('Ctrl Pts',(192.260251665246,1.17691180625858,135.58168925024));
#206190=CARTESIAN_POINT('Ctrl Pts',(192.252491222732,1.30960908320894,135.547022861951));
#206191=CARTESIAN_POINT('Ctrl Pts',(192.244730780217,1.44049317827798,135.50693039013));
#206192=CARTESIAN_POINT('Ctrl Pts',(192.236957879952,1.5715873801157,135.466773558314));
#206193=CARTESIAN_POINT('Ctrl Pts',(192.229184979687,1.70086221469286,135.42117336688));
#206194=CARTESIAN_POINT('Ctrl Pts',(192.221412079421,1.82784666917891,135.37033911253));
#206195=CARTESIAN_POINT('Ctrl Pts',(192.213921743659,1.95021491889024,135.321352811369));
#206196=CARTESIAN_POINT('Ctrl Pts',(192.206431407897,2.07045613849443,135.267506509144));
#206197=CARTESIAN_POINT('Ctrl Pts',(192.198941072135,2.18817178530026,135.209027154379));
#206198=CARTESIAN_POINT('Ctrl Pts',(192.191166738016,2.31035065663324,135.148330537103));
#206199=CARTESIAN_POINT('Ctrl Pts',(192.183392403897,2.43019568637188,135.082450339021));
#206200=CARTESIAN_POINT('Ctrl Pts',(192.175618069778,2.5472357860093,135.011589267518));
#206201=CARTESIAN_POINT('Ctrl Pts',(192.167853316831,2.66413164418405,134.940815525952));
#206202=CARTESIAN_POINT('Ctrl Pts',(192.160088563884,2.7782291190768,134.865073325257));
#206203=CARTESIAN_POINT('Ctrl Pts',(192.152323810936,2.88907911974915,134.784612481749));
#206204=CARTESIAN_POINT('Ctrl Pts',(192.144566770051,2.99981902263817,134.704231553085));
#206205=CARTESIAN_POINT('Ctrl Pts',(192.136809729166,3.10731755571858,134.619141536373));
#206206=CARTESIAN_POINT('Ctrl Pts',(192.129052688281,3.21115248827715,134.529636816659));
#206207=CARTESIAN_POINT('Ctrl Pts',(192.121301497041,3.3149091181053,134.440199593151));
#206208=CARTESIAN_POINT('Ctrl Pts',(192.113550305801,3.41500735156303,134.346354547366));
#206209=CARTESIAN_POINT('Ctrl Pts',(192.105799114561,3.51105638032787,134.248437584862));
#206210=CARTESIAN_POINT('Ctrl Pts',(192.098051217784,3.60706458569329,134.150562239679));
#206211=CARTESIAN_POINT('Ctrl Pts',(192.090303321007,3.69902673613745,134.048618698472));
#206212=CARTESIAN_POINT('Ctrl Pts',(192.08255542423,3.78658756001065,133.942980969388));
#206213=CARTESIAN_POINT('Ctrl Pts',(192.074809148146,3.87413006804709,133.83736533744));
#206214=CARTESIAN_POINT('Ctrl Pts',(192.067062872062,3.95727283142153,133.728057355462));
#206215=CARTESIAN_POINT('Ctrl Pts',(192.059316595977,4.03569996811177,133.615465174476));
#206216=CARTESIAN_POINT('Ctrl Pts',(192.051570262712,4.1141276837333,133.502872162361));
#206217=CARTESIAN_POINT('Ctrl Pts',(192.043823929447,4.18783947974799,133.386995223673));
#206218=CARTESIAN_POINT('Ctrl Pts',(192.036077596181,4.25656226304545,133.268272296851));
#206219=CARTESIAN_POINT('Ctrl Pts',(192.028329528178,4.32530043633368,133.149522782853));
#206220=CARTESIAN_POINT('Ctrl Pts',(192.020581460175,4.38904717787134,133.027926350791));
#206221=CARTESIAN_POINT('Ctrl Pts',(192.012833392173,4.4475750888561,132.903946026995));
#206222=CARTESIAN_POINT('Ctrl Pts',(192.005077089431,4.50616520400119,132.779833935435));
#206223=CARTESIAN_POINT('Ctrl Pts',(191.997320786689,4.55952524142413,132.653333245059));
#206224=CARTESIAN_POINT('Ctrl Pts',(191.989564483947,4.60747555374874,132.524927990297));
#206225=CARTESIAN_POINT('Ctrl Pts',(191.981804041433,4.65545145859881,132.396454201785));
#206226=CARTESIAN_POINT('Ctrl Pts',(191.974043598919,4.69801176383069,132.266074194861));
#206227=CARTESIAN_POINT('Ctrl Pts',(191.966283156404,4.73502688221655,132.134286738517));
#206228=CARTESIAN_POINT('Ctrl Pts',(191.958510256139,4.77210142055647,132.002287725248));
#206229=CARTESIAN_POINT('Ctrl Pts',(191.950737355874,4.80361289384034,131.868877128348));
#206230=CARTESIAN_POINT('Ctrl Pts',(191.942964455608,4.82948279537217,131.73456435423));
#206231=CARTESIAN_POINT('Ctrl Pts',(191.935474119846,4.85441226082101,131.605134187765));
#206232=CARTESIAN_POINT('Ctrl Pts',(191.927983784084,4.87410315800352,131.474866602682));
#206233=CARTESIAN_POINT('Ctrl Pts',(191.920493448322,4.88853100308117,131.344219575456));
#206234=CARTESIAN_POINT('Ctrl Pts',(191.912719114203,4.90350588429017,131.208619026484));
#206235=CARTESIAN_POINT('Ctrl Pts',(191.904944780084,4.91285817377069,131.0721801525));
#206236=CARTESIAN_POINT('Ctrl Pts',(191.897170445965,4.9165037801426,130.935408861902));
#206237=CARTESIAN_POINT('Ctrl Pts',(191.889405693018,4.92014489363048,130.798806129696));
#206238=CARTESIAN_POINT('Ctrl Pts',(191.881640940071,4.91809330722021,130.661872183078));
#206239=CARTESIAN_POINT('Ctrl Pts',(191.873876187123,4.91031645383257,130.525119886796));
#206240=CARTESIAN_POINT('Ctrl Pts',(191.866119146238,4.90254732452534,130.388503414822));
#206241=CARTESIAN_POINT('Ctrl Pts',(191.858362105353,4.88906426651891,130.252068621953));
#206242=CARTESIAN_POINT('Ctrl Pts',(191.850605064468,4.86988672827563,130.116329865154));
#206243=CARTESIAN_POINT('Ctrl Pts',(191.842853873228,4.85072365196311,129.980693470007));
#206244=CARTESIAN_POINT('Ctrl Pts',(191.835102681988,4.82587469733376,129.84575245173));
#206245=CARTESIAN_POINT('Ctrl Pts',(191.827351490748,4.79541122980165,129.712017173592));
#206246=CARTESIAN_POINT('Ctrl Pts',(191.819603593971,4.76496071005587,129.578338736515));
#206247=CARTESIAN_POINT('Ctrl Pts',(191.811855697194,4.72890051026299,129.445865400711));
#206248=CARTESIAN_POINT('Ctrl Pts',(191.804107800417,4.68735326106434,129.31509822682));
#206249=CARTESIAN_POINT('Ctrl Pts',(191.796361524333,4.64581470265456,129.184358406603));
#206250=CARTESIAN_POINT('Ctrl Pts',(191.788615248249,4.59879149613188,129.055324410796));
#206251=CARTESIAN_POINT('Ctrl Pts',(191.780868972164,4.54645628856314,128.928482615487));
#206252=CARTESIAN_POINT('Ctrl Pts',(191.773122638899,4.49412069466779,128.801639883861));
#206253=CARTESIAN_POINT('Ctrl Pts',(191.765376305634,4.43647317060039,128.676989746434));
#206254=CARTESIAN_POINT('Ctrl Pts',(191.757629972368,4.37373455287664,128.5549986806));
#206255=CARTESIAN_POINT('Ctrl Pts',(191.749881904365,4.31098188527447,128.432980295712));
#206256=CARTESIAN_POINT('Ctrl Pts',(191.742133836362,4.24313603409257,128.313622514967));
#206257=CARTESIAN_POINT('Ctrl Pts',(191.734385768359,4.17046364188854,128.197366932459));
#206258=CARTESIAN_POINT('Ctrl Pts',(191.726629465618,4.09771401260122,128.080987792135));
#206259=CARTESIAN_POINT('Ctrl Pts',(191.718873162876,4.02012780272054,127.967717768317));
#206260=CARTESIAN_POINT('Ctrl Pts',(191.711116860134,3.93801514032661,127.857969635863));
#206261=CARTESIAN_POINT('Ctrl Pts',(191.70335641762,3.85585865193233,127.748162927527));
#206262=CARTESIAN_POINT('Ctrl Pts',(191.695595975106,3.76917114412413,127.641882158914));
#206263=CARTESIAN_POINT('Ctrl Pts',(191.687835532591,3.67830220031926,127.539505952251));
#206264=CARTESIAN_POINT('Ctrl Pts',(191.680062632326,3.58728738561886,127.436965402214));
#206265=CARTESIAN_POINT('Ctrl Pts',(191.67228973206,3.49207799308258,127.338342220929));
#206266=CARTESIAN_POINT('Ctrl Pts',(191.664516831795,3.39306016596735,127.243977804914));
#206267=CARTESIAN_POINT('Ctrl Pts',(191.657026496033,3.29764188627902,127.153043773112));
#206268=CARTESIAN_POINT('Ctrl Pts',(191.649536160271,3.19868748848367,127.066064451937));
#206269=CARTESIAN_POINT('Ctrl Pts',(191.642045824509,3.09656904704697,126.983307987809));
#206270=CARTESIAN_POINT('Ctrl Pts',(191.63427149039,2.99057875386455,126.89741378719));
#206271=CARTESIAN_POINT('Ctrl Pts',(191.626497156271,2.88084400593911,126.815796897087));
#206272=CARTESIAN_POINT('Ctrl Pts',(191.618722822152,2.76774498488753,126.738801521804));
#206273=CARTESIAN_POINT('Ctrl Pts',(191.610958069205,2.65478534827152,126.661901036441));
#206274=CARTESIAN_POINT('Ctrl Pts',(191.603193316258,2.53847000824377,126.589610951247));
#206275=CARTESIAN_POINT('Ctrl Pts',(191.59542856331,2.41921284913904,126.522235881753));
#206276=CARTESIAN_POINT('Ctrl Pts',(191.587671522425,2.30007413792603,126.454927730128));
#206277=CARTESIAN_POINT('Ctrl Pts',(191.57991448154,2.17799976045686,126.392525070538));
#206278=CARTESIAN_POINT('Ctrl Pts',(191.572157440656,2.05343297218267,126.335289562945));
#206279=CARTESIAN_POINT('Ctrl Pts',(191.564406249415,1.92896012069234,126.278097217093));
#206280=CARTESIAN_POINT('Ctrl Pts',(191.556655058175,1.80199895334133,126.226064429886));
#206281=CARTESIAN_POINT('Ctrl Pts',(191.548903866935,1.67301742795112,126.179407023391));
#206282=CARTESIAN_POINT('Ctrl Pts',(191.541155970158,1.54409072314994,126.132769447539));
#206283=CARTESIAN_POINT('Ctrl Pts',(191.533408073381,1.41314573509101,126.09150284106));
#206284=CARTESIAN_POINT('Ctrl Pts',(191.525660176604,1.28067030513812,126.055774866836));
#206285=CARTESIAN_POINT('Ctrl Pts',(191.51791390052,1.14822258618934,126.020054366134));
#206286=CARTESIAN_POINT('Ctrl Pts',(191.510167624436,1.01424543935255,125.989870294983));
#206287=CARTESIAN_POINT('Ctrl Pts',(191.502421348352,0.879241386563487,
125.965340298674));
#206288=CARTESIAN_POINT('Ctrl Pts',(191.494675015086,0.744236337205225,
125.940810121289));
#206289=CARTESIAN_POINT('Ctrl Pts',(191.486928681821,0.608204751435609,
125.921934171922));
#206290=CARTESIAN_POINT('Ctrl Pts',(191.479182348555,0.471658457426965,
125.908778796981));
#206291=CARTESIAN_POINT('Ctrl Pts',(191.471434280553,0.335081584822615,
125.895620475986));
#206292=CARTESIAN_POINT('Ctrl Pts',(191.46368621255,0.197990163703318,125.888185316112));
#206293=CARTESIAN_POINT('Ctrl Pts',(191.455938144547,0.0608998465023526,
125.886487675816));
#206294=CARTESIAN_POINT('Ctrl Pts',(191.448181841805,-0.0763361719192702,
125.884788231248));
#206295=CARTESIAN_POINT('Ctrl Pts',(191.440425539063,-0.21357069252026,
125.888838492329));
#206296=CARTESIAN_POINT('Ctrl Pts',(191.432669236321,-0.350288804319249,
125.898600654414));
#206297=CARTESIAN_POINT('Ctrl Pts',(191.424908793807,-0.487079886691054,
125.908368026859));
#206298=CARTESIAN_POINT('Ctrl Pts',(191.417148351293,-0.623353622783719,
125.923853330808));
#206299=CARTESIAN_POINT('Ctrl Pts',(191.409387908778,-0.758602508617255,
125.944967106394));
#206300=CARTESIAN_POINT('Ctrl Pts',(191.401615008513,-0.894068507969185,
125.966114775688));
#206301=CARTESIAN_POINT('Ctrl Pts',(191.393842108248,-1.02850598582216,
125.992908895609));
#206302=CARTESIAN_POINT('Ctrl Pts',(191.386069207982,-1.16141899575531,
126.025209126056));
#206303=CARTESIAN_POINT('Ctrl Pts',(191.37857887222,-1.28950028298996,126.056335161768));
#206304=CARTESIAN_POINT('Ctrl Pts',(191.371088536458,-1.41616571838099,
126.092573851485));
#206305=CARTESIAN_POINT('Ctrl Pts',(191.363598200696,-1.54098858741563,
126.13375709811));
#206306=CARTESIAN_POINT('Ctrl Pts',(191.355823866577,-1.67054415346853,
126.176501820048));
#206307=CARTESIAN_POINT('Ctrl Pts',(191.348049532458,-1.79852506629693,
126.224708848623));
#206308=CARTESIAN_POINT('Ctrl Pts',(191.340275198339,-1.92443623961998,
126.278244377108));
#206309=CARTESIAN_POINT('Ctrl Pts',(191.332510445392,-2.05019223867488,
126.331713927838));
#206310=CARTESIAN_POINT('Ctrl Pts',(191.324745692445,-2.17388321715495,
126.390498760795));
#206311=CARTESIAN_POINT('Ctrl Pts',(191.316980939498,-2.29502917879571,
126.454415315499));
#206312=CARTESIAN_POINT('Ctrl Pts',(191.309223898613,-2.41605481655935,
126.51826838738));
#206313=CARTESIAN_POINT('Ctrl Pts',(191.301466857728,-2.53454012426197,
126.587242856692));
#206314=CARTESIAN_POINT('Ctrl Pts',(191.293709816843,-2.65002536956902,
126.661107233673));
#206315=CARTESIAN_POINT('Ctrl Pts',(191.285958625602,-2.76542352655441,
126.734915908953));
#206316=CARTESIAN_POINT('Ctrl Pts',(191.278207434362,-2.87782579622934,
126.813606942315));
#206317=CARTESIAN_POINT('Ctrl Pts',(191.270456243122,-2.98679765874186,
126.896903284692));
#206318=CARTESIAN_POINT('Ctrl Pts',(191.262708346345,-3.09572320530585,
126.980164223901));
#206319=CARTESIAN_POINT('Ctrl Pts',(191.254960449568,-3.20122093462301,
127.068026342114));
#206320=CARTESIAN_POINT('Ctrl Pts',(191.247212552791,-3.302886096988,127.160169830461));
#206321=CARTESIAN_POINT('Ctrl Pts',(191.239466276707,-3.40452999319271,
127.252294044376));
#206322=CARTESIAN_POINT('Ctrl Pts',(191.231720000623,-3.50234262754816,
127.348697584696));
#206323=CARTESIAN_POINT('Ctrl Pts',(191.223973724539,-3.59595339635909,
127.449021255636));
#206324=CARTESIAN_POINT('Ctrl Pts',(191.216227391273,-3.68956485618348,
127.549345667144));
#206325=CARTESIAN_POINT('Ctrl Pts',(191.208481058008,-3.77897412184559,
127.653589981163));
#206326=CARTESIAN_POINT('Ctrl Pts',(191.200734724743,-3.86384871860262,
127.761359444012));
#206327=CARTESIAN_POINT('Ctrl Pts',(191.19298665674,-3.94874232243708,127.869153041084));
#206328=CARTESIAN_POINT('Ctrl Pts',(191.185238588737,-4.02909899477355,
127.980473050777));
#206329=CARTESIAN_POINT('Ctrl Pts',(191.177490520734,-4.10462793269824,
128.094893401191));
#206330=CARTESIAN_POINT('Ctrl Pts',(191.169734217992,-4.18023714367694,
128.209435358914));
#206331=CARTESIAN_POINT('Ctrl Pts',(191.16197791525,-4.251008154845,128.327083912827));
#206332=CARTESIAN_POINT('Ctrl Pts',(191.154221612508,-4.31669445035687,
128.447385419402));
#206333=CARTESIAN_POINT('Ctrl Pts',(191.146461169994,-4.38241580462248,
128.567751134514));
#206334=CARTESIAN_POINT('Ctrl Pts',(191.13870072748,-4.44304686287264,128.690772273196));
#206335=CARTESIAN_POINT('Ctrl Pts',(191.130940284966,-4.49838857192929,
128.815973502732));
#206336=CARTESIAN_POINT('Ctrl Pts',(191.1231673847,-4.5538191204103,128.941375716397));
#206337=CARTESIAN_POINT('Ctrl Pts',(191.115394484435,-4.603943209069,129.068964650282));
#206338=CARTESIAN_POINT('Ctrl Pts',(191.107621584169,-4.64861083885302,
129.198247193365));
#206339=CARTESIAN_POINT('Ctrl Pts',(191.100131248407,-4.69165468778338,
129.322829990364));
#206340=CARTESIAN_POINT('Ctrl Pts',(191.092640912645,-4.72963181359555,
129.44898510548));
#206341=CARTESIAN_POINT('Ctrl Pts',(191.085150576883,-4.76245299152071,
129.576262671124));
#206342=CARTESIAN_POINT('Ctrl Pts',(191.085028435562,-4.76298819076576,
129.578338125491));
#206343=CARTESIAN_POINT('Ctrl Pts',(191.08490629424,-4.76352203648398,129.580413942056));
#206344=CARTESIAN_POINT('Ctrl Pts',(191.084784152919,-4.76405452823405,
129.582490119308));
#206345=CARTESIAN_POINT('',(193.110140564008,-4.91324924050575,130.80805185308));
#206346=CARTESIAN_POINT('Ctrl Pts',(193.110140564008,-4.91324924050575,
130.80805185308));
#206347=CARTESIAN_POINT('Ctrl Pts',(193.078325358477,-4.91715556795767,
131.371134307201));
#206348=CARTESIAN_POINT('Ctrl Pts',(192.953694278342,-4.56730227853154,
133.572215041493));
#206349=CARTESIAN_POINT('Ctrl Pts',(192.736247323602,-1.31701101669081,
136.470678805982));
#206350=CARTESIAN_POINT('Ctrl Pts',(192.457799699789,4.05535734608101,134.975182673953));
#206351=CARTESIAN_POINT('Ctrl Pts',(192.179352075976,5.70105042302464,129.646904828089));
#206352=CARTESIAN_POINT('Ctrl Pts',(191.900904452163,2.10775667300519,125.382272307895));
#206353=CARTESIAN_POINT('Ctrl Pts',(191.651220653561,-2.85118716275981,
126.026104000732));
#206354=CARTESIAN_POINT('Ctrl Pts',(191.494352729563,-4.4694424636812,128.488577529337));
#206355=CARTESIAN_POINT('Ctrl Pts',(191.430300680169,-4.76051597898714,
129.583432241587));
#206356=CARTESIAN_POINT('Ctrl Pts',(193.179932595466,-4.75726252818781,
129.584191622251));
#206357=CARTESIAN_POINT('Ctrl Pts',(193.15666858498,-4.85769551258501,129.983931752434));
#206358=CARTESIAN_POINT('Ctrl Pts',(193.133404574494,-4.9103928439719,130.396313003733));
#206359=CARTESIAN_POINT('Ctrl Pts',(193.110140564008,-4.91324924050575,
130.80805185308));
#206360=CARTESIAN_POINT('Origin',(213.235140564004,0.,130.804360617566));
#206361=CARTESIAN_POINT('',(194.92989654745,-4.76405452823404,129.582490119308));
#206362=CARTESIAN_POINT('',(194.584773235637,-4.76405452823404,129.582490119308));
#206363=CARTESIAN_POINT('',(213.235140564004,-4.76405452823405,129.582490119308));
#206364=CARTESIAN_POINT('',(194.514859435944,-4.91824832267119,130.808422518846));
#206365=CARTESIAN_POINT('Ctrl Pts',(194.584773235637,-4.76405452823405,
129.582490119308));
#206366=CARTESIAN_POINT('Ctrl Pts',(194.577053952228,-4.79804027850044,
129.715000043791));
#206367=CARTESIAN_POINT('Ctrl Pts',(194.569334668819,-4.82650137584579,
129.848960603857));
#206368=CARTESIAN_POINT('Ctrl Pts',(194.56161538541,-4.84932764823365,129.983870262609));
#206369=CARTESIAN_POINT('Ctrl Pts',(194.553822727173,-4.87237089332568,
130.120062290773));
#206370=CARTESIAN_POINT('Ctrl Pts',(194.546030068937,-4.88967153265256,
130.257221158943));
#206371=CARTESIAN_POINT('Ctrl Pts',(194.5382374107,-4.90116937806975,130.394822109033));
#206372=CARTESIAN_POINT('Ctrl Pts',(194.530444752464,-4.91266722348695,
130.532423059123));
#206373=CARTESIAN_POINT('Ctrl Pts',(194.522652094227,-4.91836225895716,
130.670465679262));
#206374=CARTESIAN_POINT('Ctrl Pts',(194.514859435991,-4.91824832267189,
130.808422518005));
#206375=CARTESIAN_POINT('Ctrl Pts',(194.514859435944,-4.91824832267119,
130.808422518846));
#206376=CARTESIAN_POINT('Ctrl Pts',(194.505690899192,-4.91811426966856,
130.970737137015));
#206377=CARTESIAN_POINT('Ctrl Pts',(194.49652236244,-4.90994121534633,131.132707678005));
#206378=CARTESIAN_POINT('Ctrl Pts',(194.487353825688,-4.89385416878415,
131.293619687154));
#206379=CARTESIAN_POINT('Ctrl Pts',(194.478119857513,-4.87765231673291,
131.45568004767));
#206380=CARTESIAN_POINT('Ctrl Pts',(194.468885889339,-4.85342321642564,
131.616666662758));
#206381=CARTESIAN_POINT('Ctrl Pts',(194.459651921164,-4.82134334935995,
131.775870458012));
#206382=CARTESIAN_POINT('Ctrl Pts',(194.450346899683,-4.78901663493732,
131.936299290638));
#206383=CARTESIAN_POINT('Ctrl Pts',(194.441041878201,-4.74871793267665,
132.094917714119));
#206384=CARTESIAN_POINT('Ctrl Pts',(194.43173685672,-4.70067592055807,132.251021929825));
#206385=CARTESIAN_POINT('Ctrl Pts',(194.429998592026,-4.69170122515761,
132.280183651511));
#206386=CARTESIAN_POINT('Ctrl Pts',(194.428260327332,-4.68245643851761,
132.309257694875));
#206387=CARTESIAN_POINT('Ctrl Pts',(194.426522062638,-4.67294323328106,
132.338239557063));
#206388=CARTESIAN_POINT('Ctrl Pts',(194.418747728519,-4.63039572235757,
132.467860023283));
#206389=CARTESIAN_POINT('Ctrl Pts',(194.4109733944,-4.58238351476863,132.595914150803));
#206390=CARTESIAN_POINT('Ctrl Pts',(194.403199060281,-4.5290396636491,132.721906650284));
#206391=CARTESIAN_POINT('Ctrl Pts',(194.395434307334,-4.47576155405861,
132.84774387527));
#206392=CARTESIAN_POINT('Ctrl Pts',(194.387669554386,-4.41716502578731,
132.971524171027));
#206393=CARTESIAN_POINT('Ctrl Pts',(194.379904801439,-4.35343290862853,
133.092767262498));
#206394=CARTESIAN_POINT('Ctrl Pts',(194.372147760554,-4.28976409110701,
133.213889933622));
#206395=CARTESIAN_POINT('Ctrl Pts',(194.364390719669,-4.22097001613394,
133.332480071522));
#206396=CARTESIAN_POINT('Ctrl Pts',(194.356633678784,-4.14728147357108,
133.448077592107));
#206397=CARTESIAN_POINT('Ctrl Pts',(194.348882487544,-4.07364850011134,
133.563587939702));
#206398=CARTESIAN_POINT('Ctrl Pts',(194.341131296304,-3.99512861499202,
133.676109833574));
#206399=CARTESIAN_POINT('Ctrl Pts',(194.333380105064,-3.91199820569556,
133.785208332753));
#206400=CARTESIAN_POINT('Ctrl Pts',(194.325632208287,-3.82890312904064,
133.894260462159));
#206401=CARTESIAN_POINT('Ctrl Pts',(194.31788431151,-3.74120166215483,133.999891780499));
#206402=CARTESIAN_POINT('Ctrl Pts',(194.310136414733,-3.64921299757971,
134.101697051841));
#206403=CARTESIAN_POINT('Ctrl Pts',(194.302390138649,-3.55724357505019,
134.203481027715));
#206404=CARTESIAN_POINT('Ctrl Pts',(194.294643862565,-3.46098900054278,
134.301440258582));
#206405=CARTESIAN_POINT('Ctrl Pts',(194.286897586481,-3.3608079054297,134.395203594542));
#206406=CARTESIAN_POINT('Ctrl Pts',(194.279151253215,-3.26062607080245,
134.488967622642));
#206407=CARTESIAN_POINT('Ctrl Pts',(194.27140491995,-3.15651794317866,134.578535426871));
#206408=CARTESIAN_POINT('Ctrl Pts',(194.263658586685,-3.04887776981329,
134.663573932121));
#206409=CARTESIAN_POINT('Ctrl Pts',(194.255910518682,-2.94121349117735,
134.748631481155));
#206410=CARTESIAN_POINT('Ctrl Pts',(194.248162450679,-2.83001589956761,
134.829157470545));
#206411=CARTESIAN_POINT('Ctrl Pts',(194.240414382676,-2.71571062383656,
134.904860449304));
#206412=CARTESIAN_POINT('Ctrl Pts',(194.232658079934,-2.60128386309834,
134.980643886089));
#206413=CARTESIAN_POINT('Ctrl Pts',(194.224901777192,-2.48374314685267,
135.051593856377));
#206414=CARTESIAN_POINT('Ctrl Pts',(194.21714547445,-2.36354174294401,135.11746315424));
#206415=CARTESIAN_POINT('Ctrl Pts',(194.209385031936,-2.24327618392683,
135.18336760853));
#206416=CARTESIAN_POINT('Ctrl Pts',(194.201624589422,-2.12034745785099,
135.244185813801));
#206417=CARTESIAN_POINT('Ctrl Pts',(194.193864146908,-1.99523059395582,
135.299717993731));
#206418=CARTESIAN_POINT('Ctrl Pts',(194.186091246642,-1.86991288136339,
135.355339318846));
#206419=CARTESIAN_POINT('Ctrl Pts',(194.178318346377,-1.74240037555429,
135.4056575181));
#206420=CARTESIAN_POINT('Ctrl Pts',(194.170545446111,-1.61318595870733,
135.450521842182));
#206421=CARTESIAN_POINT('Ctrl Pts',(194.16305511035,-1.48866881138538,135.493755235078));
#206422=CARTESIAN_POINT('Ctrl Pts',(194.155564774588,-1.36257163707573,
135.531924303522));
#206423=CARTESIAN_POINT('Ctrl Pts',(194.148074438826,-1.23534416706417,
135.564939138229));
#206424=CARTESIAN_POINT('Ctrl Pts',(194.140300104707,-1.10329282885606,
135.599205740429));
#206425=CARTESIAN_POINT('Ctrl Pts',(194.132525770587,-0.969605493727146,
135.628028094229));
#206426=CARTESIAN_POINT('Ctrl Pts',(194.124751436468,-0.834770781094737,
135.651250425013));
#206427=CARTESIAN_POINT('Ctrl Pts',(194.116986683521,-0.700102240195215,
135.67444413635));
#206428=CARTESIAN_POINT('Ctrl Pts',(194.109221930574,-0.564289516904608,
135.692051490933));
#206429=CARTESIAN_POINT('Ctrl Pts',(194.101457177627,-0.427835504199164,
135.703966708248));
#206430=CARTESIAN_POINT('Ctrl Pts',(194.093700136742,-0.29151701954285,
135.715870091201));
#206431=CARTESIAN_POINT('Ctrl Pts',(194.085943095857,-0.154558899969262,
135.722092553836));
#206432=CARTESIAN_POINT('Ctrl Pts',(194.078186054972,-0.0174729748113956,
135.722579579513));
#206433=CARTESIAN_POINT('Ctrl Pts',(194.070434863732,0.119509572784076,
135.723066237919));
#206434=CARTESIAN_POINT('Ctrl Pts',(194.062683672492,0.256619344746097,
135.717826066908));
#206435=CARTESIAN_POINT('Ctrl Pts',(194.054932481252,0.393341018732792,
135.706856502876));
#206436=CARTESIAN_POINT('Ctrl Pts',(194.047184584475,0.530004582360826,
135.695891601202));
#206437=CARTESIAN_POINT('Ctrl Pts',(194.039436687697,0.666279987193505,
135.679202181027));
#206438=CARTESIAN_POINT('Ctrl Pts',(194.03168879092,0.801653765399529,135.656837748158));
#206439=CARTESIAN_POINT('Ctrl Pts',(194.023942514836,0.936999226329496,
135.634477993447));
#206440=CARTESIAN_POINT('Ctrl Pts',(194.016196238752,1.07144305027789,135.606445650913));
#206441=CARTESIAN_POINT('Ctrl Pts',(194.008449962668,1.20447912930477,135.572841831702));
#206442=CARTESIAN_POINT('Ctrl Pts',(194.000703629403,1.33751619037367,135.539237764435));
#206443=CARTESIAN_POINT('Ctrl Pts',(193.992957296137,1.46914510672559,135.50006223417));
#206444=CARTESIAN_POINT('Ctrl Pts',(193.985210962872,1.59887255256962,135.455466897059));
#206445=CARTESIAN_POINT('Ctrl Pts',(193.977462894869,1.72862904997563,135.410861573131));
#206446=CARTESIAN_POINT('Ctrl Pts',(193.969714826866,1.85648285988052,135.360834154252));
#206447=CARTESIAN_POINT('Ctrl Pts',(193.961966758863,1.98195871352415,135.305585197654));
#206448=CARTESIAN_POINT('Ctrl Pts',(193.954210456121,2.10756792439832,135.250277521806));
#206449=CARTESIAN_POINT('Ctrl Pts',(193.946454153379,2.2307937720316,135.189737380293));
#206450=CARTESIAN_POINT('Ctrl Pts',(193.938697850637,2.35118327273367,135.124212499346));
#206451=CARTESIAN_POINT('Ctrl Pts',(193.930937408123,2.47163702893723,135.058652645797));
#206452=CARTESIAN_POINT('Ctrl Pts',(193.923176965609,2.58925108663829,134.988102952543));
#206453=CARTESIAN_POINT('Ctrl Pts',(193.915416523095,2.70360060345122,134.912855091156));
#206454=CARTESIAN_POINT('Ctrl Pts',(193.907643622829,2.81813368425998,134.837486435221));
#206455=CARTESIAN_POINT('Ctrl Pts',(193.899870722564,2.92939143443346,134.757404768529));
#206456=CARTESIAN_POINT('Ctrl Pts',(193.892097822299,3.03698060945102,134.672943283132));
#206457=CARTESIAN_POINT('Ctrl Pts',(193.884607486536,3.14065864695626,134.591552185475));
#206458=CARTESIAN_POINT('Ctrl Pts',(193.877117150774,3.24092996805332,134.506094375295));
#206459=CARTESIAN_POINT('Ctrl Pts',(193.869626815012,3.33747583876709,134.416899626095));
#206460=CARTESIAN_POINT('Ctrl Pts',(193.861852480893,3.43768227551313,134.32432303087));
#206461=CARTESIAN_POINT('Ctrl Pts',(193.854078146774,3.53419260818798,134.227427275858));
#206462=CARTESIAN_POINT('Ctrl Pts',(193.846303812655,3.62661166846604,134.126539250428));
#206463=CARTESIAN_POINT('Ctrl Pts',(193.838539059708,3.71891683051201,134.025775560474));
#206464=CARTESIAN_POINT('Ctrl Pts',(193.830774306761,3.80714049093836,133.921029675189));
#206465=CARTESIAN_POINT('Ctrl Pts',(193.823009553814,3.8909218276634,133.812667515725));
#206466=CARTESIAN_POINT('Ctrl Pts',(193.815252512929,3.97461995158371,133.704412983086));
#206467=CARTESIAN_POINT('Ctrl Pts',(193.807495472044,4.05388429464595,133.59254963128));
#206468=CARTESIAN_POINT('Ctrl Pts',(193.799738431159,4.12839233419866,133.477478609243));
#206469=CARTESIAN_POINT('Ctrl Pts',(193.791987239919,4.20284418665918,133.36249436316));
#206470=CARTESIAN_POINT('Ctrl Pts',(193.784236048679,4.27254666321562,133.244307588428));
#206471=CARTESIAN_POINT('Ctrl Pts',(193.776484857438,4.33721906272395,133.123350454638));
#206472=CARTESIAN_POINT('Ctrl Pts',(193.768736960661,4.40186397473727,133.002444730857));
#206473=CARTESIAN_POINT('Ctrl Pts',(193.760989063884,4.46148287789932,132.878771333985));
#206474=CARTESIAN_POINT('Ctrl Pts',(193.753241167107,4.51583988094174,132.752789018148));
#206475=CARTESIAN_POINT('Ctrl Pts',(193.745494891023,4.57018551367091,132.626833055096));
#206476=CARTESIAN_POINT('Ctrl Pts',(193.737748614939,4.61927128079769,132.498569492494));
#206477=CARTESIAN_POINT('Ctrl Pts',(193.730002338855,4.66290868628648,132.368478786329));
#206478=CARTESIAN_POINT('Ctrl Pts',(193.72225600559,4.70654641389667,132.238387119863));
#206479=CARTESIAN_POINT('Ctrl Pts',(193.714509672324,4.74473557527959,132.106468653588));
#206480=CARTESIAN_POINT('Ctrl Pts',(193.706763339059,4.77733710840989,131.973220410317));
#206481=CARTESIAN_POINT('Ctrl Pts',(193.699015271056,4.80994594242749,131.839942327026));
#206482=CARTESIAN_POINT('Ctrl Pts',(193.691267203053,4.83696456533113,131.705334253853));
#206483=CARTESIAN_POINT('Ctrl Pts',(193.68351913505,4.85830481722543,131.569904453949));
#206484=CARTESIAN_POINT('Ctrl Pts',(193.675762832308,4.87966774979339,131.434330717642));
#206485=CARTESIAN_POINT('Ctrl Pts',(193.668006529566,4.89534019475674,131.297933896828));
#206486=CARTESIAN_POINT('Ctrl Pts',(193.660250226825,4.9052857224612,131.161229001593));
#206487=CARTESIAN_POINT('Ctrl Pts',(193.65248978431,4.91523655839326,131.02445114284));
#206488=CARTESIAN_POINT('Ctrl Pts',(193.644729341796,4.91945437445847,130.887365272617));
#206489=CARTESIAN_POINT('Ctrl Pts',(193.636968899282,4.9179549245226,130.750486478465));
#206490=CARTESIAN_POINT('Ctrl Pts',(193.629195999017,4.91645306753658,130.613387954321));
#206491=CARTESIAN_POINT('Ctrl Pts',(193.621423098751,4.90921562490836,130.476497561166));
#206492=CARTESIAN_POINT('Ctrl Pts',(193.613650198486,4.89631036227887,130.340326245196));
#206493=CARTESIAN_POINT('Ctrl Pts',(193.606159862724,4.88387423845236,130.209105099557));
#206494=CARTESIAN_POINT('Ctrl Pts',(193.598669526962,4.86617526077355,130.078551963462));
#206495=CARTESIAN_POINT('Ctrl Pts',(193.5911791912,4.84331859353017,129.949113247465));
#206496=CARTESIAN_POINT('Ctrl Pts',(193.583404857081,4.81959530880109,129.814766823208));
#206497=CARTESIAN_POINT('Ctrl Pts',(193.575630522962,4.79024035808555,129.68119542462));
#206498=CARTESIAN_POINT('Ctrl Pts',(193.567856188842,4.75531516453582,129.548908209692));
#206499=CARTESIAN_POINT('Ctrl Pts',(193.560091435895,4.7204330131658,129.416784026935));
#206500=CARTESIAN_POINT('Ctrl Pts',(193.552326682948,4.67999437676145,129.285941253237));
#206501=CARTESIAN_POINT('Ctrl Pts',(193.544561930001,4.63411208200157,129.156881247757));
#206502=CARTESIAN_POINT('Ctrl Pts',(193.536804889116,4.5882753581837,129.027949426493));
#206503=CARTESIAN_POINT('Ctrl Pts',(193.529047848231,4.53700586573875,128.900797215727));
#206504=CARTESIAN_POINT('Ctrl Pts',(193.521290807346,4.48046677125739,128.775912793697));
#206505=CARTESIAN_POINT('Ctrl Pts',(193.513539616106,4.42397031334695,128.651122547982));
#206506=CARTESIAN_POINT('Ctrl Pts',(193.505788424866,4.36221232369776,128.528597041763));
#206507=CARTESIAN_POINT('Ctrl Pts',(193.498037233626,4.29540467300197,128.408806035084));
#206508=CARTESIAN_POINT('Ctrl Pts',(193.490289336849,4.22862541733986,128.289065942777));
#206509=CARTESIAN_POINT('Ctrl Pts',(193.482541440072,4.1568009593707,128.172058379152));
#206510=CARTESIAN_POINT('Ctrl Pts',(193.474793543294,4.08018975694076,128.058229774023));
#206511=CARTESIAN_POINT('Ctrl Pts',(193.46704726721,4.00359457992282,127.944424979385));
#206512=CARTESIAN_POINT('Ctrl Pts',(193.459300991126,3.92221486821154,127.833798144722));
#206513=CARTESIAN_POINT('Ctrl Pts',(193.451554715042,3.83635295632385,127.726767555284));
#206514=CARTESIAN_POINT('Ctrl Pts',(193.443808381777,3.75049041062306,127.619736175771));
#206515=CARTESIAN_POINT('Ctrl Pts',(193.436062048511,3.66014584337031,127.516301399417));
#206516=CARTESIAN_POINT('Ctrl Pts',(193.428315715246,3.56566224751357,127.416848876013));
#206517=CARTESIAN_POINT('Ctrl Pts',(193.420567647243,3.47115749271066,127.317374080907));
#206518=CARTESIAN_POINT('Ctrl Pts',(193.41281957924,3.3725121340977,127.221883596716));
#206519=CARTESIAN_POINT('Ctrl Pts',(193.405071511237,3.27010613528105,127.130726323506));
#206520=CARTESIAN_POINT('Ctrl Pts',(193.397315208495,3.16759129815017,127.03947216726));
#206521=CARTESIAN_POINT('Ctrl Pts',(193.389558905753,3.06130812916382,126.952560682118));
#206522=CARTESIAN_POINT('Ctrl Pts',(193.381802603011,2.95167022977636,126.870300892911));
#206523=CARTESIAN_POINT('Ctrl Pts',(193.374042160497,2.8419738133408,126.787997199178));
#206524=CARTESIAN_POINT('Ctrl Pts',(193.366281717983,2.72891942085808,126.710350369704));
#206525=CARTESIAN_POINT('Ctrl Pts',(193.358521275469,2.61294892541234,126.637625567711));
#206526=CARTESIAN_POINT('Ctrl Pts',(193.350748375203,2.49679226383197,126.564784021411));
#206527=CARTESIAN_POINT('Ctrl Pts',(193.342975474938,2.37771048460871,126.496880485635));
#206528=CARTESIAN_POINT('Ctrl Pts',(193.335202574673,2.25617009023159,126.434134126131));
#206529=CARTESIAN_POINT('Ctrl Pts',(193.32771223891,2.13904799533144,126.373668754842));
#206530=CARTESIAN_POINT('Ctrl Pts',(193.320221903148,2.01964321472039,126.317992247027));
#206531=CARTESIAN_POINT('Ctrl Pts',(193.312731567386,1.89838817010611,126.2672574208));
#206532=CARTESIAN_POINT('Ctrl Pts',(193.304957233267,1.77253570362098,126.214598968217));
#206533=CARTESIAN_POINT('Ctrl Pts',(193.297182899148,1.64429123515347,126.167097516029));
#206534=CARTESIAN_POINT('Ctrl Pts',(193.289408565029,1.51411633445749,126.124976599532));
#206535=CARTESIAN_POINT('Ctrl Pts',(193.281643812082,1.38410186269265,126.082907593301));
#206536=CARTESIAN_POINT('Ctrl Pts',(193.273879059135,1.25216206077593,126.046206048193));
#206537=CARTESIAN_POINT('Ctrl Pts',(193.266114306188,1.11877972194069,126.015048036801));
#206538=CARTESIAN_POINT('Ctrl Pts',(193.258357265303,0.985529860324888,
125.983920971985));
#206539=CARTESIAN_POINT('Ctrl Pts',(193.250600224418,0.850840691275775,
125.958326572221));
#206540=CARTESIAN_POINT('Ctrl Pts',(193.242843183533,0.715211128500449,
125.9383914331));
#206541=CARTESIAN_POINT('Ctrl Pts',(193.235091992293,0.579683845033364,
125.918471327223));
#206542=CARTESIAN_POINT('Ctrl Pts',(193.227340801053,0.443217964620638,
125.904202044029));
#206543=CARTESIAN_POINT('Ctrl Pts',(193.219589609812,0.306323230974984,
125.895659247482));
#206544=CARTESIAN_POINT('Ctrl Pts',(193.211841713035,0.169486681242845,
125.887120081852));
#206545=CARTESIAN_POINT('Ctrl Pts',(193.204093816258,0.0322220301962203,
125.884302586307));
#206546=CARTESIAN_POINT('Ctrl Pts',(193.196345919481,-0.10495542533834,
125.887230619163));
#206547=CARTESIAN_POINT('Ctrl Pts',(193.188599643397,-0.24210418630643,
125.890158039538));
#206548=CARTESIAN_POINT('Ctrl Pts',(193.180853367313,-0.379165397413132,
125.898828589448));
#206549=CARTESIAN_POINT('Ctrl Pts',(193.173107091229,-0.515623724240199,
125.913213999696));
#206550=CARTESIAN_POINT('Ctrl Pts',(193.165360757964,-0.65208305837159,
125.927599516134));
#206551=CARTESIAN_POINT('Ctrl Pts',(193.157614424698,-0.787939110532302,
125.947699936101));
#206552=CARTESIAN_POINT('Ctrl Pts',(193.149868091433,-0.922682026564098,
125.973435143047));
#206553=CARTESIAN_POINT('Ctrl Pts',(193.14212002343,-1.05745511733767,125.999176113215));
#206554=CARTESIAN_POINT('Ctrl Pts',(193.134371955427,-1.19111419199571,
126.030554308008));
#206555=CARTESIAN_POINT('Ctrl Pts',(193.126623887424,-1.32316033142207,
126.06743864229));
#206556=CARTESIAN_POINT('Ctrl Pts',(193.118867584682,-1.45534681105682,
126.104362177682));
#206557=CARTESIAN_POINT('Ctrl Pts',(193.11111128194,-1.58591655391597,126.146803437196));
#206558=CARTESIAN_POINT('Ctrl Pts',(193.103354979199,-1.71438600696752,
126.194581481684));
#206559=CARTESIAN_POINT('Ctrl Pts',(193.095594536684,-1.84292402803436,
126.242385026753));
#206560=CARTESIAN_POINT('Ctrl Pts',(193.08783409417,-1.96935916538758,126.295530881055));
#206561=CARTESIAN_POINT('Ctrl Pts',(193.080073651656,-2.09322948650229,
126.35379061145));
#206562=CARTESIAN_POINT('Ctrl Pts',(193.072300751391,-2.21729865525309,
126.412143865536));
#206563=CARTESIAN_POINT('Ctrl Pts',(193.064527851125,-2.33879443343359,
126.475627219245));
#206564=CARTESIAN_POINT('Ctrl Pts',(193.05675495086,-2.45728027470416,126.54396665526));
#206565=CARTESIAN_POINT('Ctrl Pts',(193.049264615098,-2.57145885719628,
126.609821780639));
#206566=CARTESIAN_POINT('Ctrl Pts',(193.041774279336,-2.68284228060499,
126.680185891838));
#206567=CARTESIAN_POINT('Ctrl Pts',(193.034283943574,-2.791068240227,126.75477778215));
#206568=CARTESIAN_POINT('Ctrl Pts',(193.026549215124,-2.90282536774334,
126.831803436867));
#206569=CARTESIAN_POINT('Ctrl Pts',(193.018814486674,-3.01157783489076,
126.913587324279));
#206570=CARTESIAN_POINT('Ctrl Pts',(193.011079758224,-3.11689046048007,
126.99986631216));
#206571=CARTESIAN_POINT('Ctrl Pts',(193.003357254067,-3.22203664554232,
127.086008941079));
#206572=CARTESIAN_POINT('Ctrl Pts',(192.995634749909,-3.32375351182408,
127.176632275114));
#206573=CARTESIAN_POINT('Ctrl Pts',(192.987912245751,-3.42163455168092,
127.271429814784));
#206574=CARTESIAN_POINT('Ctrl Pts',(192.980196799127,-3.51942613885007,
127.366140719753));
#206575=CARTESIAN_POINT('Ctrl Pts',(192.972481352503,-3.613388589409,127.465017970231));
#206576=CARTESIAN_POINT('Ctrl Pts',(192.964765905879,-3.70314804461637,
127.567714572328));
#206577=CARTESIAN_POINT('Ctrl Pts',(192.957055793399,-3.79284544381304,
127.670340174201));
#206578=CARTESIAN_POINT('Ctrl Pts',(192.949345680918,-3.87834536897914,
127.776779578253));
#206579=CARTESIAN_POINT('Ctrl Pts',(192.941635568438,-3.95931079161108,
127.886648994062));
#206580=CARTESIAN_POINT('Ctrl Pts',(192.933929070916,-4.04023825284938,
127.99646689657));
#206581=CARTESIAN_POINT('Ctrl Pts',(192.926222573394,-4.11663520834471,
128.109711292731));
#206582=CARTESIAN_POINT('Ctrl Pts',(192.918516075872,-4.18820520986374,
128.225965732648));
#206583=CARTESIAN_POINT('Ctrl Pts',(192.910809982444,-4.25977145856918,
128.342214076698));
#206584=CARTESIAN_POINT('Ctrl Pts',(192.903103889017,-4.32651104118669,
128.461471819057));
#206585=CARTESIAN_POINT('Ctrl Pts',(192.895397795589,-4.3881712193687,128.583294114283));
#206586=CARTESIAN_POINT('Ctrl Pts',(192.887692066741,-4.44982848037876,
128.705110646039));
#206587=CARTESIAN_POINT('Ctrl Pts',(192.879986337892,-4.50640664147058,
128.829491133795));
#206588=CARTESIAN_POINT('Ctrl Pts',(192.872280609043,-4.55769962141508,
128.955967471222));
#206589=CARTESIAN_POINT('Ctrl Pts',(192.864570878078,-4.60901924134692,
129.082509496546));
#206590=CARTESIAN_POINT('Ctrl Pts',(192.856861147112,-4.65504805292081,
129.211149177261));
#206591=CARTESIAN_POINT('Ctrl Pts',(192.849151416146,-4.69562867427047,
129.341399778764));
#206592=CARTESIAN_POINT('Ctrl Pts',(192.844428095933,-4.72049014737659,
129.421197024804));
#206593=CARTESIAN_POINT('Ctrl Pts',(192.839704775721,-4.74330770610149,
129.50159857469));
#206594=CARTESIAN_POINT('Ctrl Pts',(192.834981455508,-4.76405452823404,
129.582490119308));
#206595=CARTESIAN_POINT('',(194.860140564008,-4.91266023721352,130.801203006916));
#206596=CARTESIAN_POINT('Ctrl Pts',(194.860140564008,-4.91221266644762,
130.801203294592));
#206597=CARTESIAN_POINT('Ctrl Pts',(194.80188727277,-4.90617542648731,131.832747380102));
#206598=CARTESIAN_POINT('Ctrl Pts',(194.650818106927,-4.08404315233992,
134.516670434198));
#206599=CARTESIAN_POINT('Ctrl Pts',(194.406933066479,0.327902356760881,
136.612472175972));
#206600=CARTESIAN_POINT('Ctrl Pts',(194.128485442666,5.06376798164403,133.667913246476));
#206601=CARTESIAN_POINT('Ctrl Pts',(193.850037818853,5.14627821021483,128.091889343334));
#206602=CARTESIAN_POINT('Ctrl Pts',(193.57159019504,0.499610173265479,125.008494029623));
#206603=CARTESIAN_POINT('Ctrl Pts',(193.348221787245,-3.59620912304385,
126.807588037525));
#206604=CARTESIAN_POINT('Ctrl Pts',(193.217669254053,-4.59434972149962,
128.935771315469));
#206605=CARTESIAN_POINT('Ctrl Pts',(193.179932595466,-4.75726252818781,
129.584191622251));
#206606=CARTESIAN_POINT('Ctrl Pts',(194.92989654745,-4.76405452823406,129.582490119308));
#206607=CARTESIAN_POINT('Ctrl Pts',(194.921111692065,-4.80245103303602,
129.732197508783));
#206608=CARTESIAN_POINT('Ctrl Pts',(194.912326836681,-4.83383095715299,
129.883888334153));
#206609=CARTESIAN_POINT('Ctrl Pts',(194.903541981296,-4.85800796205853,
130.036935244597));
#206610=CARTESIAN_POINT('Ctrl Pts',(194.894810448159,-4.88203821756628,
130.189053192086));
#206611=CARTESIAN_POINT('Ctrl Pts',(194.886078915021,-4.89895263873311,
130.342510630792));
#206612=CARTESIAN_POINT('Ctrl Pts',(194.877347381884,-4.90861601348531,
130.496672634935));
#206613=CARTESIAN_POINT('Ctrl Pts',(194.871611775925,-4.9149637314563,130.597939216148));
#206614=CARTESIAN_POINT('Ctrl Pts',(194.865876169967,-4.91818362286876,
130.699509432803));
#206615=CARTESIAN_POINT('Ctrl Pts',(194.860140564008,-4.9182489840691,130.801199414751));
#206616=CARTESIAN_POINT('Origin',(213.235140564004,0.,130.804360617566));
#206617=CARTESIAN_POINT('',(196.680227908624,-4.76405452823405,129.582490119308));
#206618=CARTESIAN_POINT('',(196.33459504632,-4.76405452823405,129.582490119308));
#206619=CARTESIAN_POINT('',(213.235140564004,-4.76405452823405,129.582490119308));
#206620=CARTESIAN_POINT('',(196.264859436042,-4.91824930178245,130.801739927489));
#206621=CARTESIAN_POINT('Ctrl Pts',(196.33459504632,-4.76405452823405,129.582490119308));
#206622=CARTESIAN_POINT('Ctrl Pts',(196.325979820702,-4.80173843363128,
129.729419094519));
#206623=CARTESIAN_POINT('Ctrl Pts',(196.317364595083,-4.83266542359164,
129.878265641535));
#206624=CARTESIAN_POINT('Ctrl Pts',(196.308749369464,-4.85665623691895,
130.028426819555));
#206625=CARTESIAN_POINT('Ctrl Pts',(196.300175614881,-4.88053156587922,
130.177865168033));
#206626=CARTESIAN_POINT('Ctrl Pts',(196.291601860298,-4.89753723731489,
130.328605301003));
#206627=CARTESIAN_POINT('Ctrl Pts',(196.283028105715,-4.90754478717536,
130.48003481784));
#206628=CARTESIAN_POINT('Ctrl Pts',(196.276971882491,-4.91461379705869,
130.586999735934));
#206629=CARTESIAN_POINT('Ctrl Pts',(196.270915659266,-4.91819205678833,
130.694308241907));
#206630=CARTESIAN_POINT('Ctrl Pts',(196.264859436042,-4.91824930178245,
130.801739927489));
#206631=CARTESIAN_POINT('Ctrl Pts',(196.264859435991,-4.91824930178293,
130.801739928394));
#206632=CARTESIAN_POINT('Ctrl Pts',(196.257012721372,-4.9183234709409,130.940933241881));
#206633=CARTESIAN_POINT('Ctrl Pts',(196.249166006753,-4.91248424618416,
131.080125087051));
#206634=CARTESIAN_POINT('Ctrl Pts',(196.241319292134,-4.90075854751751,
131.218786390696));
#206635=CARTESIAN_POINT('Ctrl Pts',(196.233470637992,-4.88902995053467,
131.357481968145));
#206636=CARTESIAN_POINT('Ctrl Pts',(196.22562198385,-4.87141201293207,131.495646367384));
#206637=CARTESIAN_POINT('Ctrl Pts',(196.217773329708,-4.84798352666506,
131.632755926392));
#206638=CARTESIAN_POINT('Ctrl Pts',(196.209921209237,-4.82454469329633,
131.769926039314));
#206639=CARTESIAN_POINT('Ctrl Pts',(196.202069088767,-4.79529026322915,
131.906040012911));
#206640=CARTESIAN_POINT('Ctrl Pts',(196.194216968297,-4.76035005680923,
132.040584868718));
#206641=CARTESIAN_POINT('Ctrl Pts',(196.186132871399,-4.72437760638351,
132.179104604331));
#206642=CARTESIAN_POINT('Ctrl Pts',(196.1780487745,-4.68237835041523,132.315960659695));
#206643=CARTESIAN_POINT('Ctrl Pts',(196.169964677602,-4.63454850944733,
132.450611866944));
#206644=CARTESIAN_POINT('Ctrl Pts',(196.162096228248,-4.58799455469389,
132.581671182278));
#206645=CARTESIAN_POINT('Ctrl Pts',(196.154227778895,-4.53591733384053,
132.710641463661));
#206646=CARTESIAN_POINT('Ctrl Pts',(196.146359329542,-4.47854577483177,
132.837046231535));
#206647=CARTESIAN_POINT('Ctrl Pts',(196.138167408871,-4.41881567566367,
132.968647489212));
#206648=CARTESIAN_POINT('Ctrl Pts',(196.1299754882,-4.35334689846171,133.097467395895));
#206649=CARTESIAN_POINT('Ctrl Pts',(196.121783567529,-4.2824489092148,133.222999574183));
#206650=CARTESIAN_POINT('Ctrl Pts',(196.113591646858,-4.21155091996789,
133.348531752471));
#206651=CARTESIAN_POINT('Ctrl Pts',(196.105399726187,-4.13522401973526,
133.470775856601));
#206652=CARTESIAN_POINT('Ctrl Pts',(196.097207805515,-4.05382567680301,
133.589262850068));
#206653=CARTESIAN_POINT('Ctrl Pts',(196.089433471396,-3.97657664814305,
133.701709919927));
#206654=CARTESIAN_POINT('Ctrl Pts',(196.081659137277,-3.89452304616624,
133.811118503023));
#206655=CARTESIAN_POINT('Ctrl Pts',(196.073884803158,-3.80793171009603,
133.917050636464));
#206656=CARTESIAN_POINT('Ctrl Pts',(196.066120050211,-3.72144709010858,
134.022852218017));
#206657=CARTESIAN_POINT('Ctrl Pts',(196.058355297264,-3.63043610820173,
134.125185574825));
#206658=CARTESIAN_POINT('Ctrl Pts',(196.050590544317,-3.53520915752512,
134.223641137654));
#206659=CARTESIAN_POINT('Ctrl Pts',(196.042833503432,-3.44007678759841,
134.32199891303));
#206660=CARTESIAN_POINT('Ctrl Pts',(196.035076462547,-3.34073705198568,
134.41648627984));
#206661=CARTESIAN_POINT('Ctrl Pts',(196.027319421662,-3.2375407000163,134.506726520369));
#206662=CARTESIAN_POINT('Ctrl Pts',(196.019568230422,-3.13442216921906,
134.59689871003));
#206663=CARTESIAN_POINT('Ctrl Pts',(196.011817039182,-3.02745310398911,
134.68282989205));
#206664=CARTESIAN_POINT('Ctrl Pts',(196.004065847942,-2.91702095129357,
134.764180289245));
#206665=CARTESIAN_POINT('Ctrl Pts',(195.996317951164,-2.8066357352085,134.845496110351));
#206666=CARTESIAN_POINT('Ctrl Pts',(195.988570054387,-2.69279067328169,
134.92223478758));
#206667=CARTESIAN_POINT('Ctrl Pts',(195.98082215761,-2.57590594841546,134.994097077944));
#206668=CARTESIAN_POINT('Ctrl Pts',(195.973075881526,-2.45904567331386,
135.065944336265));
#206669=CARTESIAN_POINT('Ctrl Pts',(195.965329605442,-2.3391473328201,135.13291703199));
#206670=CARTESIAN_POINT('Ctrl Pts',(195.957583329358,-2.2166593843348,135.194759715181));
#206671=CARTESIAN_POINT('Ctrl Pts',(195.949836996093,-2.09417053167117,
135.256602854881));
#206672=CARTESIAN_POINT('Ctrl Pts',(195.942090662827,-1.96909238187651,
135.313315730276));
#206673=CARTESIAN_POINT('Ctrl Pts',(195.934344329562,-1.84189687727761,
135.364689438602));
#206674=CARTESIAN_POINT('Ctrl Pts',(195.926596261559,-1.7146728881277,135.416074651714));
#206675=CARTESIAN_POINT('Ctrl Pts',(195.918848193556,-1.58533096307996,
135.462118172125));
#206676=CARTESIAN_POINT('Ctrl Pts',(195.911100125553,-1.45436146849866,
135.502659861063));
#206677=CARTESIAN_POINT('Ctrl Pts',(195.903343822811,-1.32325277797986,
135.543244638191));
#206678=CARTESIAN_POINT('Ctrl Pts',(195.895587520069,-1.19051343654138,
135.578315787215));
#206679=CARTESIAN_POINT('Ctrl Pts',(195.887831217328,-1.0566479063914,135.607763397306));
#206680=CARTESIAN_POINT('Ctrl Pts',(195.880070774813,-0.922710928177224,
135.637226724474));
#206681=CARTESIAN_POINT('Ctrl Pts',(195.872310332299,-0.787646948375374,
135.661060464155));
#206682=CARTESIAN_POINT('Ctrl Pts',(195.864549889785,-0.651967989498143,
135.679206338527));
#206683=CARTESIAN_POINT('Ctrl Pts',(195.85677698952,-0.516071226711214,
135.697381342267));
#206684=CARTESIAN_POINT('Ctrl Pts',(195.849004089254,-0.379557901639337,
135.709850199137));
#206685=CARTESIAN_POINT('Ctrl Pts',(195.841231188989,-0.242943397281255,
135.716606699372));
#206686=CARTESIAN_POINT('Ctrl Pts',(195.833740853227,-0.111295174267542,
135.723117583805));
#206687=CARTESIAN_POINT('Ctrl Pts',(195.826250517465,0.0204466914981448,
135.724324215373));
#206688=CARTESIAN_POINT('Ctrl Pts',(195.818760181703,0.151825322225019,
135.720266651456));
#206689=CARTESIAN_POINT('Ctrl Pts',(195.810985847584,0.288185213667395,
135.716055243769));
#206690=CARTESIAN_POINT('Ctrl Pts',(195.803211513465,0.424585729377166,
135.706159236164));
#206691=CARTESIAN_POINT('Ctrl Pts',(195.795437179345,0.560514165651644,
135.690566398395));
#206692=CARTESIAN_POINT('Ctrl Pts',(195.787672426398,0.69627508227663,135.674992777405));
#206693=CARTESIAN_POINT('Ctrl Pts',(195.779907673451,0.831564692377237,
135.653736339747));
#206694=CARTESIAN_POINT('Ctrl Pts',(195.772142920504,0.96587063867978,135.626836845795));
#206695=CARTESIAN_POINT('Ctrl Pts',(195.764385879619,1.10004319042296,135.5999640688));
#206696=CARTESIAN_POINT('Ctrl Pts',(195.756628838734,1.23323364174855,135.567459465525));
#206697=CARTESIAN_POINT('Ctrl Pts',(195.748871797849,1.36493546079199,135.529414506187));
#206698=CARTESIAN_POINT('Ctrl Pts',(195.741120606609,1.496537962469,135.491398236849));
#206699=CARTESIAN_POINT('Ctrl Pts',(195.733369415369,1.62665369222182,135.447850035617));
#206700=CARTESIAN_POINT('Ctrl Pts',(195.725618224129,1.75478736133172,135.398912214731));
#206701=CARTESIAN_POINT('Ctrl Pts',(195.717870327352,1.88286657021454,135.349995193724));
#206702=CARTESIAN_POINT('Ctrl Pts',(195.710122430575,2.00896502951187,135.295693248354));
#206703=CARTESIAN_POINT('Ctrl Pts',(195.702374533797,2.13260385849881,135.236198142252));
#206704=CARTESIAN_POINT('Ctrl Pts',(195.694628257713,2.25621682490795,135.176715481244));
#206705=CARTESIAN_POINT('Ctrl Pts',(195.686881981629,2.37737083230292,135.112041989627));
#206706=CARTESIAN_POINT('Ctrl Pts',(195.679135705545,2.49560856123834,135.042416890384));
#206707=CARTESIAN_POINT('Ctrl Pts',(195.67138937228,2.61384716297782,134.972791277185));
#206708=CARTESIAN_POINT('Ctrl Pts',(195.663643039014,2.72916910640684,134.898214181805));
#206709=CARTESIAN_POINT('Ctrl Pts',(195.655896705749,2.84114353935931,134.818969745645));
#206710=CARTESIAN_POINT('Ctrl Pts',(195.648148637746,2.95314304820954,134.739707563244));
#206711=CARTESIAN_POINT('Ctrl Pts',(195.640400569743,3.06179323579177,134.655776186005));
#206712=CARTESIAN_POINT('Ctrl Pts',(195.63265250174,3.16669431782458,134.567501614122));
#206713=CARTESIAN_POINT('Ctrl Pts',(195.624896198998,3.27170688997588,134.479133222973));
#206714=CARTESIAN_POINT('Ctrl Pts',(195.617139896256,3.37296209730263,134.386412668355));
#206715=CARTESIAN_POINT('Ctrl Pts',(195.609383593514,3.47009479456587,134.289704959123));
#206716=CARTESIAN_POINT('Ctrl Pts',(195.601623151,3.56727933447434,134.192945634076));
#206717=CARTESIAN_POINT('Ctrl Pts',(195.593862708486,3.660336714878,134.092195201126));
#206718=CARTESIAN_POINT('Ctrl Pts',(195.586102265972,3.74894114432121,133.987852938731));
#206719=CARTESIAN_POINT('Ctrl Pts',(195.578329365706,3.83768780946045,133.883343176873));
#206720=CARTESIAN_POINT('Ctrl Pts',(195.570556465441,3.92196699860579,133.775230371938));
#206721=CARTESIAN_POINT('Ctrl Pts',(195.562783565176,4.00149491020802,133.663944773712));
#206722=CARTESIAN_POINT('Ctrl Pts',(195.555293229414,4.07813178190516,133.556704687292));
#206723=CARTESIAN_POINT('Ctrl Pts',(195.547802893651,4.15035665163739,133.446518738335));
#206724=CARTESIAN_POINT('Ctrl Pts',(195.540312557889,4.21795626720724,133.333792963059));
#206725=CARTESIAN_POINT('Ctrl Pts',(195.53253822377,4.28811894274751,133.216793155752));
#206726=CARTESIAN_POINT('Ctrl Pts',(195.524763889651,4.35352096178859,133.096686504988));
#206727=CARTESIAN_POINT('Ctrl Pts',(195.516989555532,4.41387490580435,132.973897752167));
#206728=CARTESIAN_POINT('Ctrl Pts',(195.509224802585,4.47415446897807,132.851260325509));
#206729=CARTESIAN_POINT('Ctrl Pts',(195.501460049638,4.52939816485493,132.725947721159));
#206730=CARTESIAN_POINT('Ctrl Pts',(195.493695296691,4.57936250334169,132.598412491255));
#206731=CARTESIAN_POINT('Ctrl Pts',(195.485938255806,4.62927721654309,132.47100393114));
#206732=CARTESIAN_POINT('Ctrl Pts',(195.478181214921,4.67392286552881,132.341377500251));
#206733=CARTESIAN_POINT('Ctrl Pts',(195.470424174036,4.71310261393714,132.210008800078));
#206734=CARTESIAN_POINT('Ctrl Pts',(195.462672982796,4.75225281659245,132.078739166064));
#206735=CARTESIAN_POINT('Ctrl Pts',(195.454921791556,4.78594521173213,131.945730251064));
#206736=CARTESIAN_POINT('Ctrl Pts',(195.447170600316,4.81403181502214,131.811475678746));
#206737=CARTESIAN_POINT('Ctrl Pts',(195.439422703538,4.84210648075651,131.677278168202));
#206738=CARTESIAN_POINT('Ctrl Pts',(195.431674806761,4.86458001358226,131.54183643523));
#206739=CARTESIAN_POINT('Ctrl Pts',(195.423926909984,4.88135490294342,131.405657028673));
#206740=CARTESIAN_POINT('Ctrl Pts',(195.4161806339,4.89812628335934,131.269506107912));
#206741=CARTESIAN_POINT('Ctrl Pts',(195.408434357816,4.90920134356196,131.132618208275));
#206742=CARTESIAN_POINT('Ctrl Pts',(195.400688081732,4.91453415629017,130.995507391426));
#206743=CARTESIAN_POINT('Ctrl Pts',(195.392941748467,4.919867008384,130.858395562457));
#206744=CARTESIAN_POINT('Ctrl Pts',(195.385195415201,4.91945751322652,130.721061203664));
#206745=CARTESIAN_POINT('Ctrl Pts',(195.377449081936,4.91331184090468,130.584020388543));
#206746=CARTESIAN_POINT('Ctrl Pts',(195.369701013933,4.90716479230216,130.446948884082));
#206747=CARTESIAN_POINT('Ctrl Pts',(195.36195294593,4.8952790278877,130.310171444601));
#206748=CARTESIAN_POINT('Ctrl Pts',(195.354204877927,4.8777127276868,130.174200631005));
#206749=CARTESIAN_POINT('Ctrl Pts',(195.346448575185,4.86012775781292,130.03808530601));
#206750=CARTESIAN_POINT('Ctrl Pts',(195.338692272444,4.83685024208653,129.902778707793));
#206751=CARTESIAN_POINT('Ctrl Pts',(195.330935969702,4.80798990287418,129.768785339588));
#206752=CARTESIAN_POINT('Ctrl Pts',(195.323175527188,4.77911416002987,129.634720455087));
#206753=CARTESIAN_POINT('Ctrl Pts',(195.315415084674,4.74464975455025,129.501970575457));
#206754=CARTESIAN_POINT('Ctrl Pts',(195.307654642159,4.70475651246827,129.371025618033));
#206755=CARTESIAN_POINT('Ctrl Pts',(195.299881741894,4.66479923021246,129.239870456138));
#206756=CARTESIAN_POINT('Ctrl Pts',(195.292108841629,4.61939582587396,129.11052637553));
#206757=CARTESIAN_POINT('Ctrl Pts',(195.284335941363,4.56875487911233,128.983464707008));
#206758=CARTESIAN_POINT('Ctrl Pts',(195.276845605601,4.5199548583218,128.861022050185));
#206759=CARTESIAN_POINT('Ctrl Pts',(195.269355269839,4.46629160511688,128.740699024911));
#206760=CARTESIAN_POINT('Ctrl Pts',(195.261864934077,4.40799146124495,128.622894518794));
#206761=CARTESIAN_POINT('Ctrl Pts',(195.254090599958,4.3474808496989,128.500623419023));
#206762=CARTESIAN_POINT('Ctrl Pts',(195.246316265839,4.28178311163883,128.380678269616));
#206763=CARTESIAN_POINT('Ctrl Pts',(195.23854193172,4.21110023729952,128.263530467021));
#206764=CARTESIAN_POINT('Ctrl Pts',(195.230777178773,4.14050447328558,128.146527038623));
#206765=CARTESIAN_POINT('Ctrl Pts',(195.223012425825,4.06493599723231,128.032314429117));
#206766=CARTESIAN_POINT('Ctrl Pts',(195.215247672878,3.98464394172745,127.9213421091));
#206767=CARTESIAN_POINT('Ctrl Pts',(195.207490631993,3.90443163342391,127.810480008356));
#206768=CARTESIAN_POINT('Ctrl Pts',(195.199733591108,3.81950530971266,127.702852107236));
#206769=CARTESIAN_POINT('Ctrl Pts',(195.191976550223,3.73015871273531,127.59888108397));
#206770=CARTESIAN_POINT('Ctrl Pts',(195.184225358983,3.64087949272173,127.49498846606));
#206771=CARTESIAN_POINT('Ctrl Pts',(195.176474167743,3.5471868880792,127.39474753233));
#206772=CARTESIAN_POINT('Ctrl Pts',(195.168722976503,3.44941620923195,127.29854960184));
#206773=CARTESIAN_POINT('Ctrl Pts',(195.160975079726,3.35168708553179,127.202392558036));
#206774=CARTESIAN_POINT('Ctrl Pts',(195.153227182949,3.24988361311233,127.110275373367));
#206775=CARTESIAN_POINT('Ctrl Pts',(195.145479286172,3.14437925902386,127.022553888247));
#206776=CARTESIAN_POINT('Ctrl Pts',(195.137733010088,3.03889697417174,126.934850752571));
#206777=CARTESIAN_POINT('Ctrl Pts',(195.129986734003,2.92971564790252,126.851541737333));
#206778=CARTESIAN_POINT('Ctrl Pts',(195.122240457919,2.8172429500486,126.772943345328));
#206779=CARTESIAN_POINT('Ctrl Pts',(195.114494124654,2.70476942194696,126.694344373127));
#206780=CARTESIAN_POINT('Ctrl Pts',(195.106747791389,2.58900479424786,126.620456317494));
#206781=CARTESIAN_POINT('Ctrl Pts',(195.099001458123,2.47038658928282,126.551552937692));
#206782=CARTESIAN_POINT('Ctrl Pts',(195.09125339012,2.35174182059327,126.482634127456));
#206783=CARTESIAN_POINT('Ctrl Pts',(195.083505322117,2.23024254102713,126.418702410666));
#206784=CARTESIAN_POINT('Ctrl Pts',(195.075757254114,2.10635143031566,126.359985890509));
#206785=CARTESIAN_POINT('Ctrl Pts',(195.068000951373,1.98232864665704,126.301206965734));
#206786=CARTESIAN_POINT('Ctrl Pts',(195.060244648631,1.8559093076601,126.247654477585));
#206787=CARTESIAN_POINT('Ctrl Pts',(195.052488345889,1.72757717380225,126.199508809847));
#206788=CARTESIAN_POINT('Ctrl Pts',(195.044727903375,1.59917654522038,126.151337445316));
#206789=CARTESIAN_POINT('Ctrl Pts',(195.036967460861,1.46886145881318,126.108578773192));
#206790=CARTESIAN_POINT('Ctrl Pts',(195.029207018346,1.33713048578585,126.071363139595));
#206791=CARTESIAN_POINT('Ctrl Pts',(195.021434118081,1.2051880465063,126.034087764159));
#206792=CARTESIAN_POINT('Ctrl Pts',(195.013661217816,1.0718255591914,126.002373299147));
#206793=CARTESIAN_POINT('Ctrl Pts',(195.00588831755,0.937552310192054,125.976299026394));
#206794=CARTESIAN_POINT('Ctrl Pts',(194.998397981788,0.808160232008243,
125.951172619133));
#206795=CARTESIAN_POINT('Ctrl Pts',(194.990907646026,0.677922763967373,
125.931283499663));
#206796=CARTESIAN_POINT('Ctrl Pts',(194.983417310264,0.547297844753216,
125.916656848757));
#206797=CARTESIAN_POINT('Ctrl Pts',(194.975642976145,0.411720242024034,
125.901475623937));
#206798=CARTESIAN_POINT('Ctrl Pts',(194.967868642026,0.27529575862716,125.891915708546));
#206799=CARTESIAN_POINT('Ctrl Pts',(194.960094307907,0.138530174400293,
125.888061963774));
#206800=CARTESIAN_POINT('Ctrl Pts',(194.95232955496,0.00193314153252316,
125.884212968398));
#206801=CARTESIAN_POINT('Ctrl Pts',(194.944564802013,-0.135003768683377,
125.886056162276));
#206802=CARTESIAN_POINT('Ctrl Pts',(194.936800049066,-0.271767741656031,
125.893624892942));
#206803=CARTESIAN_POINT('Ctrl Pts',(194.929043008181,-0.408395878722369,
125.901186106239));
#206804=CARTESIAN_POINT('Ctrl Pts',(194.921285967296,-0.544851032521165,
125.914461518103));
#206805=CARTESIAN_POINT('Ctrl Pts',(194.913528926411,-0.680618817085562,
125.933432462858));
#206806=CARTESIAN_POINT('Ctrl Pts',(194.90577773517,-0.816284218107408,
125.952389101476));
#206807=CARTESIAN_POINT('Ctrl Pts',(194.89802654393,-0.951262896003321,
125.977032670072));
#206808=CARTESIAN_POINT('Ctrl Pts',(194.89027535269,-1.08504437948985,126.00729258));
#206809=CARTESIAN_POINT('Ctrl Pts',(194.882527455913,-1.21876900227714,
126.037539628659));
#206810=CARTESIAN_POINT('Ctrl Pts',(194.874779559136,-1.35129706216439,
126.073398184829));
#206811=CARTESIAN_POINT('Ctrl Pts',(194.867031662359,-1.48212731246938,
126.114746380538));
#206812=CARTESIAN_POINT('Ctrl Pts',(194.859285386275,-1.61293019590674,
126.156085927097));
#206813=CARTESIAN_POINT('Ctrl Pts',(194.851539110191,-1.74203560361091,
126.202912711391));
#206814=CARTESIAN_POINT('Ctrl Pts',(194.843792834107,-1.86895689731614,
126.255054826737));
#206815=CARTESIAN_POINT('Ctrl Pts',(194.836046500841,-1.9958791279254,126.307197326983));
#206816=CARTESIAN_POINT('Ctrl Pts',(194.828300167576,-2.12061685072737,
126.364655088006));
#206817=CARTESIAN_POINT('Ctrl Pts',(194.820553834311,-2.24270325279445,
126.427207983444));
#206818=CARTESIAN_POINT('Ctrl Pts',(194.812805766308,-2.3648169952645,126.489774887168));
#206819=CARTESIAN_POINT('Ctrl Pts',(194.805057698305,-2.48427788763078,
126.557439017562));
#206820=CARTESIAN_POINT('Ctrl Pts',(194.797309630302,-2.60064393052617,
126.629934404406));
#206821=CARTESIAN_POINT('Ctrl Pts',(194.78955332756,-2.71713364863695,126.70250684021));
#206822=CARTESIAN_POINT('Ctrl Pts',(194.781797024818,-2.83052161429419,
126.779920582553));
#206823=CARTESIAN_POINT('Ctrl Pts',(194.774040722076,-2.94039458115534,
126.861866131887));
#206824=CARTESIAN_POINT('Ctrl Pts',(194.766280279562,-3.050326190527,126.943855418027));
#206825=CARTESIAN_POINT('Ctrl Pts',(194.758519837048,-3.15673875969899,
127.030381084215));
#206826=CARTESIAN_POINT('Ctrl Pts',(194.750759394534,-3.25925313487488,
127.121094123636));
#206827=CARTESIAN_POINT('Ctrl Pts',(194.742986494268,-3.36193207522668,
127.211952783681));
#206828=CARTESIAN_POINT('Ctrl Pts',(194.735213594003,-3.46070003479519,
127.307011978273));
#206829=CARTESIAN_POINT('Ctrl Pts',(194.727440693737,-3.55521502981467,
127.40588608415));
#206830=CARTESIAN_POINT('Ctrl Pts',(194.719950357975,-3.6462941666962,127.501165867229));
#206831=CARTESIAN_POINT('Ctrl Pts',(194.712460022213,-3.73342397889856,
127.599987782716));
#206832=CARTESIAN_POINT('Ctrl Pts',(194.704969686451,-3.81633575408038,
127.701980164651));
#206833=CARTESIAN_POINT('Ctrl Pts',(194.697219842191,-3.90212007209462,
127.807506151856));
#206834=CARTESIAN_POINT('Ctrl Pts',(194.68946999793,-3.98366789287206,127.916769679002));
#206835=CARTESIAN_POINT('Ctrl Pts',(194.681720153669,-4.06063403806943,
128.029394983297));
#206836=CARTESIAN_POINT('Ctrl Pts',(194.673641243833,-4.14086823717748,
128.146802462472));
#206837=CARTESIAN_POINT('Ctrl Pts',(194.665562333997,-4.21612278806056,
128.26786322798));
#206838=CARTESIAN_POINT('Ctrl Pts',(194.657483424161,-4.28605088173785,
128.39211044363));
#206839=CARTESIAN_POINT('Ctrl Pts',(194.649752999485,-4.35296261511464,
128.510998234348));
#206840=CARTESIAN_POINT('Ctrl Pts',(194.642022574809,-4.41499755592588,
128.632802943297));
#206841=CARTESIAN_POINT('Ctrl Pts',(194.634292150133,-4.47189467077365,
128.757084105708));
#206842=CARTESIAN_POINT('Ctrl Pts',(194.626567138405,-4.52875194548538,
128.881278244753));
#206843=CARTESIAN_POINT('Ctrl Pts',(194.618842126678,-4.58047838715712,
129.007945031798));
#206844=CARTESIAN_POINT('Ctrl Pts',(194.61111711495,-4.62685868724639,129.136619105595));
#206845=CARTESIAN_POINT('Ctrl Pts',(194.603396293483,-4.67321382938121,
129.265223383023));
#206846=CARTESIAN_POINT('Ctrl Pts',(194.595675472015,-4.71422847016418,
129.395832410166));
#206847=CARTESIAN_POINT('Ctrl Pts',(194.587954650547,-4.74973548014277,
129.527961020585));
#206848=CARTESIAN_POINT('Ctrl Pts',(194.58689417891,-4.75461244526093,129.546109172866));
#206849=CARTESIAN_POINT('Ctrl Pts',(194.585833707274,-4.75938558135185,
129.564285966276));
#206850=CARTESIAN_POINT('Ctrl Pts',(194.584773235637,-4.76405452823405,
129.582490119308));
#206851=CARTESIAN_POINT('',(196.610140563971,-4.91824935727201,130.801846220335));
#206852=CARTESIAN_POINT('Ctrl Pts',(196.610140563971,-4.91824935727201,
130.801846220335));
#206853=CARTESIAN_POINT('Ctrl Pts',(196.602459708905,-4.91831834504391,
130.936788726876));
#206854=CARTESIAN_POINT('Ctrl Pts',(196.59477885384,-4.91282949710972,131.071957218089));
#206855=CARTESIAN_POINT('Ctrl Pts',(196.587097998774,-4.90175335462761,
131.206849266967));
#206856=CARTESIAN_POINT('Ctrl Pts',(196.579425945198,-4.89068990429389,
131.341586743087));
#206857=CARTESIAN_POINT('Ctrl Pts',(196.571753891622,-4.87405192579336,
131.476048011019));
#206858=CARTESIAN_POINT('Ctrl Pts',(196.564081838046,-4.85186195546942,
131.60972924594));
#206859=CARTESIAN_POINT('Ctrl Pts',(196.556416637028,-4.82969180487755,
131.743291078887));
#206860=CARTESIAN_POINT('Ctrl Pts',(196.548751436009,-4.80197959258732,
131.8760738716));
#206861=CARTESIAN_POINT('Ctrl Pts',(196.541086234991,-4.76879973819775,
132.007578020808));
#206862=CARTESIAN_POINT('Ctrl Pts',(196.533377076582,-4.73542960832549,
132.139836302786));
#206863=CARTESIAN_POINT('Ctrl Pts',(196.525667918172,-4.69652895673484,
132.270800820309));
#206864=CARTESIAN_POINT('Ctrl Pts',(196.517958759763,-4.65222593936672,
132.399972372218));
#206865=CARTESIAN_POINT('Ctrl Pts',(196.51030050335,-4.60821544575988,132.528291030792));
#206866=CARTESIAN_POINT('Ctrl Pts',(196.502642246937,-4.55887385694772,
132.654839949545));
#206867=CARTESIAN_POINT('Ctrl Pts',(196.494983990524,-4.50437694002413,
132.779144515788));
#206868=CARTESIAN_POINT('Ctrl Pts',(196.487326349773,-4.44988440421434,
132.903439088945));
#206869=CARTESIAN_POINT('Ctrl Pts',(196.479668709022,-4.39023752537237,
133.025489301258));
#206870=CARTESIAN_POINT('Ctrl Pts',(196.472011068271,-4.32565999840557,
133.144841047028));
#206871=CARTESIAN_POINT('Ctrl Pts',(196.464352292712,-4.26107290151344,
133.264210479868));
#206872=CARTESIAN_POINT('Ctrl Pts',(196.456693517154,-4.19155389441899,
133.380880298477));
#206873=CARTESIAN_POINT('Ctrl Pts',(196.449034741596,-4.11737209033022,
133.494421979742));
#206874=CARTESIAN_POINT('Ctrl Pts',(196.44128738256,-4.04233227935724,133.609276914914));
#206875=CARTESIAN_POINT('Ctrl Pts',(196.433540023525,-3.96252135406451,
133.720930539313));
#206876=CARTESIAN_POINT('Ctrl Pts',(196.425792664489,-3.87826158539609,
133.82897135909));
#206877=CARTESIAN_POINT('Ctrl Pts',(196.418122442924,-3.79484075880011,
133.935936458026));
#206878=CARTESIAN_POINT('Ctrl Pts',(196.41045222136,-3.70705958893727,134.03936010492));
#206879=CARTESIAN_POINT('Ctrl Pts',(196.402781999795,-3.61526928634412,
134.138878731135));
#206880=CARTESIAN_POINT('Ctrl Pts',(196.394996072024,-3.52209431609966,
134.239898607683));
#206881=CARTESIAN_POINT('Ctrl Pts',(196.387210144253,-3.4247885873534,134.336894393959));
#206882=CARTESIAN_POINT('Ctrl Pts',(196.379424216482,-3.32375503379505,
134.429527584455));
#206883=CARTESIAN_POINT('Ctrl Pts',(196.371638288711,-3.2227214802367,134.52216077495));
#206884=CARTESIAN_POINT('Ctrl Pts',(196.36385236094,-3.1179604696731,134.610431147627));
#206885=CARTESIAN_POINT('Ctrl Pts',(196.356066433169,-3.00990550869428,
134.694045937901));
#206886=CARTESIAN_POINT('Ctrl Pts',(196.34829209905,-2.90201144717865,134.777536221399));
#206887=CARTESIAN_POINT('Ctrl Pts',(196.340517764931,-2.79047001289452,
134.856666115183));
#206888=CARTESIAN_POINT('Ctrl Pts',(196.332743430812,-2.67566902769502,
134.931100046793));
#206889=CARTESIAN_POINT('Ctrl Pts',(196.324978677865,-2.56100952444973,
135.005442245234));
#206890=CARTESIAN_POINT('Ctrl Pts',(196.317213924918,-2.44309878802772,
135.075099785956));
#206891=CARTESIAN_POINT('Ctrl Pts',(196.309449171971,-2.32235744469594,
135.139777432771));
#206892=CARTESIAN_POINT('Ctrl Pts',(196.301692131086,-2.20173602336822,
135.204390840836));
#206893=CARTESIAN_POINT('Ctrl Pts',(196.293935090201,-2.07828993234506,
135.264034014541));
#206894=CARTESIAN_POINT('Ctrl Pts',(196.286178049316,-1.95246819612849,
135.318455322555));
#206895=CARTESIAN_POINT('Ctrl Pts',(196.278426858075,-1.82674134306254,
135.372835591037));
#206896=CARTESIAN_POINT('Ctrl Pts',(196.270675666835,-1.69864276804628,
135.4220016773));
#206897=CARTESIAN_POINT('Ctrl Pts',(196.262924475595,-1.56864516146753,
135.465748331531));
#206898=CARTESIAN_POINT('Ctrl Pts',(196.255176578818,-1.43870280733915,
135.509476392268));
#206899=CARTESIAN_POINT('Ctrl Pts',(196.247428682041,-1.30686339675709,
135.547789477832));
#206900=CARTESIAN_POINT('Ctrl Pts',(196.239680785264,-1.17361841621132,
135.58053093233));
#206901=CARTESIAN_POINT('Ctrl Pts',(196.23193450918,-1.04040130764291,135.613265538021));
#206902=CARTESIAN_POINT('Ctrl Pts',(196.224188233096,-0.90577959335298,
135.640430737586));
#206903=CARTESIAN_POINT('Ctrl Pts',(196.216441957012,-0.770258312508345,
135.661920210048));
#206904=CARTESIAN_POINT('Ctrl Pts',(196.208695623746,-0.634736031276551,
135.68340984114));
#206905=CARTESIAN_POINT('Ctrl Pts',(196.200949290481,-0.49831455638039,
135.699223600296));
#206906=CARTESIAN_POINT('Ctrl Pts',(196.193202957216,-0.361507077887804,
135.709306661626));
#206907=CARTESIAN_POINT('Ctrl Pts',(196.185454889213,-0.224668962309024,
135.719391980987));
#206908=CARTESIAN_POINT('Ctrl Pts',(196.17770682121,-0.0874450609556074,
135.723744020074));
#206909=CARTESIAN_POINT('Ctrl Pts',(196.169958753207,0.0496487812816021,
135.722360013765));
#206910=CARTESIAN_POINT('Ctrl Pts',(196.162202450465,0.186888328485989,
135.720974536519));
#206911=CARTESIAN_POINT('Ctrl Pts',(196.154446147723,0.323997148879435,
135.71384083974));
#206912=CARTESIAN_POINT('Ctrl Pts',(196.146689844981,0.460461311244389,
135.701008291572));
#206913=CARTESIAN_POINT('Ctrl Pts',(196.138929402467,0.596998308641748,
135.688168894286));
#206914=CARTESIAN_POINT('Ctrl Pts',(196.131168959953,0.732889575229854,
135.669624637705));
#206915=CARTESIAN_POINT('Ctrl Pts',(196.123408517439,0.8676297459151,135.645476365666));
#206916=CARTESIAN_POINT('Ctrl Pts',(196.115635617173,1.00258621348393,135.621289328677));
#206917=CARTESIAN_POINT('Ctrl Pts',(196.107862716908,1.13638751074486,135.591480384296));
#206918=CARTESIAN_POINT('Ctrl Pts',(196.100089816642,1.268540970819,135.556200983977));
#206919=CARTESIAN_POINT('Ctrl Pts',(196.09259948088,1.39589031974556,135.522204078723));
#206920=CARTESIAN_POINT('Ctrl Pts',(196.085109145118,1.52170926338293,135.483127633423));
#206921=CARTESIAN_POINT('Ctrl Pts',(196.077618809356,1.64557497313272,135.439149293471));
#206922=CARTESIAN_POINT('Ctrl Pts',(196.069844475237,1.77413708891525,135.393503501393));
#206923=CARTESIAN_POINT('Ctrl Pts',(196.062070141118,1.90100217941226,135.342432174158));
#206924=CARTESIAN_POINT('Ctrl Pts',(196.054295806999,2.02567829082461,135.286080212162));
#206925=CARTESIAN_POINT('Ctrl Pts',(196.046531054052,2.15020075007207,135.229797698922));
#206926=CARTESIAN_POINT('Ctrl Pts',(196.038766301105,2.27253924505167,135.168247659205));
#206927=CARTESIAN_POINT('Ctrl Pts',(196.031001548158,2.3922180264252,135.101624395431));
#206928=CARTESIAN_POINT('Ctrl Pts',(196.023244507273,2.51177794114601,135.03506730282));
#206929=CARTESIAN_POINT('Ctrl Pts',(196.015487466388,2.62868305990259,134.963447202521));
#206930=CARTESIAN_POINT('Ctrl Pts',(196.007730425503,2.7424789694179,134.887005858681));
#206931=CARTESIAN_POINT('Ctrl Pts',(195.999979234263,2.85618906455235,134.810622159854));
#206932=CARTESIAN_POINT('Ctrl Pts',(195.992228043023,2.96679429415914,134.729424671326));
#206933=CARTESIAN_POINT('Ctrl Pts',(195.984476851783,3.0738664750577,134.643700138371));
#206934=CARTESIAN_POINT('Ctrl Pts',(195.976728955005,3.18089314742335,134.55801204063));
#206935=CARTESIAN_POINT('Ctrl Pts',(195.968981058228,3.28438945316746,134.467800969217));
#206936=CARTESIAN_POINT('Ctrl Pts',(195.961233161451,3.38395793279755,134.373395749301));
#206937=CARTESIAN_POINT('Ctrl Pts',(195.953486885367,3.4835055848481,134.279010276921));
#206938=CARTESIAN_POINT('Ctrl Pts',(195.945740609283,3.57912676149234,134.180432669916));
#206939=CARTESIAN_POINT('Ctrl Pts',(195.937994333199,3.67045902587537,134.078030362954));
#206940=CARTESIAN_POINT('Ctrl Pts',(195.930247999934,3.76179196445257,133.975627300082));
#206941=CARTESIAN_POINT('Ctrl Pts',(195.922501666668,3.84883566736076,133.869399772691));
#206942=CARTESIAN_POINT('Ctrl Pts',(195.914755333403,3.93126661625871,133.759749907387));
#206943=CARTESIAN_POINT('Ctrl Pts',(195.9070072654,4.01371602499605,133.650075486756));
#206944=CARTESIAN_POINT('Ctrl Pts',(195.899259197397,4.09155038929708,133.536977515595));
#206945=CARTESIAN_POINT('Ctrl Pts',(195.891511129394,4.16448855602539,133.420888494206));
#206946=CARTESIAN_POINT('Ctrl Pts',(195.883754826652,4.23750424230527,133.304676092023));
#206947=CARTESIAN_POINT('Ctrl Pts',(195.875998523911,4.3056131276605,133.185466620943));
#206948=CARTESIAN_POINT('Ctrl Pts',(195.868242221169,4.36857895453045,133.063719150542));
#206949=CARTESIAN_POINT('Ctrl Pts',(195.860481778655,4.43157838815802,132.941906699851));
#206950=CARTESIAN_POINT('Ctrl Pts',(195.85272133614,4.48942912881509,132.817553904979));
#206951=CARTESIAN_POINT('Ctrl Pts',(195.844960893626,4.5419428571012,132.691140452451));
#206952=CARTESIAN_POINT('Ctrl Pts',(195.837187993361,4.59454088508596,132.564524069826));
#206953=CARTESIAN_POINT('Ctrl Pts',(195.829415093095,4.64178464539287,132.435840786428));
#206954=CARTESIAN_POINT('Ctrl Pts',(195.82164219283,4.68353525993757,132.305586960068));
#206955=CARTESIAN_POINT('Ctrl Pts',(195.814151857068,4.72376813448038,132.180068188384));
#206956=CARTESIAN_POINT('Ctrl Pts',(195.806661521306,4.75890022668183,132.053091374545));
#206957=CARTESIAN_POINT('Ctrl Pts',(195.799171185544,4.78885244545705,131.925108277898));
#206958=CARTESIAN_POINT('Ctrl Pts',(195.791396851425,4.81994031171073,131.792272663244));
#206959=CARTESIAN_POINT('Ctrl Pts',(195.783622517306,4.84554623795796,131.657932169745));
#206960=CARTESIAN_POINT('Ctrl Pts',(195.775848183187,4.86552621996172,131.522579014271));
#206961=CARTESIAN_POINT('Ctrl Pts',(195.76808343024,4.88548157842337,131.387392669463));
#206962=CARTESIAN_POINT('Ctrl Pts',(195.760318677292,4.89982473164211,131.25119652892));
#206963=CARTESIAN_POINT('Ctrl Pts',(195.752553924345,4.90846199760866,131.114495879237));
#206964=CARTESIAN_POINT('Ctrl Pts',(195.74479688346,4.91709068492086,130.977931002566));
#206965=CARTESIAN_POINT('Ctrl Pts',(195.737039842575,4.92002473840631,130.840863001602));
#206966=CARTESIAN_POINT('Ctrl Pts',(195.72928280169,4.91722193961525,130.70380486653));
#206967=CARTESIAN_POINT('Ctrl Pts',(195.72153161045,4.91442125443657,130.566850088065));
#206968=CARTESIAN_POINT('Ctrl Pts',(195.71378041921,4.90589233599108,130.429905549986));
#206969=CARTESIAN_POINT('Ctrl Pts',(195.70602922797,4.89164498773053,130.293486487754));
#206970=CARTESIAN_POINT('Ctrl Pts',(195.698281331193,4.87740369497295,130.157125407263));
#206971=CARTESIAN_POINT('Ctrl Pts',(195.690533434416,4.85744884697578,130.021289746446));
#206972=CARTESIAN_POINT('Ctrl Pts',(195.682785537639,4.83184225710067,129.886491637266));
#206973=CARTESIAN_POINT('Ctrl Pts',(195.675039261555,4.80624102357217,129.751721724946));
#206974=CARTESIAN_POINT('Ctrl Pts',(195.667292985471,4.77499047258891,129.617989316424));
#206975=CARTESIAN_POINT('Ctrl Pts',(195.659546709387,4.73820383137157,129.485797947506));
#206976=CARTESIAN_POINT('Ctrl Pts',(195.651800376121,4.70141691860354,129.353605602781));
#206977=CARTESIAN_POINT('Ctrl Pts',(195.644054042856,4.65909393887212,129.222954697012));
#206978=CARTESIAN_POINT('Ctrl Pts',(195.63630770959,4.61139834311363,129.094334774595));
#206979=CARTESIAN_POINT('Ctrl Pts',(195.628559641587,4.5636920662572,128.965686048638));
#206980=CARTESIAN_POINT('Ctrl Pts',(195.620811573584,4.51061091513302,128.839069577583));
#206981=CARTESIAN_POINT('Ctrl Pts',(195.613063505581,4.45236679435636,128.714955680505));
#206982=CARTESIAN_POINT('Ctrl Pts',(195.60530720284,4.3940607710351,128.590709873701));
#206983=CARTESIAN_POINT('Ctrl Pts',(195.597550900098,4.33058098301466,128.468972308536));
#206984=CARTESIAN_POINT('Ctrl Pts',(195.589794597356,4.26218595554776,128.350189893506));
#206985=CARTESIAN_POINT('Ctrl Pts',(195.582034154842,4.19375442359537,128.231344080725));
#206986=CARTESIAN_POINT('Ctrl Pts',(195.574273712328,4.12040263382347,128.115456891078));
#206987=CARTESIAN_POINT('Ctrl Pts',(195.566513269813,4.04243236885387,128.002946045293));
#206988=CARTESIAN_POINT('Ctrl Pts',(195.558740369548,3.96433693909305,127.89025458711));
#206989=CARTESIAN_POINT('Ctrl Pts',(195.550967469282,3.88160845470985,127.780950615611));
#206990=CARTESIAN_POINT('Ctrl Pts',(195.543194569017,3.79458944858941,127.675419266381));
#206991=CARTESIAN_POINT('Ctrl Pts',(195.535704233255,3.71073380252928,127.573724247514));
#206992=CARTESIAN_POINT('Ctrl Pts',(195.528213897493,3.62289436686037,127.475532553891));
#206993=CARTESIAN_POINT('Ctrl Pts',(195.520723561731,3.53140846885445,127.381154914047));
#206994=CARTESIAN_POINT('Ctrl Pts',(195.512949227612,3.43645385521897,127.283198917303));
#206995=CARTESIAN_POINT('Ctrl Pts',(195.505174893493,3.33727002191439,127.189041608169));
#206996=CARTESIAN_POINT('Ctrl Pts',(195.497400559374,3.23419324712464,127.099070196728));
#206997=CARTESIAN_POINT('Ctrl Pts',(195.489635806427,3.1312435052475,127.009209667011));
#206998=CARTESIAN_POINT('Ctrl Pts',(195.48187105348,3.02441065959921,126.92352502525));
#206999=CARTESIAN_POINT('Ctrl Pts',(195.474106300532,2.91406918468932,126.842368208519));
#207000=CARTESIAN_POINT('Ctrl Pts',(195.466349259647,2.80383730248746,126.761291997883));
#207001=CARTESIAN_POINT('Ctrl Pts',(195.458592218762,2.69010403888476,126.684734892995));
#207002=CARTESIAN_POINT('Ctrl Pts',(195.450835177877,2.57327816695157,126.61300969716));
#207003=CARTESIAN_POINT('Ctrl Pts',(195.443083986637,2.45654039431791,126.541338589853));
#207004=CARTESIAN_POINT('Ctrl Pts',(195.435332795397,2.33671498721072,126.474492342605));
#207005=CARTESIAN_POINT('Ctrl Pts',(195.427581604157,2.2142407268208,126.412741204845));
#207006=CARTESIAN_POINT('Ctrl Pts',(195.41983370738,2.09181852125829,126.351016312966));
#207007=CARTESIAN_POINT('Ctrl Pts',(195.412085810603,1.96675004998067,126.294382399095));
#207008=CARTESIAN_POINT('Ctrl Pts',(195.404337913826,1.83949959574408,126.243064277735));
#207009=CARTESIAN_POINT('Ctrl Pts',(195.396591637742,1.71227575955951,126.19175689102));
#207010=CARTESIAN_POINT('Ctrl Pts',(195.388845361658,1.5828712106282,126.145763231222));
#207011=CARTESIAN_POINT('Ctrl Pts',(195.381099085574,1.45177078996202,126.105260210476));
#207012=CARTESIAN_POINT('Ctrl Pts',(195.373352752308,1.32066940154283,126.064756890746));
#207013=CARTESIAN_POINT('Ctrl Pts',(195.365606419043,1.18787248995334,126.02974440635));
#207014=CARTESIAN_POINT('Ctrl Pts',(195.357860085778,1.05388027198198,126.000349852088));
#207015=CARTESIAN_POINT('Ctrl Pts',(195.350112017775,0.919858047382009,
125.97094871512));
#207016=CARTESIAN_POINT('Ctrl Pts',(195.342363949772,0.784640365557708,
125.947168095513));
#207017=CARTESIAN_POINT('Ctrl Pts',(195.334615881769,0.648737458886747,
125.92908393086));
#207018=CARTESIAN_POINT('Ctrl Pts',(195.326859579027,0.512690112989033,
125.910980546142));
#207019=CARTESIAN_POINT('Ctrl Pts',(195.319103276285,0.375956475623729,
125.898585762068));
#207020=CARTESIAN_POINT('Ctrl Pts',(195.311346973543,0.239052282779265,
125.891923638978));
#207021=CARTESIAN_POINT('Ctrl Pts',(195.303586531029,0.102075020045067,
125.885257960113));
#207022=CARTESIAN_POINT('Ctrl Pts',(195.295826088515,-0.0350725887894774,
125.884331041572));
#207023=CARTESIAN_POINT('Ctrl Pts',(195.288065646001,-0.17187598256682,
125.889114773347));
#207024=CARTESIAN_POINT('Ctrl Pts',(195.280292745735,-0.308898985296921,
125.893906184392));
#207025=CARTESIAN_POINT('Ctrl Pts',(195.27251984547,-0.445576278733256,
125.904426534803));
#207026=CARTESIAN_POINT('Ctrl Pts',(195.264746945204,-0.58139869000898,
125.920595817153));
#207027=CARTESIAN_POINT('Ctrl Pts',(195.257256609442,-0.712283614519818,
125.936177305362));
#207028=CARTESIAN_POINT('Ctrl Pts',(195.24976627368,-0.842374427875423,
125.957004101464));
#207029=CARTESIAN_POINT('Ctrl Pts',(195.242275937918,-0.971227371730748,
125.982960358834));
#207030=CARTESIAN_POINT('Ctrl Pts',(195.234501603799,-1.10496581411534,
126.009900755591));
#207031=CARTESIAN_POINT('Ctrl Pts',(195.22672726968,-1.23779430956464,126.042452598076));
#207032=CARTESIAN_POINT('Ctrl Pts',(195.218952935561,-1.36920532069673,
126.080542262435));
#207033=CARTESIAN_POINT('Ctrl Pts',(195.211188182614,-1.50045437950196,
126.118584984687));
#207034=CARTESIAN_POINT('Ctrl Pts',(195.203423429667,-1.63028905794107,
126.162151841558));
#207035=CARTESIAN_POINT('Ctrl Pts',(195.19565867672,-1.7582108487659,126.211118007625));
#207036=CARTESIAN_POINT('Ctrl Pts',(195.187901635835,-1.88600558586439,
126.260035539804));
#207037=CARTESIAN_POINT('Ctrl Pts',(195.18014459495,-2.01189085348242,126.314341570363));
#207038=CARTESIAN_POINT('Ctrl Pts',(195.172387554065,-2.13538252951149,
126.373861264766));
#207039=CARTESIAN_POINT('Ctrl Pts',(195.164636362824,-2.25878107950726,
126.433336074905));
#207040=CARTESIAN_POINT('Ctrl Pts',(195.156885171584,-2.37978927994142,
126.498016554088));
#207041=CARTESIAN_POINT('Ctrl Pts',(195.149133980344,-2.49794259036277,
126.567679619691));
#207042=CARTESIAN_POINT('Ctrl Pts',(195.141386083567,-2.61604568247549,
126.637313076633));
#207043=CARTESIAN_POINT('Ctrl Pts',(195.13363818679,-2.73129596186393,126.711924709835));
#207044=CARTESIAN_POINT('Ctrl Pts',(195.125890290013,-2.84325332954889,
126.791245422794));
#207045=CARTESIAN_POINT('Ctrl Pts',(195.118144013929,-2.95518727816587,
126.87054954357));
#207046=CARTESIAN_POINT('Ctrl Pts',(195.110397737845,-3.06382936634111,
126.954560558935));
#207047=CARTESIAN_POINT('Ctrl Pts',(195.102651461761,-3.16876868447561,
127.042966183744));
#207048=CARTESIAN_POINT('Ctrl Pts',(195.094905128495,-3.27370877724855,
127.131372461143));
#207049=CARTESIAN_POINT('Ctrl Pts',(195.08715879523,-3.37494574643612,127.224173160824));
#207050=CARTESIAN_POINT('Ctrl Pts',(195.079412461965,-3.47210228418942,
127.321016134081));
#207051=CARTESIAN_POINT('Ctrl Pts',(195.071664393962,-3.56928057947593,
127.41788079465));
#207052=CARTESIAN_POINT('Ctrl Pts',(195.063916325959,-3.6623763481555,127.518789254161));
#207053=CARTESIAN_POINT('Ctrl Pts',(195.056168257956,-3.75104990871693,
127.62335328579));
#207054=CARTESIAN_POINT('Ctrl Pts',(195.048411955214,-3.83981771259343,
127.728028449315));
#207055=CARTESIAN_POINT('Ctrl Pts',(195.040655652472,-3.92415366637445,
127.836366647376));
#207056=CARTESIAN_POINT('Ctrl Pts',(195.03289934973,-4.00375875951405,127.947946981883));
#207057=CARTESIAN_POINT('Ctrl Pts',(195.025138907216,-4.08340634028877,
128.059586870174));
#207058=CARTESIAN_POINT('Ctrl Pts',(195.017378464702,-4.15831781570031,
128.174472015597));
#207059=CARTESIAN_POINT('Ctrl Pts',(195.009618022188,-4.22823870262148,
128.292154309128));
#207060=CARTESIAN_POINT('Ctrl Pts',(195.001845121922,-4.29827183275764,
128.410025516725));
#207061=CARTESIAN_POINT('Ctrl Pts',(194.994072221657,-4.36329817963602,
128.530702500966));
#207062=CARTESIAN_POINT('Ctrl Pts',(194.986299321391,-4.42310983539823,
128.65371363433));
#207063=CARTESIAN_POINT('Ctrl Pts',(194.978808985629,-4.48074718681689,
128.772253003149));
#207064=CARTESIAN_POINT('Ctrl Pts',(194.971318649867,-4.53354227567348,
128.892959480803));
#207065=CARTESIAN_POINT('Ctrl Pts',(194.963828314105,-4.58135270478999,
129.015397102898));
#207066=CARTESIAN_POINT('Ctrl Pts',(194.954994481147,-4.63773860762726,
129.159795636662));
#207067=CARTESIAN_POINT('Ctrl Pts',(194.946160648188,-4.68734145347547,
129.306984074171));
#207068=CARTESIAN_POINT('Ctrl Pts',(194.937326815229,-4.72991114124837,
129.456353325896));
#207069=CARTESIAN_POINT('Ctrl Pts',(194.934850059303,-4.74184647294076,
129.498232222765));
#207070=CARTESIAN_POINT('Ctrl Pts',(194.932373303377,-4.75322921960265,
129.540282405251));
#207071=CARTESIAN_POINT('Ctrl Pts',(194.92989654745,-4.76405452823406,129.582490119308));
#207072=CARTESIAN_POINT('Ctrl Pts',(196.680227908624,-4.76405452823405,
129.582490119308));
#207073=CARTESIAN_POINT('Ctrl Pts',(196.672454999871,-4.79811658810201,
129.71529757377));
#207074=CARTESIAN_POINT('Ctrl Pts',(196.664682091119,-4.82658494688575,
129.849389568182));
#207075=CARTESIAN_POINT('Ctrl Pts',(196.656909182367,-4.84939273648973,
129.984255045228));
#207076=CARTESIAN_POINT('Ctrl Pts',(196.649444140572,-4.87129716224193,
130.113778812316));
#207077=CARTESIAN_POINT('Ctrl Pts',(196.641979098777,-4.88798086211456,
130.244015655847));
#207078=CARTESIAN_POINT('Ctrl Pts',(196.634514056982,-4.89942987008945,
130.374511794635));
#207079=CARTESIAN_POINT('Ctrl Pts',(196.626389559324,-4.91189027433556,
130.516535858678));
#207080=CARTESIAN_POINT('Ctrl Pts',(196.618265061666,-4.91817638477932,
130.659109497139));
#207081=CARTESIAN_POINT('Ctrl Pts',(196.610140564008,-4.91824935727168,
130.801846219679));
#207082=CARTESIAN_POINT('Origin',(213.235140564004,0.,130.804360617566));
#207083=CARTESIAN_POINT('',(198.430216174721,-4.76405452823404,129.582490119308));
#207084=CARTESIAN_POINT('',(198.084936573762,-4.76405452823404,129.582490119308));
#207085=CARTESIAN_POINT('',(213.235140564004,-4.76405452823405,129.582490119308));
#207086=CARTESIAN_POINT('',(198.014859435953,-4.91824901604543,130.801249561772));
#207087=CARTESIAN_POINT('Ctrl Pts',(198.084936573762,-4.76405452823404,
129.582490119308));
#207088=CARTESIAN_POINT('Ctrl Pts',(198.077162780964,-4.79809767465422,
129.715223830524));
#207089=CARTESIAN_POINT('Ctrl Pts',(198.069388988166,-4.82655054116148,
129.849229756449));
#207090=CARTESIAN_POINT('Ctrl Pts',(198.061615195367,-4.84934911569474,
129.983997151406));
#207091=CARTESIAN_POINT('Ctrl Pts',(198.056523854313,-4.8642807354981,130.072261244428));
#207092=CARTESIAN_POINT('Ctrl Pts',(198.051432513259,-4.87678805849738,
130.160851841391));
#207093=CARTESIAN_POINT('Ctrl Pts',(198.046341172205,-4.88686521477497,
130.249625153473));
#207094=CARTESIAN_POINT('Ctrl Pts',(198.035847260134,-4.90763553654045,
130.43259842543));
#207095=CARTESIAN_POINT('Ctrl Pts',(198.025353348062,-4.91813231630581,
130.616759698695));
#207096=CARTESIAN_POINT('Ctrl Pts',(198.014859435991,-4.91824901604501,
130.80124956111));
#207097=CARTESIAN_POINT('Ctrl Pts',(198.014859435953,-4.91824901604543,
130.801249561772));
#207098=CARTESIAN_POINT('Ctrl Pts',(198.007194602125,-4.91833425441149,
130.936002371663));
#207099=CARTESIAN_POINT('Ctrl Pts',(197.999529768297,-4.9128772797748,131.070975950461));
#207100=CARTESIAN_POINT('Ctrl Pts',(197.991864934469,-4.90185011753594,
131.205669087091));
#207101=CARTESIAN_POINT('Ctrl Pts',(197.984208471378,-4.89083499802213,
131.340215125821));
#207102=CARTESIAN_POINT('Ctrl Pts',(197.976552008288,-4.87426182187178,
131.47448093386));
#207103=CARTESIAN_POINT('Ctrl Pts',(197.968895545198,-4.85215462495801,
131.607964100634));
#207104=CARTESIAN_POINT('Ctrl Pts',(197.961245495214,-4.83006594518477,
131.741335460987));
#207105=CARTESIAN_POINT('Ctrl Pts',(197.95359544523,-4.80245253092967,131.873925089211));
#207106=CARTESIAN_POINT('Ctrl Pts',(197.945945395246,-4.76939029060855,
132.005235014974));
#207107=CARTESIAN_POINT('Ctrl Pts',(197.938299305357,-4.73634516515454,
132.136476967365));
#207108=CARTESIAN_POINT('Ctrl Pts',(197.930653215467,-4.69785692034788,
132.266440145392));
#207109=CARTESIAN_POINT('Ctrl Pts',(197.923007125577,-4.65405260327977,
132.394636514511));
#207110=CARTESIAN_POINT('Ctrl Pts',(197.915363000358,-4.61025954177498,
132.522799943444));
#207111=CARTESIAN_POINT('Ctrl Pts',(197.907718875139,-4.56115325357192,
132.649197085549));
#207112=CARTESIAN_POINT('Ctrl Pts',(197.90007474992,-4.50691057686776,132.773355314008));
#207113=CARTESIAN_POINT('Ctrl Pts',(197.892430829445,-4.45266935302643,
132.897510216952));
#207114=CARTESIAN_POINT('Ctrl Pts',(197.88478690897,-4.3932921754651,133.019425956816));
#207115=CARTESIAN_POINT('Ctrl Pts',(197.877142988494,-4.32900370978916,
133.138650647346));
#207116=CARTESIAN_POINT('Ctrl Pts',(197.869497513223,-4.26470216764921,
133.257899588531));
#207117=CARTESIAN_POINT('Ctrl Pts',(197.861852037952,-4.19548754221391,
133.374456038018));
#207118=CARTESIAN_POINT('Ctrl Pts',(197.854206562681,-4.12162977785966,
133.487893929593));
#207119=CARTESIAN_POINT('Ctrl Pts',(197.846553256078,-4.04769636030815,
133.60144801666));
#207120=CARTESIAN_POINT('Ctrl Pts',(197.838899949475,-3.9691105266443,133.711876829538));
#207121=CARTESIAN_POINT('Ctrl Pts',(197.831246642873,-3.8861849641364,133.818784192152));
#207122=CARTESIAN_POINT('Ctrl Pts',(197.823589202619,-3.80321461244542,
133.925749296834));
#207123=CARTESIAN_POINT('Ctrl Pts',(197.815931762365,-3.71590012432521,
134.029188857436));
#207124=CARTESIAN_POINT('Ctrl Pts',(197.808274322111,-3.62459270805556,
134.128741877772));
#207125=CARTESIAN_POINT('Ctrl Pts',(197.800605170645,-3.53314564714557,
134.228447153492));
#207126=CARTESIAN_POINT('Ctrl Pts',(197.792936019179,-3.43769374582733,
134.324253733522));
#207127=CARTESIAN_POINT('Ctrl Pts',(197.785266867713,-3.33862350365245,
134.415839007832));
#207128=CARTESIAN_POINT('Ctrl Pts',(197.779475761273,-3.26381388226844,
134.484996602939));
#207129=CARTESIAN_POINT('Ctrl Pts',(197.773684654833,-3.18694180385115,
134.55174800559));
#207130=CARTESIAN_POINT('Ctrl Pts',(197.767893548393,-3.10818467377065,
134.615970657462));
#207131=CARTESIAN_POINT('Ctrl Pts',(197.760119214274,-3.00245630392844,
134.702187058218));
#207132=CARTESIAN_POINT('Ctrl Pts',(197.752344880155,-2.89297047802538,
134.784137565104));
#207133=CARTESIAN_POINT('Ctrl Pts',(197.744570546035,-2.78010632827789,
134.861476818264));
#207134=CARTESIAN_POINT('Ctrl Pts',(197.736805793088,-2.66738127350782,
134.938720757708));
#207135=CARTESIAN_POINT('Ctrl Pts',(197.729041040141,-2.55128649839717,
135.011364531943));
#207136=CARTESIAN_POINT('Ctrl Pts',(197.721276287194,-2.43223495821874,
135.07910226713));
#207137=CARTESIAN_POINT('Ctrl Pts',(197.713519246309,-2.31330166170844,
135.146772724244));
#207138=CARTESIAN_POINT('Ctrl Pts',(197.705762205424,-2.19141778190944,
135.209546647202));
#207139=CARTESIAN_POINT('Ctrl Pts',(197.698005164539,-2.06702577581684,
135.267161028139));
#207140=CARTESIAN_POINT('Ctrl Pts',(197.690253973299,-1.94272757470384,
135.324731961623));
#207141=CARTESIAN_POINT('Ctrl Pts',(197.682502782059,-1.8159253653342,135.377150933938));
#207142=CARTESIAN_POINT('Ctrl Pts',(197.674751590819,-1.68708644647367,
135.424200699714));
#207143=CARTESIAN_POINT('Ctrl Pts',(197.667003694042,-1.55830228759047,
135.471230468085));
#207144=CARTESIAN_POINT('Ctrl Pts',(197.659255797265,-1.42748350741483,
135.512895434921));
#207145=CARTESIAN_POINT('Ctrl Pts',(197.651507900488,-1.29511743474276,
135.549026453294));
#207146=CARTESIAN_POINT('Ctrl Pts',(197.643761624403,-1.16277905019961,
135.585149913837));
#207147=CARTESIAN_POINT('Ctrl Pts',(197.636015348319,-1.02889439386554,
135.615741625526));
#207148=CARTESIAN_POINT('Ctrl Pts',(197.628269072235,-0.89396562727687,
135.640682414112));
#207149=CARTESIAN_POINT('Ctrl Pts',(197.62052273897,-0.759035864674597,
135.665623386805));
#207150=CARTESIAN_POINT('Ctrl Pts',(197.612776405705,-0.623062360890706,
135.684913282095));
#207151=CARTESIAN_POINT('Ctrl Pts',(197.605030072439,-0.486556739791109,
135.698484196049));
#207152=CARTESIAN_POINT('Ctrl Pts',(197.597282004436,-0.350020549204351,
135.712058149115));
#207153=CARTESIAN_POINT('Ctrl Pts',(197.589533936433,-0.212952393152231,
135.71991053368));
#207154=CARTESIAN_POINT('Ctrl Pts',(197.58178586843,-0.0758678779773515,
135.72202542188));
#207155=CARTESIAN_POINT('Ctrl Pts',(197.574029565689,0.061362332251699,
135.724142557809));
#207156=CARTESIAN_POINT('Ctrl Pts',(197.566273262947,0.198608544793241,
135.720510010164));
#207157=CARTESIAN_POINT('Ctrl Pts',(197.558516960205,0.335355735986595,
135.711164016199));
#207158=CARTESIAN_POINT('Ctrl Pts',(197.550756517691,0.472175913273558,
135.701813033997));
#207159=CARTESIAN_POINT('Ctrl Pts',(197.542996075176,0.608496150094301,
135.686742572151));
#207160=CARTESIAN_POINT('Ctrl Pts',(197.535235632662,0.743808672534506,
135.666040545447));
#207161=CARTESIAN_POINT('Ctrl Pts',(197.527462732397,0.879338410648007,
135.645305286012));
#207162=CARTESIAN_POINT('Ctrl Pts',(197.519689832131,1.01385681788001,135.618920471637));
#207163=CARTESIAN_POINT('Ctrl Pts',(197.511916931866,1.14686752295984,135.587024932284));
#207164=CARTESIAN_POINT('Ctrl Pts',(197.504426596104,1.27504295387604,135.556288876127));
#207165=CARTESIAN_POINT('Ctrl Pts',(197.496936260342,1.40181810066686,135.52043588028));
#207166=CARTESIAN_POINT('Ctrl Pts',(197.48944592458,1.52676573916633,135.479632742289));
#207167=CARTESIAN_POINT('Ctrl Pts',(197.481671590461,1.65645080535675,135.437282540919));
#207168=CARTESIAN_POINT('Ctrl Pts',(197.473897256342,1.78457785099881,135.38946526551));
#207169=CARTESIAN_POINT('Ctrl Pts',(197.466122922223,1.91065138484321,135.336313215299));
#207170=CARTESIAN_POINT('Ctrl Pts',(197.458358169276,2.03656954432468,135.283226670239));
#207171=CARTESIAN_POINT('Ctrl Pts',(197.450593416329,2.16043887068706,135.22481858236));
#207172=CARTESIAN_POINT('Ctrl Pts',(197.442828663381,2.28177881119425,135.161271050348));
#207173=CARTESIAN_POINT('Ctrl Pts',(197.435071622496,2.40299823516199,135.097786634641));
#207174=CARTESIAN_POINT('Ctrl Pts',(197.427314581611,2.52169292860744,135.029173113332));
#207175=CARTESIAN_POINT('Ctrl Pts',(197.419557540726,2.63740245675027,134.955660575847));
#207176=CARTESIAN_POINT('Ctrl Pts',(197.411806349486,2.7530247274378,134.882203474739));
#207177=CARTESIAN_POINT('Ctrl Pts',(197.404055158246,2.86566598491015,134.803854919712));
#207178=CARTESIAN_POINT('Ctrl Pts',(197.396303967006,2.97489086808598,134.720890636023));
#207179=CARTESIAN_POINT('Ctrl Pts',(197.388556070229,3.08406932777271,134.637961614368));
#207180=CARTESIAN_POINT('Ctrl Pts',(197.380808173452,3.18983399049617,134.550421001924));
#207181=CARTESIAN_POINT('Ctrl Pts',(197.373060276675,3.2917791350376,134.458587374163));
#207182=CARTESIAN_POINT('Ctrl Pts',(197.365314000591,3.39370295485246,134.366772956017));
#207183=CARTESIAN_POINT('Ctrl Pts',(197.357567724507,3.49180855536177,134.270667570245));
#207184=CARTESIAN_POINT('Ctrl Pts',(197.349821448422,3.58572424131846,134.170629282976));
#207185=CARTESIAN_POINT('Ctrl Pts',(197.342075115157,3.67964062053938,134.070590257247));
#207186=CARTESIAN_POINT('Ctrl Pts',(197.334328781892,3.76936675589715,133.96661855713));
#207187=CARTESIAN_POINT('Ctrl Pts',(197.326582448626,3.85456897269458,133.859107922539));
#207188=CARTESIAN_POINT('Ctrl Pts',(197.318834380623,3.93979026993763,133.751573211687));
#207189=CARTESIAN_POINT('Ctrl Pts',(197.31108631262,4.02048538988445,133.640498295691));
#207190=CARTESIAN_POINT('Ctrl Pts',(197.303338244617,4.09636223415192,133.52630835937));
#207191=CARTESIAN_POINT('Ctrl Pts',(197.295581941876,4.17231972123249,133.411997060627));
#207192=CARTESIAN_POINT('Ctrl Pts',(197.287825639134,4.24344848632279,133.294564454268));
#207193=CARTESIAN_POINT('Ctrl Pts',(197.280069336392,4.3095006339843,133.17446343141));
#207194=CARTESIAN_POINT('Ctrl Pts',(197.272308893878,4.37558803566593,133.054298307018));
#207195=CARTESIAN_POINT('Ctrl Pts',(197.264548451364,4.43659324710592,132.931462278247));
#207196=CARTESIAN_POINT('Ctrl Pts',(197.256788008849,4.49231576929894,132.80643006976));
#207197=CARTESIAN_POINT('Ctrl Pts',(197.249015108584,4.54812774223136,132.681197148472));
#207198=CARTESIAN_POINT('Ctrl Pts',(197.241242208318,4.59863993554477,132.553761366054));
#207199=CARTESIAN_POINT('Ctrl Pts',(197.233469308053,4.64370085002127,132.424615374699));
#207200=CARTESIAN_POINT('Ctrl Pts',(197.225978972291,4.68712368675483,132.300164165429));
#207201=CARTESIAN_POINT('Ctrl Pts',(197.218488636529,4.72548460943441,132.174125223962));
#207202=CARTESIAN_POINT('Ctrl Pts',(197.210998300767,4.75869302446231,132.046948144235));
#207203=CARTESIAN_POINT('Ctrl Pts',(197.203223966648,4.79316054663953,131.914949106876));
#207204=CARTESIAN_POINT('Ctrl Pts',(197.195449632529,4.82218631642961,131.781305789271));
#207205=CARTESIAN_POINT('Ctrl Pts',(197.18767529841,4.84561381580234,131.646506573209));
#207206=CARTESIAN_POINT('Ctrl Pts',(197.179910545463,4.86901244287585,131.511873485134));
#207207=CARTESIAN_POINT('Ctrl Pts',(197.172145792516,4.88682646091603,131.376087714508));
#207208=CARTESIAN_POINT('Ctrl Pts',(197.164381039568,4.8989493242116,131.239651992747));
#207209=CARTESIAN_POINT('Ctrl Pts',(197.156623998683,4.91106014690847,131.103351780867));
#207210=CARTESIAN_POINT('Ctrl Pts',(197.148866957798,4.91749102928209,130.966403289417));
#207211=CARTESIAN_POINT('Ctrl Pts',(197.141109916913,4.91818667583652,130.829318264172));
#207212=CARTESIAN_POINT('Ctrl Pts',(197.133358725673,4.91888179779847,130.692336615812));
#207213=CARTESIAN_POINT('Ctrl Pts',(197.125607534433,4.91385029058759,130.555219027973));
#207214=CARTESIAN_POINT('Ctrl Pts',(197.117856343193,4.90308880637215,130.418480818499));
#207215=CARTESIAN_POINT('Ctrl Pts',(197.110108446416,4.89233189607456,130.281800726411));
#207216=CARTESIAN_POINT('Ctrl Pts',(197.102360549639,4.87584988319397,130.145500080927));
#207217=CARTESIAN_POINT('Ctrl Pts',(197.094612652862,4.85369149206835,130.010092424621));
#207218=CARTESIAN_POINT('Ctrl Pts',(197.086866376778,4.83153773600045,129.874713092679));
#207219=CARTESIAN_POINT('Ctrl Pts',(197.079120100694,4.80371002654195,129.740226763961));
#207220=CARTESIAN_POINT('Ctrl Pts',(197.071373824609,4.77030870450874,129.607139699695));
#207221=CARTESIAN_POINT('Ctrl Pts',(197.063627491344,4.7369071359146,129.474051653011));
#207222=CARTESIAN_POINT('Ctrl Pts',(197.055881158079,4.69793196781799,129.342363270595));
#207223=CARTESIAN_POINT('Ctrl Pts',(197.048134824813,4.65353410543624,129.212568108461));
#207224=CARTESIAN_POINT('Ctrl Pts',(197.04038675681,4.60912630046099,129.082743879601));
#207225=CARTESIAN_POINT('Ctrl Pts',(197.032638688807,4.55929351124709,128.954814084533));
#207226=CARTESIAN_POINT('Ctrl Pts',(197.024890620804,4.50423557151517,128.829254296682));
#207227=CARTESIAN_POINT('Ctrl Pts',(197.017134318063,4.44911911554975,128.703561062393));
#207228=CARTESIAN_POINT('Ctrl Pts',(197.009378015321,4.3887665729042,128.580243225664));
#207229=CARTESIAN_POINT('Ctrl Pts',(197.001621712579,4.32342498015975,128.459754146657));
#207230=CARTESIAN_POINT('Ctrl Pts',(196.993861270065,4.25804851263973,128.339200759));
#207231=CARTESIAN_POINT('Ctrl Pts',(196.986100827551,4.18767788965592,128.22147947287));
#207232=CARTESIAN_POINT('Ctrl Pts',(196.978340385036,4.11260413590295,128.107015574036));
#207233=CARTESIAN_POINT('Ctrl Pts',(196.970567484771,4.03740986709589,127.992367927591));
#207234=CARTESIAN_POINT('Ctrl Pts',(196.962794584506,3.95749760849355,127.880988435588));
#207235=CARTESIAN_POINT('Ctrl Pts',(196.95502168424,3.87319995331092,127.773270849154));
#207236=CARTESIAN_POINT('Ctrl Pts',(196.947531348478,3.79196673022726,127.669469068311));
#207237=CARTESIAN_POINT('Ctrl Pts',(196.940041012716,3.70666161488837,127.569067811088));
#207238=CARTESIAN_POINT('Ctrl Pts',(196.932550676954,3.61761389535537,127.472386312948));
#207239=CARTESIAN_POINT('Ctrl Pts',(196.924776342835,3.52518990447059,127.372039106421));
#207240=CARTESIAN_POINT('Ctrl Pts',(196.917002008716,3.42844113395928,127.275381426659));
#207241=CARTESIAN_POINT('Ctrl Pts',(196.909227674597,3.32769387143375,127.182808939));
#207242=CARTESIAN_POINT('Ctrl Pts',(196.90146292165,3.22707077090526,127.090350538659));
#207243=CARTESIAN_POINT('Ctrl Pts',(196.893698168703,3.12245926830746,127.001967574988));
#207244=CARTESIAN_POINT('Ctrl Pts',(196.885933415755,3.01422473525758,126.91802142652));
#207245=CARTESIAN_POINT('Ctrl Pts',(196.87817637487,2.90609770227194,126.83415865455));
#207246=CARTESIAN_POINT('Ctrl Pts',(196.870419333985,2.79435510683866,126.754724166296));
#207247=CARTESIAN_POINT('Ctrl Pts',(196.8626622931,2.67939760660565,126.680041094515));
#207248=CARTESIAN_POINT('Ctrl Pts',(196.85491110186,2.56452679671837,126.605414341821));
#207249=CARTESIAN_POINT('Ctrl Pts',(196.84715991062,2.44644623414905,126.535532085827));
#207250=CARTESIAN_POINT('Ctrl Pts',(196.83940871938,2.32558766080939,126.470675685041));
#207251=CARTESIAN_POINT('Ctrl Pts',(196.831660822603,2.20478045558657,126.405846849956));
#207252=CARTESIAN_POINT('Ctrl Pts',(196.823912925826,2.08119793174799,126.346039805974));
#207253=CARTESIAN_POINT('Ctrl Pts',(196.816165029049,1.95529848390204,126.291491142238));
#207254=CARTESIAN_POINT('Ctrl Pts',(196.808418752965,1.82942537150677,126.236953888906));
#207255=CARTESIAN_POINT('Ctrl Pts',(196.800672476881,1.70123665761377,126.187672983311));
#207256=CARTESIAN_POINT('Ctrl Pts',(196.792926200797,1.57121251079405,126.143837652445));
#207257=CARTESIAN_POINT('Ctrl Pts',(196.785179867531,1.44118740416556,126.100001997995));
#207258=CARTESIAN_POINT('Ctrl Pts',(196.777433534266,1.30932720805258,126.061612123386));
#207259=CARTESIAN_POINT('Ctrl Pts',(196.769687201001,1.17612873306436,126.028807846864));
#207260=CARTESIAN_POINT('Ctrl Pts',(196.761939132998,1.04290042920136,125.995996224052));
#207261=CARTESIAN_POINT('Ctrl Pts',(196.754191064995,0.908333629647398,
125.968772781862));
#207262=CARTESIAN_POINT('Ctrl Pts',(196.746442996992,0.772936462800047,
125.947226453579));
#207263=CARTESIAN_POINT('Ctrl Pts',(196.73868669425,0.63739539423235,125.925657225601));
#207264=CARTESIAN_POINT('Ctrl Pts',(196.730930391508,0.501022582156627,
125.909777226043));
#207265=CARTESIAN_POINT('Ctrl Pts',(196.723174088766,0.364332980624142,
125.899623668276));
#207266=CARTESIAN_POINT('Ctrl Pts',(196.715413646252,0.227570423735663,
125.88946469125));
#207267=CARTESIAN_POINT('Ctrl Pts',(196.707653203738,0.0904911310544043,
125.88503825871));
#207268=CARTESIAN_POINT('Ctrl Pts',(196.699892761224,-0.0463897865020519,
125.886329400686));
#207269=CARTESIAN_POINT('Ctrl Pts',(196.692119860958,-0.183490437459122,
125.887622615317));
#207270=CARTESIAN_POINT('Ctrl Pts',(196.684346960693,-0.320391686252509,
125.894651725689));
#207271=CARTESIAN_POINT('Ctrl Pts',(196.676574060427,-0.456582484150821,
125.907349743812));
#207272=CARTESIAN_POINT('Ctrl Pts',(196.669083724665,-0.587822403502649,
125.919586156992));
#207273=CARTESIAN_POINT('Ctrl Pts',(196.661593388903,-0.718402323251377,
125.937086434526));
#207274=CARTESIAN_POINT('Ctrl Pts',(196.654103053141,-0.847875673318612,
125.959746091611));
#207275=CARTESIAN_POINT('Ctrl Pts',(196.646328719022,-0.982258044805317,
125.983264896481));
#207276=CARTESIAN_POINT('Ctrl Pts',(196.638554384903,-1.11587396195838,
126.012416540273));
#207277=CARTESIAN_POINT('Ctrl Pts',(196.630780050784,-1.24821417389864,
126.047140374758));
#207278=CARTESIAN_POINT('Ctrl Pts',(196.623015297837,-1.38039128835494,
126.081821415221));
#207279=CARTESIAN_POINT('Ctrl Pts',(196.61525054489,-1.51129545125909,126.12206088437));
#207280=CARTESIAN_POINT('Ctrl Pts',(196.607485791943,-1.64042513233221,
126.16774671864));
#207281=CARTESIAN_POINT('Ctrl Pts',(196.599728751058,-1.76942655998645,
126.213387177096));
#207282=CARTESIAN_POINT('Ctrl Pts',(196.591971710173,-1.89665664695338,
126.264463106153));
#207283=CARTESIAN_POINT('Ctrl Pts',(196.584214669288,-2.02162696724649,
126.320812082332));
#207284=CARTESIAN_POINT('Ctrl Pts',(196.576463478048,-2.14650304644767,
126.377118565309));
#207285=CARTESIAN_POINT('Ctrl Pts',(196.568712286808,-2.26912239593048,
126.43869002048));
#207286=CARTESIAN_POINT('Ctrl Pts',(196.560961095568,-2.38901493376489,
126.505315292293));
#207287=CARTESIAN_POINT('Ctrl Pts',(196.55321319879,-2.50885651407307,126.571912246589));
#207288=CARTESIAN_POINT('Ctrl Pts',(196.545465302013,-2.62597324680375,
126.643558555793));
#207289=CARTESIAN_POINT('Ctrl Pts',(196.537717405236,-2.73991830932937,
126.719996441748));
#207290=CARTESIAN_POINT('Ctrl Pts',(196.529971129152,-2.85383953700426,
126.796418338546));
#207291=CARTESIAN_POINT('Ctrl Pts',(196.522224853068,-2.96459008963101,
126.87762960081));
#207292=CARTESIAN_POINT('Ctrl Pts',(196.514478576984,-3.07175122234275,
126.963328530934));
#207293=CARTESIAN_POINT('Ctrl Pts',(196.506732243719,-3.17891314609344,
127.049028093668));
#207294=CARTESIAN_POINT('Ctrl Pts',(196.498985910453,-3.28248529172354,
127.139215146181));
#207295=CARTESIAN_POINT('Ctrl Pts',(196.491239577188,-3.38208148791119,
127.233547282816));
#207296=CARTESIAN_POINT('Ctrl Pts',(196.483491509185,-3.48169998797647,
127.327900544479));
#207297=CARTESIAN_POINT('Ctrl Pts',(196.475743441182,-3.57734048303421,
127.426400468601));
#207298=CARTESIAN_POINT('Ctrl Pts',(196.467995373179,-3.6686534951838,127.528667622981));
#207299=CARTESIAN_POINT('Ctrl Pts',(196.460239070437,-3.76006355588962,
127.631043468109));
#207300=CARTESIAN_POINT('Ctrl Pts',(196.452482767696,-3.8471366852804,127.737194249536));
#207301=CARTESIAN_POINT('Ctrl Pts',(196.444726464954,-3.92956322945105,
127.846706836569));
#207302=CARTESIAN_POINT('Ctrl Pts',(196.43696602244,-4.01203376715042,127.956277873767));
#207303=CARTESIAN_POINT('Ctrl Pts',(196.429205579925,-4.08985255625137,
128.069213970078));
#207304=CARTESIAN_POINT('Ctrl Pts',(196.421445137411,-4.16275376138207,
128.185073656464));
#207305=CARTESIAN_POINT('Ctrl Pts',(196.413672237146,-4.23577199399886,
128.301119331103));
#207306=CARTESIAN_POINT('Ctrl Pts',(196.40589933688,-4.30385667334007,128.42009763481));
#207307=CARTESIAN_POINT('Ctrl Pts',(196.398126436615,-4.36678792397595,
128.541542399167));
#207308=CARTESIAN_POINT('Ctrl Pts',(196.390636100853,-4.42743146513705,
128.65857234044));
#207309=CARTESIAN_POINT('Ctrl Pts',(196.383145765091,-4.48328962222919,
128.777892252615));
#207310=CARTESIAN_POINT('Ctrl Pts',(196.375655429329,-4.53420891924256,
128.899069947048));
#207311=CARTESIAN_POINT('Ctrl Pts',(196.366995286457,-4.59308056412885,
129.03917263136));
#207312=CARTESIAN_POINT('Ctrl Pts',(196.358335143585,-4.64550922581911,
129.182135375472));
#207313=CARTESIAN_POINT('Ctrl Pts',(196.349675000714,-4.69123825435021,
129.327381706606));
#207314=CARTESIAN_POINT('Ctrl Pts',(196.344648349249,-4.71778099061184,
129.411687784913));
#207315=CARTESIAN_POINT('Ctrl Pts',(196.339621697785,-4.74206742463025,
129.496762736058));
#207316=CARTESIAN_POINT('Ctrl Pts',(196.33459504632,-4.76405452823405,129.582490119308));
#207317=CARTESIAN_POINT('',(198.360140564038,-4.91824805313947,130.80873672198));
#207318=CARTESIAN_POINT('Ctrl Pts',(198.360140564008,-4.918248053139,130.808736722507));
#207319=CARTESIAN_POINT('Ctrl Pts',(198.348902089221,-4.91807175747449,
131.006873152139));
#207320=CARTESIAN_POINT('Ctrl Pts',(198.337663614434,-4.90591901972274,
131.20449843287));
#207321=CARTESIAN_POINT('Ctrl Pts',(198.326425139647,-4.8819937463978,131.400447962368));
#207322=CARTESIAN_POINT('Ctrl Pts',(198.319350026384,-4.86693173648915,
131.523806793625));
#207323=CARTESIAN_POINT('Ctrl Pts',(198.312274913122,-4.84720485499847,
131.646502289585));
#207324=CARTESIAN_POINT('Ctrl Pts',(198.30519979986,-4.82287271835716,131.768249514185));
#207325=CARTESIAN_POINT('Ctrl Pts',(198.297425465741,-4.79613587993932,
131.902028800401));
#207326=CARTESIAN_POINT('Ctrl Pts',(198.289651131622,-4.76378621750837,
132.0349066804));
#207327=CARTESIAN_POINT('Ctrl Pts',(198.281876797503,-4.7258965824454,132.166375505345));
#207328=CARTESIAN_POINT('Ctrl Pts',(198.274112044556,-4.68805364297136,
132.297682306713));
#207329=CARTESIAN_POINT('Ctrl Pts',(198.266347291608,-4.64468442282832,
132.427583136145));
#207330=CARTESIAN_POINT('Ctrl Pts',(198.258582538661,-4.59591298865343,
132.555579297008));
#207331=CARTESIAN_POINT('Ctrl Pts',(198.250825497776,-4.54718999495454,
132.683448330279));
#207332=CARTESIAN_POINT('Ctrl Pts',(198.243068456891,-4.49307560322901,
132.809416096658));
#207333=CARTESIAN_POINT('Ctrl Pts',(198.235311416006,-4.43374391105737,
132.932998208529));
#207334=CARTESIAN_POINT('Ctrl Pts',(198.227560224766,-4.37445696137642,
133.056487126168));
#207335=CARTESIAN_POINT('Ctrl Pts',(198.219809033526,-4.30996071097418,
133.177593619155));
#207336=CARTESIAN_POINT('Ctrl Pts',(198.212057842286,-4.24047753526522,
133.295852808084));
#207337=CARTESIAN_POINT('Ctrl Pts',(198.204309945509,-4.17102389175934,
133.414061733703));
#207338=CARTESIAN_POINT('Ctrl Pts',(198.196562048732,-4.09658773626326,
133.529425425838));
#207339=CARTESIAN_POINT('Ctrl Pts',(198.188814151955,-4.01743749521107,
133.6415033765));
#207340=CARTESIAN_POINT('Ctrl Pts',(198.181067875871,-3.93830381068304,
133.753557882871));
#207341=CARTESIAN_POINT('Ctrl Pts',(198.173321599787,-3.85445822736556,
133.862327695705));
#207342=CARTESIAN_POINT('Ctrl Pts',(198.165575323702,-3.76621240470724,
133.967401430633));
#207343=CARTESIAN_POINT('Ctrl Pts',(198.157828990437,-3.67796593063832,
134.072475941192));
#207344=CARTESIAN_POINT('Ctrl Pts',(198.150082657172,-3.58531940385276,
134.173854020016));
#207345=CARTESIAN_POINT('Ctrl Pts',(198.142336323906,-3.48862439845058,
134.271157823783));
#207346=CARTESIAN_POINT('Ctrl Pts',(198.134588255903,-3.3919077388725,134.368483418062));
#207347=CARTESIAN_POINT('Ctrl Pts',(198.126840187901,-3.29114107212411,
134.461732644436));
#207348=CARTESIAN_POINT('Ctrl Pts',(198.119092119898,-3.18671210764418,
134.550565230971));
#207349=CARTESIAN_POINT('Ctrl Pts',(198.111335817156,-3.08217215481793,
134.639492229836));
#207350=CARTESIAN_POINT('Ctrl Pts',(198.103579514414,-2.97396242717541,
134.723992958252));
#207351=CARTESIAN_POINT('Ctrl Pts',(198.095823211672,-2.86250336727734,
134.803767765485));
#207352=CARTESIAN_POINT('Ctrl Pts',(198.088062769158,-2.75098481832297,
134.883585150935));
#207353=CARTESIAN_POINT('Ctrl Pts',(198.080302326644,-2.63621380844923,
134.958671375235));
#207354=CARTESIAN_POINT('Ctrl Pts',(198.07254188413,-2.51863805887903,135.028771273606));
#207355=CARTESIAN_POINT('Ctrl Pts',(198.064768983864,-2.40087356627779,
135.098983702558));
#207356=CARTESIAN_POINT('Ctrl Pts',(198.056996083599,-2.2802956808095,135.164193623964));
#207357=CARTESIAN_POINT('Ctrl Pts',(198.049223183333,-2.15737571304909,
135.22419241247));
#207358=CARTESIAN_POINT('Ctrl Pts',(198.041732847571,-2.03892419573207,
135.282010093887));
#207359=CARTESIAN_POINT('Ctrl Pts',(198.034242511809,-1.91829820299034,
135.33498881632));
#207360=CARTESIAN_POINT('Ctrl Pts',(198.026752176047,-1.79593348200914,
135.382985519291));
#207361=CARTESIAN_POINT('Ctrl Pts',(198.018977841928,-1.66892926544145,
135.432802031844));
#207362=CARTESIAN_POINT('Ctrl Pts',(198.011203507809,-1.53964955897284,
135.477409084513));
#207363=CARTESIAN_POINT('Ctrl Pts',(198.00342917369,-1.40856083989839,135.516593572631));
#207364=CARTESIAN_POINT('Ctrl Pts',(197.995664420743,-1.27763367595456,
135.555729769371));
#207365=CARTESIAN_POINT('Ctrl Pts',(197.987899667796,-1.14490230633097,
135.589456587496));
#207366=CARTESIAN_POINT('Ctrl Pts',(197.980134914848,-1.01085335967749,
135.617608850073));
#207367=CARTESIAN_POINT('Ctrl Pts',(197.972377873963,-0.876937552327542,
135.645733151425));
#207368=CARTESIAN_POINT('Ctrl Pts',(197.964620833078,-0.741707152334974,
135.668293835729));
#207369=CARTESIAN_POINT('Ctrl Pts',(197.956863792193,-0.605663792714778,
135.685175552871));
#207370=CARTESIAN_POINT('Ctrl Pts',(197.949112600953,-0.469723024450324,
135.702044539379));
#207371=CARTESIAN_POINT('Ctrl Pts',(197.941361409713,-0.332970903234851,
135.713243034937));
#207372=CARTESIAN_POINT('Ctrl Pts',(197.933610218473,-0.195918744622959,
135.718706851604));
#207373=CARTESIAN_POINT('Ctrl Pts',(197.925862321696,-0.0589248368344638,
135.724168346004));
#207374=CARTESIAN_POINT('Ctrl Pts',(197.918114424919,0.0783684648781298,
135.723899993757));
#207375=CARTESIAN_POINT('Ctrl Pts',(197.910366528142,0.215445457623812,
135.717889524298));
#207376=CARTESIAN_POINT('Ctrl Pts',(197.902620252058,0.352493776817673,
135.711880312099));
#207377=CARTESIAN_POINT('Ctrl Pts',(197.894873975974,0.489325486701273,
135.700131388911));
#207378=CARTESIAN_POINT('Ctrl Pts',(197.88712769989,0.625426018410143,135.682682599354));
#207379=CARTESIAN_POINT('Ctrl Pts',(197.879381366624,0.761527554782069,
135.665233680994));
#207380=CARTESIAN_POINT('Ctrl Pts',(197.871635033359,0.896897514417944,
135.642084862025));
#207381=CARTESIAN_POINT('Ctrl Pts',(197.863888700093,1.03102797264083,135.613327698149));
#207382=CARTESIAN_POINT('Ctrl Pts',(197.856140632091,1.16518846844996,135.584564094306));
#207383=CARTESIAN_POINT('Ctrl Pts',(197.848392564088,1.29810852829368,135.550189728304));
#207384=CARTESIAN_POINT('Ctrl Pts',(197.840644496085,1.42929230533578,135.510346865783));
#207385=CARTESIAN_POINT('Ctrl Pts',(197.832888193343,1.56061550605723,135.470461657794));
#207386=CARTESIAN_POINT('Ctrl Pts',(197.825131890601,1.69019836301931,135.425096457024));
#207387=CARTESIAN_POINT('Ctrl Pts',(197.817375587859,1.81756151209824,135.374443025164));
#207388=CARTESIAN_POINT('Ctrl Pts',(197.809615145345,1.94499263872476,135.323762558043));
#207389=CARTESIAN_POINT('Ctrl Pts',(197.801854702831,2.0702013400551,135.267788395269));
#207390=CARTESIAN_POINT('Ctrl Pts',(197.794094260316,2.19273093447755,135.206759294593));
#207391=CARTESIAN_POINT('Ctrl Pts',(197.786321360051,2.3154572242826,135.145632224586));
#207392=CARTESIAN_POINT('Ctrl Pts',(197.778548459786,2.43549547037675,135.079434189959));
#207393=CARTESIAN_POINT('Ctrl Pts',(197.77077555952,2.55241539546258,135.008448950547));
#207394=CARTESIAN_POINT('Ctrl Pts',(197.763285223758,2.66508498676848,134.940044203388));
#207395=CARTESIAN_POINT('Ctrl Pts',(197.755794887996,2.77485878191613,134.867194432942));
#207396=CARTESIAN_POINT('Ctrl Pts',(197.748304552234,2.88138088807747,134.790188917973));
#207397=CARTESIAN_POINT('Ctrl Pts',(197.740530218115,2.99194181227019,134.710263715498));
#207398=CARTESIAN_POINT('Ctrl Pts',(197.732755883996,3.09934982819655,134.62560823861));
#207399=CARTESIAN_POINT('Ctrl Pts',(197.724981549877,3.20317350249298,134.53649975959));
#207400=CARTESIAN_POINT('Ctrl Pts',(197.71721679693,3.3068692233898,134.447501098806));
#207401=CARTESIAN_POINT('Ctrl Pts',(197.709452043983,3.40698909809778,134.354060607414));
#207402=CARTESIAN_POINT('Ctrl Pts',(197.701687291035,3.50313112391044,134.256498417711));
#207403=CARTESIAN_POINT('Ctrl Pts',(197.69393025015,3.5991776601077,134.15903312815));
#207404=CARTESIAN_POINT('Ctrl Pts',(197.686173209265,3.6912539371464,134.057454563654));
#207405=CARTESIAN_POINT('Ctrl Pts',(197.67841616838,3.77899176281173,133.952122412731));
#207406=CARTESIAN_POINT('Ctrl Pts',(197.67066497714,3.86666342470019,133.846869693603));
#207407=CARTESIAN_POINT('Ctrl Pts',(197.6629137859,3.95000289804419,133.737869321391));
#207408=CARTESIAN_POINT('Ctrl Pts',(197.65516259466,4.02867980116461,133.625516785202));
#207409=CARTESIAN_POINT('Ctrl Pts',(197.647414697883,4.10732326450247,133.513212001837));
#207410=CARTESIAN_POINT('Ctrl Pts',(197.639666801106,4.18130787530829,133.397558207814));
#207411=CARTESIAN_POINT('Ctrl Pts',(197.631918904329,4.25034455999749,133.278982646038));
#207412=CARTESIAN_POINT('Ctrl Pts',(197.624172628245,4.31936680370051,133.160431887714));
#207413=CARTESIAN_POINT('Ctrl Pts',(197.616426352161,4.38344298336774,133.038960914946));
#207414=CARTESIAN_POINT('Ctrl Pts',(197.608680076076,4.4423284843672,132.915024186087));
#207415=CARTESIAN_POINT('Ctrl Pts',(197.600933742811,4.50121442004603,132.791086542354));
#207416=CARTESIAN_POINT('Ctrl Pts',(197.593187409546,4.55490943281703,132.664683459342));
#207417=CARTESIAN_POINT('Ctrl Pts',(197.58544107628,4.60321600539095,132.536291756559));
#207418=CARTESIAN_POINT('Ctrl Pts',(197.577693008277,4.65153339588684,132.407871301344));
#207419=CARTESIAN_POINT('Ctrl Pts',(197.569944940274,4.69445980733516,132.277461706041));
#207420=CARTESIAN_POINT('Ctrl Pts',(197.562196872271,4.73184691452124,132.14555703869));
#207421=CARTESIAN_POINT('Ctrl Pts',(197.55444056953,4.76927375716978,132.013512181488));
#207422=CARTESIAN_POINT('Ctrl Pts',(197.546684266788,4.80114942837765,131.879969454826));
#207423=CARTESIAN_POINT('Ctrl Pts',(197.538927964046,4.82737615466953,131.745435813195));
#207424=CARTESIAN_POINT('Ctrl Pts',(197.531167521532,4.85361687895492,131.610830366909));
#207425=CARTESIAN_POINT('Ctrl Pts',(197.523407079018,4.87420259200423,131.475233338161));
#207426=CARTESIAN_POINT('Ctrl Pts',(197.515646636503,4.88908731990802,131.33915800052));
#207427=CARTESIAN_POINT('Ctrl Pts',(197.507873736238,4.90399594209845,131.202864222668));
#207428=CARTESIAN_POINT('Ctrl Pts',(197.500100835973,4.91318526485212,131.066090991876));
#207429=CARTESIAN_POINT('Ctrl Pts',(197.492327935707,4.91666144796523,130.929353691744));
#207430=CARTESIAN_POINT('Ctrl Pts',(197.484837599945,4.9200112630662,130.797587136892));
#207431=CARTESIAN_POINT('Ctrl Pts',(197.477347264183,4.91805610562799,130.665854253699));
#207432=CARTESIAN_POINT('Ctrl Pts',(197.469856928421,4.91084698530234,130.534610827118));
#207433=CARTESIAN_POINT('Ctrl Pts',(197.462082594302,4.90336452898838,130.398391266127));
#207434=CARTESIAN_POINT('Ctrl Pts',(197.454308260183,4.89019813490943,130.262267507292));
#207435=CARTESIAN_POINT('Ctrl Pts',(197.446533926064,4.87134787981786,130.126752400162));
#207436=CARTESIAN_POINT('Ctrl Pts',(197.438769173117,4.852520855981,129.991404303289));
#207437=CARTESIAN_POINT('Ctrl Pts',(197.43100442017,4.82802396204446,129.856663749147));
#207438=CARTESIAN_POINT('Ctrl Pts',(197.423239667222,4.79790924209346,129.723041993323));
#207439=CARTESIAN_POINT('Ctrl Pts',(197.415482626337,4.76782443250686,129.589552952511));
#207440=CARTESIAN_POINT('Ctrl Pts',(197.407725585452,4.73213298616931,129.457180877599));
#207441=CARTESIAN_POINT('Ctrl Pts',(197.399968544567,4.69093850232438,129.326429959548));
#207442=CARTESIAN_POINT('Ctrl Pts',(197.392217353327,4.64977508356018,129.195777641781));
#207443=CARTESIAN_POINT('Ctrl Pts',(197.384466162087,4.60311700438922,129.066744418897));
#207444=CARTESIAN_POINT('Ctrl Pts',(197.376714970847,4.55111842163095,128.939822021883));
#207445=CARTESIAN_POINT('Ctrl Pts',(197.36896707407,4.49914193965744,128.812953570273));
#207446=CARTESIAN_POINT('Ctrl Pts',(197.361219177293,4.44182961657508,128.688194521179));
#207447=CARTESIAN_POINT('Ctrl Pts',(197.353471280516,4.37938465260795,128.56601901562));
#207448=CARTESIAN_POINT('Ctrl Pts',(197.345725004432,4.3169527507811,128.443869066543));
#207449=CARTESIAN_POINT('Ctrl Pts',(197.337978728348,4.24939052141315,128.324301933984));
#207450=CARTESIAN_POINT('Ctrl Pts',(197.330232452263,4.17694809300133,128.207769064997));
#207451=CARTESIAN_POINT('Ctrl Pts',(197.322486118998,4.10450512983598,128.091235335791));
#207452=CARTESIAN_POINT('Ctrl Pts',(197.314739785733,4.02718210215263,127.97773624689));
#207453=CARTESIAN_POINT('Ctrl Pts',(197.306993452467,3.9452734087893,127.867695707775));
#207454=CARTESIAN_POINT('Ctrl Pts',(197.299245384464,3.86334637254203,127.757630525843));
#207455=CARTESIAN_POINT('Ctrl Pts',(197.291497316461,3.77683186054576,127.65102574846));
#207456=CARTESIAN_POINT('Ctrl Pts',(197.283749248458,3.68606537283357,127.548273221672));
#207457=CARTESIAN_POINT('Ctrl Pts',(197.275992945717,3.59520241741809,127.445411488276));
#207458=CARTESIAN_POINT('Ctrl Pts',(197.268236642975,3.50007871824481,127.3464104776));
#207459=CARTESIAN_POINT('Ctrl Pts',(197.260480340233,3.4010679415342,127.251626470523));
#207460=CARTESIAN_POINT('Ctrl Pts',(197.252719897719,3.30200431979083,127.156791874367));
#207461=CARTESIAN_POINT('Ctrl Pts',(197.244959455205,3.19904977993481,127.066179024781));
#207462=CARTESIAN_POINT('Ctrl Pts',(197.23719901269,3.09261130353576,126.980104037818));
#207463=CARTESIAN_POINT('Ctrl Pts',(197.229426112425,2.98600196264525,126.893890875646));
#207464=CARTESIAN_POINT('Ctrl Pts',(197.22165321216,2.87589782337121,126.812230366043));
#207465=CARTESIAN_POINT('Ctrl Pts',(197.213880311894,2.76273582205164,126.735395904024));
#207466=CARTESIAN_POINT('Ctrl Pts',(197.206389976132,2.65368754451797,126.661354568233));
#207467=CARTESIAN_POINT('Ctrl Pts',(197.19889964037,2.54180012866534,126.591794656438));
#207468=CARTESIAN_POINT('Ctrl Pts',(197.191409304608,2.4274846112473,126.526919615675));
#207469=CARTESIAN_POINT('Ctrl Pts',(197.183634970489,2.30883478624092,126.459584818023));
#207470=CARTESIAN_POINT('Ctrl Pts',(197.17586063637,2.18719325510115,126.397083861596));
#207471=CARTESIAN_POINT('Ctrl Pts',(197.168086302251,2.06299153416462,126.339693889526));
#207472=CARTESIAN_POINT('Ctrl Pts',(197.160321549304,1.93894288074894,126.282374645468));
#207473=CARTESIAN_POINT('Ctrl Pts',(197.152556796357,1.81234066695579,126.230154015391));
#207474=CARTESIAN_POINT('Ctrl Pts',(197.144792043409,1.68364315769026,126.183264559263));
#207475=CARTESIAN_POINT('Ctrl Pts',(197.137035002524,1.55507347260519,126.136421674404));
#207476=CARTESIAN_POINT('Ctrl Pts',(197.129277961639,1.42441299845145,126.094899559184));
#207477=CARTESIAN_POINT('Ctrl Pts',(197.121520920754,1.29214192328729,126.058883580156));
#207478=CARTESIAN_POINT('Ctrl Pts',(197.113769729514,1.15997059476984,126.022894761058));
#207479=CARTESIAN_POINT('Ctrl Pts',(197.106018538274,1.02619145846807,125.99240391571));
#207480=CARTESIAN_POINT('Ctrl Pts',(197.098267347034,0.891301547113867,
125.967547140222));
#207481=CARTESIAN_POINT('Ctrl Pts',(197.090519450257,0.756468967570347,
125.942700929528));
#207482=CARTESIAN_POINT('Ctrl Pts',(197.08277155348,0.620526935649892,125.923484096662));
#207483=CARTESIAN_POINT('Ctrl Pts',(197.075023656703,0.483984194306158,
125.909981968323));
#207484=CARTESIAN_POINT('Ctrl Pts',(197.067277380619,0.347470014760427,
125.896482664339));
#207485=CARTESIAN_POINT('Ctrl Pts',(197.059531104535,0.210355764548132,
125.88869572563));
#207486=CARTESIAN_POINT('Ctrl Pts',(197.051784828451,0.0731564594262019,
125.886654730168));
#207487=CARTESIAN_POINT('Ctrl Pts',(197.044038495185,-0.0640438584697734,
125.884613719641));
#207488=CARTESIAN_POINT('Ctrl Pts',(197.03629216192,-0.201328841606274,
125.888318742812));
#207489=CARTESIAN_POINT('Ctrl Pts',(197.028545828654,-0.338182713167988,
125.897751247032));
#207490=CARTESIAN_POINT('Ctrl Pts',(197.020797760651,-0.475067232205337,
125.907185863595));
#207491=CARTESIAN_POINT('Ctrl Pts',(197.013049692649,-0.611520057590418,
125.922350486614));
#207492=CARTESIAN_POINT('Ctrl Pts',(197.005301624646,-0.747030172182732,
125.943174652768));
#207493=CARTESIAN_POINT('Ctrl Pts',(196.997545321904,-0.882684308537553,
125.964020951094));
#207494=CARTESIAN_POINT('Ctrl Pts',(196.989789019162,-1.01739334560279,
125.990538748746));
#207495=CARTESIAN_POINT('Ctrl Pts',(196.98203271642,-1.15065555846418,126.022606248271));
#207496=CARTESIAN_POINT('Ctrl Pts',(196.974272273906,-1.28398889738112,
126.054690863185));
#207497=CARTESIAN_POINT('Ctrl Pts',(196.966511831392,-1.41587349762368,
126.092330974847));
#207498=CARTESIAN_POINT('Ctrl Pts',(196.958751388877,-1.5458234183235,126.135355046584));
#207499=CARTESIAN_POINT('Ctrl Pts',(196.950978488612,-1.67598194617242,
126.17844818438));
#207500=CARTESIAN_POINT('Ctrl Pts',(196.943205588347,-1.80419922236758,
126.226942414954));
#207501=CARTESIAN_POINT('Ctrl Pts',(196.935432688081,-1.93000905717825,
126.280617908071));
#207502=CARTESIAN_POINT('Ctrl Pts',(196.927942352319,-2.05124538759802,
126.332342161813));
#207503=CARTESIAN_POINT('Ctrl Pts',(196.920452016557,-2.17024599270099,
126.388877382166));
#207504=CARTESIAN_POINT('Ctrl Pts',(196.912961680795,-2.28661753132807,
126.44998772036));
#207505=CARTESIAN_POINT('Ctrl Pts',(196.905186437551,-2.40741545658494,
126.513422492751));
#207506=CARTESIAN_POINT('Ctrl Pts',(196.897411194306,-2.52576305120591,
126.581988282265));
#207507=CARTESIAN_POINT('Ctrl Pts',(196.889635951062,-2.6411937391818,126.655471766969));
#207508=CARTESIAN_POINT('Ctrl Pts',(196.881870490011,-2.75647920144334,
126.728862800595));
#207509=CARTESIAN_POINT('Ctrl Pts',(196.874105028959,-2.86885473277439,
126.807159009799));
#207510=CARTESIAN_POINT('Ctrl Pts',(196.866339567908,-2.97787685313513,
126.890100469075));
#207511=CARTESIAN_POINT('Ctrl Pts',(196.858583393819,-3.08676859046736,
126.972942736017));
#207512=CARTESIAN_POINT('Ctrl Pts',(196.85082721973,-3.19231459493436,127.060418953556));
#207513=CARTESIAN_POINT('Ctrl Pts',(196.843071045641,-3.294099502712,127.152225416244));
#207514=CARTESIAN_POINT('Ctrl Pts',(196.835320138421,-3.39581529293819,
127.243969537295));
#207515=CARTESIAN_POINT('Ctrl Pts',(196.827569231201,-3.49377477829833,
127.340037793094));
#207516=CARTESIAN_POINT('Ctrl Pts',(196.819818323981,-3.58759484370538,
127.440085613955));
#207517=CARTESIAN_POINT('Ctrl Pts',(196.812071001449,-3.6813715186174,127.54008716407));
#207518=CARTESIAN_POINT('Ctrl Pts',(196.804323678917,-3.77101231623895,
127.644064332384));
#207519=CARTESIAN_POINT('Ctrl Pts',(196.796576356385,-3.85617053877141,
127.751635304274));
#207520=CARTESIAN_POINT('Ctrl Pts',(196.788830939126,-3.94130781864133,
127.859179821613));
#207521=CARTESIAN_POINT('Ctrl Pts',(196.781085521866,-4.02196447570508,
127.970316076795));
#207522=CARTESIAN_POINT('Ctrl Pts',(196.773340104606,-4.09783398032599,
128.084629062396));
#207523=CARTESIAN_POINT('Ctrl Pts',(196.765580754941,-4.17383995850953,
128.19914767344));
#207524=CARTESIAN_POINT('Ctrl Pts',(196.757821405275,-4.24504131628586,
128.316854134644));
#207525=CARTESIAN_POINT('Ctrl Pts',(196.75006205561,-4.31117357625514,128.437302219913));
#207526=CARTESIAN_POINT('Ctrl Pts',(196.742313049751,-4.37721767686617,
128.557589738676));
#207527=CARTESIAN_POINT('Ctrl Pts',(196.734564043892,-4.43820602078034,
128.680611220613));
#207528=CARTESIAN_POINT('Ctrl Pts',(196.726815038034,-4.49392167184312,
128.805898441332));
#207529=CARTESIAN_POINT('Ctrl Pts',(196.719050516465,-4.54974888145534,
128.931436522632));
#207530=CARTESIAN_POINT('Ctrl Pts',(196.711285994897,-4.60028211429378,
129.059249060427));
#207531=CARTESIAN_POINT('Ctrl Pts',(196.703521473329,-4.64535222085451,
129.188846517751));
#207532=CARTESIAN_POINT('Ctrl Pts',(196.69575695176,-4.69042232741525,129.318443975074));
#207533=CARTESIAN_POINT('Ctrl Pts',(196.687992430192,-4.73002922227267,
129.449825967771));
#207534=CARTESIAN_POINT('Ctrl Pts',(196.680227908624,-4.76405452823405,
129.582490119308));
#207535=CARTESIAN_POINT('Ctrl Pts',(198.430216174721,-4.76405452823404,
129.582490119308));
#207536=CARTESIAN_POINT('Ctrl Pts',(198.422577902284,-4.7976789144689,129.713591090917));
#207537=CARTESIAN_POINT('Ctrl Pts',(198.414939629846,-4.82587604532326,
129.846036456349));
#207538=CARTESIAN_POINT('Ctrl Pts',(198.407301357409,-4.84855734705283,
129.97933048791));
#207539=CARTESIAN_POINT('Ctrl Pts',(198.399441225181,-4.87189744550764,
130.116496152261));
#207540=CARTESIAN_POINT('Ctrl Pts',(198.391581092952,-4.88939633379473,
130.254560081246));
#207541=CARTESIAN_POINT('Ctrl Pts',(198.383720960724,-4.90101480488931,
130.392976436106));
#207542=CARTESIAN_POINT('Ctrl Pts',(198.375860828495,-4.91263327598389,
130.531392790965));
#207543=CARTESIAN_POINT('Ctrl Pts',(198.368000696266,-4.91837135341764,
130.670161108681));
#207544=CARTESIAN_POINT('Ctrl Pts',(198.360140564038,-4.91824805313947,
130.80873672198));
#207545=CARTESIAN_POINT('Origin',(213.235140564004,0.,130.804360617566));
#207546=CARTESIAN_POINT('',(200.179870531952,-4.76405452823405,129.582490119308));
#207547=CARTESIAN_POINT('',(199.834960626423,-4.76405452823405,129.582490119308));
#207548=CARTESIAN_POINT('',(213.235140564004,-4.76405452823405,129.582490119308));
#207549=CARTESIAN_POINT('',(199.76485943604,-4.91824827604694,130.808478585671));
#207550=CARTESIAN_POINT('Ctrl Pts',(199.834960626423,-4.76405452823405,
129.582490119308));
#207551=CARTESIAN_POINT('Ctrl Pts',(199.827324041593,-4.79766326068053,
129.713530057033));
#207552=CARTESIAN_POINT('Ctrl Pts',(199.819687456764,-4.82584625215587,
129.845899345302));
#207553=CARTESIAN_POINT('Ctrl Pts',(199.812050871934,-4.84851847510395,
129.979102076819));
#207554=CARTESIAN_POINT('Ctrl Pts',(199.804185632618,-4.87186954934494,
130.116293162135));
#207555=CARTESIAN_POINT('Ctrl Pts',(199.796320393303,-4.88937460082088,
130.254367925497));
#207556=CARTESIAN_POINT('Ctrl Pts',(199.788455153987,-4.90099827408403,
130.392779544234));
#207557=CARTESIAN_POINT('Ctrl Pts',(199.780589914672,-4.91262194734719,
130.53119116297));
#207558=CARTESIAN_POINT('Ctrl Pts',(199.772724675356,-4.91836427281118,
130.669939172252));
#207559=CARTESIAN_POINT('Ctrl Pts',(199.76485943604,-4.91824827604694,130.808478585671));
#207560=CARTESIAN_POINT('Ctrl Pts',(199.764859435991,-4.91824827604621,
130.808478586542));
#207561=CARTESIAN_POINT('Ctrl Pts',(199.752723897668,-4.91806930075772,
131.022235637443));
#207562=CARTESIAN_POINT('Ctrl Pts',(199.740588359346,-4.90395198746022,
131.235429274479));
#207563=CARTESIAN_POINT('Ctrl Pts',(199.728452821023,-4.87613221702235,
131.446635998237));
#207564=CARTESIAN_POINT('Ctrl Pts',(199.72464418571,-4.86740121908247,131.512921429102));
#207565=CARTESIAN_POINT('Ctrl Pts',(199.720835550396,-4.85732086664738,
131.57901143828));
#207566=CARTESIAN_POINT('Ctrl Pts',(199.717026915083,-4.84589923841166,
131.64486263045));
#207567=CARTESIAN_POINT('Ctrl Pts',(199.709252580964,-4.82258496786947,
131.779280637941));
#207568=CARTESIAN_POINT('Ctrl Pts',(199.701478246845,-4.79363669851475,
131.912940764209));
#207569=CARTESIAN_POINT('Ctrl Pts',(199.693703912726,-4.75911430351347,
132.045333666666));
#207570=CARTESIAN_POINT('Ctrl Pts',(199.685939159779,-4.7246344542787,132.177563406704));
#207571=CARTESIAN_POINT('Ctrl Pts',(199.678174406832,-4.68459424557846,
132.308528655646));
#207572=CARTESIAN_POINT('Ctrl Pts',(199.670409653885,-4.63910497760412,
132.437727713252));
#207573=CARTESIAN_POINT('Ctrl Pts',(199.662652613,-4.59366089021201,132.566798448532));
#207574=CARTESIAN_POINT('Ctrl Pts',(199.654895572115,-4.54277864283484,
132.694106117038));
#207575=CARTESIAN_POINT('Ctrl Pts',(199.64713853123,-4.48661991546082,132.819162046166));
#207576=CARTESIAN_POINT('Ctrl Pts',(199.63938733999,-4.43050353782002,132.944123669646));
#207577=CARTESIAN_POINT('Ctrl Pts',(199.631636148749,-4.36911875972351,
133.066836578412));
#207578=CARTESIAN_POINT('Ctrl Pts',(199.623884957509,-4.30267602109411,
133.186830369735));
#207579=CARTESIAN_POINT('Ctrl Pts',(199.616137060732,-4.23626152240097,
133.306773160497));
#207580=CARTESIAN_POINT('Ctrl Pts',(199.608389163955,-4.16479352789244,
133.423998791095));
#207581=CARTESIAN_POINT('Ctrl Pts',(199.600641267178,-4.08852913543883,
133.538060047124));
#207582=CARTESIAN_POINT('Ctrl Pts',(199.592894991094,-4.01228069585204,
133.652097443998));
#207583=CARTESIAN_POINT('Ctrl Pts',(199.58514871501,-3.93123807111655,133.762971458094));
#207584=CARTESIAN_POINT('Ctrl Pts',(199.577402438926,-3.84570232123248,
133.870262885899));
#207585=CARTESIAN_POINT('Ctrl Pts',(199.56965610566,-3.76016593994299,133.977555105704));
#207586=CARTESIAN_POINT('Ctrl Pts',(199.561909772395,-3.67013661103911,
134.081264380741));
#207587=CARTESIAN_POINT('Ctrl Pts',(199.554163439129,-3.57595615209479,
134.181004019051));
#207588=CARTESIAN_POINT('Ctrl Pts',(199.546415371126,-3.48175460208978,
134.280765993363));
#207589=CARTESIAN_POINT('Ctrl Pts',(199.538667303124,-3.38340034058184,
134.376556277787));
#207590=CARTESIAN_POINT('Ctrl Pts',(199.530919235121,-3.28127226748557,
134.468024817398));
#207591=CARTESIAN_POINT('Ctrl Pts',(199.523162932379,-3.17903565145775,
134.559590570861));
#207592=CARTESIAN_POINT('Ctrl Pts',(199.515406629637,-3.07301750343207,
134.646825142842));
#207593=CARTESIAN_POINT('Ctrl Pts',(199.507650326895,-2.96363048238186,
134.729418251079));
#207594=CARTESIAN_POINT('Ctrl Pts',(199.499889884381,-2.85418507818486,
134.812055441745));
#207595=CARTESIAN_POINT('Ctrl Pts',(199.492129441867,-2.7413675396017,134.890046010246));
#207596=CARTESIAN_POINT('Ctrl Pts',(199.484368999352,-2.62561893060417,
134.963123449678));
#207597=CARTESIAN_POINT('Ctrl Pts',(199.476596099087,-2.50968451166382,
135.036318199503));
#207598=CARTESIAN_POINT('Ctrl Pts',(199.468823198821,-2.3908099590241,135.104583864727));
#207599=CARTESIAN_POINT('Ctrl Pts',(199.461050298556,-2.26946110594807,
135.167699860748));
#207600=CARTESIAN_POINT('Ctrl Pts',(199.453559962794,-2.15252358934225,
135.228521431332));
#207601=CARTESIAN_POINT('Ctrl Pts',(199.446069627032,-2.03328882194573,
135.284561108335));
#207602=CARTESIAN_POINT('Ctrl Pts',(199.43857929127,-1.91218875833745,135.335664758207));
#207603=CARTESIAN_POINT('Ctrl Pts',(199.430804957151,-1.78649714900839,
135.388706018497));
#207604=CARTESIAN_POINT('Ctrl Pts',(199.423030623032,-1.65839785264128,
135.436597582708));
#207605=CARTESIAN_POINT('Ctrl Pts',(199.415256288913,-1.52835175648752,
135.479114511724));
#207606=CARTESIAN_POINT('Ctrl Pts',(199.407491535966,-1.39846593052474,
135.521579042424));
#207607=CARTESIAN_POINT('Ctrl Pts',(199.399726783019,-1.26663844662274,
135.558681996903));
#207608=CARTESIAN_POINT('Ctrl Pts',(199.391962030072,-1.13335155987423,
135.590245833932));
#207609=CARTESIAN_POINT('Ctrl Pts',(199.384204989187,-1.00019705554075,
135.621778321313));
#207610=CARTESIAN_POINT('Ctrl Pts',(199.376447948302,-0.865586410911478,
135.647782550024));
#207611=CARTESIAN_POINT('Ctrl Pts',(199.368690907417,-0.730018152069129,
135.668130406541));
#207612=CARTESIAN_POINT('Ctrl Pts',(199.360939716176,-0.594552126305398,
135.688462918582));
#207613=CARTESIAN_POINT('Ctrl Pts',(199.353188524936,-0.458130308783093,
135.703147490879));
#207614=CARTESIAN_POINT('Ctrl Pts',(199.345437333696,-0.321262210558749,
135.712106908336));
#207615=CARTESIAN_POINT('Ctrl Pts',(199.337689436919,-0.184452284927075,
135.721062517801));
#207616=CARTESIAN_POINT('Ctrl Pts',(199.329941540142,-0.0471968451682756,
135.724297786676));
#207617=CARTESIAN_POINT('Ctrl Pts',(199.322193643365,0.0899888868944208,
135.72178728837));
#207618=CARTESIAN_POINT('Ctrl Pts',(199.314447367281,0.227145922659364,
135.719277315206));
#207619=CARTESIAN_POINT('Ctrl Pts',(199.306701091197,0.3642328890792,135.711023972638));
#207620=CARTESIAN_POINT('Ctrl Pts',(199.298954815113,0.500734368080969,
135.697053961229));
#207621=CARTESIAN_POINT('Ctrl Pts',(199.291208481847,0.637236854705554,
135.683083846697));
#207622=CARTESIAN_POINT('Ctrl Pts',(199.283462148582,0.773153456354327,
135.663397018924));
#207623=CARTESIAN_POINT('Ctrl Pts',(199.275715815317,0.907974077383442,
135.638072042269));
#207624=CARTESIAN_POINT('Ctrl Pts',(199.267967747314,1.04282489055591,135.61274139426));
#207625=CARTESIAN_POINT('Ctrl Pts',(199.260219679311,1.17657885054553,135.581770157055));
#207626=CARTESIAN_POINT('Ctrl Pts',(199.252471611308,1.30873664156906,135.545287896645));
#207627=CARTESIAN_POINT('Ctrl Pts',(199.244715308566,1.4410348914656,135.508766862454));
#207628=CARTESIAN_POINT('Ctrl Pts',(199.236959005824,1.57173320612938,135.466723208909));
#207629=CARTESIAN_POINT('Ctrl Pts',(199.229202703082,1.70034748405164,135.419336402549));
#207630=CARTESIAN_POINT('Ctrl Pts',(199.221442260568,1.82903040728659,135.371924304424));
#207631=CARTESIAN_POINT('Ctrl Pts',(199.213681818054,1.95562671669996,135.319163521356));
#207632=CARTESIAN_POINT('Ctrl Pts',(199.20592137554,2.0796737866346,135.261281079464));
#207633=CARTESIAN_POINT('Ctrl Pts',(199.198148475274,2.2039199879383,135.203305719538));
#207634=CARTESIAN_POINT('Ctrl Pts',(199.190375575009,2.32560842485003,135.140192451236));
#207635=CARTESIAN_POINT('Ctrl Pts',(199.182602674743,2.44430171903778,135.072213961908));
#207636=CARTESIAN_POINT('Ctrl Pts',(199.175112338981,2.55868021301209,135.006706661894));
#207637=CARTESIAN_POINT('Ctrl Pts',(199.167622003219,2.67027728465172,134.936681889443));
#207638=CARTESIAN_POINT('Ctrl Pts',(199.160131667457,2.7787297750351,134.862419747228));
#207639=CARTESIAN_POINT('Ctrl Pts',(199.152357333338,2.89129427455412,134.78534193332));
#207640=CARTESIAN_POINT('Ctrl Pts',(199.144582999219,3.00082760257082,134.703454927598));
#207641=CARTESIAN_POINT('Ctrl Pts',(199.1368086651,3.10689139061681,134.617024902474));
#207642=CARTESIAN_POINT('Ctrl Pts',(199.129043912153,3.21282446452324,134.530701394631));
#207643=CARTESIAN_POINT('Ctrl Pts',(199.121279159206,3.31529620605177,134.439846252062));
#207644=CARTESIAN_POINT('Ctrl Pts',(199.113514406258,3.41389657407908,134.344769244263));
#207645=CARTESIAN_POINT('Ctrl Pts',(199.105757365373,3.51239901083084,134.249786668289));
#207646=CARTESIAN_POINT('Ctrl Pts',(199.098000324488,3.60703744639372,134.150590841398));
#207647=CARTESIAN_POINT('Ctrl Pts',(199.090243283603,3.69743462970616,134.047531939212));
#207648=CARTESIAN_POINT('Ctrl Pts',(199.082492092363,3.78776364379947,133.944550754547));
#207649=CARTESIAN_POINT('Ctrl Pts',(199.074740901123,3.87385751502113,133.837712585816));
#207650=CARTESIAN_POINT('Ctrl Pts',(199.066989709883,3.95537587695083,133.727404362455));
#207651=CARTESIAN_POINT('Ctrl Pts',(199.059241813106,4.03685959140212,133.617143023032));
#207652=CARTESIAN_POINT('Ctrl Pts',(199.051493916329,4.11377143257403,133.503414876139));
#207653=CARTESIAN_POINT('Ctrl Pts',(199.043746019552,4.18581151837598,133.386639648796));
#207654=CARTESIAN_POINT('Ctrl Pts',(199.035999743468,4.25783653494499,133.269888848313));
#207655=CARTESIAN_POINT('Ctrl Pts',(199.028253467384,4.32499161798016,133.150092567702));
#207656=CARTESIAN_POINT('Ctrl Pts',(199.020507191299,4.38702063536518,133.027698875092));
#207657=CARTESIAN_POINT('Ctrl Pts',(199.012760858034,4.44905011063427,132.905304279));
#207658=CARTESIAN_POINT('Ctrl Pts',(199.005014524769,4.50595326800805,132.780312581386));
#207659=CARTESIAN_POINT('Ctrl Pts',(198.997268191503,4.55752048674992,132.653195406117));
#207660=CARTESIAN_POINT('Ctrl Pts',(198.9895201235,4.60909925361287,132.526049763837));
#207661=CARTESIAN_POINT('Ctrl Pts',(198.981772055497,4.65533955709796,132.396778058965));
#207662=CARTESIAN_POINT('Ctrl Pts',(198.974023987494,4.6960805123652,132.265870413593));
#207663=CARTESIAN_POINT('Ctrl Pts',(198.966267684753,4.73686476760453,132.134823638018));
#207664=CARTESIAN_POINT('Ctrl Pts',(198.958511382011,4.77213788269821,132.002137822608));
#207665=CARTESIAN_POINT('Ctrl Pts',(198.950755079269,4.80178917923892,131.868317261722));
#207666=CARTESIAN_POINT('Ctrl Pts',(198.942994636755,4.8314563015694,131.734425276773));
#207667=CARTESIAN_POINT('Ctrl Pts',(198.935234194241,4.85549555803585,131.599397724268));
#207668=CARTESIAN_POINT('Ctrl Pts',(198.927473751726,4.87384789167415,131.463746537436));
#207669=CARTESIAN_POINT('Ctrl Pts',(198.919700851461,4.89222968610765,131.327877591277));
#207670=CARTESIAN_POINT('Ctrl Pts',(198.911927951196,4.90490627858033,131.191383399763));
#207671=CARTESIAN_POINT('Ctrl Pts',(198.90415505093,4.91187067501122,131.054779335846));
#207672=CARTESIAN_POINT('Ctrl Pts',(198.896664715168,4.91858189808959,130.923141173736));
#207673=CARTESIAN_POINT('Ctrl Pts',(198.889174379406,4.91998901695341,130.791401296814));
#207674=CARTESIAN_POINT('Ctrl Pts',(198.881684043644,4.91613139364612,130.660016643299));
#207675=CARTESIAN_POINT('Ctrl Pts',(198.873909709525,4.91212750737863,130.523650500714));
#207676=CARTESIAN_POINT('Ctrl Pts',(198.866135375406,4.90243908959812,130.387235082915));
#207677=CARTESIAN_POINT('Ctrl Pts',(198.858361041287,4.88705312982617,130.251283074398));
#207678=CARTESIAN_POINT('Ctrl Pts',(198.85059628834,4.87168613187456,130.115498614582));
#207679=CARTESIAN_POINT('Ctrl Pts',(198.842831535393,4.85063560658772,129.980176812465));
#207680=CARTESIAN_POINT('Ctrl Pts',(198.835066782445,4.82394053457245,129.845830085236));
#207681=CARTESIAN_POINT('Ctrl Pts',(198.82730974156,4.79727197647905,129.71161679307));
#207682=CARTESIAN_POINT('Ctrl Pts',(198.819552700675,4.7649701040377,129.578377029504));
#207683=CARTESIAN_POINT('Ctrl Pts',(198.81179565979,4.72712561650387,129.446617465017));
#207684=CARTESIAN_POINT('Ctrl Pts',(198.80404446855,4.68930966779249,129.314957261443));
#207685=CARTESIAN_POINT('Ctrl Pts',(198.79629327731,4.64595953098006,129.184775409413));
#207686=CARTESIAN_POINT('Ctrl Pts',(198.78854208607,4.59721676439492,129.056567413647));
#207687=CARTESIAN_POINT('Ctrl Pts',(198.780794189293,4.54849471478581,128.928413909699));
#207688=CARTESIAN_POINT('Ctrl Pts',(198.773046292516,4.49438473268614,128.802232958104));
#207689=CARTESIAN_POINT('Ctrl Pts',(198.765298395739,4.43507785272916,128.678503730866));
#207690=CARTESIAN_POINT('Ctrl Pts',(198.757552119655,4.37578337849294,128.554800385114));
#207691=CARTESIAN_POINT('Ctrl Pts',(198.749805843571,4.31129433754229,128.433548095968));
#207692=CARTESIAN_POINT('Ctrl Pts',(198.742059567486,4.24184925661964,128.315204546401));
#207693=CARTESIAN_POINT('Ctrl Pts',(198.734313234221,4.1724036630692,128.196860123249));
#207694=CARTESIAN_POINT('Ctrl Pts',(198.726566900956,4.0980021544152,128.081424819717));
#207695=CARTESIAN_POINT('Ctrl Pts',(198.71882056769,4.01892821604465,127.969329919887));
#207696=CARTESIAN_POINT('Ctrl Pts',(198.711072499687,3.93983656961388,127.857209917182));
#207697=CARTESIAN_POINT('Ctrl Pts',(198.703324431684,3.85607063665606,127.748432126146));
#207698=CARTESIAN_POINT('Ctrl Pts',(198.695576363682,3.76795580858273,127.643396826716));
#207699=CARTESIAN_POINT('Ctrl Pts',(198.68782006094,3.67974733102151,127.538249894519));
#207700=CARTESIAN_POINT('Ctrl Pts',(198.680063758198,3.58718097696145,127.436853699544));
#207701=CARTESIAN_POINT('Ctrl Pts',(198.672307455456,3.49062119914604,127.339573942088));
#207702=CARTESIAN_POINT('Ctrl Pts',(198.664547012942,3.39400988446978,127.242242263496));
#207703=CARTESIAN_POINT('Ctrl Pts',(198.656786570428,3.29340118567955,127.149031665843));
#207704=CARTESIAN_POINT('Ctrl Pts',(198.649026127913,3.1891938849692,127.060268547841));
#207705=CARTESIAN_POINT('Ctrl Pts',(198.641253227648,3.08481930144869,126.971362939403));
#207706=CARTESIAN_POINT('Ctrl Pts',(198.633480327383,2.97683488028589,126.886919318566));
#207707=CARTESIAN_POINT('Ctrl Pts',(198.625707427117,2.86567043886961,126.80722214132));
#207708=CARTESIAN_POINT('Ctrl Pts',(198.618217091355,2.7585471049054,126.730422157211));
#207709=CARTESIAN_POINT('Ctrl Pts',(198.610726755593,2.64847119750003,126.658029686858));
#207710=CARTESIAN_POINT('Ctrl Pts',(198.603236419831,2.53584842786697,126.590258600127));
#207711=CARTESIAN_POINT('Ctrl Pts',(198.595462085712,2.4189555316921,126.519917952044));
#207712=CARTESIAN_POINT('Ctrl Pts',(198.587687751593,2.29894855074917,126.454333226861));
#207713=CARTESIAN_POINT('Ctrl Pts',(198.579913417474,2.1762517885438,126.393792489154));
#207714=CARTESIAN_POINT('Ctrl Pts',(198.572148664527,2.05370623913212,126.333326362497));
#207715=CARTESIAN_POINT('Ctrl Pts',(198.56438391158,1.92847785139323,126.277892026139));
#207716=CARTESIAN_POINT('Ctrl Pts',(198.556619158633,1.80101880639067,126.227733658601));
#207717=CARTESIAN_POINT('Ctrl Pts',(198.548862117748,1.6736863555085,126.17762510906));
#207718=CARTESIAN_POINT('Ctrl Pts',(198.541105076863,1.54412801780239,126.132782242412));
#207719=CARTESIAN_POINT('Ctrl Pts',(198.533348035978,1.41281909465994,126.093402618574));
#207720=CARTESIAN_POINT('Ctrl Pts',(198.525596844738,1.2816091925979,126.054052691217));
#207721=CARTESIAN_POINT('Ctrl Pts',(198.517845653498,1.14865170571014,126.020157918166));
#207722=CARTESIAN_POINT('Ctrl Pts',(198.510094462257,1.01444003188544,125.991867034795));
#207723=CARTESIAN_POINT('Ctrl Pts',(198.50234656548,0.880285401602321,125.963588175804));
#207724=CARTESIAN_POINT('Ctrl Pts',(198.494598668703,0.744878026361152,
125.940908549741));
#207725=CARTESIAN_POINT('Ctrl Pts',(198.486850771926,0.608724306023622,
125.92392643793));
#207726=CARTESIAN_POINT('Ctrl Pts',(198.479104495842,0.472599066109263,
125.906947878411));
#207727=CARTESIAN_POINT('Ctrl Pts',(198.471358219758,0.335728179341729,
125.895664510952));
#207728=CARTESIAN_POINT('Ctrl Pts',(198.463611943674,0.198625636898631,
125.890123045077));
#207729=CARTESIAN_POINT('Ctrl Pts',(198.455865610409,0.061522082395698,
125.884581538295));
#207730=CARTESIAN_POINT('Ctrl Pts',(198.448119277143,-0.0758127405487922,
125.884782033463));
#207731=CARTESIAN_POINT('Ctrl Pts',(198.440372943878,-0.212862749645825,
125.890719145876));
#207732=CARTESIAN_POINT('Ctrl Pts',(198.432624875875,-0.349943450142099,
125.896657587864));
#207733=CARTESIAN_POINT('Ctrl Pts',(198.424876807872,-0.486738819347844,
125.908335186536));
#207734=CARTESIAN_POINT('Ctrl Pts',(198.417128739869,-0.622736208410933,
125.925694541964));
#207735=CARTESIAN_POINT('Ctrl Pts',(198.409372437127,-0.75887813711759,
125.943072347121));
#207736=CARTESIAN_POINT('Ctrl Pts',(198.401616134385,-0.894220003067948,
125.966143922283));
#207737=CARTESIAN_POINT('Ctrl Pts',(198.393859831644,-1.02825713663446,
125.994800312979));
#207738=CARTESIAN_POINT('Ctrl Pts',(198.386099389129,-1.16236580985501,
126.023471998453));
#207739=CARTESIAN_POINT('Ctrl Pts',(198.378338946615,-1.2951679847218,126.057734341305));
#207740=CARTESIAN_POINT('Ctrl Pts',(198.370578504101,-1.42617350123758,
126.097428261257));
#207741=CARTESIAN_POINT('Ctrl Pts',(198.362805603836,-1.55738931943859,
126.137185901413));
#207742=CARTESIAN_POINT('Ctrl Pts',(198.35503270357,-1.68680234652046,126.182392413503));
#207743=CARTESIAN_POINT('Ctrl Pts',(198.347259803305,-1.81394093480719,
126.232839935394));
#207744=CARTESIAN_POINT('Ctrl Pts',(198.339769467543,-1.93645771516747,
126.281453562794));
#207745=CARTESIAN_POINT('Ctrl Pts',(198.332279131781,-2.05686226744433,
126.334933642695));
#207746=CARTESIAN_POINT('Ctrl Pts',(198.324788796019,-2.17475536003933,
126.393054440652));
#207747=CARTESIAN_POINT('Ctrl Pts',(198.317013701679,-2.29713037045767,
126.453384805213));
#207748=CARTESIAN_POINT('Ctrl Pts',(198.309238607339,-2.41718687346733,
126.518906845975));
#207749=CARTESIAN_POINT('Ctrl Pts',(198.301463513,-2.53445302826001,126.589419228882));
#207750=CARTESIAN_POINT('Ctrl Pts',(198.293698169544,-2.65157211748876,
126.659843180958));
#207751=CARTESIAN_POINT('Ctrl Pts',(198.285932826088,-2.76590748987507,
126.735244822049));
#207752=CARTESIAN_POINT('Ctrl Pts',(198.278167482632,-2.87700919668973,
126.815375640825));
#207753=CARTESIAN_POINT('Ctrl Pts',(198.270116194762,-2.99220201841537,
126.89845712883));
#207754=CARTESIAN_POINT('Ctrl Pts',(198.262064906893,-3.10391807437486,
126.986622596305));
#207755=CARTESIAN_POINT('Ctrl Pts',(198.254013619023,-3.21168484940525,
127.079543374989));
#207756=CARTESIAN_POINT('Ctrl Pts',(198.246262861591,-3.31542901381586,
127.168995699587));
#207757=CARTESIAN_POINT('Ctrl Pts',(198.23851210416,-3.4155130831933,127.262854447875));
#207758=CARTESIAN_POINT('Ctrl Pts',(198.230761346728,-3.51154654453313,
127.360783418188));
#207759=CARTESIAN_POINT('Ctrl Pts',(198.223014065701,-3.60753693251182,
127.458668464957));
#207760=CARTESIAN_POINT('Ctrl Pts',(198.215266784674,-3.69948005432967,
127.560619822749));
#207761=CARTESIAN_POINT('Ctrl Pts',(198.207519503647,-3.78702100058199,
127.666263263491));
#207762=CARTESIAN_POINT('Ctrl Pts',(198.199774019722,-3.8745416403494,127.771882198593));
#207763=CARTESIAN_POINT('Ctrl Pts',(198.192028535798,-3.95766188812499,
127.881191211036));
#207764=CARTESIAN_POINT('Ctrl Pts',(198.184283051873,-4.036066276408,127.993782016114));
#207765=CARTESIAN_POINT('Ctrl Pts',(198.176537687326,-4.1144694562842,128.106371085887));
#207766=CARTESIAN_POINT('Ctrl Pts',(198.168792322778,-4.18815669953273,
128.222241525939));
#207767=CARTESIAN_POINT('Ctrl Pts',(198.161046958231,-4.25685536445191,
128.340955358857));
#207768=CARTESIAN_POINT('Ctrl Pts',(198.153297277113,-4.32559231583465,
128.459735352199));
#207769=CARTESIAN_POINT('Ctrl Pts',(198.145547595995,-4.38933494059853,
128.581361564616));
#207770=CARTESIAN_POINT('Ctrl Pts',(198.137797914878,-4.44785607756905,
128.705370532851));
#207771=CARTESIAN_POINT('Ctrl Pts',(198.130045641782,-4.50639678766299,
128.82942097743));
#207772=CARTESIAN_POINT('Ctrl Pts',(198.122293368687,-4.55971237526599,
128.955855407105));
#207773=CARTESIAN_POINT('Ctrl Pts',(198.114541095592,-4.60762386482984,
129.084190456579));
#207774=CARTESIAN_POINT('Ctrl Pts',(198.106781573825,-4.65558015346834,
129.212645504231));
#207775=CARTESIAN_POINT('Ctrl Pts',(198.099022052058,-4.69812213230576,
129.343004349367));
#207776=CARTESIAN_POINT('Ctrl Pts',(198.091262530291,-4.73512064756484,
129.474768381012));
#207777=CARTESIAN_POINT('Ctrl Pts',(198.089153878115,-4.74517500427239,
129.510575292887));
#207778=CARTESIAN_POINT('Ctrl Pts',(198.087045225939,-4.75482027712228,
129.546485914373));
#207779=CARTESIAN_POINT('Ctrl Pts',(198.084936573762,-4.76405452823404,
129.582490119308));
#207780=CARTESIAN_POINT('',(200.110140563961,-4.91824997595732,130.804846925942));
#207781=CARTESIAN_POINT('Ctrl Pts',(200.110140563961,-4.91824997595732,
130.804846925942));
#207782=CARTESIAN_POINT('Ctrl Pts',(200.101963209632,-4.91823561914748,
130.95004364306));
#207783=CARTESIAN_POINT('Ctrl Pts',(200.093785855304,-4.91178722962492,
131.095096221673));
#207784=CARTESIAN_POINT('Ctrl Pts',(200.085608500975,-4.8989686251045,131.239434717854));
#207785=CARTESIAN_POINT('Ctrl Pts',(200.077418065999,-4.88612951570811,
131.384004100554));
#207786=CARTESIAN_POINT('Ctrl Pts',(200.069227631024,-4.86689987818642,
131.527856800843));
#207787=CARTESIAN_POINT('Ctrl Pts',(200.061037196048,-4.84139484664338,
131.670431631626));
#207788=CARTESIAN_POINT('Ctrl Pts',(200.052825216095,-4.81582272399528,
131.81338150617));
#207789=CARTESIAN_POINT('Ctrl Pts',(200.044613236142,-4.78394225338721,
131.955046471638));
#207790=CARTESIAN_POINT('Ctrl Pts',(200.036401256189,-4.74591932059585,
132.094877128462));
#207791=CARTESIAN_POINT('Ctrl Pts',(200.028177613076,-4.70784238529188,
132.234906381402));
#207792=CARTESIAN_POINT('Ctrl Pts',(200.019953969963,-4.66360567060591,
132.373095819458));
#207793=CARTESIAN_POINT('Ctrl Pts',(200.01173032685,-4.61342381118858,132.508914459737));
#207794=CARTESIAN_POINT('Ctrl Pts',(200.003487519808,-4.56312501070649,
132.645049604358));
#207795=CARTESIAN_POINT('Ctrl Pts',(199.995244712766,-4.50685348823889,
132.778802607651));
#207796=CARTESIAN_POINT('Ctrl Pts',(199.987001905724,-4.4448713186341,132.90966392666));
#207797=CARTESIAN_POINT('Ctrl Pts',(199.983296451395,-4.41700798305935,
132.96849105176));
#207798=CARTESIAN_POINT('Ctrl Pts',(199.979590997066,-4.38799121645204,
133.026734176052));
#207799=CARTESIAN_POINT('Ctrl Pts',(199.975885542737,-4.35784769754507,
133.084348886725));
#207800=CARTESIAN_POINT('Ctrl Pts',(199.968111208618,-4.29460422813576,
133.205229073381));
#207801=CARTESIAN_POINT('Ctrl Pts',(199.960336874499,-4.22622722019875,
133.3236673123));
#207802=CARTESIAN_POINT('Ctrl Pts',(199.95256254038,-4.15292920796671,133.43919686601));
#207803=CARTESIAN_POINT('Ctrl Pts',(199.944797787433,-4.07972152898389,
133.554584039872));
#207804=CARTESIAN_POINT('Ctrl Pts',(199.937033034486,-4.00160512008709,
133.667069334041));
#207805=CARTESIAN_POINT('Ctrl Pts',(199.929268281538,-3.91883915315159,
133.776208990923));
#207806=CARTESIAN_POINT('Ctrl Pts',(199.921511240653,-3.83615539054131,
133.88524024876));
#207807=CARTESIAN_POINT('Ctrl Pts',(199.913754199768,-3.74883149464554,
133.990932172596));
#207808=CARTESIAN_POINT('Ctrl Pts',(199.905997158883,-3.65717063344393,
134.092868793073));
#207809=CARTESIAN_POINT('Ctrl Pts',(199.898245967643,-3.56557889441098,
134.194728542351));
#207810=CARTESIAN_POINT('Ctrl Pts',(199.890494776403,-3.46965696023711,
134.292838335461));
#207811=CARTESIAN_POINT('Ctrl Pts',(199.882743585163,-3.36974885186079,
134.386814488572));
#207812=CARTESIAN_POINT('Ctrl Pts',(199.874995688386,-3.26988320709536,
134.48075069931));
#207813=CARTESIAN_POINT('Ctrl Pts',(199.867247791609,-3.16603504200538,
134.570556497095));
#207814=CARTESIAN_POINT('Ctrl Pts',(199.859499894832,-3.05858572710474,
134.655884525378));
#207815=CARTESIAN_POINT('Ctrl Pts',(199.851753618747,-2.95115888828444,
134.741194704878));
#207816=CARTESIAN_POINT('Ctrl Pts',(199.844007342663,-2.84013270394872,
134.822028734951));
#207817=CARTESIAN_POINT('Ctrl Pts',(199.836261066579,-2.72592185460808,
134.89807935547));
#207818=CARTESIAN_POINT('Ctrl Pts',(199.828514733314,-2.61171016218902,
134.974130537379));
#207819=CARTESIAN_POINT('Ctrl Pts',(199.820768400049,-2.49431408327654,
135.045398022584));
#207820=CARTESIAN_POINT('Ctrl Pts',(199.813022066783,-2.37417718264307,
135.111617954656));
#207821=CARTESIAN_POINT('Ctrl Pts',(199.80527399878,-2.25401337818375,135.177852716222));
#207822=CARTESIAN_POINT('Ctrl Pts',(199.797525930777,-2.13110787296654,
135.239037486666));
#207823=CARTESIAN_POINT('Ctrl Pts',(199.789777862774,-2.00592835665058,
135.294954619531));
#207824=CARTESIAN_POINT('Ctrl Pts',(199.782021560032,-1.88061579805486,
135.35093118179));
#207825=CARTESIAN_POINT('Ctrl Pts',(199.77426525729,-1.75302475798892,135.401628763137));
#207826=CARTESIAN_POINT('Ctrl Pts',(199.766508954549,-1.623642929,135.446877898267));
#207827=CARTESIAN_POINT('Ctrl Pts',(199.758748512034,-1.49419204503319,
135.492151184223));
#207828=CARTESIAN_POINT('Ctrl Pts',(199.75098806952,-1.362948841577,135.531970116074));
#207829=CARTESIAN_POINT('Ctrl Pts',(199.743227627006,-1.23041469352731,
135.566215586426));
#207830=CARTESIAN_POINT('Ctrl Pts',(199.73545472674,-1.09766778989741,135.600516030646));
#207831=CARTESIAN_POINT('Ctrl Pts',(199.727681826475,-0.96362618299564,
135.629225052453));
#207832=CARTESIAN_POINT('Ctrl Pts',(199.71990892621,-0.828800812444949,
135.65227483667));
#207833=CARTESIAN_POINT('Ctrl Pts',(199.712418590448,-0.698876683722678,
135.674486703171));
#207834=CARTESIAN_POINT('Ctrl Pts',(199.704928254686,-0.568225091055471,
135.691443604055));
#207835=CARTESIAN_POINT('Ctrl Pts',(199.697437918924,-0.437304423404299,
135.703130657461));
#207836=CARTESIAN_POINT('Ctrl Pts',(199.689663584805,-0.301419858842875,
135.715260829049));
#207837=CARTESIAN_POINT('Ctrl Pts',(199.681889250686,-0.164814971104963,
135.721752076884));
#207838=CARTESIAN_POINT('Ctrl Pts',(199.674114916567,-0.0279973195866715,
135.722530929033));
#207839=CARTESIAN_POINT('Ctrl Pts',(199.66635016362,0.10865171640381,135.723308821316));
#207840=CARTESIAN_POINT('Ctrl Pts',(199.658585410673,0.245512607244556,
135.718388323244));
#207841=CARTESIAN_POINT('Ctrl Pts',(199.650820657726,0.382071918374638,
135.707747621637));
#207842=CARTESIAN_POINT('Ctrl Pts',(199.643063616841,0.518495596871722,
135.697117488524));
#207843=CARTESIAN_POINT('Ctrl Pts',(199.635306575956,0.654617904481336,
135.680778488268));
#207844=CARTESIAN_POINT('Ctrl Pts',(199.627549535071,0.789925004703764,
135.658760843077));
#207845=CARTESIAN_POINT('Ctrl Pts',(199.619798343831,0.925130068789412,
135.636759801564));
#207846=CARTESIAN_POINT('Ctrl Pts',(199.612047152591,1.05952076479068,135.609088701334));
#207847=CARTESIAN_POINT('Ctrl Pts',(199.604295961351,1.19258833691385,135.575829586464));
#207848=CARTESIAN_POINT('Ctrl Pts',(199.596548064574,1.32559935176917,135.542584607605));
#207849=CARTESIAN_POINT('Ctrl Pts',(199.588800167797,1.45728798274033,135.503756432513));
#207850=CARTESIAN_POINT('Ctrl Pts',(199.581052271019,1.58715584884965,135.459478164306));
#207851=CARTESIAN_POINT('Ctrl Pts',(199.573305994935,1.71699654940101,135.415209158157));
#207852=CARTESIAN_POINT('Ctrl Pts',(199.565559718851,1.84501687283777,135.365492452586));
#207853=CARTESIAN_POINT('Ctrl Pts',(199.557813442767,1.97073416756975,135.310510848447));
#207854=CARTESIAN_POINT('Ctrl Pts',(199.550067109502,2.09645239031821,135.255528838447));
#207855=CARTESIAN_POINT('Ctrl Pts',(199.542320776237,2.21986719223249,135.195282008988));
#207856=CARTESIAN_POINT('Ctrl Pts',(199.534574442971,2.34051682582934,135.130000922828));
#207857=CARTESIAN_POINT('Ctrl Pts',(199.526826374968,2.46119347807506,135.064705217422));
#207858=CARTESIAN_POINT('Ctrl Pts',(199.519078306965,2.57910338599568,134.994373197965));
#207859=CARTESIAN_POINT('Ctrl Pts',(199.511330238962,2.6938106397786,134.919280701786));
#207860=CARTESIAN_POINT('Ctrl Pts',(199.503573936221,2.80863980579594,134.844108396408));
#207861=CARTESIAN_POINT('Ctrl Pts',(199.495817633479,2.92025919055272,134.764165721911));
#207862=CARTESIAN_POINT('Ctrl Pts',(199.488061330737,3.02826260835506,134.679771387709));
#207863=CARTESIAN_POINT('Ctrl Pts',(199.480300888223,3.13632367083349,134.595332009709));
#207864=CARTESIAN_POINT('Ctrl Pts',(199.472540445709,3.24076462319159,134.506436490939));
#207865=CARTESIAN_POINT('Ctrl Pts',(199.464780003195,3.34121425162771,134.41344227184));
#207866=CARTESIAN_POINT('Ctrl Pts',(199.457007102929,3.44182513072487,134.320298770166));
#207867=CARTESIAN_POINT('Ctrl Pts',(199.449234202664,3.53843160653162,134.223043697568));
#207868=CARTESIAN_POINT('Ctrl Pts',(199.441461302398,3.63070044887218,134.122070266263));
#207869=CARTESIAN_POINT('Ctrl Pts',(199.433970966636,3.71961508638472,134.024767473521));
#207870=CARTESIAN_POINT('Ctrl Pts',(199.426480630874,3.8045017845271,133.924012207482));
#207871=CARTESIAN_POINT('Ctrl Pts',(199.418990295112,3.88510025233675,133.820182079754));
#207872=CARTESIAN_POINT('Ctrl Pts',(199.411215960993,3.96875463554883,133.712415201177));
#207873=CARTESIAN_POINT('Ctrl Pts',(199.403441626874,4.04805418477677,133.600994318284));
#207874=CARTESIAN_POINT('Ctrl Pts',(199.395667292754,4.12266273775037,133.486306741795));
#207875=CARTESIAN_POINT('Ctrl Pts',(199.387902539807,4.19717934235037,133.371760507494));
#207876=CARTESIAN_POINT('Ctrl Pts',(199.38013778686,4.26701624247923,133.253955914529));
#207877=CARTESIAN_POINT('Ctrl Pts',(199.372373033913,4.33187756216918,133.133313139382));
#207878=CARTESIAN_POINT('Ctrl Pts',(199.364615993028,4.39667446068206,133.01279018834));
#207879=CARTESIAN_POINT('Ctrl Pts',(199.356858952143,4.45650542925731,132.889435007023));
#207880=CARTESIAN_POINT('Ctrl Pts',(199.349101911258,4.51111815351607,132.763696236473));
#207881=CARTESIAN_POINT('Ctrl Pts',(199.341350720018,4.56568969389464,132.638052286508));
#207882=CARTESIAN_POINT('Ctrl Pts',(199.333599528778,4.61505066744896,132.510028682241));
#207883=CARTESIAN_POINT('Ctrl Pts',(199.325848337538,4.65899510525039,132.380097801158));
#207884=CARTESIAN_POINT('Ctrl Pts',(199.318100440761,4.7029208654935,132.250222144165));
#207885=CARTESIAN_POINT('Ctrl Pts',(199.310352543983,4.74143454383123,132.118441192244));
#207886=CARTESIAN_POINT('Ctrl Pts',(199.302604647206,4.77437873659335,131.985246192914));
#207887=CARTESIAN_POINT('Ctrl Pts',(199.294858371122,4.80731603814052,131.852079055106));
#207888=CARTESIAN_POINT('Ctrl Pts',(199.287112095038,4.83468607758103,131.717498837516));
#207889=CARTESIAN_POINT('Ctrl Pts',(199.279365818954,4.85638176547755,131.582010416921));
#207890=CARTESIAN_POINT('Ctrl Pts',(199.271619485689,4.8780776135267,131.446520996182));
#207891=CARTESIAN_POINT('Ctrl Pts',(199.263873152423,4.89409896463232,131.310123745109));
#207892=CARTESIAN_POINT('Ctrl Pts',(199.256126819158,4.9043902119798,131.17333176974));
#207893=CARTESIAN_POINT('Ctrl Pts',(199.248378751155,4.91468376398078,131.036509160757));
#207894=CARTESIAN_POINT('Ctrl Pts',(199.240630683152,4.91924462944542,130.899292041369));
#207895=CARTESIAN_POINT('Ctrl Pts',(199.232882615149,4.91806925823009,130.762196251662));
#207896=CARTESIAN_POINT('Ctrl Pts',(199.225126312407,4.91689263781624,130.624954754918));
#207897=CARTESIAN_POINT('Ctrl Pts',(199.217370009665,4.90996760558296,130.487835237022));
#207898=CARTESIAN_POINT('Ctrl Pts',(199.209613706923,4.8973427474991,130.351351703727));
#207899=CARTESIAN_POINT('Ctrl Pts',(199.201853264409,4.88471115114836,130.21479532506));
#207900=CARTESIAN_POINT('Ctrl Pts',(199.194092821895,4.86637371941593,130.07887599463));
#207901=CARTESIAN_POINT('Ctrl Pts',(199.186332379381,4.8424305269433,129.944099230412));
#207902=CARTESIAN_POINT('Ctrl Pts',(199.178559479115,4.81844889873255,129.809106110568));
#207903=CARTESIAN_POINT('Ctrl Pts',(199.17078657885,4.788843611667,129.675259604108));
#207904=CARTESIAN_POINT('Ctrl Pts',(199.163013678584,4.75376536727037,129.543052607823));
#207905=CARTESIAN_POINT('Ctrl Pts',(199.155523342822,4.71996230541452,129.415651668864));
#207906=CARTESIAN_POINT('Ctrl Pts',(199.14803300706,4.68107738037903,129.289773403227));
#207907=CARTESIAN_POINT('Ctrl Pts',(199.140542671298,4.63728759387846,129.165840909366));
#207908=CARTESIAN_POINT('Ctrl Pts',(199.132768337179,4.59183750431285,129.037209477331));
#207909=CARTESIAN_POINT('Ctrl Pts',(199.12499400306,4.54095930328843,128.910266811875));
#207910=CARTESIAN_POINT('Ctrl Pts',(199.117219668941,4.48479714236479,128.785505086742));
#207911=CARTESIAN_POINT('Ctrl Pts',(199.109454915994,4.42870419628514,128.660897119286));
#207912=CARTESIAN_POINT('Ctrl Pts',(199.101690163047,4.36734040620565,128.538465097289));
#207913=CARTESIAN_POINT('Ctrl Pts',(199.0939254101,4.30089935031177,128.418685065235));
#207914=CARTESIAN_POINT('Ctrl Pts',(199.086168369215,4.23452428461125,128.299024000398));
#207915=CARTESIAN_POINT('Ctrl Pts',(199.07841132833,4.16308217693648,128.182010023415));
#207916=CARTESIAN_POINT('Ctrl Pts',(199.070654287445,4.08681409961739,128.068097914961));
#207917=CARTESIAN_POINT('Ctrl Pts',(199.062903096205,4.01060353664873,127.954271708514));
#207918=CARTESIAN_POINT('Ctrl Pts',(199.055151904965,3.92957446447712,127.84354303823));
#207919=CARTESIAN_POINT('Ctrl Pts',(199.047400713724,3.84401297642226,127.736340523173));
#207920=CARTESIAN_POINT('Ctrl Pts',(199.039652816947,3.75848785428223,127.629183572045));
#207921=CARTESIAN_POINT('Ctrl Pts',(199.03190492017,3.66843439109177,127.525550100254));
#207922=CARTESIAN_POINT('Ctrl Pts',(199.024157023393,3.57418080677142,127.425838067248));
#207923=CARTESIAN_POINT('Ctrl Pts',(199.016410747309,3.47994693826904,127.32614689185));
#207924=CARTESIAN_POINT('Ctrl Pts',(199.008664471225,3.38151496456809,127.230375807597));
#207925=CARTESIAN_POINT('Ctrl Pts',(199.000918195141,3.27925176834539,127.138887810096));
#207926=CARTESIAN_POINT('Ctrl Pts',(198.993171861876,3.17698781723904,127.047399137251));
#207927=CARTESIAN_POINT('Ctrl Pts',(198.98542552861,3.07089287855635,126.960193874925));
#207928=CARTESIAN_POINT('Ctrl Pts',(198.977679195345,2.96136858609743,126.877596153051));
#207929=CARTESIAN_POINT('Ctrl Pts',(198.969931127342,2.85181976643257,126.794979933991));
#207930=CARTESIAN_POINT('Ctrl Pts',(198.962183059339,2.73884037688976,126.716973543961));
#207931=CARTESIAN_POINT('Ctrl Pts',(198.954434991336,2.62286248940288,126.643858793965));
#207932=CARTESIAN_POINT('Ctrl Pts',(198.946678688594,2.50676133923701,126.570666336743));
#207933=CARTESIAN_POINT('Ctrl Pts',(198.938922385852,2.38765565632938,126.502376113735));
#207934=CARTESIAN_POINT('Ctrl Pts',(198.931166083111,2.26600415017978,126.439225080854));
#207935=CARTESIAN_POINT('Ctrl Pts',(198.923405640596,2.14428771495838,126.376040342365));
#207936=CARTESIAN_POINT('Ctrl Pts',(198.915645198082,2.02002310306419,126.318000424913));
#207937=CARTESIAN_POINT('Ctrl Pts',(198.907884755568,1.8936897138752,126.265294377681));
#207938=CARTESIAN_POINT('Ctrl Pts',(198.900111855303,1.76715352311459,126.212503722024));
#207939=CARTESIAN_POINT('Ctrl Pts',(198.892338955037,1.63854228569136,126.165064182373));
#207940=CARTESIAN_POINT('Ctrl Pts',(198.884566054772,1.50835214749063,126.123115392024));
#207941=CARTESIAN_POINT('Ctrl Pts',(198.87707571901,1.38289474874265,126.082691545867));
#207942=CARTESIAN_POINT('Ctrl Pts',(198.869585383248,1.25597154700458,126.047366257253));
#207943=CARTESIAN_POINT('Ctrl Pts',(198.862095047486,1.12803418073941,126.017219304675));
#207944=CARTESIAN_POINT('Ctrl Pts',(198.854320713367,0.995246030346574,
125.985929321228));
#207945=CARTESIAN_POINT('Ctrl Pts',(198.846546379248,0.860944660272916,
125.96011898127));
#207946=CARTESIAN_POINT('Ctrl Pts',(198.838772045129,0.72562206766675,125.939933037941));
#207947=CARTESIAN_POINT('Ctrl Pts',(198.831007292181,0.590466248061855,
125.919771971984));
#207948=CARTESIAN_POINT('Ctrl Pts',(198.823242539234,0.454292093069238,
125.905221568033));
#207949=CARTESIAN_POINT('Ctrl Pts',(198.815477786287,0.317604746131932,
125.89637627695));
#207950=CARTESIAN_POINT('Ctrl Pts',(198.807720745402,0.181053158994685,
125.887539771135));
#207951=CARTESIAN_POINT('Ctrl Pts',(198.799963704517,0.0439897818821281,
125.884397126882));
#207952=CARTESIAN_POINT('Ctrl Pts',(198.792206663632,-0.0930724598611862,
125.886991343278));
#207953=CARTESIAN_POINT('Ctrl Pts',(198.784455472392,-0.230031341901755,
125.889583603354));
#207954=CARTESIAN_POINT('Ctrl Pts',(198.776704281152,-0.366988700963738,
125.897904105649));
#207955=CARTESIAN_POINT('Ctrl Pts',(198.768953089912,-0.503429287263447,
125.911943830821));
#207956=CARTESIAN_POINT('Ctrl Pts',(198.761205193135,-0.639811882674504,
125.925977588736));
#207957=CARTESIAN_POINT('Ctrl Pts',(198.753457296358,-0.775677754077462,
125.945725694873));
#207958=CARTESIAN_POINT('Ctrl Pts',(198.745709399581,-0.910514676033535,
125.971127115321));
#207959=CARTESIAN_POINT('Ctrl Pts',(198.737963123496,-1.04532339301227,
125.996523222339));
#207960=CARTESIAN_POINT('Ctrl Pts',(198.730216847412,-1.17910320469284,
126.027570219174));
#207961=CARTESIAN_POINT('Ctrl Pts',(198.722470571328,-1.31135040354105,
126.064155645032));
#207962=CARTESIAN_POINT('Ctrl Pts',(198.714724238063,-1.44359857860805,
126.100741340956));
#207963=CARTESIAN_POINT('Ctrl Pts',(198.706977904797,-1.57431374145571,
126.14286544324));
#207964=CARTESIAN_POINT('Ctrl Pts',(198.699231571532,-1.70300609951057,
126.190365246141));
#207965=CARTESIAN_POINT('Ctrl Pts',(198.691483503529,-1.83172727732661,
126.237875686293));
#207966=CARTESIAN_POINT('Ctrl Pts',(198.683735435526,-1.95842438223704,
126.290764087235));
#207967=CARTESIAN_POINT('Ctrl Pts',(198.675987367523,-2.08262677322981,
126.348819260343));
#207968=CARTESIAN_POINT('Ctrl Pts',(198.668231064781,-2.20696116800184,
126.406936135179));
#207969=CARTESIAN_POINT('Ctrl Pts',(198.660474762039,-2.32879519762787,
126.47023058584));
#207970=CARTESIAN_POINT('Ctrl Pts',(198.652718459298,-2.44768156069828,
126.538444767491));
#207971=CARTESIAN_POINT('Ctrl Pts',(198.644958016783,-2.56663137700036,
126.606695357105));
#207972=CARTESIAN_POINT('Ctrl Pts',(198.637197574269,-2.68263006138942,
126.679870701362));
#207973=CARTESIAN_POINT('Ctrl Pts',(198.629437131755,-2.79525943435933,
126.757669653689));
#207974=CARTESIAN_POINT('Ctrl Pts',(198.62166423149,-2.90806960999747,126.835593495801));
#207975=CARTESIAN_POINT('Ctrl Pts',(198.613891331224,-3.01749935359477,
126.918155542348));
#207976=CARTESIAN_POINT('Ctrl Pts',(198.606118430959,-3.12316300873507,
127.005013846953));
#207977=CARTESIAN_POINT('Ctrl Pts',(198.598628095197,-3.22498552385993,
127.088714633402));
#207978=CARTESIAN_POINT('Ctrl Pts',(198.591137759435,-3.32331078044587,
127.176404536312));
#207979=CARTESIAN_POINT('Ctrl Pts',(198.583647423673,-3.41782753696518,
127.267746701677));
#207980=CARTESIAN_POINT('Ctrl Pts',(198.575987342496,-3.51448622497807,
127.361158856193));
#207981=CARTESIAN_POINT('Ctrl Pts',(198.568327261318,-3.60748705227816,
127.458705550652));
#207982=CARTESIAN_POINT('Ctrl Pts',(198.560667180141,-3.69644762254403,
127.560064386287));
#207983=CARTESIAN_POINT('Ctrl Pts',(198.553016015211,-3.78530464372584,
127.6613052414));
#207984=CARTESIAN_POINT('Ctrl Pts',(198.545364850281,-3.87013049362145,
127.766349116946));
#207985=CARTESIAN_POINT('Ctrl Pts',(198.53771368535,-3.95057739062617,127.874834829461));
#207986=CARTESIAN_POINT('Ctrl Pts',(198.530069653823,-4.03094928465215,
127.983219397595));
#207987=CARTESIAN_POINT('Ctrl Pts',(198.522425622296,-4.10695010528644,
128.095039100229));
#207988=CARTESIAN_POINT('Ctrl Pts',(198.514781590769,-4.17827075473654,
128.209897944369));
#207989=CARTESIAN_POINT('Ctrl Pts',(198.507143088631,-4.24953981365601,
128.324673704173));
#207990=CARTESIAN_POINT('Ctrl Pts',(198.499504586494,-4.31613522474468,
128.442483890537));
#207991=CARTESIAN_POINT('Ctrl Pts',(198.491866084356,-4.37779019060595,
128.562902139357));
#207992=CARTESIAN_POINT('Ctrl Pts',(198.484230874548,-4.43941858208351,
128.683268485777));
#207993=CARTESIAN_POINT('Ctrl Pts',(198.47659566474,-4.49611058101027,128.806240300078));
#207994=CARTESIAN_POINT('Ctrl Pts',(198.468960454932,-4.54764472612785,
128.931365554192));
#207995=CARTESIAN_POINT('Ctrl Pts',(198.461325447542,-4.5991775050181,129.056487491098));
#207996=CARTESIAN_POINT('Ctrl Pts',(198.453690440153,-4.64555254017037,
129.183762384902));
#207997=CARTESIAN_POINT('Ctrl Pts',(198.446055432763,-4.68659615849717,
129.312717392911));
#207998=CARTESIAN_POINT('Ctrl Pts',(198.440775680082,-4.71497860042732,
129.401892231183));
#207999=CARTESIAN_POINT('Ctrl Pts',(198.435495927401,-4.74081256549775,
129.491870059345));
#208000=CARTESIAN_POINT('Ctrl Pts',(198.430216174721,-4.76405452823404,
129.582490119308));
#208001=CARTESIAN_POINT('Ctrl Pts',(200.179870531952,-4.76405452823405,
129.582490119308));
#208002=CARTESIAN_POINT('Ctrl Pts',(200.171798423708,-4.79949019568666,
129.720653248895));
#208003=CARTESIAN_POINT('Ctrl Pts',(200.163726315465,-4.8289461026174,129.860494510444));
#208004=CARTESIAN_POINT('Ctrl Pts',(200.155654207222,-4.85227401211597,
130.001478326166));
#208005=CARTESIAN_POINT('Ctrl Pts',(200.147594415967,-4.87556632625476,
130.142247018897));
#208006=CARTESIAN_POINT('Ctrl Pts',(200.139534624712,-4.89274923115088,
130.284154452949));
#208007=CARTESIAN_POINT('Ctrl Pts',(200.131474833457,-4.90372514985256,
130.426653433092));
#208008=CARTESIAN_POINT('Ctrl Pts',(200.124363410307,-4.91340956969396,
130.552385045013));
#208009=CARTESIAN_POINT('Ctrl Pts',(200.117251987158,-4.91826246131281,
130.678576831645));
#208010=CARTESIAN_POINT('Ctrl Pts',(200.110140564008,-4.9182499759574,130.804846925109));
#208011=CARTESIAN_POINT('Origin',(213.235140564004,0.,130.804360617566));
#208012=CARTESIAN_POINT('',(201.930097584127,-4.76405452823404,129.582490119308));
#208013=CARTESIAN_POINT('',(201.584606355351,-4.76405452823405,129.582490119308));
#208014=CARTESIAN_POINT('',(213.235140564004,-4.76405452823405,129.582490119308));
#208015=CARTESIAN_POINT('',(201.51485943594,-4.91824986053202,130.805531888988));
#208016=CARTESIAN_POINT('Ctrl Pts',(201.584606355351,-4.76405452823405,
129.582490119308));
#208017=CARTESIAN_POINT('Ctrl Pts',(201.576612163084,-4.79917136563237,
129.719410135352));
#208018=CARTESIAN_POINT('Ctrl Pts',(201.568617970816,-4.82841256673479,
129.857966876512));
#208019=CARTESIAN_POINT('Ctrl Pts',(201.560623778548,-4.85163618075089,
129.997633010422));
#208020=CARTESIAN_POINT('Ctrl Pts',(201.55263857145,-4.87483369230245,130.137142164875));
#208021=CARTESIAN_POINT('Ctrl Pts',(201.544653364352,-4.89202704125614,
130.277757877198));
#208022=CARTESIAN_POINT('Ctrl Pts',(201.536668157254,-4.90312503397178,
130.418941412363));
#208023=CARTESIAN_POINT('Ctrl Pts',(201.5293985835,-4.91322842585438,130.547472095315));
#208024=CARTESIAN_POINT('Ctrl Pts',(201.522129009746,-4.9182805956174,130.676473036305));
#208025=CARTESIAN_POINT('Ctrl Pts',(201.514859435991,-4.91824986053224,
130.805531888085));
#208026=CARTESIAN_POINT('Ctrl Pts',(201.51485943594,-4.91824986053202,130.805531888988));
#208027=CARTESIAN_POINT('Ctrl Pts',(201.506582193965,-4.9182148650919,130.952480167015));
#208028=CARTESIAN_POINT('Ctrl Pts',(201.49830495199,-4.91158982122124,131.099253060515));
#208029=CARTESIAN_POINT('Ctrl Pts',(201.490027710014,-4.89844708438231,
131.245267891272));
#208030=CARTESIAN_POINT('Ctrl Pts',(201.481501455677,-4.88490896174189,
131.395675428935));
#208031=CARTESIAN_POINT('Ctrl Pts',(201.472975201339,-4.86445493793769,
131.545278220582));
#208032=CARTESIAN_POINT('Ctrl Pts',(201.464448947001,-4.83721994611014,
131.693453557283));
#208033=CARTESIAN_POINT('Ctrl Pts',(201.456128501245,-4.81064235843921,
131.838052205476));
#208034=CARTESIAN_POINT('Ctrl Pts',(201.447808055489,-4.77760755788874,
131.981291262248));
#208035=CARTESIAN_POINT('Ctrl Pts',(201.439487609733,-4.73829111258486,
132.122609605769));
#208036=CARTESIAN_POINT('Ctrl Pts',(201.430858451104,-4.69751591217013,
132.269171273154));
#208037=CARTESIAN_POINT('Ctrl Pts',(201.422229292475,-4.6499841405859,132.413666610456));
#208038=CARTESIAN_POINT('Ctrl Pts',(201.413600133847,-4.59594544262833,
132.555494122152));
#208039=CARTESIAN_POINT('Ctrl Pts',(201.404970975218,-4.54190674467076,
132.697321633848));
#208040=CARTESIAN_POINT('Ctrl Pts',(201.396341816589,-4.48136133127772,
132.836481025787));
#208041=CARTESIAN_POINT('Ctrl Pts',(201.38771265796,-4.41461067614117,132.972400202214));
#208042=CARTESIAN_POINT('Ctrl Pts',(201.379938323841,-4.3544724960429,133.094854909123));
#208043=CARTESIAN_POINT('Ctrl Pts',(201.372163989722,-4.28914013406402,
133.21499946427));
#208044=CARTESIAN_POINT('Ctrl Pts',(201.364389655603,-4.21881414473507,
133.332361858603));
#208045=CARTESIAN_POINT('Ctrl Pts',(201.356624902656,-4.14857482590277,
133.449579614273));
#208046=CARTESIAN_POINT('Ctrl Pts',(201.348860149708,-4.07335432377154,
133.564021699203));
#208047=CARTESIAN_POINT('Ctrl Pts',(201.341095396761,-3.9934004017413,133.675237886603));
#208048=CARTESIAN_POINT('Ctrl Pts',(201.333338355876,-3.91352589107348,
133.786343612518));
#208049=CARTESIAN_POINT('Ctrl Pts',(201.325581314991,-3.8289275430417,133.89422950163));
#208050=CARTESIAN_POINT('Ctrl Pts',(201.317824274106,-3.73989781193985,
133.998471983619));
#208051=CARTESIAN_POINT('Ctrl Pts',(201.310073082865,-3.65093521885079,
134.102635855541));
#208052=CARTESIAN_POINT('Ctrl Pts',(201.302321891625,-3.55754814710466,
134.203161493023));
#208053=CARTESIAN_POINT('Ctrl Pts',(201.294570700385,-3.46007071453197,
134.299656558247));
#208054=CARTESIAN_POINT('Ctrl Pts',(201.286822803607,-3.36263471246837,
134.396110610494));
#208055=CARTESIAN_POINT('Ctrl Pts',(201.27907490683,-3.26111208461592,134.488537223235));
#208056=CARTESIAN_POINT('Ctrl Pts',(201.271327010053,-3.15587521323921,
134.576579420998));
#208057=CARTESIAN_POINT('Ctrl Pts',(201.263580733969,-3.05066035514734,
134.664603202231));
#208058=CARTESIAN_POINT('Ctrl Pts',(201.255834457884,-2.94173309858087,
134.748244141987));
#208059=CARTESIAN_POINT('Ctrl Pts',(201.2480881818,-2.82950014815832,134.827184498134));
#208060=CARTESIAN_POINT('Ctrl Pts',(201.240341848535,-2.71726636925778,
134.906125437001));
#208061=CARTESIAN_POINT('Ctrl Pts',(201.232595515269,-2.60172716759431,
134.980365498095));
#208062=CARTESIAN_POINT('Ctrl Pts',(201.224849182004,-2.48331923024386,
135.049629591754));
#208063=CARTESIAN_POINT('Ctrl Pts',(201.217101114,-2.36488477625662,135.118909196626));
#208064=CARTESIAN_POINT('Ctrl Pts',(201.209353045997,-2.24358064561767,
135.183210419302));
#208065=CARTESIAN_POINT('Ctrl Pts',(201.201604977994,-2.11986882164754,
135.242303749413));
#208066=CARTESIAN_POINT('Ctrl Pts',(201.193848675252,-1.99602551527869,
135.301459884618));
#208067=CARTESIAN_POINT('Ctrl Pts',(201.18609237251,-1.8697697571969,135.355396901697));
#208068=CARTESIAN_POINT('Ctrl Pts',(201.178336069768,-1.74158475661268,
135.403932945298));
#208069=CARTESIAN_POINT('Ctrl Pts',(201.170575627254,-1.61333133983404,
135.452494894046));
#208070=CARTESIAN_POINT('Ctrl Pts',(201.162815184739,-1.4831469997239,135.49565000241));
#208071=CARTESIAN_POINT('Ctrl Pts',(201.155054742225,-1.35152990844939,
135.533266407394));
#208072=CARTESIAN_POINT('Ctrl Pts',(201.147281841959,-1.21970153373557,
135.57094319757));
#208073=CARTESIAN_POINT('Ctrl Pts',(201.139508941694,-1.08643619206553,
135.603063425218));
#208074=CARTESIAN_POINT('Ctrl Pts',(201.131736041428,-0.952242926124562,
135.629546258777));
#208075=CARTESIAN_POINT('Ctrl Pts',(201.124245705668,-0.822927923447469,
135.655066374622));
#208076=CARTESIAN_POINT('Ctrl Pts',(201.116755369908,-0.692751594327094,
135.675351800014));
#208077=CARTESIAN_POINT('Ctrl Pts',(201.109265034147,-0.562171798684125,
135.690375960488));
#208078=CARTESIAN_POINT('Ctrl Pts',(201.101490700028,-0.426641030368497,
135.705969766576));
#208079=CARTESIAN_POINT('Ctrl Pts',(201.093716365909,-0.290246275975597,
135.715944866885));
#208080=CARTESIAN_POINT('Ctrl Pts',(201.08594203179,-0.153493054712102,
135.7202148612));
#208081=CARTESIAN_POINT('Ctrl Pts',(201.078177278843,-0.0169083695718419,
135.724479593129));
#208082=CARTESIAN_POINT('Ctrl Pts',(201.070412525896,0.12003351640835,135.723053196639));
#208083=CARTESIAN_POINT('Ctrl Pts',(201.062647772949,0.256819892510846,
135.715900763519));
#208084=CARTESIAN_POINT('Ctrl Pts',(201.054890732064,0.39347041045627,135.708755434297));
#208085=CARTESIAN_POINT('Ctrl Pts',(201.047133691179,0.52996533799027,135.695895406474));
#208086=CARTESIAN_POINT('Ctrl Pts',(201.039376650294,0.665790234716704,
135.677337780026));
#208087=CARTESIAN_POINT('Ctrl Pts',(201.031625459054,0.801512704831837,
135.658794148028));
#208088=CARTESIAN_POINT('Ctrl Pts',(201.023874267814,0.936565764060569,
135.634561522245));
#208089=CARTESIAN_POINT('Ctrl Pts',(201.016123076574,1.07043872863637,135.604708937296));
#208090=CARTESIAN_POINT('Ctrl Pts',(201.008375179797,1.20425479363109,135.574869040492));
#208091=CARTESIAN_POINT('Ctrl Pts',(201.00062728302,1.33689138076679,135.539414020244));
#208092=CARTESIAN_POINT('Ctrl Pts',(200.992879386243,1.46784687475884,135.498464218336));
#208093=CARTESIAN_POINT('Ctrl Pts',(200.985133110159,1.59877497568463,135.457522982243));
#208094=CARTESIAN_POINT('Ctrl Pts',(200.977386834075,1.72802231000401,135.411089367299));
#208095=CARTESIAN_POINT('Ctrl Pts',(200.969640557991,1.85510171848053,135.359333798232));
#208096=CARTESIAN_POINT('Ctrl Pts',(200.961894224726,1.98218206502826,135.307577847118));
#208097=CARTESIAN_POINT('Ctrl Pts',(200.954147891461,2.10709409171268,135.250500010957));
#208098=CARTESIAN_POINT('Ctrl Pts',(200.946401558195,2.22937031777955,135.188318994273));
#208099=CARTESIAN_POINT('Ctrl Pts',(200.938653490193,2.35167392675948,135.126124052582));
#208100=CARTESIAN_POINT('Ctrl Pts',(200.93090542219,2.47134021212813,135.058823833469));
#208101=CARTESIAN_POINT('Ctrl Pts',(200.923157354187,2.58792636704384,134.986682960626));
#208102=CARTESIAN_POINT('Ctrl Pts',(200.915401051445,2.70463643111238,134.914465415605));
#208103=CARTESIAN_POINT('Ctrl Pts',(200.907644748703,2.81825949236634,134.837397145802));
#208104=CARTESIAN_POINT('Ctrl Pts',(200.899888445961,2.92838136436711,134.755786391553));
#208105=CARTESIAN_POINT('Ctrl Pts',(200.892128003447,3.03856201172679,134.674132079186));
#208106=CARTESIAN_POINT('Ctrl Pts',(200.884367560933,3.14523744236723,134.587930697037));
#208107=CARTESIAN_POINT('Ctrl Pts',(200.876607118419,3.24802744199153,134.497530096289));
#208108=CARTESIAN_POINT('Ctrl Pts',(200.868834218154,3.35098244924848,134.406984376471));
#208109=CARTESIAN_POINT('Ctrl Pts',(200.861061317888,3.45003927881987,134.312226237882));
#208110=CARTESIAN_POINT('Ctrl Pts',(200.853288417623,3.54485477481942,134.213640261118));
#208111=CARTESIAN_POINT('Ctrl Pts',(200.84579808186,3.63622348872338,134.118638132923));
#208112=CARTESIAN_POINT('Ctrl Pts',(200.838307746098,3.723653677273,134.020081868339));
#208113=CARTESIAN_POINT('Ctrl Pts',(200.830817410335,3.80687549814816,133.918342313739));
#208114=CARTESIAN_POINT('Ctrl Pts',(200.823043076216,3.8932526996479,133.812745273014));
#208115=CARTESIAN_POINT('Ctrl Pts',(200.815268742097,3.97536973042481,133.703384288615));
#208116=CARTESIAN_POINT('Ctrl Pts',(200.807494407978,4.052880654051,133.59063796674));
#208117=CARTESIAN_POINT('Ctrl Pts',(200.799729655031,4.13029605239111,133.47803059463));
#208118=CARTESIAN_POINT('Ctrl Pts',(200.791964902084,4.20311641899065,133.362046505414));
#208119=CARTESIAN_POINT('Ctrl Pts',(200.784200149136,4.27103525191642,133.243098188398));
#208120=CARTESIAN_POINT('Ctrl Pts',(200.776443108251,4.33888662689985,133.124268012527));
#208121=CARTESIAN_POINT('Ctrl Pts',(200.768686067366,4.40184596368367,133.002479805092));
#208122=CARTESIAN_POINT('Ctrl Pts',(200.760929026481,4.45964958136172,132.878175622324));
#208123=CARTESIAN_POINT('Ctrl Pts',(200.753177835241,4.51740960888204,132.753965178307));
#208124=CARTESIAN_POINT('Ctrl Pts',(200.745426644001,4.57002149187464,132.627242888525));
#208125=CARTESIAN_POINT('Ctrl Pts',(200.737675452761,4.61726727407009,132.498475720592));
#208126=CARTESIAN_POINT('Ctrl Pts',(200.729927555984,4.66449297554781,132.369763282141));
#208127=CARTESIAN_POINT('Ctrl Pts',(200.722179659207,4.70635697805043,132.239008060438));
#208128=CARTESIAN_POINT('Ctrl Pts',(200.71443176243,4.74268939321458,132.106697126303));
#208129=CARTESIAN_POINT('Ctrl Pts',(200.706685486346,4.77901420842072,131.974413868764));
#208130=CARTESIAN_POINT('Ctrl Pts',(200.698939210262,4.80980963434076,131.840575922843));
#208131=CARTESIAN_POINT('Ctrl Pts',(200.691192934178,4.83495573265951,131.705685268135));
#208132=CARTESIAN_POINT('Ctrl Pts',(200.683446600912,4.86010201660105,131.570793617694));
#208133=CARTESIAN_POINT('Ctrl Pts',(200.675700267647,4.8795988180791,131.434849627302));
#208134=CARTESIAN_POINT('Ctrl Pts',(200.667953934382,4.89337745463654,131.298364816895));
#208135=CARTESIAN_POINT('Ctrl Pts',(200.660205866379,4.90715917682409,131.161849441661));
#208136=CARTESIAN_POINT('Ctrl Pts',(200.652457798376,4.91522014669572,131.024793394324));
#208137=CARTESIAN_POINT('Ctrl Pts',(200.644709730373,4.91754365174374,130.887712256391));
#208138=CARTESIAN_POINT('Ctrl Pts',(200.636953427631,4.91986962624059,130.750485426993));
#208139=CARTESIAN_POINT('Ctrl Pts',(200.629197124889,4.91644594817341,130.613233845261));
#208140=CARTESIAN_POINT('Ctrl Pts',(200.621440822147,4.90730807097843,130.476472589407));
#208141=CARTESIAN_POINT('Ctrl Pts',(200.613680379633,4.89816531662325,130.339638339953));
#208142=CARTESIAN_POINT('Ctrl Pts',(200.605919937119,4.88330232842366,130.203295326312));
#208143=CARTESIAN_POINT('Ctrl Pts',(200.598159494605,4.86280624831729,130.067951455601));
#208144=CARTESIAN_POINT('Ctrl Pts',(200.590386594339,4.84227726608359,129.932390318894));
#208145=CARTESIAN_POINT('Ctrl Pts',(200.582613694074,4.81609719637891,129.797831914236));
#208146=CARTESIAN_POINT('Ctrl Pts',(200.574840793809,4.78440411361137,129.664772823599));
#208147=CARTESIAN_POINT('Ctrl Pts',(200.567350458046,4.75386315423193,129.53655076606));
#208148=CARTESIAN_POINT('Ctrl Pts',(200.559860122284,4.71820313009367,129.409721203914));
#208149=CARTESIAN_POINT('Ctrl Pts',(200.552369786522,4.67759018838714,129.284711614669));
#208150=CARTESIAN_POINT('Ctrl Pts',(200.544595452403,4.63543739465235,129.154962248855));
#208151=CARTESIAN_POINT('Ctrl Pts',(200.536821118284,4.58781516216797,129.026762581828));
#208152=CARTESIAN_POINT('Ctrl Pts',(200.529046784165,4.53485503596222,128.900608305602));
#208153=CARTESIAN_POINT('Ctrl Pts',(200.521282031218,4.48196017837884,128.774609503247));
#208154=CARTESIAN_POINT('Ctrl Pts',(200.51351727827,4.42374066616417,128.650651433156));
#208155=CARTESIAN_POINT('Ctrl Pts',(200.505752525323,4.36037786647262,128.529214924632));
#208156=CARTESIAN_POINT('Ctrl Pts',(200.497995484438,4.29707799960699,128.407899028561));
#208157=CARTESIAN_POINT('Ctrl Pts',(200.490238443553,4.22864519086966,128.289100054462));
#208158=CARTESIAN_POINT('Ctrl Pts',(200.482481402668,4.15530882871568,128.173278786741));
#208159=CARTESIAN_POINT('Ctrl Pts',(200.474730211428,4.08202777008282,128.057544860739));
#208160=CARTESIAN_POINT('Ctrl Pts',(200.466979020188,4.00385072660107,127.944784500539));
#208161=CARTESIAN_POINT('Ctrl Pts',(200.459227828948,3.92105276066194,127.835433486327));
#208162=CARTESIAN_POINT('Ctrl Pts',(200.451479932171,3.83828998606706,127.726128949213));
#208163=CARTESIAN_POINT('Ctrl Pts',(200.443732035394,3.75091043080558,127.620231187053));
#208164=CARTESIAN_POINT('Ctrl Pts',(200.435984138616,3.65923205254183,127.518146405414));
#208165=CARTESIAN_POINT('Ctrl Pts',(200.428237862532,3.56757285141844,127.41608297771));
#208166=CARTESIAN_POINT('Ctrl Pts',(200.420491586448,3.47161687695752,127.317831234768));
#208167=CARTESIAN_POINT('Ctrl Pts',(200.412745310364,3.37172162921752,127.223763416321));
#208168=CARTESIAN_POINT('Ctrl Pts',(200.404998977099,3.27182564407353,127.129694903486));
#208169=CARTESIAN_POINT('Ctrl Pts',(200.397252643833,3.16799061225729,127.039810644801));
#208170=CARTESIAN_POINT('Ctrl Pts',(200.389506310568,3.06060976543159,126.954444913782));
#208171=CARTESIAN_POINT('Ctrl Pts',(200.381758242565,2.95320487140979,126.869060065699));
#208172=CARTESIAN_POINT('Ctrl Pts',(200.374010174562,2.84225288827149,126.788196002082));
#208173=CARTESIAN_POINT('Ctrl Pts',(200.366262106559,2.72817855582115,126.712145468034));
#208174=CARTESIAN_POINT('Ctrl Pts',(200.358505803817,2.61398298381271,126.636014106574));
#208175=CARTESIAN_POINT('Ctrl Pts',(200.350749501075,2.49665875931106,126.564706711413));
#208176=CARTESIAN_POINT('Ctrl Pts',(200.342993198333,2.37665839565136,126.498471866927));
#208177=CARTESIAN_POINT('Ctrl Pts',(200.335232755819,2.25659398418439,126.43220167091));
#208178=CARTESIAN_POINT('Ctrl Pts',(200.327472313305,2.13385093720195,126.371009594588));
#208179=CARTESIAN_POINT('Ctrl Pts',(200.319711870791,2.00890367369267,126.315096859184));
#208180=CARTESIAN_POINT('Ctrl Pts',(200.311938970525,1.8837558337437,126.259094367693));
#208181=CARTESIAN_POINT('Ctrl Pts',(200.30416607026,1.75639706985327,126.208388297305));
#208182=CARTESIAN_POINT('Ctrl Pts',(200.296393169994,1.62731980308813,126.163130896794));
#208183=CARTESIAN_POINT('Ctrl Pts',(200.288902834233,1.50293482010056,126.11951871679));
#208184=CARTESIAN_POINT('Ctrl Pts',(200.281412498471,1.37695440338238,126.08096602872));
#208185=CARTESIAN_POINT('Ctrl Pts',(200.273922162709,1.24982800848328,126.047564110282));
#208186=CARTESIAN_POINT('Ctrl Pts',(200.26614782859,1.11788157767805,126.012895747953));
#208187=CARTESIAN_POINT('Ctrl Pts',(200.258373494471,0.984282587110447,
125.983666629395));
#208188=CARTESIAN_POINT('Ctrl Pts',(200.250599160352,0.849519179810192,
125.960034015691));
#208189=CARTESIAN_POINT('Ctrl Pts',(200.242834407405,0.714921856365283,
125.936430527071));
#208190=CARTESIAN_POINT('Ctrl Pts',(200.235069654458,0.579163352880725,
125.918409886831));
#208191=CARTESIAN_POINT('Ctrl Pts',(200.227304901511,0.442746238043899,
125.906079405631));
#208192=CARTESIAN_POINT('Ctrl Pts',(200.219547860626,0.306464614608663,
125.893761171238));
#208193=CARTESIAN_POINT('Ctrl Pts',(200.211790819741,0.1695260684516,125.88712188402));
#208194=CARTESIAN_POINT('Ctrl Pts',(200.204033778856,0.0324422606050424,
125.886217618199));
#208195=CARTESIAN_POINT('Ctrl Pts',(200.196282587615,-0.104538171275545,
125.885314034291));
#208196=CARTESIAN_POINT('Ctrl Pts',(200.188531396375,-0.241663257432193,
125.890136866048));
#208197=CARTESIAN_POINT('Ctrl Pts',(200.180780205135,-0.378417685712695,
125.900690245524));
#208198=CARTESIAN_POINT('Ctrl Pts',(200.173032308358,-0.515113989713261,
125.911239139532));
#208199=CARTESIAN_POINT('Ctrl Pts',(200.165284411581,-0.651439560181567,
125.927513706947));
#208200=CARTESIAN_POINT('Ctrl Pts',(200.157536514804,-0.78688078098602,
125.949466005011));
#208201=CARTESIAN_POINT('Ctrl Pts',(200.14979023872,-0.922293670406798,
125.971413711128));
#208202=CARTESIAN_POINT('Ctrl Pts',(200.142043962636,-1.05682219242837,
125.999036723063));
#208203=CARTESIAN_POINT('Ctrl Pts',(200.134297686552,-1.18995993370752,
126.032235470562));
#208204=CARTESIAN_POINT('Ctrl Pts',(200.126551353286,-1.3230986577791,126.065434463126));
#208205=CARTESIAN_POINT('Ctrl Pts',(200.118805020021,-1.454846201273,126.104209178789));
#208206=CARTESIAN_POINT('Ctrl Pts',(200.111058686756,-1.58470877909421,
126.148409463617));
#208207=CARTESIAN_POINT('Ctrl Pts',(200.103310618753,-1.71460043873933,
126.192619646792));
#208208=CARTESIAN_POINT('Ctrl Pts',(200.09556255075,-1.84260592268838,126.242257690929));
#208209=CARTESIAN_POINT('Ctrl Pts',(200.087814482747,-1.96824935395539,
126.297124486282));
#208210=CARTESIAN_POINT('Ctrl Pts',(200.080058180005,-2.09402632055645,
126.352049594717));
#208211=CARTESIAN_POINT('Ctrl Pts',(200.072301877263,-2.21743586078181,
126.41221439872));
#208212=CARTESIAN_POINT('Ctrl Pts',(200.064545574521,-2.33802423904589,
126.477372551933));
#208213=CARTESIAN_POINT('Ctrl Pts',(200.056785132007,-2.45867697895829,
126.542565482013));
#208214=CARTESIAN_POINT('Ctrl Pts',(200.049024689493,-2.57650522087711,
126.612756871751));
#208215=CARTESIAN_POINT('Ctrl Pts',(200.041264246979,-2.69108323663666,
126.687656344));
#208216=CARTESIAN_POINT('Ctrl Pts',(200.033491346713,-2.80584518319893,
126.762676051532));
#208217=CARTESIAN_POINT('Ctrl Pts',(200.025718446448,-2.91734615908058,
126.842418716971));
#208218=CARTESIAN_POINT('Ctrl Pts',(200.017945546182,-3.02519190746045,
126.926552346708));
#208219=CARTESIAN_POINT('Ctrl Pts',(200.01045521042,-3.12911719124147,127.007627507086));
#208220=CARTESIAN_POINT('Ctrl Pts',(200.002964874658,-3.22964815206794,
127.092779730022));
#208221=CARTESIAN_POINT('Ctrl Pts',(199.995474538896,-3.32646505372397,
127.181680213659));
#208222=CARTESIAN_POINT('Ctrl Pts',(199.987817885007,-3.42543171291799,
127.272554675822));
#208223=CARTESIAN_POINT('Ctrl Pts',(199.980161231117,-3.52085100355156,
127.367652463917));
#208224=CARTESIAN_POINT('Ctrl Pts',(199.972504577228,-3.61233263415092,
127.466661409616));
#208225=CARTESIAN_POINT('Ctrl Pts',(199.964856779005,-3.7037084573244,127.565555841815));
#208226=CARTESIAN_POINT('Ctrl Pts',(199.957208980783,-3.79115540274886,
127.668352146295));
#208227=CARTESIAN_POINT('Ctrl Pts',(199.94956118256,-3.87431677020004,127.774698486792));
#208228=CARTESIAN_POINT('Ctrl Pts',(199.941920455469,-3.95740124690412,
127.880946499786));
#208229=CARTESIAN_POINT('Ctrl Pts',(199.934279728377,-4.03620777736056,
127.990737706671));
#208230=CARTESIAN_POINT('Ctrl Pts',(199.926639001285,-4.11041742727574,
128.10368447333));
#208231=CARTESIAN_POINT('Ctrl Pts',(199.918999136713,-4.18461870007081,
128.216618490047));
#208232=CARTESIAN_POINT('Ctrl Pts',(199.911359272141,-4.2542238720399,128.332707043142));
#208233=CARTESIAN_POINT('Ctrl Pts',(199.90371940757,-4.31895501961334,128.451530279217));
#208234=CARTESIAN_POINT('Ctrl Pts',(199.896087179009,-4.38362146868872,
128.570234751988));
#208235=CARTESIAN_POINT('Ctrl Pts',(199.888454950448,-4.44342342148269,
128.69166809915));
#208236=CARTESIAN_POINT('Ctrl Pts',(199.880822721887,-4.49812811338532,
128.815384363793));
#208237=CARTESIAN_POINT('Ctrl Pts',(199.87317903931,-4.55291490299365,128.939286294805));
#208238=CARTESIAN_POINT('Ctrl Pts',(199.865535356733,-4.60258893508908,
129.065477639417));
#208239=CARTESIAN_POINT('Ctrl Pts',(199.857891674155,-4.64696388063631,
129.19348825932));
#208240=CARTESIAN_POINT('Ctrl Pts',(199.850247991578,-4.69133882618354,
129.321498879223));
#208241=CARTESIAN_POINT('Ctrl Pts',(199.842604309,-4.73041455848543,129.451328387816));
#208242=CARTESIAN_POINT('Ctrl Pts',(199.834960626423,-4.76405452823405,
129.582490119308));
#208243=CARTESIAN_POINT('',(201.860140564039,-4.91824790150174,130.799817284683));
#208244=CARTESIAN_POINT('Ctrl Pts',(201.860140564008,-4.91824790150225,
130.799817285234));
#208245=CARTESIAN_POINT('Ctrl Pts',(201.852483585455,-4.91837276654937,
130.934986190149));
#208246=CARTESIAN_POINT('Ctrl Pts',(201.844826606902,-4.91292114291673,
131.07031288466));
#208247=CARTESIAN_POINT('Ctrl Pts',(201.83716962835,-4.90188083750575,131.205293676061));
#208248=CARTESIAN_POINT('Ctrl Pts',(201.829228030736,-4.89043015072319,
131.345291865101));
#208249=CARTESIAN_POINT('Ctrl Pts',(201.821286433122,-4.8729672167622,131.484917501621));
#208250=CARTESIAN_POINT('Ctrl Pts',(201.813344835508,-4.84953772420023,
131.62360839697));
#208251=CARTESIAN_POINT('Ctrl Pts',(201.80569610997,-4.82697226989009,131.757184617366));
#208252=CARTESIAN_POINT('Ctrl Pts',(201.798047384431,-4.79887259272399,
131.889893384014));
#208253=CARTESIAN_POINT('Ctrl Pts',(201.790398658893,-4.76533224076631,
132.021238465837));
#208254=CARTESIAN_POINT('Ctrl Pts',(201.782750978392,-4.73179647139039,
132.152565602125));
#208255=CARTESIAN_POINT('Ctrl Pts',(201.775103297891,-4.69282160461944,
132.282529034708));
#208256=CARTESIAN_POINT('Ctrl Pts',(201.767455617389,-4.64855188812975,
132.410644654051));
#208257=CARTESIAN_POINT('Ctrl Pts',(201.759807225106,-4.60427805138161,
132.538772197334));
#208258=CARTESIAN_POINT('Ctrl Pts',(201.752158832822,-4.5547085165048,132.665051205577));
#208259=CARTESIAN_POINT('Ctrl Pts',(201.744510440538,-4.50003661315956,
132.789015132267));
#208260=CARTESIAN_POINT('Ctrl Pts',(201.736859579318,-4.44534706147838,
132.913019075069));
#208261=CARTESIAN_POINT('Ctrl Pts',(201.729208718099,-4.38555202834284,
133.034706082836));
#208262=CARTESIAN_POINT('Ctrl Pts',(201.72155785688,-4.32089170944105,133.153632397881));
#208263=CARTESIAN_POINT('Ctrl Pts',(201.713898683524,-4.25616114153522,
133.272687918215));
#208264=CARTESIAN_POINT('Ctrl Pts',(201.706239510168,-4.18655493051007,
133.388976406699));
#208265=CARTESIAN_POINT('Ctrl Pts',(201.698580336813,-4.11235781880762,
133.502081179928));
#208266=CARTESIAN_POINT('Ctrl Pts',(201.690916213761,-4.03811275765906,
133.615259046451));
#208267=CARTESIAN_POINT('Ctrl Pts',(201.68325209071,-3.95927112365503,133.725248776863));
#208268=CARTESIAN_POINT('Ctrl Pts',(201.675587967659,-3.87615836955861,
133.831666244126));
#208269=CARTESIAN_POINT('Ctrl Pts',(201.667913108811,-3.79292919227884,
133.938232779488));
#208270=CARTESIAN_POINT('Ctrl Pts',(201.660238249964,-3.70541721587963,
134.041216762563));
#208271=CARTESIAN_POINT('Ctrl Pts',(201.652563391116,-3.61398532778852,
134.140270255585));
#208272=CARTESIAN_POINT('Ctrl Pts',(201.650566022616,-3.59019033991468,
134.166048752722));
#208273=CARTESIAN_POINT('Ctrl Pts',(201.648568654115,-3.56613003589684,
134.191561251679));
#208274=CARTESIAN_POINT('Ctrl Pts',(201.646571285615,-3.54181117222063,
134.216802072424));
#208275=CARTESIAN_POINT('Ctrl Pts',(201.638796951494,-3.44715514275093,
134.315046624639));
#208276=CARTESIAN_POINT('Ctrl Pts',(201.631022617374,-3.34825835130227,
134.409505379128));
#208277=CARTESIAN_POINT('Ctrl Pts',(201.623248283254,-3.24545589596689,
134.499790104085));
#208278=CARTESIAN_POINT('Ctrl Pts',(201.615483530306,-3.14278013546986,
134.589963561187));
#208279=CARTESIAN_POINT('Ctrl Pts',(201.607718777357,-3.03620857922076,
134.675972968507));
#208280=CARTESIAN_POINT('Ctrl Pts',(201.599954024409,-2.92611462881938,
134.757465250827));
#208281=CARTESIAN_POINT('Ctrl Pts',(201.592196983523,-2.8161300252812,134.838876593864));
#208282=CARTESIAN_POINT('Ctrl Pts',(201.584439942637,-2.70263030195642,
134.915779509083));
#208283=CARTESIAN_POINT('Ctrl Pts',(201.576682901751,-2.58602327795652,
134.987859950465));
#208284=CARTESIAN_POINT('Ctrl Pts',(201.568931710509,-2.46950418822028,
135.059886035426));
#208285=CARTESIAN_POINT('Ctrl Pts',(201.561180519268,-2.3498827930975,135.127096680372));
#208286=CARTESIAN_POINT('Ctrl Pts',(201.553429328027,-2.22759704920044,
135.189220301626));
#208287=CARTESIAN_POINT('Ctrl Pts',(201.545681431248,-2.10536328000659,
135.251317518684));
#208288=CARTESIAN_POINT('Ctrl Pts',(201.53793353447,-1.98046776216892,135.308331835635));
#208289=CARTESIAN_POINT('Ctrl Pts',(201.530185637692,-1.85337409203519,
135.360037025902));
#208290=CARTESIAN_POINT('Ctrl Pts',(201.522439361606,-1.72630700715721,
135.411731400558));
#208291=CARTESIAN_POINT('Ctrl Pts',(201.514693085521,-1.59704304647646,
135.458118710247));
#208292=CARTESIAN_POINT('Ctrl Pts',(201.506946809436,-1.46606651029953,
135.499020567965));
#208293=CARTESIAN_POINT('Ctrl Pts',(201.499200476169,-1.33508900728361,
135.539922727611));
#208294=CARTESIAN_POINT('Ctrl Pts',(201.491454142903,-1.20239927673706,
135.575339237944));
#208295=CARTESIAN_POINT('Ctrl Pts',(201.483707809636,-1.0684971462986,135.605141482264));
#208296=CARTESIAN_POINT('Ctrl Pts',(201.475959741632,-0.934565029406161,
135.63495040059));
#208297=CARTESIAN_POINT('Ctrl Pts',(201.468211673628,-0.799420353905459,
135.659142466148));
#208298=CARTESIAN_POINT('Ctrl Pts',(201.460463605623,-0.663573118682993,
135.677640188724));
#208299=CARTESIAN_POINT('Ctrl Pts',(201.45270730288,-0.527581503402445,
135.696157570899));
#208300=CARTESIAN_POINT('Ctrl Pts',(201.444951000137,-0.390886224816852,
135.708968467706));
#208301=CARTESIAN_POINT('Ctrl Pts',(201.437194697394,-0.254002943294543,
135.716047249192));
#208302=CARTESIAN_POINT('Ctrl Pts',(201.429434254879,-0.117046603043397,
135.723129808838));
#208303=CARTESIAN_POINT('Ctrl Pts',(201.421673812363,0.0200975493309183,
135.724474153213));
#208304=CARTESIAN_POINT('Ctrl Pts',(201.413913369848,0.156914869496959,
135.720106826051));
#208305=CARTESIAN_POINT('Ctrl Pts',(201.406140469581,0.293951820971461,
135.715732488067));
#208306=CARTESIAN_POINT('Ctrl Pts',(201.398367569315,0.430660501673616,
135.705628185033));
#208307=CARTESIAN_POINT('Ctrl Pts',(201.390594669048,0.566531497579824,
135.689872374255));
#208308=CARTESIAN_POINT('Ctrl Pts',(201.383104333299,0.697463240297336,
135.674689326915));
#208309=CARTESIAN_POINT('Ctrl Pts',(201.37561399755,0.827616840453072,135.654258578995));
#208310=CARTESIAN_POINT('Ctrl Pts',(201.368123661801,0.956548189162586,
135.628694625935));
#208311=CARTESIAN_POINT('Ctrl Pts',(201.360349327683,1.09036800937337,135.60216140778));
#208312=CARTESIAN_POINT('Ctrl Pts',(201.352574993564,1.22329496617451,135.570014000326));
#208313=CARTESIAN_POINT('Ctrl Pts',(201.344800659445,1.35482130044931,135.532324482313));
#208314=CARTESIAN_POINT('Ctrl Pts',(201.337035906498,1.48618554027203,135.494681413262));
#208315=CARTESIAN_POINT('Ctrl Pts',(201.329271153552,1.61615221984584,135.451509930292));
#208316=CARTESIAN_POINT('Ctrl Pts',(201.321506400605,1.74422245430599,135.402933340966));
#208317=CARTESIAN_POINT('Ctrl Pts',(201.31374935972,1.87216548760419,135.354404998592));
#208318=CARTESIAN_POINT('Ctrl Pts',(201.305992318836,1.99821546100229,135.300482371031));
#208319=CARTESIAN_POINT('Ctrl Pts',(201.298235277951,2.12188772249806,135.241338818505));
#208320=CARTESIAN_POINT('Ctrl Pts',(201.290484086711,2.24546672177877,135.182239866593));
#208321=CARTESIAN_POINT('Ctrl Pts',(201.282732895472,2.36667122683608,135.117927994348));
#208322=CARTESIAN_POINT('Ctrl Pts',(201.274981704232,2.48503602038379,135.048624869459));
#208323=CARTESIAN_POINT('Ctrl Pts',(201.267233807455,2.60335050573666,134.979351200247));
#208324=CARTESIAN_POINT('Ctrl Pts',(201.259485910679,2.71882734343585,134.905090694853));
#208325=CARTESIAN_POINT('Ctrl Pts',(201.251738013902,2.83102561750346,134.826111109024));
#208326=CARTESIAN_POINT('Ctrl Pts',(201.243991737818,2.94320042211094,134.747148044021));
#208327=CARTESIAN_POINT('Ctrl Pts',(201.236245461735,3.0520977076928,134.663468086941));
#208328=CARTESIAN_POINT('Ctrl Pts',(201.228499185651,3.15730561606483,134.575382270814));
#208329=CARTESIAN_POINT('Ctrl Pts',(201.220752852386,3.26251430105758,134.487295804458));
#208330=CARTESIAN_POINT('Ctrl Pts',(201.213006519121,3.36403325472788,134.394803665141));
#208331=CARTESIAN_POINT('Ctrl Pts',(201.205260185856,3.46148409915498,134.298256851543));
#208332=CARTESIAN_POINT('Ctrl Pts',(201.197512117854,3.55895676702291,134.201688416955));
#208333=CARTESIAN_POINT('Ctrl Pts',(201.189764049851,3.6523592351274,134.101063776349));
#208334=CARTESIAN_POINT('Ctrl Pts',(201.182015981848,3.74135064190172,133.996770120879));
#208335=CARTESIAN_POINT('Ctrl Pts',(201.174259679107,3.8304366298024,133.89236562087));
#208336=CARTESIAN_POINT('Ctrl Pts',(201.166503376366,3.91510193715322,133.784284614265));
#208337=CARTESIAN_POINT('Ctrl Pts',(201.158747073624,3.99504627372427,133.672947087119));
#208338=CARTESIAN_POINT('Ctrl Pts',(201.15098663111,4.07503327899471,133.561550135783));
#208339=CARTESIAN_POINT('Ctrl Pts',(201.143226188597,4.1502940782862,133.446893527272));
#208340=CARTESIAN_POINT('Ctrl Pts',(201.135465746083,4.22057282576062,133.329424593974));
#208341=CARTESIAN_POINT('Ctrl Pts',(201.127692845818,4.2909643909197,133.211767089115));
#208342=CARTESIAN_POINT('Ctrl Pts',(201.119919945553,4.35635773583158,133.091288581682));
#208343=CARTESIAN_POINT('Ctrl Pts',(201.112147045288,4.41654351812895,132.968460064212));
#208344=CARTESIAN_POINT('Ctrl Pts',(201.104656709521,4.47454139567703,132.850096672665));
#208345=CARTESIAN_POINT('Ctrl Pts',(201.097166373755,4.5277036290204,132.729551444137));
#208346=CARTESIAN_POINT('Ctrl Pts',(201.089676037989,4.57588649471474,132.607259907595));
#208347=CARTESIAN_POINT('Ctrl Pts',(201.08190170387,4.62589622837748,132.48033165035));
#208348=CARTESIAN_POINT('Ctrl Pts',(201.074127369751,4.67069997109745,132.351119977928));
#208349=CARTESIAN_POINT('Ctrl Pts',(201.066353035632,4.71008390855603,132.220091042775));
#208350=CARTESIAN_POINT('Ctrl Pts',(201.058588282685,4.74941930883149,132.089223589074));
#208351=CARTESIAN_POINT('Ctrl Pts',(201.050823529738,4.78334808245175,131.956543699629));
#208352=CARTESIAN_POINT('Ctrl Pts',(201.043058776791,4.81170431210567,131.822537751155));
#208353=CARTESIAN_POINT('Ctrl Pts',(201.035301735906,4.84003237795253,131.688664899279));
#208354=CARTESIAN_POINT('Ctrl Pts',(201.027544695021,4.86279883378002,131.553468989404));
#208355=CARTESIAN_POINT('Ctrl Pts',(201.019787654136,4.87988756620843,131.417451478421));
#208356=CARTESIAN_POINT('Ctrl Pts',(201.012036462896,4.89696341189084,131.281536539302));
#208357=CARTESIAN_POINT('Ctrl Pts',(201.004285271656,4.90837000793079,131.144801618648));
#208358=CARTESIAN_POINT('Ctrl Pts',(200.996534080416,4.91404238832683,131.007757933741));
#208359=CARTESIAN_POINT('Ctrl Pts',(200.988786183639,4.91971235780988,130.870772496056));
#208360=CARTESIAN_POINT('Ctrl Pts',(200.981038286862,4.91965294290856,130.733478944942));
#208361=CARTESIAN_POINT('Ctrl Pts',(200.973290390085,4.91385108825839,130.596392964019));
#208362=CARTESIAN_POINT('Ctrl Pts',(200.965544114001,4.90805044723114,130.459335658529));
#208363=CARTESIAN_POINT('Ctrl Pts',(200.957797837917,4.89650977221841,130.322486227234));
#208364=CARTESIAN_POINT('Ctrl Pts',(200.950051561833,4.87926812470907,130.186359299041));
#208365=CARTESIAN_POINT('Ctrl Pts',(200.942305228568,4.86202634992579,130.050231365991));
#208366=CARTESIAN_POINT('Ctrl Pts',(200.934558895303,4.83908356779839,129.91482633455));
#208367=CARTESIAN_POINT('Ctrl Pts',(200.926812562038,4.81053056094829,129.780652268141));
#208368=CARTESIAN_POINT('Ctrl Pts',(200.919064494035,4.78197115985042,129.646448154381));
#208369=CARTESIAN_POINT('Ctrl Pts',(200.911316426032,4.74779911535903,129.513475936524));
#208370=CARTESIAN_POINT('Ctrl Pts',(200.903568358029,4.70815593835484,129.382231677338));
#208371=CARTESIAN_POINT('Ctrl Pts',(200.895812055287,4.66847062811032,129.250847930191));
#208372=CARTESIAN_POINT('Ctrl Pts',(200.888055752546,4.62330268292331,129.121196185172));
#208373=CARTESIAN_POINT('Ctrl Pts',(200.880299449804,4.57284313475343,128.993756097678));
#208374=CARTESIAN_POINT('Ctrl Pts',(200.87253900729,4.52235665480324,128.866247991572));
#208375=CARTESIAN_POINT('Ctrl Pts',(200.864778564776,4.46657310317764,128.740954252085));
#208376=CARTESIAN_POINT('Ctrl Pts',(200.857018122262,4.40573054235811,128.618331923648));
#208377=CARTESIAN_POINT('Ctrl Pts',(200.849245221996,4.34479031165874,128.495512750964));
#208378=CARTESIAN_POINT('Ctrl Pts',(200.841472321731,4.27877503146672,128.375373901733));
#208379=CARTESIAN_POINT('Ctrl Pts',(200.833699421466,4.20796780647951,128.258346084589));
#208380=CARTESIAN_POINT('Ctrl Pts',(200.826209085702,4.13973460246116,128.145572523353));
#208381=CARTESIAN_POINT('Ctrl Pts',(200.818718749939,4.06705197339164,128.035687990354));
#208382=CARTESIAN_POINT('Ctrl Pts',(200.811228414176,3.99020865609362,127.929048818241));
#208383=CARTESIAN_POINT('Ctrl Pts',(200.803454080057,3.91045180107535,127.818366389521));
#208384=CARTESIAN_POINT('Ctrl Pts',(200.795679745938,3.82595987893068,127.710829666744));
#208385=CARTESIAN_POINT('Ctrl Pts',(200.787905411818,3.73700950505258,127.606870504736));
#208386=CARTESIAN_POINT('Ctrl Pts',(200.780140658871,3.64816875456051,127.503039463103));
#208387=CARTESIAN_POINT('Ctrl Pts',(200.772375905924,3.55488073677464,127.402777503809));
#208388=CARTESIAN_POINT('Ctrl Pts',(200.764611152976,3.45746497184096,127.306487116281));
#208389=CARTESIAN_POINT('Ctrl Pts',(200.756854112091,3.36014596161846,127.210292365723));
#208390=CARTESIAN_POINT('Ctrl Pts',(200.749097071206,3.25870763916541,127.118061610023));
#208391=CARTESIAN_POINT('Ctrl Pts',(200.741340030321,3.15350913224816,127.030163588352));
#208392=CARTESIAN_POINT('Ctrl Pts',(200.733588839081,3.04838995634344,126.942331851264));
#208393=CARTESIAN_POINT('Ctrl Pts',(200.72583764784,2.93951653884054,126.858826594413));
#208394=CARTESIAN_POINT('Ctrl Pts',(200.7180864566,2.82728386560443,126.779978800964));
#208395=CARTESIAN_POINT('Ctrl Pts',(200.710338559823,2.71509889424786,126.701164519931));
#208396=CARTESIAN_POINT('Ctrl Pts',(200.702590663046,2.59955782612968,126.627003989411));
#208397=CARTESIAN_POINT('Ctrl Pts',(200.694842766268,2.48108746374105,126.557786932845));
#208398=CARTESIAN_POINT('Ctrl Pts',(200.687096490184,2.36264188279868,126.488584354995));
#208399=CARTESIAN_POINT('Ctrl Pts',(200.6793502141,2.24126856372764,126.424323391385));
#208400=CARTESIAN_POINT('Ctrl Pts',(200.671603938015,2.11742159208994,126.36524934797));
#208401=CARTESIAN_POINT('Ctrl Pts',(200.66385760475,1.99357370624226,126.306174868485));
#208402=CARTESIAN_POINT('Ctrl Pts',(200.656111271484,1.86725248426869,126.252287553918));
#208403=CARTESIAN_POINT('Ctrl Pts',(200.648364938219,1.7389344445388,126.203785646968));
#208404=CARTESIAN_POINT('Ctrl Pts',(200.640616870216,1.61058766887319,126.155272878351));
#208405=CARTESIAN_POINT('Ctrl Pts',(200.632868802213,1.48024355127012,126.112148055408));
#208406=CARTESIAN_POINT('Ctrl Pts',(200.625120734209,1.34839593347158,126.074560255067));
#208407=CARTESIAN_POINT('Ctrl Pts',(200.617364431467,1.21640818645573,126.036932505965));
#208408=CARTESIAN_POINT('Ctrl Pts',(200.609608128725,1.08291412377568,126.004853642373));
#208409=CARTESIAN_POINT('Ctrl Pts',(200.601851825983,0.948420550542189,
125.978422209152));
#208410=CARTESIAN_POINT('Ctrl Pts',(200.594091383469,0.813855194038882,
125.951976668679));
#208411=CARTESIAN_POINT('Ctrl Pts',(200.586330940955,0.678289650257551,
125.931184623874));
#208412=CARTESIAN_POINT('Ctrl Pts',(200.57857049844,0.54223712220886,125.916092829709));
#208413=CARTESIAN_POINT('Ctrl Pts',(200.570797598175,0.405966190564276,
125.900976808856));
#208414=CARTESIAN_POINT('Ctrl Pts',(200.563024697909,0.269207102735885,
125.891579351172));
#208415=CARTESIAN_POINT('Ctrl Pts',(200.555251797643,0.132475251099434,
125.887895081193));
#208416=CARTESIAN_POINT('Ctrl Pts',(200.547761461883,0.000713946712914748,
125.884344743708));
#208417=CARTESIAN_POINT('Ctrl Pts',(200.540271126123,-0.131021759319523,
125.88609942386));
#208418=CARTESIAN_POINT('Ctrl Pts',(200.532780790363,-0.262276004943429,
125.893108805682));
#208419=CARTESIAN_POINT('Ctrl Pts',(200.525006456244,-0.398506795217166,
125.900383950348));
#208420=CARTESIAN_POINT('Ctrl Pts',(200.517232122125,-0.534650433432306,
125.913343171992));
#208421=CARTESIAN_POINT('Ctrl Pts',(200.509457788006,-0.670194070517084,
125.931987174331));
#208422=CARTESIAN_POINT('Ctrl Pts',(200.501693035059,-0.805570662182922,
125.950608199603));
#208423=CARTESIAN_POINT('Ctrl Pts',(200.493928282112,-0.940348340398937,
125.974900012985));
#208424=CARTESIAN_POINT('Ctrl Pts',(200.486163529165,-1.07401577096679,
126.004811348498));
#208425=CARTESIAN_POINT('Ctrl Pts',(200.47840648828,-1.20755044115865,126.03469297565));
#208426=CARTESIAN_POINT('Ctrl Pts',(200.470649447395,-1.33997667909172,
126.070182932893));
#208427=CARTESIAN_POINT('Ctrl Pts',(200.46289240651,-1.47079013672649,126.111178388395));
#208428=CARTESIAN_POINT('Ctrl Pts',(200.45514121527,-1.60150494691511,126.152142928905));
#208429=CARTESIAN_POINT('Ctrl Pts',(200.44739002403,-1.73060902603362,126.198604587446));
#208430=CARTESIAN_POINT('Ctrl Pts',(200.43963883279,-1.85761040906449,126.250409955708));
#208431=CARTESIAN_POINT('Ctrl Pts',(200.431890936013,-1.9845578131194,126.302193305306));
#208432=CARTESIAN_POINT('Ctrl Pts',(200.424143039236,-2.10940393734354,
126.359315699986));
#208433=CARTESIAN_POINT('Ctrl Pts',(200.416395142459,-2.23167433202904,
126.421574661321));
#208434=CARTESIAN_POINT('Ctrl Pts',(200.408648866375,-2.35391915038416,
126.483820599422));
#208435=CARTESIAN_POINT('Ctrl Pts',(200.400902590291,-2.47358896269875,
126.551200789732));
#208436=CARTESIAN_POINT('Ctrl Pts',(200.393156314207,-2.59023194178586,
126.623465791066));
#208437=CARTESIAN_POINT('Ctrl Pts',(200.385409980941,-2.70687578190523,
126.695731325845));
#208438=CARTESIAN_POINT('Ctrl Pts',(200.377663647676,-2.82049241186166,
126.772881537696));
#208439=CARTESIAN_POINT('Ctrl Pts',(200.369917314411,-2.93065747463995,
126.854622673241));
#208440=CARTESIAN_POINT('Ctrl Pts',(200.362169246408,-3.04084720811968,
126.936382114147));
#208441=CARTESIAN_POINT('Ctrl Pts',(200.354421178405,-3.14758352241582,
127.022734291636));
#208442=CARTESIAN_POINT('Ctrl Pts',(200.346673110402,-3.25047406136048,
127.113344302386));
#208443=CARTESIAN_POINT('Ctrl Pts',(200.33891680766,-3.3534739535945,127.204050614535));
#208444=CARTESIAN_POINT('Ctrl Pts',(200.331160504918,-3.45261961170661,
127.29902354087));
#208445=CARTESIAN_POINT('Ctrl Pts',(200.323404202176,-3.54755418657293,
127.397889957803));
#208446=CARTESIAN_POINT('Ctrl Pts',(200.315643759662,-3.64253943088031,
127.496809142719));
#208447=CARTESIAN_POINT('Ctrl Pts',(200.307883317148,-3.73330885482172,
127.599625666022));
#208448=CARTESIAN_POINT('Ctrl Pts',(200.300122874634,-3.8195457233528,127.705933027688));
#208449=CARTESIAN_POINT('Ctrl Pts',(200.292349974369,-3.90592102696098,
127.812411043368));
#208450=CARTESIAN_POINT('Ctrl Pts',(200.284577074103,-3.98774900175901,
127.922390781748));
#208451=CARTESIAN_POINT('Ctrl Pts',(200.276804173838,-4.06475558810789,
128.035435723054));
#208452=CARTESIAN_POINT('Ctrl Pts',(200.269313838075,-4.13896279108229,
128.144371196012));
#208453=CARTESIAN_POINT('Ctrl Pts',(200.261823502312,-4.20869289593499,
128.256152623966));
#208454=CARTESIAN_POINT('Ctrl Pts',(200.25433316655,-4.27374183033709,128.37036928025));
#208455=CARTESIAN_POINT('Ctrl Pts',(200.246220788594,-4.34419281654029,
128.494071169452));
#208456=CARTESIAN_POINT('Ctrl Pts',(200.238108410639,-4.40935986504164,
128.620992964794));
#208457=CARTESIAN_POINT('Ctrl Pts',(200.229996032683,-4.46895007272139,
128.750664362025));
#208458=CARTESIAN_POINT('Ctrl Pts',(200.221641782561,-4.53031697432501,
128.88420193782));
#208459=CARTESIAN_POINT('Ctrl Pts',(200.213287532439,-4.58576906133034,
129.02065536604));
#208460=CARTESIAN_POINT('Ctrl Pts',(200.204933282317,-4.6350349423211,129.159479422475));
#208461=CARTESIAN_POINT('Ctrl Pts',(200.196579032196,-4.68430082331187,
129.298303478911));
#208462=CARTESIAN_POINT('Ctrl Pts',(200.188224782074,-4.7273802889641,129.439497817004));
#208463=CARTESIAN_POINT('Ctrl Pts',(200.179870531952,-4.76405452823405,
129.582490119308));
#208464=CARTESIAN_POINT('Ctrl Pts',(201.930097584127,-4.76405452823404,
129.582490119308));
#208465=CARTESIAN_POINT('Ctrl Pts',(201.928404692561,-4.77143981658942,
129.611285246518));
#208466=CARTESIAN_POINT('Ctrl Pts',(201.926711800994,-4.77856158153426,
129.640137793894));
#208467=CARTESIAN_POINT('Ctrl Pts',(201.925018909427,-4.78541909345683,
129.669042528888));
#208468=CARTESIAN_POINT('Ctrl Pts',(201.914205851863,-4.82922028700719,
129.853666617963));
#208469=CARTESIAN_POINT('Ctrl Pts',(201.903392794298,-4.86235268751459,
130.040911499407));
#208470=CARTESIAN_POINT('Ctrl Pts',(201.892579736733,-4.88456555156559,
130.22972818291));
#208471=CARTESIAN_POINT('Ctrl Pts',(201.882347687665,-4.90558487136082,
130.408399345895));
#208472=CARTESIAN_POINT('Ctrl Pts',(201.872115638597,-4.91682686629452,
130.58847825068));
#208473=CARTESIAN_POINT('Ctrl Pts',(201.861883589529,-4.91812325643309,
130.769052020427));
#208474=CARTESIAN_POINT('Ctrl Pts',(201.861302581032,-4.91819686961459,
130.779305577046));
#208475=CARTESIAN_POINT('Ctrl Pts',(201.860721572536,-4.91823842679033,
130.789560721775));
#208476=CARTESIAN_POINT('Ctrl Pts',(201.860140564039,-4.91824790150174,
130.799817284683));
#208477=CARTESIAN_POINT('Origin',(213.235140564004,0.,130.804360617566));
#208478=CARTESIAN_POINT('',(203.680274487341,-4.76405452823405,129.582490119308));
#208479=CARTESIAN_POINT('',(203.334773566427,-4.76405452823405,129.582490119308));
#208480=CARTESIAN_POINT('',(213.235140564004,-4.76405452823405,129.582490119308));
#208481=CARTESIAN_POINT('',(203.264859436027,-4.91824791911963,130.799836396593));
#208482=CARTESIAN_POINT('Ctrl Pts',(203.334773566427,-4.76405452823405,
129.582490119308));
#208483=CARTESIAN_POINT('Ctrl Pts',(203.32473014209,-4.80784291725373,129.753220383514));
#208484=CARTESIAN_POINT('Ctrl Pts',(203.314686717754,-4.84247434312161,
129.926402595191));
#208485=CARTESIAN_POINT('Ctrl Pts',(203.304643293417,-4.86772242676584,
130.101181096774));
#208486=CARTESIAN_POINT('Ctrl Pts',(203.294796401501,-4.89247644913987,
130.272539485777));
#208487=CARTESIAN_POINT('Ctrl Pts',(203.284949509584,-4.90821079695266,
130.445432509572));
#208488=CARTESIAN_POINT('Ctrl Pts',(203.275102617668,-4.91475699054651,
130.619031757498));
#208489=CARTESIAN_POINT('Ctrl Pts',(203.271688223788,-4.9170268726106,130.679227016553));
#208490=CARTESIAN_POINT('Ctrl Pts',(203.268273829907,-4.91819242300989,
130.739506976807));
#208491=CARTESIAN_POINT('Ctrl Pts',(203.264859436027,-4.91824791911963,
130.799836396593));
#208492=CARTESIAN_POINT('Ctrl Pts',(203.264859435991,-4.91824791912021,
130.799836397221));
#208493=CARTESIAN_POINT('Ctrl Pts',(203.257189383465,-4.91837258488303,
130.935359665711));
#208494=CARTESIAN_POINT('Ctrl Pts',(203.249519330939,-4.91289148263668,
131.071020543707));
#208495=CARTESIAN_POINT('Ctrl Pts',(203.241849278414,-4.90179734488421,
131.206313167236));
#208496=CARTESIAN_POINT('Ctrl Pts',(203.234183418891,-4.89070927198605,
131.341531830077));
#208497=CARTESIAN_POINT('Ctrl Pts',(203.226517559368,-4.8740142988451,131.476382241115));
#208498=CARTESIAN_POINT('Ctrl Pts',(203.218851699845,-4.85175723294996,
131.610359882465));
#208499=CARTESIAN_POINT('Ctrl Pts',(203.211187985896,-4.82950639651798,
131.744300025216));
#208500=CARTESIAN_POINT('Ctrl Pts',(203.203524271947,-4.80169662793145,
131.877367489554));
#208501=CARTESIAN_POINT('Ctrl Pts',(203.195860557999,-4.76842439234139,
132.009064679576));
#208502=CARTESIAN_POINT('Ctrl Pts',(203.18819724317,-4.73515388954357,132.140755010911));
#208503=CARTESIAN_POINT('Ctrl Pts',(203.180533928342,-4.69642158345535,
132.271074821851));
#208504=CARTESIAN_POINT('Ctrl Pts',(203.172870613514,-4.6523745561182,132.399538993825));
#208505=CARTESIAN_POINT('Ctrl Pts',(203.165205951912,-4.60831978783102,
132.528025742458));
#208506=CARTESIAN_POINT('Ctrl Pts',(203.157541290311,-4.55894857073882,
132.654655825109));
#208507=CARTESIAN_POINT('Ctrl Pts',(203.14987662871,-4.50445695066178,132.778962005729));
#208508=CARTESIAN_POINT('Ctrl Pts',(203.142204113634,-4.44990949660173,
132.903395554725));
#208509=CARTESIAN_POINT('Ctrl Pts',(203.134531598558,-4.39023132120439,
133.025500078541));
#208510=CARTESIAN_POINT('Ctrl Pts',(203.126859083481,-4.32566565593964,
133.144830590782));
#208511=CARTESIAN_POINT('Ctrl Pts',(203.119182649825,-4.26106701508398,
133.264222048637));
#208512=CARTESIAN_POINT('Ctrl Pts',(203.111506216169,-4.19157611789148,
133.380836329876));
#208513=CARTESIAN_POINT('Ctrl Pts',(203.103829782513,-4.11748010840755,
133.494256641461));
#208514=CARTESIAN_POINT('Ctrl Pts',(203.096141011026,-4.04326500925227,
133.607859246098));
#208515=CARTESIAN_POINT('Ctrl Pts',(203.08845223954,-3.9644302428689,133.718257299233));
#208516=CARTESIAN_POINT('Ctrl Pts',(203.080763468054,-3.88130435803297,
133.825065757565));
#208517=CARTESIAN_POINT('Ctrl Pts',(203.073308445649,-3.80070561283009,
133.928627093911));
#208518=CARTESIAN_POINT('Ctrl Pts',(203.065853423243,-3.71607313595503,
134.028813718384));
#208519=CARTESIAN_POINT('Ctrl Pts',(203.058398400838,-3.62773852230693,
134.125308716569));
#208520=CARTESIAN_POINT('Ctrl Pts',(203.050624066711,-3.53562038179653,
134.225936765238));
#208521=CARTESIAN_POINT('Ctrl Pts',(203.042849732584,-3.43916625203493,
134.322888467361));
#208522=CARTESIAN_POINT('Ctrl Pts',(203.035075398457,-3.33870121485528,
134.415767166326));
#208523=CARTESIAN_POINT('Ctrl Pts',(203.027310645502,-3.23835999185389,
134.508531400596));
#208524=CARTESIAN_POINT('Ctrl Pts',(203.019545892547,-3.13401798102474,
134.597232356386));
#208525=CARTESIAN_POINT('Ctrl Pts',(203.011781139593,-3.026039452382,134.68150754477));
#208526=CARTESIAN_POINT('Ctrl Pts',(203.0040240987,-2.91816816953492,134.76569902985));
#208527=CARTESIAN_POINT('Ctrl Pts',(202.996267057807,-2.80666786281095,
134.845473256243));
#208528=CARTESIAN_POINT('Ctrl Pts',(202.988510016914,-2.69193820449843,
134.920505873222));
#208529=CARTESIAN_POINT('Ctrl Pts',(202.980758825666,-2.57729506471272,
134.995481907523));
#208530=CARTESIAN_POINT('Ctrl Pts',(202.973007634418,-2.45942774649362,
135.065723236469));
#208531=CARTESIAN_POINT('Ctrl Pts',(202.96525644317,-2.33876713339567,135.130947188784));
#208532=CARTESIAN_POINT('Ctrl Pts',(202.957508546385,-2.21815780427522,
135.196143419181));
#208533=CARTESIAN_POINT('Ctrl Pts',(202.949760649599,-2.09475788478772,
135.256326328838));
#208534=CARTESIAN_POINT('Ctrl Pts',(202.942012752814,-1.96902504732344,
135.311257934514));
#208535=CARTESIAN_POINT('Ctrl Pts',(202.934266476722,-1.84331851045724,
135.366178049683));
#208536=CARTESIAN_POINT('Ctrl Pts',(202.92652020063,-1.71528038430399,135.415848889344));
#208537=CARTESIAN_POINT('Ctrl Pts',(202.918773924538,-1.58539025926972,
135.460079765916));
#208538=CARTESIAN_POINT('Ctrl Pts',(202.911027591264,-1.45549917541524,
135.504310968991));
#208539=CARTESIAN_POINT('Ctrl Pts',(202.903281257991,-1.32375643549607,
135.54310200282));
#208540=CARTESIAN_POINT('Ctrl Pts',(202.895534924717,-1.19065842226258,
135.576311537682));
#208541=CARTESIAN_POINT('Ctrl Pts',(202.887786856706,-1.05753060265117,
135.609528509589));
#208542=CARTESIAN_POINT('Ctrl Pts',(202.880038788695,-0.923047285050385,
135.637161400668));
#208543=CARTESIAN_POINT('Ctrl Pts',(202.872290720684,-0.787716324822747,
135.659119731478));
#208544=CARTESIAN_POINT('Ctrl Pts',(202.864534417934,-0.65224153324019,
135.681101399863));
#208545=CARTESIAN_POINT('Ctrl Pts',(202.856778115184,-0.515917685950118,
135.697396397709));
#208546=CARTESIAN_POINT('Ctrl Pts',(202.849021812434,-0.379259621354758,
135.707965944477));
#208547=CARTESIAN_POINT('Ctrl Pts',(202.841261369911,-0.242528618235135,
135.71854113253));
#208548=CARTESIAN_POINT('Ctrl Pts',(202.833500927389,-0.105463432899442,
135.723384766673));
#208549=CARTESIAN_POINT('Ctrl Pts',(202.825740484867,0.0314207805563875,
135.722510248987));
#208550=CARTESIAN_POINT('Ctrl Pts',(202.817967584593,0.168524732702548,
135.721634327448));
#208551=CARTESIAN_POINT('Ctrl Pts',(202.810194684319,0.305446741698207,
135.715021929815));
#208552=CARTESIAN_POINT('Ctrl Pts',(202.802421784046,0.441675557289912,
135.70273848831));
#208553=CARTESIAN_POINT('Ctrl Pts',(202.794931448372,0.572952110607848,
135.690901580996));
#208554=CARTESIAN_POINT('Ctrl Pts',(202.787441112698,0.703584688784279,
135.673798825022));
#208555=CARTESIAN_POINT('Ctrl Pts',(202.779950777025,0.833126405809881,
135.651533345502));
#208556=CARTESIAN_POINT('Ctrl Pts',(202.772176442908,0.96757973795983,135.628423663291));
#208557=CARTESIAN_POINT('Ctrl Pts',(202.764402108791,1.10128376375181,135.599678835429));
#208558=CARTESIAN_POINT('Ctrl Pts',(202.756627774674,1.23372905007338,135.565357959878));
#208559=CARTESIAN_POINT('Ctrl Pts',(202.748863021729,1.36601110941638,135.53107938174));
#208560=CARTESIAN_POINT('Ctrl Pts',(202.741098268784,1.49703714105001,135.491238526238));
#208561=CARTESIAN_POINT('Ctrl Pts',(202.733333515839,1.62630527593573,135.445945929931));
#208562=CARTESIAN_POINT('Ctrl Pts',(202.725576474956,1.75544501988741,135.40069831887));
#208563=CARTESIAN_POINT('Ctrl Pts',(202.717819434073,1.88282997506119,135.350009871036));
#208564=CARTESIAN_POINT('Ctrl Pts',(202.710062393191,2.00797122337188,135.294041522554));
#208565=CARTESIAN_POINT('Ctrl Pts',(202.702311201953,2.13301810169324,135.238115380238));
#208566=CARTESIAN_POINT('Ctrl Pts',(202.694560010715,2.25582428551557,135.17691742141));
#208567=CARTESIAN_POINT('Ctrl Pts',(202.686808819477,2.37591905240151,135.110657369874));
#208568=CARTESIAN_POINT('Ctrl Pts',(202.679060922702,2.49596277580801,135.044425480627));
#208569=CARTESIAN_POINT('Ctrl Pts',(202.671313025927,2.61329703275995,134.973135966364));
#208570=CARTESIAN_POINT('Ctrl Pts',(202.663565129152,2.72747421811156,134.897045244072));
#208571=CARTESIAN_POINT('Ctrl Pts',(202.65581885307,2.84162752005722,134.820970438319));
#208572=CARTESIAN_POINT('Ctrl Pts',(202.648072576988,2.95262473882447,134.740096638841));
#208573=CARTESIAN_POINT('Ctrl Pts',(202.640326300906,3.06004621322242,134.654724267332));
#208574=CARTESIAN_POINT('Ctrl Pts',(202.632579967643,3.1674684805811,134.569351265625));
#208575=CARTESIAN_POINT('Ctrl Pts',(202.62483363438,3.27131464482454,134.479479868875));
#208576=CARTESIAN_POINT('Ctrl Pts',(202.617087301116,3.37119749425472,134.385451305782));
#208577=CARTESIAN_POINT('Ctrl Pts',(202.609339233116,3.47110271175664,134.291401685645));
#208578=CARTESIAN_POINT('Ctrl Pts',(202.601591165115,3.56704256369362,134.193193314579));
#208579=CARTESIAN_POINT('Ctrl Pts',(202.593843097114,3.65866641892285,134.091204559335));
#208580=CARTESIAN_POINT('Ctrl Pts',(202.586086794374,3.75038765307602,133.989107409229));
#208581=CARTESIAN_POINT('Ctrl Pts',(202.578330491635,3.83778346561284,133.883222140185));
#208582=CARTESIAN_POINT('Ctrl Pts',(202.570574188895,3.92054294663494,133.7739609385));
#208583=CARTESIAN_POINT('Ctrl Pts',(202.562813746383,4.00334659888406,133.664641420822));
#208584=CARTESIAN_POINT('Ctrl Pts',(202.555053303871,4.08150876616667,133.551942701296));
#208585=CARTESIAN_POINT('Ctrl Pts',(202.547292861359,4.15476227066247,133.436305437804));
#208586=CARTESIAN_POINT('Ctrl Pts',(202.539519961095,4.22813336818707,133.320482543111));
#208587=CARTESIAN_POINT('Ctrl Pts',(202.531747060832,4.29657986120505,133.201712016897));
#208588=CARTESIAN_POINT('Ctrl Pts',(202.523974160569,4.35988045644892,133.080459356192));
#208589=CARTESIAN_POINT('Ctrl Pts',(202.516483824783,4.42087991581972,132.963614534721));
#208590=CARTESIAN_POINT('Ctrl Pts',(202.508993488998,4.47710098314102,132.844465187877));
#208591=CARTESIAN_POINT('Ctrl Pts',(202.501503153212,4.52838886767896,132.723443035176));
#208592=CARTESIAN_POINT('Ctrl Pts',(202.493728819094,4.58162134777368,132.597832291183));
#208593=CARTESIAN_POINT('Ctrl Pts',(202.485954484976,4.62970780184522,132.46980602598));
#208594=CARTESIAN_POINT('Ctrl Pts',(202.478180150858,4.67242258964327,132.339824783964));
#208595=CARTESIAN_POINT('Ctrl Pts',(202.470415397911,4.7150847352829,132.210003732212));
#208596=CARTESIAN_POINT('Ctrl Pts',(202.462650644965,4.75238826578558,132.078232865362));
#208597=CARTESIAN_POINT('Ctrl Pts',(202.454885892019,4.78415490621555,131.944994167762));
#208598=CARTESIAN_POINT('Ctrl Pts',(202.447128851135,4.81588999557021,131.811887804716));
#208599=CARTESIAN_POINT('Ctrl Pts',(202.439371810251,4.8420990486564,131.677316889991));
#208600=CARTESIAN_POINT('Ctrl Pts',(202.431614769367,4.86265319342588,131.541779754126));
#208601=CARTESIAN_POINT('Ctrl Pts',(202.423863578128,4.88319183815493,131.406344827869));
#208602=CARTESIAN_POINT('Ctrl Pts',(202.416112386889,4.89808400423516,131.269945515757));
#208603=CARTESIAN_POINT('Ctrl Pts',(202.40836119565,4.90725170126882,131.133091210749));
#208604=CARTESIAN_POINT('Ctrl Pts',(202.400613298874,4.91641550178662,130.996295072471));
#208605=CARTESIAN_POINT('Ctrl Pts',(202.392865402097,4.91985964633597,130.859044715197));
#208606=CARTESIAN_POINT('Ctrl Pts',(202.385117505321,4.91755792427646,130.721855321458));
#208607=CARTESIAN_POINT('Ctrl Pts',(202.377371229238,4.91525668368759,130.584694624784));
#208608=CARTESIAN_POINT('Ctrl Pts',(202.369624953155,4.907211973712,130.447595256941));
#208609=CARTESIAN_POINT('Ctrl Pts',(202.361878677072,4.89344971050554,130.311072676042));
#208610=CARTESIAN_POINT('Ctrl Pts',(202.354132343808,4.8796873457092,130.174549087364));
#208611=CARTESIAN_POINT('Ctrl Pts',(202.346386010544,4.86020738267642,130.038602683118));
#208612=CARTESIAN_POINT('Ctrl Pts',(202.338639677279,4.83508760939448,129.903743677918));
#208613=CARTESIAN_POINT('Ctrl Pts',(202.330891609277,4.80996221071351,129.76885447198));
#208614=CARTESIAN_POINT('Ctrl Pts',(202.323143541275,4.77919456014558,129.635053533938));
#208615=CARTESIAN_POINT('Ctrl Pts',(202.315395473273,4.74291346365742,129.502840376172));
#208616=CARTESIAN_POINT('Ctrl Pts',(202.307639170533,4.70659380718827,129.37048670069));
#208617=CARTESIAN_POINT('Ctrl Pts',(202.299882867792,4.66474910293164,129.239724554101));
#208618=CARTESIAN_POINT('Ctrl Pts',(202.292126565051,4.6175580804997,129.111038310469));
#208619=CARTESIAN_POINT('Ctrl Pts',(202.284366122538,4.57034187079823,128.982283383115));
#208620=CARTESIAN_POINT('Ctrl Pts',(202.276605680025,4.51777380687754,128.855606927377));
#208621=CARTESIAN_POINT('Ctrl Pts',(202.268845237512,4.46008021055639,128.731471913872));
#208622=CARTESIAN_POINT('Ctrl Pts',(202.261072337248,4.40229399935262,128.607137627823));
#208623=CARTESIAN_POINT('Ctrl Pts',(202.253299436983,4.33936599324112,128.485353284181));
#208624=CARTESIAN_POINT('Ctrl Pts',(202.245526536719,4.27156821364134,128.366556675755));
#208625=CARTESIAN_POINT('Ctrl Pts',(202.238036200946,4.20623505399508,128.252078623088));
#208626=CARTESIAN_POINT('Ctrl Pts',(202.230545865172,4.13638019427766,128.140375114719));
#208627=CARTESIAN_POINT('Ctrl Pts',(202.223055529399,4.06228318417237,128.03180973542));
#208628=CARTESIAN_POINT('Ctrl Pts',(202.215281195279,3.98537676351187,127.919128066919));
#208629=CARTESIAN_POINT('Ctrl Pts',(202.207506861159,3.90365654367928,127.80947024764));
#208630=CARTESIAN_POINT('Ctrl Pts',(202.199732527038,3.81738802965387,127.703275050614));
#208631=CARTESIAN_POINT('Ctrl Pts',(202.19196777409,3.73122583386185,127.597210729678));
#208632=CARTESIAN_POINT('Ctrl Pts',(202.184203021142,3.64052674103213,127.494600840736));
#208633=CARTESIAN_POINT('Ctrl Pts',(202.176438268194,3.54559989628898,127.395855895854));
#208634=CARTESIAN_POINT('Ctrl Pts',(202.168681227307,3.45076733422572,127.297209025842));
#208635=CARTESIAN_POINT('Ctrl Pts',(202.160924186421,3.35171564577153,127.202419740696));
#208636=CARTESIAN_POINT('Ctrl Pts',(202.153167145535,3.24879443203218,127.111865823948));
#208637=CARTESIAN_POINT('Ctrl Pts',(202.145415954294,3.14595083198053,127.021380194613));
#208638=CARTESIAN_POINT('Ctrl Pts',(202.137664763052,3.03924380716249,126.935123833573));
#208639=CARTESIAN_POINT('Ctrl Pts',(202.129913571811,2.92905976858584,126.853437695697));
#208640=CARTESIAN_POINT('Ctrl Pts',(202.122165675033,2.818922561165,126.771786276608));
#208641=CARTESIAN_POINT('Ctrl Pts',(202.114417778254,2.70531159267622,126.694701449615));
#208642=CARTESIAN_POINT('Ctrl Pts',(202.106669881476,2.58864613328299,126.622483735215));
#208643=CARTESIAN_POINT('Ctrl Pts',(202.098923605391,2.47200507778859,126.550281127204));
#208644=CARTESIAN_POINT('Ctrl Pts',(202.091177329306,2.35231113448206,126.482943812387));
#208645=CARTESIAN_POINT('Ctrl Pts',(202.08343105322,2.23001198118519,126.420728604467));
#208646=CARTESIAN_POINT('Ctrl Pts',(202.075684719954,2.10771192510372,126.358512937288));
#208647=CARTESIAN_POINT('Ctrl Pts',(202.067938386687,1.98280696912467,126.301419629723));
#208648=CARTESIAN_POINT('Ctrl Pts',(202.060192053421,1.85576841756085,126.249659019999));
#208649=CARTESIAN_POINT('Ctrl Pts',(202.052443985416,1.7287014165942,126.197886818844));
#208650=CARTESIAN_POINT('Ctrl Pts',(202.044695917412,1.5995002312647,126.151449839382));
#208651=CARTESIAN_POINT('Ctrl Pts',(202.036947849408,1.46865473825808,126.110509712148));
#208652=CARTESIAN_POINT('Ctrl Pts',(202.029191546665,1.33767018110433,126.06952607326));
#208653=CARTESIAN_POINT('Ctrl Pts',(202.021435243922,1.20503819899675,126.034051073798));
#208654=CARTESIAN_POINT('Ctrl Pts',(202.013678941179,1.07126291727623,126.004196159491));
#208655=CARTESIAN_POINT('Ctrl Pts',(202.005918498663,0.937416235660115,
125.974325310717));
#208656=CARTESIAN_POINT('Ctrl Pts',(201.998158056148,0.802425423148925,
125.950080593152));
#208657=CARTESIAN_POINT('Ctrl Pts',(201.990397613633,0.666802322505834,
125.931521842765));
#208658=CARTESIAN_POINT('Ctrl Pts',(201.982624713366,0.530961507621308,
125.912933300225));
#208659=CARTESIAN_POINT('Ctrl Pts',(201.974851813099,0.394486765759838,
125.900049001524));
#208660=CARTESIAN_POINT('Ctrl Pts',(201.967078912833,0.257893458632686,
125.892876725045));
#208661=CARTESIAN_POINT('Ctrl Pts',(201.959588577084,0.126265662529295,
125.885965178895));
#208662=CARTESIAN_POINT('Ctrl Pts',(201.952098241335,-0.00547192021256673,
125.884357576005));
#208663=CARTESIAN_POINT('Ctrl Pts',(201.944607905586,-0.136862291999976,
125.888015249762));
#208664=CARTESIAN_POINT('Ctrl Pts',(201.936833571467,-0.273234369901628,
125.891811605337));
#208665=CARTESIAN_POINT('Ctrl Pts',(201.929059237349,-0.409664373849437,
125.901292410854));
#208666=CARTESIAN_POINT('Ctrl Pts',(201.92128490323,-0.545639639740232,
125.916471456993));
#208667=CARTESIAN_POINT('Ctrl Pts',(201.913520150283,-0.681447328268266,
125.931631796315));
#208668=CARTESIAN_POINT('Ctrl Pts',(201.905755397337,-0.816801008994345,
125.952476360477));
#208669=CARTESIAN_POINT('Ctrl Pts',(201.89799064439,-0.951188206001152,
125.978966948728));
#208670=CARTESIAN_POINT('Ctrl Pts',(201.890233603505,-1.08544192774853,
126.005431226153));
#208671=CARTESIAN_POINT('Ctrl Pts',(201.882476562621,-1.21873069496959,
126.037530292947));
#208672=CARTESIAN_POINT('Ctrl Pts',(201.874719521736,-1.35054769974211,
126.075174221026));
#208673=CARTESIAN_POINT('Ctrl Pts',(201.866968330497,-1.48226530028765,
126.112789761526));
#208674=CARTESIAN_POINT('Ctrl Pts',(201.859217139257,-1.6125129730937,126.155941733518));
#208675=CARTESIAN_POINT('Ctrl Pts',(201.851465948017,-1.74079499858619,
126.204489332911));
#208676=CARTESIAN_POINT('Ctrl Pts',(201.84371805124,-1.86902250079471,126.253016298278));
#208677=CARTESIAN_POINT('Ctrl Pts',(201.835970154464,-1.99528565245025,
126.306934191786));
#208678=CARTESIAN_POINT('Ctrl Pts',(201.828222257687,-2.11910499138351,
126.366052708239));
#208679=CARTESIAN_POINT('Ctrl Pts',(201.820475981603,-2.24289842998043,
126.425158858373));
#208680=CARTESIAN_POINT('Ctrl Pts',(201.81272970552,-2.36424872005608,126.489463299298));
#208681=CARTESIAN_POINT('Ctrl Pts',(201.804983429436,-2.48269781617095,
126.558728201061));
#208682=CARTESIAN_POINT('Ctrl Pts',(201.797237096171,-2.60114778665004,
126.627993614122));
#208683=CARTESIAN_POINT('Ctrl Pts',(201.789490762906,-2.71669618293738,
126.702219363732));
#208684=CARTESIAN_POINT('Ctrl Pts',(201.781744429641,-2.82891129003388,
126.781122621173));
#208685=CARTESIAN_POINT('Ctrl Pts',(201.773996361638,-2.94115152692565,
126.860043548452));
#208686=CARTESIAN_POINT('Ctrl Pts',(201.766248293636,-3.05005666948663,
126.943643843122));
#208687=CARTESIAN_POINT('Ctrl Pts',(201.758500225633,-3.15522594305475,
127.031598723307));
#208688=CARTESIAN_POINT('Ctrl Pts',(201.750743922892,-3.26050699177834,
127.119647082985));
#208689=CARTESIAN_POINT('Ctrl Pts',(201.74298762015,-3.36204393957021,127.212059022098));
#208690=CARTESIAN_POINT('Ctrl Pts',(201.735231317409,-3.45947053192138,
127.30847064486));
#208691=CARTESIAN_POINT('Ctrl Pts',(201.727470874895,-3.55694912377835,
127.404933725407));
#208692=CARTESIAN_POINT('Ctrl Pts',(201.719710432381,-3.65031272280732,
127.505400457023));
#208693=CARTESIAN_POINT('Ctrl Pts',(201.711949989868,-3.73923432379541,
127.609472554699));
#208694=CARTESIAN_POINT('Ctrl Pts',(201.704177089603,-3.82829866963167,
127.713711718145));
#208695=CARTESIAN_POINT('Ctrl Pts',(201.696404189338,-3.9129065265913,127.821567505439));
#208696=CARTESIAN_POINT('Ctrl Pts',(201.688631289073,-3.99277278490735,
127.932610532582));
#208697=CARTESIAN_POINT('Ctrl Pts',(201.681140953306,-4.06973570361064,
128.039616866056));
#208698=CARTESIAN_POINT('Ctrl Pts',(201.67365061754,-4.14229560697238,128.14958247704));
#208699=CARTESIAN_POINT('Ctrl Pts',(201.666160281774,-4.21023800794793,
128.262101980265));
#208700=CARTESIAN_POINT('Ctrl Pts',(201.658128312424,-4.28309339110042,
128.382757879996));
#208701=CARTESIAN_POINT('Ctrl Pts',(201.650096343074,-4.35085732043947,
128.506711456361));
#208702=CARTESIAN_POINT('Ctrl Pts',(201.642064373724,-4.41322893384724,
128.633509761345));
#208703=CARTESIAN_POINT('Ctrl Pts',(201.634043232433,-4.47551646283025,
128.760137126988));
#208704=CARTESIAN_POINT('Ctrl Pts',(201.626022091142,-4.53242599296163,
128.889601270105));
#208705=CARTESIAN_POINT('Ctrl Pts',(201.618000949852,-4.58370062266684,
129.021421565253));
#208706=CARTESIAN_POINT('Ctrl Pts',(201.609992618133,-4.63489336800769,
129.153031346524));
#208707=CARTESIAN_POINT('Ctrl Pts',(201.601984286414,-4.68046901878164,
129.286989451782));
#208708=CARTESIAN_POINT('Ctrl Pts',(201.593975954695,-4.72021745497381,
129.422792580783));
#208709=CARTESIAN_POINT('Ctrl Pts',(201.590852754914,-4.73571909895888,
129.475754960174));
#208710=CARTESIAN_POINT('Ctrl Pts',(201.587729555133,-4.75033495592387,
129.528997715094));
#208711=CARTESIAN_POINT('Ctrl Pts',(201.584606355351,-4.76405452823405,
129.582490119308));
#208712=CARTESIAN_POINT('',(203.610140564065,-4.91824975435206,130.805915067923));
#208713=CARTESIAN_POINT('Ctrl Pts',(203.610140564008,-4.91824975435174,
130.80591506892));
#208714=CARTESIAN_POINT('Ctrl Pts',(203.60532859344,-4.91822305432427,130.890393366163));
#208715=CARTESIAN_POINT('Ctrl Pts',(203.600516622872,-4.91601993127815,
130.974834611061));
#208716=CARTESIAN_POINT('Ctrl Pts',(203.595704652304,-4.91164526425146,
131.059162227954));
#208717=CARTESIAN_POINT('Ctrl Pts',(203.587930318251,-4.90457744819619,
131.195403930679));
#208718=CARTESIAN_POINT('Ctrl Pts',(203.580155984198,-4.89182542922343,
131.331567131691));
#208719=CARTESIAN_POINT('Ctrl Pts',(203.572381650145,-4.87338772313762,
131.467138983592));
#208720=CARTESIAN_POINT('Ctrl Pts',(203.564616897265,-4.85497273987956,
131.60254375528));
#208721=CARTESIAN_POINT('Ctrl Pts',(203.556852144384,-4.83088606373339,
131.737358244241));
#208722=CARTESIAN_POINT('Ctrl Pts',(203.549087391504,-4.80117818244719,
131.871071038858));
#208723=CARTESIAN_POINT('Ctrl Pts',(203.541330350687,-4.77149980745165,
132.004651028024));
#208724=CARTESIAN_POINT('Ctrl Pts',(203.53357330987,-4.73621142210639,132.1371311212));
#208725=CARTESIAN_POINT('Ctrl Pts',(203.525816269053,-4.69541509058143,
132.268006814446));
#208726=CARTESIAN_POINT('Ctrl Pts',(203.518065077882,-4.65464952389258,
132.398783813296));
#208727=CARTESIAN_POINT('Ctrl Pts',(203.510313886711,-4.60838439436307,
132.527958448688));
#208728=CARTESIAN_POINT('Ctrl Pts',(203.50256269554,-4.55677236142872,132.655038522718));
#208729=CARTESIAN_POINT('Ctrl Pts',(203.494814798833,-4.50518226499348,
132.782064584306));
#208730=CARTESIAN_POINT('Ctrl Pts',(203.487066902126,-4.44824993194415,
132.906997493689));
#208731=CARTESIAN_POINT('Ctrl Pts',(203.479319005419,-4.38617711843204,
133.029362493575));
#208732=CARTESIAN_POINT('Ctrl Pts',(203.471572729406,-4.32411728922029,
133.151701897329));
#208733=CARTESIAN_POINT('Ctrl Pts',(203.463826453393,-4.25691929509247,
133.271474111561));
#208734=CARTESIAN_POINT('Ctrl Pts',(203.456080177379,-4.18483188932866,
133.388226930005));
#208735=CARTESIAN_POINT('Ctrl Pts',(203.448333844186,-4.11274395143813,
133.504980610282));
#208736=CARTESIAN_POINT('Ctrl Pts',(203.440587510992,-4.03576673529106,
133.618714517632));
#208737=CARTESIAN_POINT('Ctrl Pts',(203.432841177798,-3.95419334811849,
133.729003848491));
#208738=CARTESIAN_POINT('Ctrl Pts',(203.425093109867,-3.87260169315755,
133.839317877873));
#208739=CARTESIAN_POINT('Ctrl Pts',(203.417345041936,-3.78641205146594,
133.946185481521));
#208740=CARTESIAN_POINT('Ctrl Pts',(203.409596974005,-3.69595872886982,
134.049213794058));
#208741=CARTESIAN_POINT('Ctrl Pts',(203.401840671336,-3.60540927141139,
134.152351606306));
#208742=CARTESIAN_POINT('Ctrl Pts',(203.394084368667,-3.51058733926155,
134.251641682045));
#208743=CARTESIAN_POINT('Ctrl Pts',(203.386328065998,-3.41186551250551,
134.346726604738));
#208744=CARTESIAN_POINT('Ctrl Pts',(203.378567623557,-3.3130909949427,134.441862277113));
#208745=CARTESIAN_POINT('Ctrl Pts',(203.370807181116,-3.21041272778059,
134.532788065183));
#208746=CARTESIAN_POINT('Ctrl Pts',(203.363046738675,-3.10423672854745,
134.619186615647));
#208747=CARTESIAN_POINT('Ctrl Pts',(203.355273838482,-2.99789028617232,
134.705723860737));
#208748=CARTESIAN_POINT('Ctrl Pts',(203.34750093829,-2.8880352049204,134.787719111404));
#208749=CARTESIAN_POINT('Ctrl Pts',(203.339728038097,-2.77510758697802,
134.864897644019));
#208750=CARTESIAN_POINT('Ctrl Pts',(203.332237701562,-2.66628516014054,
134.939270550948));
#208751=CARTESIAN_POINT('Ctrl Pts',(203.324747365027,-2.55460996759745,
135.009170695082));
#208752=CARTESIAN_POINT('Ctrl Pts',(203.317257028492,-2.44049242510876,
135.074393379207));
#208753=CARTESIAN_POINT('Ctrl Pts',(203.309482694322,-2.32204809275828,
135.142088994682));
#208754=CARTESIAN_POINT('Ctrl Pts',(203.301708360151,-2.20059735556435,
135.204959896962));
#208755=CARTESIAN_POINT('Ctrl Pts',(203.293934025981,-2.0765708843453,135.262727630811));
#208756=CARTESIAN_POINT('Ctrl Pts',(203.286169272982,-1.95269726465683,
135.320424171095));
#208757=CARTESIAN_POINT('Ctrl Pts',(203.278404519984,-1.82625457798257,
135.373029893092));
#208758=CARTESIAN_POINT('Ctrl Pts',(203.270639766985,-1.69770037928056,
135.420310843109));
#208759=CARTESIAN_POINT('Ctrl Pts',(203.262882726048,-1.56927386241116,
135.467544833023));
#208760=CARTESIAN_POINT('Ctrl Pts',(203.25512568511,-1.43874037156367,135.509464441505));
#208761=CARTESIAN_POINT('Ctrl Pts',(203.247368644173,-1.30657952838765,
135.545882841335));
#208762=CARTESIAN_POINT('Ctrl Pts',(203.23961745288,-1.1745183487227,135.582273777769));
#208763=CARTESIAN_POINT('Ctrl Pts',(203.231866261587,-1.04083263478582,
135.613171659453));
#208764=CARTESIAN_POINT('Ctrl Pts',(203.224115070294,-0.906019002783906,
135.638438878113));
#208765=CARTESIAN_POINT('Ctrl Pts',(203.216367173464,-0.771262670161606,
135.663695357533));
#208766=CARTESIAN_POINT('Ctrl Pts',(203.208619276634,-0.635379756424377,
135.683325861913));
#208767=CARTESIAN_POINT('Ctrl Pts',(203.200871379803,-0.498878742470774,
135.697243516513));
#208768=CARTESIAN_POINT('Ctrl Pts',(203.193125103666,-0.362406281580614,
135.711158259841));
#208769=CARTESIAN_POINT('Ctrl Pts',(203.185378827528,-0.22531636634765,
135.719362490687));
#208770=CARTESIAN_POINT('Ctrl Pts',(203.17763255139,-0.0881239079495214,
135.721821063706));
#208771=CARTESIAN_POINT('Ctrl Pts',(203.169886218071,0.0490695631770811,
135.724279654873));
#208772=CARTESIAN_POINT('Ctrl Pts',(203.162139884752,0.186365188076857,
135.720992496577));
#208773=CARTESIAN_POINT('Ctrl Pts',(203.154393551432,0.323247135849997,
135.711976571536));
#208774=CARTESIAN_POINT('Ctrl Pts',(203.146645483375,0.4601597373901,135.702958627442));
#208775=CARTESIAN_POINT('Ctrl Pts',(203.138897415318,0.596658087415218,
135.688209389437));
#208776=CARTESIAN_POINT('Ctrl Pts',(203.131149347261,0.73223095668038,135.667797765158));
#208777=CARTESIAN_POINT('Ctrl Pts',(203.123393044465,0.867947914404447,
135.647364447162));
#208778=CARTESIAN_POINT('Ctrl Pts',(203.115636741669,1.00273703927327,135.621256779485));
#208779=CARTESIAN_POINT('Ctrl Pts',(203.107880438873,1.13609623798184,135.589595031944));
#208780=CARTESIAN_POINT('Ctrl Pts',(203.100119996304,1.26952661451173,135.557916385574));
#208781=CARTESIAN_POINT('Ctrl Pts',(203.092359553736,1.40152516805726,135.520677858664));
#208782=CARTESIAN_POINT('Ctrl Pts',(203.084599111167,1.53160543789726,135.478049508057));
#208783=CARTESIAN_POINT('Ctrl Pts',(203.076826210848,1.66189452412713,135.435352726641));
#208784=CARTESIAN_POINT('Ctrl Pts',(203.069053310528,1.79025880671704,135.387248968902));
#208785=CARTESIAN_POINT('Ctrl Pts',(203.061280410209,1.9162314290031,135.333956645139));
#208786=CARTESIAN_POINT('Ctrl Pts',(203.053790075032,2.03762461883292,135.282601635949));
#208787=CARTESIAN_POINT('Ctrl Pts',(203.046299739856,2.15679673695984,135.226428878422));
#208788=CARTESIAN_POINT('Ctrl Pts',(203.038809404679,2.27335372629928,135.16567302298));
#208789=CARTESIAN_POINT('Ctrl Pts',(203.031035070571,2.39433001860291,135.102613585972));
#208790=CARTESIAN_POINT('Ctrl Pts',(203.023260736462,2.51287217837938,135.034416900165));
#208791=CARTESIAN_POINT('Ctrl Pts',(203.015486402354,2.62851314525934,134.961294789248));
#208792=CARTESIAN_POINT('Ctrl Pts',(203.007721649418,2.74401159498189,134.888262794799));
#208793=CARTESIAN_POINT('Ctrl Pts',(202.999956896482,2.85661563863572,134.810317659964));
#208794=CARTESIAN_POINT('Ctrl Pts',(202.992192143545,2.96588112472585,134.727717880994));
#208795=CARTESIAN_POINT('Ctrl Pts',(202.984435102671,3.07503808679438,134.64520014129));
#208796=CARTESIAN_POINT('Ctrl Pts',(202.976678061797,3.18086278023441,134.558037191785));
#208797=CARTESIAN_POINT('Ctrl Pts',(202.968921020923,3.28293877480054,134.466531567073));
#208798=CARTESIAN_POINT('Ctrl Pts',(202.961169829694,3.38493779306489,134.375094947464));
#208799=CARTESIAN_POINT('Ctrl Pts',(202.953418638464,3.483193449336,134.279322430943));
#208800=CARTESIAN_POINT('Ctrl Pts',(202.945667447235,3.57732153668663,134.179557454146));
#208801=CARTESIAN_POINT('Ctrl Pts',(202.937919550469,3.67140961708933,134.079834880125));
#208802=CARTESIAN_POINT('Ctrl Pts',(202.930171653703,3.76137335005203,133.976123504614));
#208803=CARTESIAN_POINT('Ctrl Pts',(202.922423756936,3.84686479905085,133.868804169065));
#208804=CARTESIAN_POINT('Ctrl Pts',(202.914677480863,3.93233836508166,133.761507282408));
#208805=CARTESIAN_POINT('Ctrl Pts',(202.90693120479,4.01334126447339,133.650604242471));
#208806=CARTESIAN_POINT('Ctrl Pts',(202.899184928717,4.08956560638427,133.536509261688));
#208807=CARTESIAN_POINT('Ctrl Pts',(202.891438595462,4.16579051096613,133.422413438681));
#208808=CARTESIAN_POINT('Ctrl Pts',(202.883692262207,4.23723657049395,133.305125952902));
#208809=CARTESIAN_POINT('Ctrl Pts',(202.875945928953,4.30363925381155,133.185089967062));
#208810=CARTESIAN_POINT('Ctrl Pts',(202.868197860961,4.37005680754998,133.065027099995));
#208811=CARTESIAN_POINT('Ctrl Pts',(202.860449792968,4.43142854843043,132.942214850122));
#208812=CARTESIAN_POINT('Ctrl Pts',(202.852701724976,4.48753611850486,132.817120575339));
#208813=CARTESIAN_POINT('Ctrl Pts',(202.844945422245,4.54370332037339,132.69189334887));
#208814=CARTESIAN_POINT('Ctrl Pts',(202.837189119514,4.59459501491842,132.564379609861));
#208815=CARTESIAN_POINT('Ctrl Pts',(202.829432816783,4.64004099484783,132.435066792397));
#208816=CARTESIAN_POINT('Ctrl Pts',(202.821672374279,4.68551123066541,132.305684956788));
#208817=CARTESIAN_POINT('Ctrl Pts',(202.813911931776,4.72552984631434,132.174502503168));
#208818=CARTESIAN_POINT('Ctrl Pts',(202.806151489272,4.75997697153195,132.04202062459));
#208819=CARTESIAN_POINT('Ctrl Pts',(202.798378589017,4.79447939433392,131.909326074335));
#208820=CARTESIAN_POINT('Ctrl Pts',(202.790605688762,4.82339237153089,131.775328313116));
#208821=CARTESIAN_POINT('Ctrl Pts',(202.782832788507,4.84664731046149,131.640538176758));
#208822=CARTESIAN_POINT('Ctrl Pts',(202.775342452627,4.86905687417027,131.510647999147));
#208823=CARTESIAN_POINT('Ctrl Pts',(202.767852116746,4.8862125852588,131.380022361244));
#208824=CARTESIAN_POINT('Ctrl Pts',(202.760361780866,4.89809886429187,131.249119628855));
#208825=CARTESIAN_POINT('Ctrl Pts',(202.752587446755,4.91043581499945,131.113253681868));
#208826=CARTESIAN_POINT('Ctrl Pts',(202.744813112644,4.91713494470752,130.976658831053));
#208827=CARTESIAN_POINT('Ctrl Pts',(202.737038778533,4.91812200914719,130.839842523405));
#208828=CARTESIAN_POINT('Ctrl Pts',(202.729274025594,4.91910785711814,130.703194829631));
#208829=CARTESIAN_POINT('Ctrl Pts',(202.721509272656,4.91439564375304,130.566326609267));
#208830=CARTESIAN_POINT('Ctrl Pts',(202.713744519717,4.90396277453586,130.429751263082));
#208831=CARTESIAN_POINT('Ctrl Pts',(202.70598747884,4.89354026739166,130.293311565459));
#208832=CARTESIAN_POINT('Ctrl Pts',(202.698230437964,4.87740844109174,130.157164550445));
#208833=CARTESIAN_POINT('Ctrl Pts',(202.690473397087,4.8555967358373,130.021824099935));
#208834=CARTESIAN_POINT('Ctrl Pts',(202.682722205856,4.83380147895985,129.886585710714));
#208835=CARTESIAN_POINT('Ctrl Pts',(202.674971014624,4.80633493061361,129.752153059763));
#208836=CARTESIAN_POINT('Ctrl Pts',(202.667219823393,4.77327836053893,129.619035027143));
#208837=CARTESIAN_POINT('Ctrl Pts',(202.659471926624,4.74023584038906,129.485973573241));
#208838=CARTESIAN_POINT('Ctrl Pts',(202.651724029856,4.70160811803909,129.35422600501));
#208839=CARTESIAN_POINT('Ctrl Pts',(202.643976133088,4.6575275379995,129.224290905409));
#208840=CARTESIAN_POINT('Ctrl Pts',(202.636229857012,4.61345617866757,129.094382985432));
#208841=CARTESIAN_POINT('Ctrl Pts',(202.628483580937,4.56393435592693,128.966287149981));
#208842=CARTESIAN_POINT('Ctrl Pts',(202.620737304862,4.50914413590637,128.840486328279));
#208843=CARTESIAN_POINT('Ctrl Pts',(202.612990971605,4.45435351143753,128.714684577946));
#208844=CARTESIAN_POINT('Ctrl Pts',(202.605244638349,4.39429456820026,128.591178233612));
#208845=CARTESIAN_POINT('Ctrl Pts',(202.597498305092,4.3291971659843,128.470429393101));
#208846=CARTESIAN_POINT('Ctrl Pts',(202.589750237099,4.26408518565718,128.349653511726));
#208847=CARTESIAN_POINT('Ctrl Pts',(202.582002169105,4.19393268660458,128.231636707049));
#208848=CARTESIAN_POINT('Ctrl Pts',(202.574254101111,4.11901484245543,128.116815308156));
#208849=CARTESIAN_POINT('Ctrl Pts',(202.566497798378,4.04401737473066,128.001871875715));
#208850=CARTESIAN_POINT('Ctrl Pts',(202.558741495645,3.9642446586756,127.890130961117));
#208851=CARTESIAN_POINT('Ctrl Pts',(202.550985192912,3.88001478519079,127.781999234607));
#208852=CARTESIAN_POINT('Ctrl Pts',(202.543224750407,3.79573995568691,127.67380979494));
#208853=CARTESIAN_POINT('Ctrl Pts',(202.535464307902,3.70700348138614,127.569233679702));
#208854=CARTESIAN_POINT('Ctrl Pts',(202.527703865397,3.61416223739328,127.468642646229));
#208855=CARTESIAN_POINT('Ctrl Pts',(202.519930965141,3.52117195639349,127.367890135099));
#208856=CARTESIAN_POINT('Ctrl Pts',(202.512158064885,3.42406401521649,127.2711357655));
#208857=CARTESIAN_POINT('Ctrl Pts',(202.504385164629,3.32323111850202,127.178713365623));
#208858=CARTESIAN_POINT('Ctrl Pts',(202.49689482877,3.22606375019959,127.089650751528));
#208859=CARTESIAN_POINT('Ctrl Pts',(202.489404492912,3.12543778266822,127.004610818164));
#208860=CARTESIAN_POINT('Ctrl Pts',(202.481914157053,3.02173043097238,126.923854430864));
#208861=CARTESIAN_POINT('Ctrl Pts',(202.474139822926,2.91409098479571,126.84003614159));
#208862=CARTESIAN_POINT('Ctrl Pts',(202.466365488799,2.80279091121412,126.760567120498));
#208863=CARTESIAN_POINT('Ctrl Pts',(202.458591154673,2.68821700891863,126.685784118888));
#208864=CARTESIAN_POINT('Ctrl Pts',(202.450826401718,2.57378430871652,126.611093280644));
#208865=CARTESIAN_POINT('Ctrl Pts',(202.443061648763,2.45608613190742,126.541077182797));
#208866=CARTESIAN_POINT('Ctrl Pts',(202.435296895808,2.33554220421387,126.476032340409));
#208867=CARTESIAN_POINT('Ctrl Pts',(202.427539854915,2.21511800244725,126.411052101475));
#208868=CARTESIAN_POINT('Ctrl Pts',(202.419782814022,2.09185401638329,126.351033476568));
#208869=CARTESIAN_POINT('Ctrl Pts',(202.412025773129,1.96619850256614,126.29622946253));
#208870=CARTESIAN_POINT('Ctrl Pts',(202.404274581881,1.8406377465481,126.241466776625));
#208871=CARTESIAN_POINT('Ctrl Pts',(202.396523390633,1.71268940938756,126.191911030093));
#208872=CARTESIAN_POINT('Ctrl Pts',(202.388772199385,1.58282555457417,126.147768910503));
#208873=CARTESIAN_POINT('Ctrl Pts',(202.3810243026,1.45301689536158,126.103645552491));
#208874=CARTESIAN_POINT('Ctrl Pts',(202.373276405815,1.3212947071609,126.064931370595));
#208875=CARTESIAN_POINT('Ctrl Pts',(202.36552850903,1.18814999737997,126.031784515897));
#208876=CARTESIAN_POINT('Ctrl Pts',(202.357782232937,1.05503313860108,125.998644594806));
#208877=CARTESIAN_POINT('Ctrl Pts',(202.350035956845,0.92049472925159,125.97106977892));
#208878=CARTESIAN_POINT('Ctrl Pts',(202.342289680753,0.785039482555496,
125.949167925887));
#208879=CARTESIAN_POINT('Ctrl Pts',(202.33454334748,0.649583235958816,125.927265911181));
#208880=CARTESIAN_POINT('Ctrl Pts',(202.326797014206,0.513210524463309,
125.911037005295));
#208881=CARTESIAN_POINT('Ctrl Pts',(202.319050680933,0.376434368889621,
125.900537595839));
#208882=CARTESIAN_POINT('Ctrl Pts',(202.311302612921,0.239627583243728,
125.890035835114));
#208883=CARTESIAN_POINT('Ctrl Pts',(202.30355454491,0.102417563480344,125.885266153919));
#208884=CARTESIAN_POINT('Ctrl Pts',(202.295806476899,-0.0346798563142518,
125.886232887416));
#208885=CARTESIAN_POINT('Ctrl Pts',(202.288050174149,-0.17192298487841,
125.887200648369));
#208886=CARTESIAN_POINT('Ctrl Pts',(202.280293871399,-0.309052882836018,
125.893917000127));
#208887=CARTESIAN_POINT('Ctrl Pts',(202.272537568649,-0.445555471089543,
125.906334139005));
#208888=CARTESIAN_POINT('Ctrl Pts',(202.264777126127,-0.58213091488482,
125.918757905285));
#208889=CARTESIAN_POINT('Ctrl Pts',(202.257016683604,-0.718077994486212,
125.936888469828));
#208890=CARTESIAN_POINT('Ctrl Pts',(202.249256241082,-0.852891040206172,
125.960626527421));
#208891=CARTESIAN_POINT('Ctrl Pts',(202.241483340808,-0.987920499794184,
125.984402691451));
#208892=CARTESIAN_POINT('Ctrl Pts',(202.233710440535,-1.12181190557149,
126.013804252784));
#208893=CARTESIAN_POINT('Ctrl Pts',(202.225937540261,-1.25407213197427,
126.048681260176));
#208894=CARTESIAN_POINT('Ctrl Pts',(202.218447204587,-1.38152436436558,
126.082290400067));
#208895=CARTESIAN_POINT('Ctrl Pts',(202.210956868914,-1.50746165896199,
126.120983714381));
#208896=CARTESIAN_POINT('Ctrl Pts',(202.20346653324,-1.63146064844767,126.164584845498));
#208897=CARTESIAN_POINT('Ctrl Pts',(202.195692103635,-1.76016267956143,
126.209839683114));
#208898=CARTESIAN_POINT('Ctrl Pts',(202.187917674029,-1.88718416540828,
126.260525329425));
#208899=CARTESIAN_POINT('Ctrl Pts',(202.180143244423,-2.01203269537097,
126.316498376447));
#208900=CARTESIAN_POINT('Ctrl Pts',(202.172378418318,-2.1367270040091,126.372402281787));
#208901=CARTESIAN_POINT('Ctrl Pts',(202.164613592212,-2.2592533441934,126.433580433836));
#208902=CARTESIAN_POINT('Ctrl Pts',(202.156848766106,-2.37913536422814,
126.499839972804));
#208903=CARTESIAN_POINT('Ctrl Pts',(202.149091674296,-2.49889797360211,
126.566033512757));
#208904=CARTESIAN_POINT('Ctrl Pts',(202.141334582486,-2.61602116454483,
126.637298179153));
#208905=CARTESIAN_POINT('Ctrl Pts',(202.133577490676,-2.73004978163739,
126.713393586132));
#208906=CARTESIAN_POINT('Ctrl Pts',(202.125826270674,-2.84399208364077,
126.78943139194));
#208907=CARTESIAN_POINT('Ctrl Pts',(202.118075050671,-2.95484415052419,
126.870292443658));
#208908=CARTESIAN_POINT('Ctrl Pts',(202.110323830669,-3.06217692439492,
126.955691296073));
#208909=CARTESIAN_POINT('Ctrl Pts',(202.102576019855,-3.16946249051467,
127.041052587846));
#208910=CARTESIAN_POINT('Ctrl Pts',(202.094828209041,-3.27323153754679,
127.130947467042));
#208911=CARTESIAN_POINT('Ctrl Pts',(202.087080398227,-3.37308562112851,
127.225048329565));
#208912=CARTESIAN_POINT('Ctrl Pts',(202.079334239672,-3.47291841033375,
127.319129124614));
#208913=CARTESIAN_POINT('Ctrl Pts',(202.071588081117,-3.568837612584,127.417413850761));
#208914=CARTESIAN_POINT('Ctrl Pts',(202.063841922562,-3.66047969139515,
127.519536194346));
#208915=CARTESIAN_POINT('Ctrl Pts',(202.056095738413,-3.75212207299657,
127.621658875349));
#208916=CARTESIAN_POINT('Ctrl Pts',(202.048349554264,-3.83948704196994,
127.727618908041));
#208917=CARTESIAN_POINT('Ctrl Pts',(202.040603370115,-3.92224987613099,
127.837015175645));
#208918=CARTESIAN_POINT('Ctrl Pts',(202.032855482865,-4.0050309067957,127.946435495465));
#208919=CARTESIAN_POINT('Ctrl Pts',(202.025107595616,-4.08320755361812,
128.059293241692));
#208920=CARTESIAN_POINT('Ctrl Pts',(202.017359708366,-4.1564973670384,128.175156802663));
#208921=CARTESIAN_POINT('Ctrl Pts',(202.00960402534,-4.22986092326722,128.291136943332));
#208922=CARTESIAN_POINT('Ctrl Pts',(202.001848342314,-4.29832761616902,
128.410128608468));
#208923=CARTESIAN_POINT('Ctrl Pts',(201.994092659288,-4.36165984536912,
128.531673561283));
#208924=CARTESIAN_POINT('Ctrl Pts',(201.986332849536,-4.42502577306113,
128.653283187041));
#208925=CARTESIAN_POINT('Ctrl Pts',(201.978573039783,-4.48325162754233,
128.777448453866));
#208926=CARTESIAN_POINT('Ctrl Pts',(201.97081323003,-4.5361476689452,128.903690370516));
#208927=CARTESIAN_POINT('Ctrl Pts',(201.9630419948,-4.58912159402284,129.030118164673));
#208928=CARTESIAN_POINT('Ctrl Pts',(201.955270759571,-4.63674989270561,
129.158628350682));
#208929=CARTESIAN_POINT('Ctrl Pts',(201.947499524341,-4.67889225145815,
129.28872531785));
#208930=CARTESIAN_POINT('Ctrl Pts',(201.941698877603,-4.71034837504711,
129.385832988111));
#208931=CARTESIAN_POINT('Ctrl Pts',(201.935898230865,-4.73874903929908,
129.483824402015));
#208932=CARTESIAN_POINT('Ctrl Pts',(201.930097584127,-4.76405452823404,
129.582490119308));
#208933=CARTESIAN_POINT('Ctrl Pts',(203.680274487341,-4.76405452823405,
129.582490119308));
#208934=CARTESIAN_POINT('Ctrl Pts',(203.672576598541,-4.7978764752882,129.714361377553));
#208935=CARTESIAN_POINT('Ctrl Pts',(203.664878709741,-4.82619293906168,
129.847536976704));
#208936=CARTESIAN_POINT('Ctrl Pts',(203.65718082094,-4.84892836211919,129.981513850825));
#208937=CARTESIAN_POINT('Ctrl Pts',(203.649340778128,-4.87208363166798,
130.1179648254));
#208938=CARTESIAN_POINT('Ctrl Pts',(203.641500735315,-4.88944965601479,
130.255246526921));
#208939=CARTESIAN_POINT('Ctrl Pts',(203.633660692502,-4.90100205051574,
130.392824515455));
#208940=CARTESIAN_POINT('Ctrl Pts',(203.62582064969,-4.9125544450167,130.530402503989));
#208941=CARTESIAN_POINT('Ctrl Pts',(203.617980606877,-4.91829325611943,
130.668276348449));
#208942=CARTESIAN_POINT('Ctrl Pts',(203.610140564065,-4.91824975435206,
130.805915067923));
#208943=CARTESIAN_POINT('Origin',(213.235140564004,0.,130.804360617566));
#208944=CARTESIAN_POINT('',(205.430026442963,-4.76405452823405,129.582490119308));
#208945=CARTESIAN_POINT('',(205.084976592678,-4.76405452823405,129.582490119308));
#208946=CARTESIAN_POINT('',(213.235140564004,-4.76405452823405,129.582490119308));
#208947=CARTESIAN_POINT('',(205.014859436024,-4.91824993440617,130.805163869501));
#208948=CARTESIAN_POINT('Ctrl Pts',(205.084976592678,-4.76405452823405,
129.582490119308));
#208949=CARTESIAN_POINT('Ctrl Pts',(205.077250789112,-4.79798664166829,
129.714790914597));
#208950=CARTESIAN_POINT('Ctrl Pts',(205.069524985546,-4.82637681902747,
129.848402380795));
#208951=CARTESIAN_POINT('Ctrl Pts',(205.06179918198,-4.84914957344003,129.982818484193));
#208952=CARTESIAN_POINT('Ctrl Pts',(205.053975890988,-4.87220968401055,
130.118930706311));
#208953=CARTESIAN_POINT('Ctrl Pts',(205.046152599995,-4.88950959216643,
130.255867593678));
#208954=CARTESIAN_POINT('Ctrl Pts',(205.038329309002,-4.90102524937068,
130.393100885121));
#208955=CARTESIAN_POINT('Ctrl Pts',(205.030506018009,-4.91254090657492,
130.530334176563));
#208956=CARTESIAN_POINT('Ctrl Pts',(205.022682727017,-4.9182723584033,130.667863456436));
#208957=CARTESIAN_POINT('Ctrl Pts',(205.014859436024,-4.91824993440617,
130.805163869501));
#208958=CARTESIAN_POINT('Ctrl Pts',(205.014859435991,-4.91824993440608,
130.80516387008));
#208959=CARTESIAN_POINT('Ctrl Pts',(205.012416879836,-4.91824293327168,
130.848031247661));
#208960=CARTESIAN_POINT('Ctrl Pts',(205.009974323682,-4.91767549764493,
130.890893474637));
#208961=CARTESIAN_POINT('Ctrl Pts',(205.007531767528,-4.91654795620673,
130.933740897437));
#208962=CARTESIAN_POINT('Ctrl Pts',(204.999757433917,-4.91295914074164,
131.070118584653));
#208963=CARTESIAN_POINT('Ctrl Pts',(204.991983100306,-4.9036859709115,131.206562848942));
#208964=CARTESIAN_POINT('Ctrl Pts',(204.984208766695,-4.88871387579036,
131.342561047847));
#208965=CARTESIAN_POINT('Ctrl Pts',(204.976444014264,-4.87376023245488,
131.478391640977));
#208966=CARTESIAN_POINT('Ctrl Pts',(204.968679261833,-4.85312168071783,
131.613776877648));
#208967=CARTESIAN_POINT('Ctrl Pts',(204.960914509402,-4.82683564131106,
131.748204224457));
#208968=CARTESIAN_POINT('Ctrl Pts',(204.95315746904,-4.80057570959591,131.882498055994));
#208969=CARTESIAN_POINT('Ctrl Pts',(204.945400428679,-4.76867952725585,
132.015835509765));
#208970=CARTESIAN_POINT('Ctrl Pts',(204.937643388317,-4.73123625092355,
132.147709641627));
#208971=CARTESIAN_POINT('Ctrl Pts',(204.929892197607,-4.69382121089179,
132.27948432606));
#208972=CARTESIAN_POINT('Ctrl Pts',(204.922141006897,-4.65086750945265,
132.409797510464));
#208973=CARTESIAN_POINT('Ctrl Pts',(204.914389816187,-4.60251519606229,
132.538153261603));
#208974=CARTESIAN_POINT('Ctrl Pts',(204.906641919949,-4.55418343374924,
132.666454457979));
#208975=CARTESIAN_POINT('Ctrl Pts',(204.898894023711,-4.50045776072558,
132.792799510701));
#208976=CARTESIAN_POINT('Ctrl Pts',(204.891146127472,-4.44152775223612,
132.916708668579));
#208977=CARTESIAN_POINT('Ctrl Pts',(204.883399851932,-4.38261007067356,
133.040591907248));
#208978=CARTESIAN_POINT('Ctrl Pts',(204.875653576392,-4.31849038681639,
133.162039911728));
#208979=CARTESIAN_POINT('Ctrl Pts',(204.867907300851,-4.2494058332061,133.280594275203));
#208980=CARTESIAN_POINT('Ctrl Pts',(204.860160968134,-4.18032076967024,
133.399149513749));
#208981=CARTESIAN_POINT('Ctrl Pts',(204.852414635417,-4.10627096009826,
133.514810730874));
#208982=CARTESIAN_POINT('Ctrl Pts',(204.8446683027,-4.02753857581953,133.627145781688));
#208983=CARTESIAN_POINT('Ctrl Pts',(204.83692023525,-3.94878856000942,133.7395059891));
#208984=CARTESIAN_POINT('Ctrl Pts',(204.829172167799,-3.86535410719281,
133.848538227898));
#208985=CARTESIAN_POINT('Ctrl Pts',(204.821424100349,-3.77755938889782,
133.953841229643));
#208986=CARTESIAN_POINT('Ctrl Pts',(204.813667798163,-3.68967136136312,
134.059256148634));
#208987=CARTESIAN_POINT('Ctrl Pts',(204.805911495977,-3.5974140619154,134.160933612335));
#208988=CARTESIAN_POINT('Ctrl Pts',(204.798155193791,-3.50115082848458,
134.258506812894));
#208989=CARTESIAN_POINT('Ctrl Pts',(204.790394751835,-3.40483621649768,
134.356132091179));
#208990=CARTESIAN_POINT('Ctrl Pts',(204.782634309879,-3.30451169605726,
134.449648474981));
#208991=CARTESIAN_POINT('Ctrl Pts',(204.774873867924,-3.20057505400699,
134.538728353364));
#208992=CARTESIAN_POINT('Ctrl Pts',(204.767100968216,-3.09647156360682,
134.627951230698));
#208993=CARTESIAN_POINT('Ctrl Pts',(204.759328068508,-2.98874467176853,
134.712723128926));
#208994=CARTESIAN_POINT('Ctrl Pts',(204.7515551688,-2.87782332804817,134.792758285182));
#208995=CARTESIAN_POINT('Ctrl Pts',(204.744064827105,-2.77093416223283,
134.869884028534));
#208996=CARTESIAN_POINT('Ctrl Pts',(204.73657448541,-2.66107901674024,134.942611258251));
#208997=CARTESIAN_POINT('Ctrl Pts',(204.729084143715,-2.54866295096712,
135.010724870085));
#208998=CARTESIAN_POINT('Ctrl Pts',(204.721309809264,-2.43198468332284,
135.08142097724));
#208999=CARTESIAN_POINT('Ctrl Pts',(204.713535474812,-2.31217786981156,
135.147370661178));
#209000=CARTESIAN_POINT('Ctrl Pts',(204.70576114036,-2.18966593526101,135.208284567234));
#209001=CARTESIAN_POINT('Ctrl Pts',(204.697996387077,-2.0673049856553,135.269123402377));
#209002=CARTESIAN_POINT('Ctrl Pts',(204.690231633794,-1.94224589503469,
135.324938635623));
#209003=CARTESIAN_POINT('Ctrl Pts',(204.682466880511,-1.8149400992257,135.375484713313));
#209004=CARTESIAN_POINT('Ctrl Pts',(204.674709839286,-1.68776074526766,
135.425980587951));
#209005=CARTESIAN_POINT('Ctrl Pts',(204.666952798062,-1.55833948784361,
135.471217578389));
#209006=CARTESIAN_POINT('Ctrl Pts',(204.659195756837,-1.42715102488418,
135.510996678987));
#209007=CARTESIAN_POINT('Ctrl Pts',(204.651444565255,-1.29606149211033,
135.550745781873));
#209008=CARTESIAN_POINT('Ctrl Pts',(204.643693373672,-1.16320777901492,
135.585045074249));
#209009=CARTESIAN_POINT('Ctrl Pts',(204.635942182089,-1.02908282854748,
135.613744319714));
#209010=CARTESIAN_POINT('Ctrl Pts',(204.628194284967,-0.895014884701764,
135.642431367248));
#209011=CARTESIAN_POINT('Ctrl Pts',(204.620446387844,-0.759677159628549,
135.665523020208));
#209012=CARTESIAN_POINT('Ctrl Pts',(204.612698490721,-0.623575751751765,
135.682919456437));
#209013=CARTESIAN_POINT('Ctrl Pts',(204.604952214289,-0.487502813319543,
135.700312253712));
#209014=CARTESIAN_POINT('Ctrl Pts',(204.597205937857,-0.350666897391173,
135.712012154308));
#209015=CARTESIAN_POINT('Ctrl Pts',(204.589459661425,-0.213581850635355,
135.717970884526));
#209016=CARTESIAN_POINT('Ctrl Pts',(204.58171332781,-0.0764957919198511,
135.723929658732));
#209017=CARTESIAN_POINT('Ctrl Pts',(204.573966994196,0.0608390106965075,
135.724147161014));
#209018=CARTESIAN_POINT('Ctrl Pts',(204.566220660581,0.197906460888714,
135.718627205292));
#209019=CARTESIAN_POINT('Ctrl Pts',(204.558472592227,0.335004606408075,
135.713106013413));
#209020=CARTESIAN_POINT('Ctrl Pts',(204.550724523873,0.471834889791658,
135.701844822528));
#209021=CARTESIAN_POINT('Ctrl Pts',(204.54297645552,0.607884489820787,135.684899471989));
#209022=CARTESIAN_POINT('Ctrl Pts',(204.535220152427,0.744078684979407,
135.667936111731));
#209023=CARTESIAN_POINT('Ctrl Pts',(204.527463849334,0.879490150743396,
135.645276572288));
#209024=CARTESIAN_POINT('Ctrl Pts',(204.519707546241,1.01361388816882,135.617028271603));
#209025=CARTESIAN_POINT('Ctrl Pts',(204.511947103376,1.14780921147885,135.588764893948));
#209026=CARTESIAN_POINT('Ctrl Pts',(204.50418666051,1.28071505826876,135.554906907859));
#209027=CARTESIAN_POINT('Ctrl Pts',(204.496426217644,1.41184078659271,135.515611901016));
#209028=CARTESIAN_POINT('Ctrl Pts',(204.48865331703,1.54317700952478,135.476253814356));
#209029=CARTESIAN_POINT('Ctrl Pts',(204.480880416416,1.67272703389122,135.431441393526));
#209030=CARTESIAN_POINT('Ctrl Pts',(204.473107515801,1.80001858150718,135.381381064181));
#209031=CARTESIAN_POINT('Ctrl Pts',(204.465617183835,1.9226826930735,135.333140580513));
#209032=CARTESIAN_POINT('Ctrl Pts',(204.458126851868,2.04324940016541,135.280027243014));
#209033=CARTESIAN_POINT('Ctrl Pts',(204.450636519902,2.16131878660124,135.222265569598));
#209034=CARTESIAN_POINT('Ctrl Pts',(204.442862185831,2.28386487105517,135.162313814766));
#209035=CARTESIAN_POINT('Ctrl Pts',(204.435087851759,2.40410871112534,135.097164368467));
#209036=CARTESIAN_POINT('Ctrl Pts',(204.427313517688,2.52157799309945,135.027017066677));
#209037=CARTESIAN_POINT('Ctrl Pts',(204.419548764789,2.63890250468257,134.956956215167));
#209038=CARTESIAN_POINT('Ctrl Pts',(204.411784011889,2.75345892929808,134.881909962079));
#209039=CARTESIAN_POINT('Ctrl Pts',(204.40401925899,2.86479666362884,134.802125385353));
#209040=CARTESIAN_POINT('Ctrl Pts',(204.396262218153,2.9760238157537,134.722420051793));
#209041=CARTESIAN_POINT('Ctrl Pts',(204.388505177315,3.08403832372975,134.637985986342));
#209042=CARTESIAN_POINT('Ctrl Pts',(204.380748136478,3.18841617266462,134.549114998349));
#209043=CARTESIAN_POINT('Ctrl Pts',(204.372996945285,3.29271530945384,134.460311028657));
#209044=CARTESIAN_POINT('Ctrl Pts',(204.365245754092,3.39338294937173,134.3670770487));
#209045=CARTESIAN_POINT('Ctrl Pts',(204.357494562899,3.49002624658722,134.269746578845));
#209046=CARTESIAN_POINT('Ctrl Pts',(204.349746666169,3.58662846782897,134.172457477031));
#209047=CARTESIAN_POINT('Ctrl Pts',(204.341998769439,3.67920947343216,134.07107562512));
#209048=CARTESIAN_POINT('Ctrl Pts',(204.334250872709,3.76741172163867,133.965972861684));
#209049=CARTESIAN_POINT('Ctrl Pts',(204.326504596671,3.85559551983956,133.860892083477));
#209050=CARTESIAN_POINT('Ctrl Pts',(204.318758320634,3.9394021313356,133.752092241188));
#209051=CARTESIAN_POINT('Ctrl Pts',(204.311012044596,4.01851319542896,133.639979555411));
#209052=CARTESIAN_POINT('Ctrl Pts',(204.303265711377,4.09762484350567,133.527866042038));
#209053=CARTESIAN_POINT('Ctrl Pts',(204.295519378158,4.17204064960371,133.412439955821));
#209054=CARTESIAN_POINT('Ctrl Pts',(204.287773044939,4.24148485981986,133.294137564688));
#209055=CARTESIAN_POINT('Ctrl Pts',(204.280024976982,4.31094462158894,133.175808680548));
#209056=CARTESIAN_POINT('Ctrl Pts',(204.272276909025,4.37543037414788,133.054602546852));
#209057=CARTESIAN_POINT('Ctrl Pts',(204.264528841068,4.43471190433788,132.930980797105));
#209058=CARTESIAN_POINT('Ctrl Pts',(204.256772538371,4.49405643965077,132.807227660677));
#209059=CARTESIAN_POINT('Ctrl Pts',(204.249016235674,4.54818553428607,132.681054132738));
#209060=CARTESIAN_POINT('Ctrl Pts',(204.241259932977,4.59691659774419,132.552943145182));
#209061=CARTESIAN_POINT('Ctrl Pts',(204.233499490508,4.64567367044088,132.424763780927));
#209062=CARTESIAN_POINT('Ctrl Pts',(204.225739048038,4.68902684761736,132.2946452673));
#209063=CARTESIAN_POINT('Ctrl Pts',(204.217978605568,4.72684350830149,132.163085575211));
#209064=CARTESIAN_POINT('Ctrl Pts',(204.210205705346,4.76472087565255,132.031314691805));
#209065=CARTESIAN_POINT('Ctrl Pts',(204.202432805124,4.79704387379708,131.898098386972));
#209066=CARTESIAN_POINT('Ctrl Pts',(204.194659904902,4.82373089659542,131.763945579792));
#209067=CARTESIAN_POINT('Ctrl Pts',(204.187169568631,4.849447780786,131.634669555555));
#209068=CARTESIAN_POINT('Ctrl Pts',(204.17967923236,4.86993129066992,131.504524239439));
#209069=CARTESIAN_POINT('Ctrl Pts',(204.172188896089,4.88515415502804,131.373967450489));
#209070=CARTESIAN_POINT('Ctrl Pts',(204.164414562036,4.90095419770749,131.238460571561));
#209071=CARTESIAN_POINT('Ctrl Pts',(204.156640227983,4.91113685606931,131.102081156815));
#209072=CARTESIAN_POINT('Ctrl Pts',(204.14886589393,4.915614960675,130.965334593376));
#209073=CARTESIAN_POINT('Ctrl Pts',(204.141101141049,4.9200875464163,130.828756557876));
#209074=CARTESIAN_POINT('Ctrl Pts',(204.133336388169,4.91886955403614,130.691812660983));
#209075=CARTESIAN_POINT('Ctrl Pts',(204.125571635289,4.9119252950968,130.555015559688));
#209076=CARTESIAN_POINT('Ctrl Pts',(204.117814594472,4.90498793329431,130.418354327222));
#209077=CARTESIAN_POINT('Ctrl Pts',(204.110057553655,4.892335642827,130.281839988143));
#209078=CARTESIAN_POINT('Ctrl Pts',(204.102300512838,4.87398474075138,130.145987008266));
#209079=CARTESIAN_POINT('Ctrl Pts',(204.094549321667,4.85564767723613,130.010236476196));
#209080=CARTESIAN_POINT('Ctrl Pts',(204.086798130496,4.83162060788727,129.875146696503));
#209081=CARTESIAN_POINT('Ctrl Pts',(204.079046939325,4.80197179006196,129.741228457414));
#209082=CARTESIAN_POINT('Ctrl Pts',(204.071299042618,4.77233557377983,129.607367137171));
#209083=CARTESIAN_POINT('Ctrl Pts',(204.063551145911,4.73708244567803,129.474676748098));
#209084=CARTESIAN_POINT('Ctrl Pts',(204.055803249204,4.69633198401899,129.343659088033));
#209085=CARTESIAN_POINT('Ctrl Pts',(204.048056973191,4.65559004648194,129.21266883405));
#209086=CARTESIAN_POINT('Ctrl Pts',(204.040310697177,4.60935317869152,129.083350986195));
#209087=CARTESIAN_POINT('Ctrl Pts',(204.032564421164,4.55779106379823,128.956192962492));
#209088=CARTESIAN_POINT('Ctrl Pts',(204.02481808797,4.50622856828952,128.829034000148));
#209089=CARTESIAN_POINT('Ctrl Pts',(204.017071754777,4.44934089415499,128.704035256081));
#209090=CARTESIAN_POINT('Ctrl Pts',(204.009325421583,4.3873460342304,128.58166454333));
#209091=CARTESIAN_POINT('Ctrl Pts',(204.001577353652,4.3253372909914,128.459266426516));
#209092=CARTESIAN_POINT('Ctrl Pts',(203.993829285721,4.25821926274942,128.339497860818));
#209093=CARTESIAN_POINT('Ctrl Pts',(203.98608121779,4.18625589900541,128.222802055274));
#209094=CARTESIAN_POINT('Ctrl Pts',(203.978324915121,4.1142160517463,128.105982224046));
#209095=CARTESIAN_POINT('Ctrl Pts',(203.970568612452,4.03732078748716,127.992242009999));
#209096=CARTESIAN_POINT('Ctrl Pts',(203.962812309783,3.95587771587694,127.881996068177));
#209097=CARTESIAN_POINT('Ctrl Pts',(203.955051867342,3.87439117565101,127.771691284781));
#209098=CARTESIAN_POINT('Ctrl Pts',(203.9472914249,3.78835223661492,127.664884794093));
#209099=CARTESIAN_POINT('Ctrl Pts',(203.939530982459,3.6981081709207,127.561957339337));
#209100=CARTESIAN_POINT('Ctrl Pts',(203.931758082267,3.60771923743896,127.458864656291));
#209101=CARTESIAN_POINT('Ctrl Pts',(203.923985182075,3.51311195774471,127.359663735743));
#209102=CARTESIAN_POINT('Ctrl Pts',(203.916212281882,3.41467038975604,127.264698318444));
#209103=CARTESIAN_POINT('Ctrl Pts',(203.908721945347,3.3198074100404,127.173185122963));
#209104=CARTESIAN_POINT('Ctrl Pts',(203.901231608812,3.22138430351891,127.085605040283));
#209105=CARTESIAN_POINT('Ctrl Pts',(203.893741272277,3.11977150560056,127.002228476866));
#209106=CARTESIAN_POINT('Ctrl Pts',(203.885966938106,3.01430603775704,126.915690674068));
#209107=CARTESIAN_POINT('Ctrl Pts',(203.878192603936,2.90507014731187,126.83340730906));
#209108=CARTESIAN_POINT('Ctrl Pts',(203.870418269766,2.79244191357776,126.755724894042));
#209109=CARTESIAN_POINT('Ctrl Pts',(203.862653516767,2.67995248406615,126.678138215651));
#209110=CARTESIAN_POINT('Ctrl Pts',(203.854888763768,2.56407934847872,126.605141424973));
#209111=CARTESIAN_POINT('Ctrl Pts',(203.84712401077,2.44523452920922,126.537041651322));
#209112=CARTESIAN_POINT('Ctrl Pts',(203.839366969832,2.32650774828062,126.469009515322));
#209113=CARTESIAN_POINT('Ctrl Pts',(203.831609928895,2.20481549434958,126.405864910317));
#209114=CARTESIAN_POINT('Ctrl Pts',(203.823852887958,2.08059942186419,126.34787218964));
#209115=CARTESIAN_POINT('Ctrl Pts',(203.816101696665,1.95647702167689,126.289923201721));
#209116=CARTESIAN_POINT('Ctrl Pts',(203.808350505372,1.82983494402628,126.237118529847));
#209117=CARTESIAN_POINT('Ctrl Pts',(203.800599314079,1.70113982430083,126.189676840678));
#209118=CARTESIAN_POINT('Ctrl Pts',(203.792851417249,1.57249940342463,126.142255315488));
#209119=CARTESIAN_POINT('Ctrl Pts',(203.785103520418,1.44180804206936,126.100192374375));
#209120=CARTESIAN_POINT('Ctrl Pts',(203.777355623588,1.30955255195562,126.063658646743));
#209121=CARTESIAN_POINT('Ctrl Pts',(203.76960934745,1.17732472683343,126.027132561177));
#209122=CARTESIAN_POINT('Ctrl Pts',(203.761863071312,1.04353380034826,125.996133492601));
#209123=CARTESIAN_POINT('Ctrl Pts',(203.754116795175,0.908681568991501,
125.970782143115));
#209124=CARTESIAN_POINT('Ctrl Pts',(203.746370461855,0.77382834218146,125.945430606491));
#209125=CARTESIAN_POINT('Ctrl Pts',(203.738624128536,0.637914179101389,
125.925726944381));
#209126=CARTESIAN_POINT('Ctrl Pts',(203.730877795217,0.501450494577304,
125.911740617608));
#209127=CARTESIAN_POINT('Ctrl Pts',(203.72312972716,0.364956249953434,125.897751158694));
#209128=CARTESIAN_POINT('Ctrl Pts',(203.715381659102,0.227912627860709,
125.889481622733));
#209129=CARTESIAN_POINT('Ctrl Pts',(203.707633591045,0.0908351837803655,
125.88694950684));
#209130=CARTESIAN_POINT('Ctrl Pts',(203.699877288249,-0.0463879478389493,
125.884414699785));
#209131=CARTESIAN_POINT('Ctrl Pts',(203.692120985453,-0.183644581730893,
125.887629501038));
#209132=CARTESIAN_POINT('Ctrl Pts',(203.684364682657,-0.320419586321026,
125.896559241063));
#209133=CARTESIAN_POINT('Ctrl Pts',(203.676604240088,-0.457267591850978,
125.90549374716));
#209134=CARTESIAN_POINT('Ctrl Pts',(203.66884379752,-0.593633067328671,
125.920149228124));
#209135=CARTESIAN_POINT('Ctrl Pts',(203.661083354951,-0.729007973603942,
125.940439315065));
#209136=CARTESIAN_POINT('Ctrl Pts',(203.653310454632,-0.864600195689189,
125.960761973454));
#209137=CARTESIAN_POINT('Ctrl Pts',(203.645537554313,-0.999198286843428,
125.986737238823));
#209138=CARTESIAN_POINT('Ctrl Pts',(203.637764653993,-1.13230545553917,
126.018227792638));
#209139=CARTESIAN_POINT('Ctrl Pts',(203.630274318817,-1.26057383246008,
126.048573582918));
#209140=CARTESIAN_POINT('Ctrl Pts',(203.62278398364,-1.38745750614367,126.084040550359));
#209141=CARTESIAN_POINT('Ctrl Pts',(203.615293648463,-1.51252874683208,
126.124463198551));
#209142=CARTESIAN_POINT('Ctrl Pts',(203.607519314355,-1.64234211159146,
126.166418486956));
#209143=CARTESIAN_POINT('Ctrl Pts',(203.599744980247,-1.77061410292081,
126.213845566141));
#209144=CARTESIAN_POINT('Ctrl Pts',(203.591970646139,-1.89684882919352,
126.266613645589));
#209145=CARTESIAN_POINT('Ctrl Pts',(203.584205893202,-2.02292798244727,
126.319316693095));
#209146=CARTESIAN_POINT('Ctrl Pts',(203.576441140266,-2.14697450902767,
126.377347494701));
#209147=CARTESIAN_POINT('Ctrl Pts',(203.56867638733,-2.2685073041796,126.440525415203));
#209148=CARTESIAN_POINT('Ctrl Pts',(203.560919346456,-2.38991939124546,
126.503640586503));
#209149=CARTESIAN_POINT('Ctrl Pts',(203.553162305581,-2.50882237072727,
126.571892524047));
#209150=CARTESIAN_POINT('Ctrl Pts',(203.545405264707,-2.62475510966509,
126.64505254088));
#209151=CARTESIAN_POINT('Ctrl Pts',(203.537654073478,-2.74060042282238,
126.718157387175));
#209152=CARTESIAN_POINT('Ctrl Pts',(203.529902882249,-2.853479624487,126.7961627379));
#209153=CARTESIAN_POINT('Ctrl Pts',(203.52215169102,-2.96295651638203,126.878794194166));
#209154=CARTESIAN_POINT('Ctrl Pts',(203.514403794253,-3.07238687767773,
126.961390529858));
#209155=CARTESIAN_POINT('Ctrl Pts',(203.506655897487,-3.17841749393087,
127.048608825393));
#209156=CARTESIAN_POINT('Ctrl Pts',(203.498908000721,-3.28064167616848,
127.140131741651));
#209157=CARTESIAN_POINT('Ctrl Pts',(203.491161724648,-3.38284447531104,
127.231635513289));
#209158=CARTESIAN_POINT('Ctrl Pts',(203.483415448574,-3.48124213307604,
127.327441854015));
#209159=CARTESIAN_POINT('Ctrl Pts',(203.475669172501,-3.57546186610856,
127.427193830671));
#209160=CARTESIAN_POINT('Ctrl Pts',(203.467922839247,-3.66968229464993,
127.526946543675));
#209161=CARTESIAN_POINT('Ctrl Pts',(203.460176505992,-3.75972446845858,
127.630644666505));
#209162=CARTESIAN_POINT('Ctrl Pts',(203.452430172738,-3.8452535159746,127.737895476661));
#209163=CARTESIAN_POINT('Ctrl Pts',(203.444682104745,-3.93080171712827,
127.845170304894));
#209164=CARTESIAN_POINT('Ctrl Pts',(203.436934036753,-4.01183453713135,
127.955999097993));
#209165=CARTESIAN_POINT('Ctrl Pts',(203.429185968761,-4.08805858483793,
128.069957562156));
#209166=CARTESIAN_POINT('Ctrl Pts',(203.42142966603,-4.16436364437073,128.184037142734));
#209167=CARTESIAN_POINT('Ctrl Pts',(203.413673363299,-4.23584950448076,
128.301252713431));
#209168=CARTESIAN_POINT('Ctrl Pts',(203.405917060567,-4.30226689243356,
128.421152139742));
#209169=CARTESIAN_POINT('Ctrl Pts',(203.398156618064,-4.3687197293466,128.541115559989));
#209170=CARTESIAN_POINT('Ctrl Pts',(203.39039617556,-4.4300985288876,128.663765340678));
#209171=CARTESIAN_POINT('Ctrl Pts',(203.382635733057,-4.48620134808193,
128.788627369597));
#209172=CARTESIAN_POINT('Ctrl Pts',(203.374862832802,-4.54239422850365,
128.913689838133));
#209173=CARTESIAN_POINT('Ctrl Pts',(203.367089932547,-4.59329405862153,
129.040971288298));
#209174=CARTESIAN_POINT('Ctrl Pts',(203.359317032292,-4.63874784045621,
129.169979531294));
#209175=CARTESIAN_POINT('Ctrl Pts',(203.351826696411,-4.68254926358041,
129.294298001835));
#209176=CARTESIAN_POINT('Ctrl Pts',(203.344336360531,-4.72129362844921,
129.420219603998));
#209177=CARTESIAN_POINT('Ctrl Pts',(203.336846024651,-4.75488897347145,
129.54729502164));
#209178=CARTESIAN_POINT('Ctrl Pts',(203.336155205243,-4.75798740813817,
129.55901494531));
#209179=CARTESIAN_POINT('Ctrl Pts',(203.335464385835,-4.76104262034663,
129.570746736167));
#209180=CARTESIAN_POINT('Ctrl Pts',(203.334773566427,-4.76405452823405,
129.582490119308));
#209181=CARTESIAN_POINT('',(205.360140563955,-4.91824853905311,130.808151475242));
#209182=CARTESIAN_POINT('Ctrl Pts',(205.360140563955,-4.91824853905311,
130.808151475242));
#209183=CARTESIAN_POINT('Ctrl Pts',(205.351139825899,-4.91812565127672,
130.967585745387));
#209184=CARTESIAN_POINT('Ctrl Pts',(205.342139087842,-4.91024632687204,
131.126698725876));
#209185=CARTESIAN_POINT('Ctrl Pts',(205.333138349785,-4.89472759256679,
131.284802973177));
#209186=CARTESIAN_POINT('Ctrl Pts',(205.324085898924,-4.87911969698644,
131.443815592));
#209187=CARTESIAN_POINT('Ctrl Pts',(205.315033448062,-4.85578446545969,
131.601807746443));
#209188=CARTESIAN_POINT('Ctrl Pts',(205.3059809972,-4.82489013514455,131.758099704678));
#209189=CARTESIAN_POINT('Ctrl Pts',(205.296866878366,-4.79378534351451,
131.915456369954));
#209190=CARTESIAN_POINT('Ctrl Pts',(205.287752759532,-4.75501819248919,
132.071089491341));
#209191=CARTESIAN_POINT('Ctrl Pts',(205.278638640698,-4.70880867544122,
132.224326786385));
#209192=CARTESIAN_POINT('Ctrl Pts',(205.274555892192,-4.68810872187624,
132.292970760494));
#209193=CARTESIAN_POINT('Ctrl Pts',(205.270473143687,-4.6659159667685,132.361134266192));
#209194=CARTESIAN_POINT('Ctrl Pts',(205.266390395182,-4.64225323707004,
132.42875833531));
#209195=CARTESIAN_POINT('Ctrl Pts',(205.25861606485,-4.59719489536611,132.557527435603));
#209196=CARTESIAN_POINT('Ctrl Pts',(205.250841734518,-4.54670333252088,
132.684624302624));
#209197=CARTESIAN_POINT('Ctrl Pts',(205.243067404185,-4.49092120076951,
132.809556326463));
#209198=CARTESIAN_POINT('Ctrl Pts',(205.235302655081,-4.43520781594627,
132.934334381772));
#209199=CARTESIAN_POINT('Ctrl Pts',(205.227537905977,-4.3742169933291,133.05695254884));
#209200=CARTESIAN_POINT('Ctrl Pts',(205.219773156873,-4.30814086066012,
133.176934196448));
#209201=CARTESIAN_POINT('Ctrl Pts',(205.212016119882,-4.24213035621027,
133.296796675734));
#209202=CARTESIAN_POINT('Ctrl Pts',(205.204259082892,-4.17104478048607,
133.414027506535));
#209203=CARTESIAN_POINT('Ctrl Pts',(205.196502045902,-4.0951238198962,133.528171176731));
#209204=CARTESIAN_POINT('Ctrl Pts',(205.188750858604,-4.0192601123862,133.642228769556));
#209205=CARTESIAN_POINT('Ctrl Pts',(205.180999671306,-3.93856849366088,
133.753203511446));
#209206=CARTESIAN_POINT('Ctrl Pts',(205.173248484008,-3.85333375056227,
133.860665914698));
#209207=CARTESIAN_POINT('Ctrl Pts',(205.165500591231,-3.76813523516348,
133.96808264273));
#209208=CARTESIAN_POINT('Ctrl Pts',(205.157752698454,-3.67839767841762,
134.071989695647));
#209209=CARTESIAN_POINT('Ctrl Pts',(205.150004805678,-3.58444808691414,
134.171988116966));
#209210=CARTESIAN_POINT('Ctrl Pts',(205.142258533629,-3.49051814807432,
134.271965620309));
#209211=CARTESIAN_POINT('Ctrl Pts',(205.134512261581,-3.39237819453857,
134.368035833586));
#209212=CARTESIAN_POINT('Ctrl Pts',(205.126765989532,-3.29039400191811,
134.459834646285));
#209213=CARTESIAN_POINT('Ctrl Pts',(205.119019660333,-3.18840905688475,
134.551634136252));
#209214=CARTESIAN_POINT('Ctrl Pts',(205.111273331135,-3.0825801067567,134.639161901196));
#209215=CARTESIAN_POINT('Ctrl Pts',(205.103527001936,-2.97330779642674,
134.722092590303));
#209216=CARTESIAN_POINT('Ctrl Pts',(205.095778938027,-2.86401101569629,
134.805041850878));
#209217=CARTESIAN_POINT('Ctrl Pts',(205.088030874119,-2.75126965172672,
134.883391750785));
#209218=CARTESIAN_POINT('Ctrl Pts',(205.08028281021,-2.63551491623087,134.956859165287));
#209219=CARTESIAN_POINT('Ctrl Pts',(205.072526511583,-2.51963715546859,
135.030404661676));
#209220=CARTESIAN_POINT('Ctrl Pts',(205.064770212956,-2.40073995618037,
135.09905709693));
#209221=CARTESIAN_POINT('Ctrl Pts',(205.057013914329,-2.27928130406476,
135.162578120105));
#209222=CARTESIAN_POINT('Ctrl Pts',(205.049253475948,-2.15775782605347,
135.226133046236));
#209223=CARTESIAN_POINT('Ctrl Pts',(205.041493037566,-2.03367052466753,
135.284550936595));
#209224=CARTESIAN_POINT('Ctrl Pts',(205.033732599185,-1.90749822121525,
135.337641283768));
#209225=CARTESIAN_POINT('Ctrl Pts',(205.025959703041,-1.78112337448988,
135.390816856402));
#209226=CARTESIAN_POINT('Ctrl Pts',(205.018186806897,-1.65265720386027,
135.438647659219));
#209227=CARTESIAN_POINT('Ctrl Pts',(205.010413910753,-1.52259542748432,
135.480992549491));
#209228=CARTESIAN_POINT('Ctrl Pts',(205.002923530958,-1.39726092104092,
135.521798357858));
#209229=CARTESIAN_POINT('Ctrl Pts',(204.995433151164,-1.27044508084342,
135.557510033643));
#209230=CARTESIAN_POINT('Ctrl Pts',(204.987942771369,-1.14259930875746,
135.588046422688));
#209231=CARTESIAN_POINT('Ctrl Pts',(204.980168435136,-1.00990696933439,
135.619740430505));
#209232=CARTESIAN_POINT('Ctrl Pts',(204.972394098903,-0.875684739349071,
135.645959422382));
#209233=CARTESIAN_POINT('Ctrl Pts',(204.964619762671,-0.740424173411585,
135.666557148552));
#209234=CARTESIAN_POINT('Ctrl Pts',(204.956855007588,-0.605330303598526,
135.687129489931));
#209235=CARTESIAN_POINT('Ctrl Pts',(204.949090252504,-0.469201026759951,
135.702094291348));
#209236=CARTESIAN_POINT('Ctrl Pts',(204.941325497421,-0.332541196813679,
135.711355565079));
#209237=CARTESIAN_POINT('Ctrl Pts',(204.93356845438,-0.196017098948459,
135.720607640409));
#209238=CARTESIAN_POINT('Ctrl Pts',(204.925811411339,-0.0589638841786129,
135.724167435013));
#209239=CARTESIAN_POINT('Ctrl Pts',(204.918054368298,0.0781056551375337,
135.721990389025));
#209240=CARTESIAN_POINT('Ctrl Pts',(204.910303174885,0.215071829587541,
135.719814984758));
#209241=CARTESIAN_POINT('Ctrl Pts',(204.902551981471,0.35205391474676,135.711911357085));
#209242=CARTESIAN_POINT('Ctrl Pts',(204.894800788057,0.488536635525835,
135.69828695725));
#209243=CARTESIAN_POINT('Ctrl Pts',(204.887052889087,0.624961347859993,
135.684668348112));
#209244=CARTESIAN_POINT('Ctrl Pts',(204.879304990118,0.760886729730015,
135.665333841567));
#209245=CARTESIAN_POINT('Ctrl Pts',(204.871557091148,0.895800372082467,
135.640342912393));
#209246=CARTESIAN_POINT('Ctrl Pts',(204.86381081286,1.03068579361427,135.615357210744));
#209247=CARTESIAN_POINT('Ctrl Pts',(204.856064534572,1.16455951239554,135.584717511067));
#209248=CARTESIAN_POINT('Ctrl Pts',(204.848318256284,1.29691748072938,135.548534740707));
#209249=CARTESIAN_POINT('Ctrl Pts',(204.840571920805,1.42927642625718,135.512351703211));
#209250=CARTESIAN_POINT('Ctrl Pts',(204.832825585326,1.56011922188006,135.470625616466));
#209251=CARTESIAN_POINT('Ctrl Pts',(204.825079249848,1.68895558188255,135.423517694883));
#209252=CARTESIAN_POINT('Ctrl Pts',(204.817331179624,1.81782079400553,135.376399223767));
#209253=CARTESIAN_POINT('Ctrl Pts',(204.809583109401,1.9446783092763,135.323896653782));
#209254=CARTESIAN_POINT('Ctrl Pts',(204.801835039178,2.06905684589674,135.26621974028));
#209255=CARTESIAN_POINT('Ctrl Pts',(204.794078734217,2.19356757344921,135.208481527095));
#209256=CARTESIAN_POINT('Ctrl Pts',(204.786322429256,2.31559370402974,135.145558149584));
#209257=CARTESIAN_POINT('Ctrl Pts',(204.778566124295,2.43468715333658,135.077706090129));
#209258=CARTESIAN_POINT('Ctrl Pts',(204.770805679558,2.55384416642928,135.009817815973));
#209259=CARTESIAN_POINT('Ctrl Pts',(204.763045234822,2.67006504819365,134.936995825692));
#209260=CARTESIAN_POINT('Ctrl Pts',(204.755284790086,2.78293070430418,134.85953999184));
#209261=CARTESIAN_POINT('Ctrl Pts',(204.747511887616,2.89597754207783,134.78195981922));
#209262=CARTESIAN_POINT('Ctrl Pts',(204.739738985146,3.00565807806422,134.699731172902));
#209263=CARTESIAN_POINT('Ctrl Pts',(204.731966082676,3.11158561669959,134.613194824045));
#209264=CARTESIAN_POINT('Ctrl Pts',(204.724475770969,3.21366206571824,134.529804580902));
#209265=CARTESIAN_POINT('Ctrl Pts',(204.716985459263,3.31225343579821,134.442414621717));
#209266=CARTESIAN_POINT('Ctrl Pts',(204.709495147556,3.40704746464756,134.351360848203));
#209267=CARTESIAN_POINT('Ctrl Pts',(204.701720813585,3.50543595201642,134.256854441481));
#209268=CARTESIAN_POINT('Ctrl Pts',(204.693946479614,3.60004509988113,134.158101516487));
#209269=CARTESIAN_POINT('Ctrl Pts',(204.686172145643,3.69048616693734,134.055436580097));
#209270=CARTESIAN_POINT('Ctrl Pts',(204.678407392841,3.78081577349329,133.952898169028));
#209271=CARTESIAN_POINT('Ctrl Pts',(204.670642640039,3.86698726395705,133.846457629871));
#209272=CARTESIAN_POINT('Ctrl Pts',(204.662877887237,3.94864699528088,133.736487826464));
#209273=CARTESIAN_POINT('Ctrl Pts',(204.655120846494,4.03022562103922,133.626627246574));
#209274=CARTESIAN_POINT('Ctrl Pts',(204.647363805751,4.107301173756,133.513244690025));
#209275=CARTESIAN_POINT('Ctrl Pts',(204.639606765008,4.17955898715758,133.396747497522));
#209276=CARTESIAN_POINT('Ctrl Pts',(204.631855573906,4.25176231040909,133.280338156412));
#209277=CARTESIAN_POINT('Ctrl Pts',(204.624104382805,4.31915492055407,133.160819185333));
#209278=CARTESIAN_POINT('Ctrl Pts',(204.616353191703,4.38146456774871,133.038628127078));
#209279=CARTESIAN_POINT('Ctrl Pts',(204.60860529506,4.44374773172442,132.916489003198));
#209280=CARTESIAN_POINT('Ctrl Pts',(204.600857398416,4.50095205236715,132.79168039854));
#209281=CARTESIAN_POINT('Ctrl Pts',(204.593109501772,4.55285059786026,132.664665564628));
#209282=CARTESIAN_POINT('Ctrl Pts',(204.585363225818,4.60473828731866,132.537677299427));
#209283=CARTESIAN_POINT('Ctrl Pts',(204.577616949864,4.65132226139587,132.4084840846));
#209284=CARTESIAN_POINT('Ctrl Pts',(204.56987067391,4.6924233962874,132.277569948406));
#209285=CARTESIAN_POINT('Ctrl Pts',(204.562124340771,4.73352483459662,132.146654845776));
#209286=CARTESIAN_POINT('Ctrl Pts',(204.554378007632,4.7691432358447,132.014019169442));
#209287=CARTESIAN_POINT('Ctrl Pts',(204.546631674493,4.7991492228434,131.880162550722));
#209288=CARTESIAN_POINT('Ctrl Pts',(204.538883606613,4.82916192948898,131.746275955676));
#209289=CARTESIAN_POINT('Ctrl Pts',(204.531135538733,4.85355963536943,131.611168255589));
#209290=CARTESIAN_POINT('Ctrl Pts',(204.523387470853,4.87226407424628,131.475349330816));
#209291=CARTESIAN_POINT('Ctrl Pts',(204.515631168227,4.89098839243932,131.339386055957));
#209292=CARTESIAN_POINT('Ctrl Pts',(204.507874865602,4.90400730292682,131.202710434351));
#209293=CARTESIAN_POINT('Ctrl Pts',(204.500118562976,4.91129439105524,131.065838086747));
#209294=CARTESIAN_POINT('Ctrl Pts',(204.492358120575,4.91858536852522,130.92889268619));
#209295=CARTESIAN_POINT('Ctrl Pts',(204.484597678174,4.92013842339908,130.791750741167));
#209296=CARTESIAN_POINT('Ctrl Pts',(204.476837235773,4.91597931619433,130.654926935789));
#209297=CARTESIAN_POINT('Ctrl Pts',(204.469064335614,4.91181353241767,130.517883488567));
#209298=CARTESIAN_POINT('Ctrl Pts',(204.461291435454,4.90191729087102,130.381159591714));
#209299=CARTESIAN_POINT('Ctrl Pts',(204.453518535295,4.88636827354715,130.245264778043));
#209300=CARTESIAN_POINT('Ctrl Pts',(204.446028198111,4.87138449911938,130.114310056498));
#209301=CARTESIAN_POINT('Ctrl Pts',(204.438537860927,4.85115184404818,129.984125490812));
#209302=CARTESIAN_POINT('Ctrl Pts',(204.431047523743,4.8257841278719,129.855155363851));
#209303=CARTESIAN_POINT('Ctrl Pts',(204.423273190132,4.79945459374589,129.721295329489));
#209304=CARTESIAN_POINT('Ctrl Pts',(204.415498856521,4.7675095188085,129.588319613196));
#209305=CARTESIAN_POINT('Ctrl Pts',(204.40772452291,4.73002020891244,129.456736083143));
#209306=CARTESIAN_POINT('Ctrl Pts',(204.399959770479,4.69257710128169,129.325314718175));
#209307=CARTESIAN_POINT('Ctrl Pts',(204.392195018048,4.64960345998627,129.195282498014));
#209308=CARTESIAN_POINT('Ctrl Pts',(204.384430265617,4.60122183314642,129.067138494556));
#209309=CARTESIAN_POINT('Ctrl Pts',(204.376673225255,4.55288825966949,128.939121765658));
#209310=CARTESIAN_POINT('Ctrl Pts',(204.368916184894,4.49915752696644,128.812989884719));
#209311=CARTESIAN_POINT('Ctrl Pts',(204.361159144532,4.44020225742291,128.689227766969));
#209312=CARTESIAN_POINT('Ctrl Pts',(204.353407953822,4.38129144656131,128.565558979308));
#209313=CARTESIAN_POINT('Ctrl Pts',(204.345656763112,4.31716410838634,128.444256749339));
#209314=CARTESIAN_POINT('Ctrl Pts',(204.337905572402,4.24804120227294,128.325786631119));
#209315=CARTESIAN_POINT('Ctrl Pts',(204.330157676164,4.17894767531605,128.207366865993));
#209316=CARTESIAN_POINT('Ctrl Pts',(204.322409779926,4.10486300002969,128.091777155478));
#209317=CARTESIAN_POINT('Ctrl Pts',(204.314661883687,4.02605426077588,127.979458822496));
#209318=CARTESIAN_POINT('Ctrl Pts',(204.306915608147,3.94726200666425,127.867163984164));
#209319=CARTESIAN_POINT('Ctrl Pts',(204.299169332607,3.86374787853738,127.758139482086));
#209320=CARTESIAN_POINT('Ctrl Pts',(204.291423057066,3.77582228221695,127.65279764729));
#209321=CARTESIAN_POINT('Ctrl Pts',(204.283676724349,3.68789603690174,127.547455034947));
#209322=CARTESIAN_POINT('Ctrl Pts',(204.275930391632,3.59555850894457,127.445795444277));
#209323=CARTESIAN_POINT('Ctrl Pts',(204.268184058915,3.49916012072415,127.348197786906));
#209324=CARTESIAN_POINT('Ctrl Pts',(204.260435991465,3.40274014480243,127.250578273267));
#209325=CARTESIAN_POINT('Ctrl Pts',(204.252687924014,3.30225777370524,127.15702278111));
#209326=CARTESIAN_POINT('Ctrl Pts',(204.244939856564,3.19809967933992,127.067872760834));
#209327=CARTESIAN_POINT('Ctrl Pts',(204.237183554378,3.09383088454986,126.978627990887));
#209328=CARTESIAN_POINT('Ctrl Pts',(204.229427252191,2.9858788601325,126.893798300623));
#209329=CARTESIAN_POINT('Ctrl Pts',(204.221670950005,2.87466313460505,126.813684619061));
#209330=CARTESIAN_POINT('Ctrl Pts',(204.21391050805,2.76338804993092,126.73352817844));
#209331=CARTESIAN_POINT('Ctrl Pts',(204.206150066094,2.64884611955096,126.658092976936));
#209332=CARTESIAN_POINT('Ctrl Pts',(204.198389624139,2.53148428592039,126.587635540846));
#209333=CARTESIAN_POINT('Ctrl Pts',(204.190616724431,2.41393405262733,126.517065000208));
#209334=CARTESIAN_POINT('Ctrl Pts',(204.182843824723,2.29355521370091,126.451488380188));
#209335=CARTESIAN_POINT('Ctrl Pts',(204.175070925015,2.17081844249119,126.391115739674));
#209336=CARTESIAN_POINT('Ctrl Pts',(204.16758058332,2.05254335990331,126.332937746457));
#209337=CARTESIAN_POINT('Ctrl Pts',(204.160090241625,1.932079080105,126.279592079101));
#209338=CARTESIAN_POINT('Ctrl Pts',(204.15259989993,1.80986091391834,126.231223124032));
#209339=CARTESIAN_POINT('Ctrl Pts',(204.144825565478,1.68300890386598,126.181020282947));
#209340=CARTESIAN_POINT('Ctrl Pts',(204.137051231027,1.55386555861245,126.136019952371));
#209341=CARTESIAN_POINT('Ctrl Pts',(204.129276896576,1.42289670472903,126.096436655757));
#209342=CARTESIAN_POINT('Ctrl Pts',(204.121512143292,1.2920892581833,126.056902141999));
#209343=CARTESIAN_POINT('Ctrl Pts',(204.113747390009,1.15946115004296,126.022771490962));
#209344=CARTESIAN_POINT('Ctrl Pts',(204.105982636726,1.02549850401181,125.994211359927));
#209345=CARTESIAN_POINT('Ctrl Pts',(204.098225595501,0.891668911505565,
125.965679595202));
#209346=CARTESIAN_POINT('Ctrl Pts',(204.090468554277,0.756507798773581,
125.942707421116));
#209347=CARTESIAN_POINT('Ctrl Pts',(204.082711513052,0.620516445466882,
125.925411714021));
#209348=CARTESIAN_POINT('Ctrl Pts',(204.07496032147,0.484627644240924,125.908129049746));
#209349=CARTESIAN_POINT('Ctrl Pts',(204.067209129887,0.347910234907202,
125.896514381183));
#209350=CARTESIAN_POINT('Ctrl Pts',(204.059457938304,0.210875335327797,
125.890633452221));
#209351=CARTESIAN_POINT('Ctrl Pts',(204.051710041182,0.0738986791749443,
125.884755022807));
#209352=CARTESIAN_POINT('Ctrl Pts',(204.043962144059,-0.0633948090470082,
125.884605502735));
#209353=CARTESIAN_POINT('Ctrl Pts',(204.036214246936,-0.200489466144424,
125.89019873211));
#209354=CARTESIAN_POINT('Ctrl Pts',(204.028467970504,-0.337555446031198,
125.895790791504));
#209355=CARTESIAN_POINT('Ctrl Pts',(204.020721694072,-0.474422287127775,
125.907123195051));
#209356=CARTESIAN_POINT('Ctrl Pts',(204.01297541764,-0.61057530164394,125.924157664458));
#209357=CARTESIAN_POINT('Ctrl Pts',(204.005229084025,-0.746729321239624,
125.941192259614));
#209358=CARTESIAN_POINT('Ctrl Pts',(203.997482750411,-0.882169115799372,
125.963928956088));
#209359=CARTESIAN_POINT('Ctrl Pts',(203.989736416796,-1.0163864843013,125.992277744523));
#209360=CARTESIAN_POINT('Ctrl Pts',(203.981988348442,-1.15063390987372,
126.020632881478));
#209361=CARTESIAN_POINT('Ctrl Pts',(203.974240280088,-1.28365798219704,
126.054602530483));
#209362=CARTESIAN_POINT('Ctrl Pts',(203.966492211735,-1.41496242369231,
126.094045935717));
#209363=CARTESIAN_POINT('Ctrl Pts',(203.958735908642,-1.54640641710633,
126.133531261871));
#209364=CARTESIAN_POINT('Ctrl Pts',(203.950979605549,-1.67612675374356,
126.178501852826));
#209365=CARTESIAN_POINT('Ctrl Pts',(203.943223302457,-1.80364348801349,
126.228767406774));
#209366=CARTESIAN_POINT('Ctrl Pts',(203.935462859591,-1.93122828181124,
126.279059788964));
#209367=CARTESIAN_POINT('Ctrl Pts',(203.927702416725,-2.05660677247295,
126.334652606956));
#209368=CARTESIAN_POINT('Ctrl Pts',(203.91994197386,-2.17932155377599,126.395308494065));
#209369=CARTESIAN_POINT('Ctrl Pts',(203.912169073245,-2.30223332769157,
126.456061751365));
#209370=CARTESIAN_POINT('Ctrl Pts',(203.904396172631,-2.42247250426769,
126.521894131622));
#209371=CARTESIAN_POINT('Ctrl Pts',(203.896623272017,-2.53960794450345,
126.592523185908));
#209372=CARTESIAN_POINT('Ctrl Pts',(203.88913294005,-2.65248515417354,126.660584658622));
#209373=CARTESIAN_POINT('Ctrl Pts',(203.881642608084,-2.76248011304978,
126.733099943225));
#209374=CARTESIAN_POINT('Ctrl Pts',(203.874152276117,-2.86923605004317,
126.809780845971));
#209375=CARTESIAN_POINT('Ctrl Pts',(203.866074034918,-2.98437116185463,
126.892480361897));
#209376=CARTESIAN_POINT('Ctrl Pts',(203.857995793719,-3.09613368668095,
126.980309741443));
#209377=CARTESIAN_POINT('Ctrl Pts',(203.84991755252,-3.20403203740082,127.07295849962));
#209378=CARTESIAN_POINT('Ctrl Pts',(203.842215517175,-3.30690553306662,
127.161292580348));
#209379=CARTESIAN_POINT('Ctrl Pts',(203.834513481829,-3.40626624325742,
127.25400703648));
#209380=CARTESIAN_POINT('Ctrl Pts',(203.826811446484,-3.50171630356533,
127.350787686261));
#209381=CARTESIAN_POINT('Ctrl Pts',(203.819116363939,-3.59708019895571,
127.447480969971));
#209382=CARTESIAN_POINT('Ctrl Pts',(203.811421281394,-3.68854018756952,
127.548232866472));
#209383=CARTESIAN_POINT('Ctrl Pts',(203.803726198849,-3.77573196917681,
127.65268944826));
#209384=CARTESIAN_POINT('Ctrl Pts',(203.796036329942,-3.8628646758669,127.757075257736));
#209385=CARTESIAN_POINT('Ctrl Pts',(203.788346461035,-3.94573467410029,
127.86516045547));
#209386=CARTESIAN_POINT('Ctrl Pts',(203.780656592127,-4.02401534417658,
127.976555183606));
#209387=CARTESIAN_POINT('Ctrl Pts',(203.772970201974,-4.10226060153588,
128.087899518843));
#209388=CARTESIAN_POINT('Ctrl Pts',(203.76528381182,-4.17592043400376,128.202550080349));
#209389=CARTESIAN_POINT('Ctrl Pts',(203.757597421666,-4.24470957225871,
128.320085328941));
#209390=CARTESIAN_POINT('Ctrl Pts',(203.749911435145,-4.31349509821327,
128.437614405444));
#209391=CARTESIAN_POINT('Ctrl Pts',(203.742225448624,-4.37741023070302,
128.558027528844));
#209392=CARTESIAN_POINT('Ctrl Pts',(203.734539462103,-4.4362141058302,128.680875870803));
#209393=CARTESIAN_POINT('Ctrl Pts',(203.726853680479,-4.49501641333659,
128.803720937816));
#209394=CARTESIAN_POINT('Ctrl Pts',(203.719167898855,-4.54870756838372,
128.929000732856));
#209395=CARTESIAN_POINT('Ctrl Pts',(203.71148211723,-4.59709392678213,129.056244348308));
#209396=CARTESIAN_POINT('Ctrl Pts',(203.703792765134,-4.64550276332794,
129.183547075479));
#209397=CARTESIAN_POINT('Ctrl Pts',(203.696103413038,-4.68860174757454,
129.312815070517));
#209398=CARTESIAN_POINT('Ctrl Pts',(203.688414060942,-4.72624641962959,
129.443560175386));
#209399=CARTESIAN_POINT('Ctrl Pts',(203.685700869741,-4.73952935838289,
129.489693641968));
#209400=CARTESIAN_POINT('Ctrl Pts',(203.682987678541,-4.752133674154,129.536010890174));
#209401=CARTESIAN_POINT('Ctrl Pts',(203.680274487341,-4.76405452823405,
129.582490119308));
#209402=CARTESIAN_POINT('Ctrl Pts',(205.430026442963,-4.76405452823405,
129.582490119308));
#209403=CARTESIAN_POINT('Ctrl Pts',(205.422281762578,-4.79814669522109,
129.71541496097));
#209404=CARTESIAN_POINT('Ctrl Pts',(205.414537082193,-4.82668292020064,
129.849812538585));
#209405=CARTESIAN_POINT('Ctrl Pts',(205.406792401809,-4.8495489326977,129.985179189633));
#209406=CARTESIAN_POINT('Ctrl Pts',(205.399017095509,-4.87250536759203,
130.121081140708));
#209407=CARTESIAN_POINT('Ctrl Pts',(205.391241789208,-4.88974655166597,
130.257959461279));
#209408=CARTESIAN_POINT('Ctrl Pts',(205.383466482908,-4.90120888938085,
130.395295237518));
#209409=CARTESIAN_POINT('Ctrl Pts',(205.375691176608,-4.91267122709574,
130.532631013756));
#209410=CARTESIAN_POINT('Ctrl Pts',(205.367915870308,-4.91835469588896,
130.670423848268));
#209411=CARTESIAN_POINT('Ctrl Pts',(205.360140564008,-4.91824853905384,
130.808151474305));
#209412=CARTESIAN_POINT('Origin',(213.235140564004,0.,130.804360617566));
#209413=CARTESIAN_POINT('',(207.179891338435,-4.76405452823405,129.582490119308));
#209414=CARTESIAN_POINT('',(206.834782106149,-4.76405452823405,129.582490119308));
#209415=CARTESIAN_POINT('',(213.235140564004,-4.76405452823405,129.582490119308));
#209416=CARTESIAN_POINT('',(207.388365636076,-2.6602809725928,126.667684632024));
#209417=CARTESIAN_POINT('Ctrl Pts',(207.388365636076,-2.66028097259279,
126.667684632024));
#209418=CARTESIAN_POINT('Ctrl Pts',(207.380618347121,-2.7756419670554,126.741872859388));
#209419=CARTESIAN_POINT('Ctrl Pts',(207.372871058166,-2.88794064863019,
126.820918329725));
#209420=CARTESIAN_POINT('Ctrl Pts',(207.365123769211,-2.99675018972373,
126.904530959377));
#209421=CARTESIAN_POINT('Ctrl Pts',(207.357377200615,-3.10554961348789,
126.988135814559));
#209422=CARTESIAN_POINT('Ctrl Pts',(207.349630632018,-3.21086023212209,
127.076306746294));
#209423=CARTESIAN_POINT('Ctrl Pts',(207.341884063422,-3.31228656623825,
127.168712014412));
#209424=CARTESIAN_POINT('Ctrl Pts',(207.334136538062,-3.41372542731635,
127.261128695318));
#209425=CARTESIAN_POINT('Ctrl Pts',(207.326389012703,-3.51127876024814,
127.357780490032));
#209426=CARTESIAN_POINT('Ctrl Pts',(207.318641487343,-3.60458666572251,
127.458297553038));
#209427=CARTESIAN_POINT('Ctrl Pts',(207.31089132783,-3.69792629581925,127.558848791775));
#209428=CARTESIAN_POINT('Ctrl Pts',(207.303141168318,-3.78701736032166,
127.663267627633));
#209429=CARTESIAN_POINT('Ctrl Pts',(207.295391008805,-3.8715393602353,127.771150099872));
#209430=CARTESIAN_POINT('Ctrl Pts',(207.287632207676,-3.95615560423753,
127.879152863696));
#209431=CARTESIAN_POINT('Ctrl Pts',(207.279873406546,-4.03619237033408,
127.990626667092));
#209432=CARTESIAN_POINT('Ctrl Pts',(207.272114605417,-4.11137146976527,
128.105137081047));
#209433=CARTESIAN_POINT('Ctrl Pts',(207.264350856575,-4.18659851018636,
128.219720517193));
#209434=CARTESIAN_POINT('Ctrl Pts',(207.256587107732,-4.25696151306608,
128.33734408662));
#209435=CARTESIAN_POINT('Ctrl Pts',(207.24882335889,-4.3222281122226,128.457548480131));
#209436=CARTESIAN_POINT('Ctrl Pts',(207.24104833483,-4.38758949743189,128.577927445323));
#209437=CARTESIAN_POINT('Ctrl Pts',(207.23327331077,-4.44783952903662,128.700894368445));
#209438=CARTESIAN_POINT('Ctrl Pts',(207.22549828671,-4.5027936406439,128.825969227503));
#209439=CARTESIAN_POINT('Ctrl Pts',(207.222173445098,-4.52629372445711,
128.879455119364));
#209440=CARTESIAN_POINT('Ctrl Pts',(207.218848603485,-4.54882597142772,
128.93332628573));
#209441=CARTESIAN_POINT('Ctrl Pts',(207.215523761872,-4.57037874948208,
128.987544405402));
#209442=CARTESIAN_POINT('Ctrl Pts',(207.206734347059,-4.6273547888774,129.130873201093));
#209443=CARTESIAN_POINT('Ctrl Pts',(207.197944932245,-4.67763395894565,
129.2770080242));
#209444=CARTESIAN_POINT('Ctrl Pts',(207.189155517432,-4.72096468861576,
129.425348118949));
#209445=CARTESIAN_POINT('Ctrl Pts',(207.186067457766,-4.73618844143788,
129.47746570278));
#209446=CARTESIAN_POINT('Ctrl Pts',(207.1829793981,-4.75055490266602,129.529855284104));
#209447=CARTESIAN_POINT('Ctrl Pts',(207.179891338435,-4.76405452823404,
129.582490119308));
#209448=CARTESIAN_POINT('',(207.162232148078,-0.703339529199327,125.936661307916));
#209449=CARTESIAN_POINT('Ctrl Pts',(207.162254451653,-0.702949340845361,
125.936604945112));
#209450=CARTESIAN_POINT('Ctrl Pts',(207.181804583648,-1.10465555699531,
125.994615071104));
#209451=CARTESIAN_POINT('Ctrl Pts',(207.218751347755,-1.507343617162,126.104644931362));
#209452=CARTESIAN_POINT('Ctrl Pts',(207.303215754353,-2.15815824480352,
126.375258708658));
#209453=CARTESIAN_POINT('Ctrl Pts',(207.344364632467,-2.41764010127658,
126.511643188268));
#209454=CARTESIAN_POINT('Ctrl Pts',(207.388365636076,-2.66028097259279,
126.667684632024));
#209455=CARTESIAN_POINT('Ctrl Pts',(207.162232148078,-0.703339529199318,
125.936661307916));
#209456=CARTESIAN_POINT('Ctrl Pts',(207.154481493481,-0.838932135396659,
125.956253241135));
#209457=CARTESIAN_POINT('Ctrl Pts',(207.146730838883,-0.973806675997351,
125.981529605001));
#209458=CARTESIAN_POINT('Ctrl Pts',(207.138980184285,-1.10745311122064,
126.012416265954));
#209459=CARTESIAN_POINT('Ctrl Pts',(207.131232508695,-1.24104817869023,
126.043291055446));
#209460=CARTESIAN_POINT('Ctrl Pts',(207.123484833105,-1.37341569924148,
126.079771766144));
#209461=CARTESIAN_POINT('Ctrl Pts',(207.115737157515,-1.5040552264814,126.121733049822));
#209462=CARTESIAN_POINT('Ctrl Pts',(207.10799088649,-1.63467107025817,126.163686726396));
#209463=CARTESIAN_POINT('Ctrl Pts',(207.100244615465,-1.7635591717869,126.211118880199));
#209464=CARTESIAN_POINT('Ctrl Pts',(207.092498344441,-1.89023407151358,
126.2638542342));
#209465=CARTESIAN_POINT('Ctrl Pts',(207.084751800286,-2.01691343773256,
126.316591447622));
#209466=CARTESIAN_POINT('Ctrl Pts',(207.077005256132,-2.14137908586176,
126.374632083229));
#209467=CARTESIAN_POINT('Ctrl Pts',(207.069258711978,-2.2631657454553,126.437752795572));
#209468=CARTESIAN_POINT('Ctrl Pts',(207.061510217176,-2.38498307199125,
126.50088940226));
#209469=CARTESIAN_POINT('Ctrl Pts',(207.053761722375,-2.50411972061654,
126.569108451315));
#209470=CARTESIAN_POINT('Ctrl Pts',(207.046013227573,-2.6201355790416,126.64214094413));
#209471=CARTESIAN_POINT('Ctrl Pts',(207.038256395599,-2.73627626742322,
126.715252017951));
#209472=CARTESIAN_POINT('Ctrl Pts',(207.030499563624,-2.84928912735338,
126.793186671612));
#209473=CARTESIAN_POINT('Ctrl Pts',(207.02274273165,-2.95876314281126,126.875632613842));
#209474=CARTESIAN_POINT('Ctrl Pts',(207.014981565943,-3.06829832127006,
126.958124618521));
#209475=CARTESIAN_POINT('Ctrl Pts',(207.007220400236,-3.17429041402738,
127.045132685755));
#209476=CARTESIAN_POINT('Ctrl Pts',(206.999459234529,-3.27636279218891,
127.13630528586));
#209477=CARTESIAN_POINT('Ctrl Pts',(206.991685903546,-3.37859516417064,
127.227620794877));
#209478=CARTESIAN_POINT('Ctrl Pts',(206.983912572564,-3.47689526586364,
127.323113606467));
#209479=CARTESIAN_POINT('Ctrl Pts',(206.976139241582,-3.57092397027851,
127.422395942855));
#209480=CARTESIAN_POINT('Ctrl Pts',(206.969647872461,-3.64944565290829,
127.50530483921));
#209481=CARTESIAN_POINT('Ctrl Pts',(206.963156503339,-3.72498926082491,
127.59085569901));
#209482=CARTESIAN_POINT('Ctrl Pts',(206.956665134218,-3.79738005623955,
127.678806623316));
#209483=CARTESIAN_POINT('Ctrl Pts',(206.94892298064,-3.88371941628531,127.783704303698));
#209484=CARTESIAN_POINT('Ctrl Pts',(206.941180827061,-3.96585449861086,
127.892359049907));
#209485=CARTESIAN_POINT('Ctrl Pts',(206.933438673483,-4.04343822436111,
128.004398048481));
#209486=CARTESIAN_POINT('Ctrl Pts',(206.925706075313,-4.12092619585383,
128.116298767913));
#209487=CARTESIAN_POINT('Ctrl Pts',(206.917973477143,-4.19387376171754,
128.231575110577));
#209488=CARTESIAN_POINT('Ctrl Pts',(206.910240878973,-4.26197290981029,
128.349819931706));
#209489=CARTESIAN_POINT('Ctrl Pts',(206.902517710807,-4.32998901010194,
128.46792055173));
#209490=CARTESIAN_POINT('Ctrl Pts',(206.894794542642,-4.39316827069869,
128.588982102231));
#209491=CARTESIAN_POINT('Ctrl Pts',(206.887071374476,-4.45124539391761,
128.712567724943));
#209492=CARTESIAN_POINT('Ctrl Pts',(206.879353629328,-4.50928173682043,
128.836066568895));
#209493=CARTESIAN_POINT('Ctrl Pts',(206.871635884179,-4.56222290117221,
128.962085604512));
#209494=CARTESIAN_POINT('Ctrl Pts',(206.863918139031,-4.60984903857043,
129.090162582305));
#209495=CARTESIAN_POINT('Ctrl Pts',(206.85620451266,-4.65744975902884,129.218171208454));
#209496=CARTESIAN_POINT('Ctrl Pts',(206.848490886289,-4.69974096176777,
129.348235221747));
#209497=CARTESIAN_POINT('Ctrl Pts',(206.840777259918,-4.73655075729556,
129.47987204228));
#209498=CARTESIAN_POINT('Ctrl Pts',(206.838778875329,-4.74608714453973,
129.513975456282));
#209499=CARTESIAN_POINT('Ctrl Pts',(206.836780490739,-4.75525588437593,
129.548184340444));
#209500=CARTESIAN_POINT('Ctrl Pts',(206.834782106149,-4.76405452823405,
129.582490119308));
#209501=CARTESIAN_POINT('Ctrl Pts',(210.578629502474,3.43871735229388,135.623751273273));
#209502=CARTESIAN_POINT('Ctrl Pts',(210.532211638871,4.24191310225744,135.050661598608));
#209503=CARTESIAN_POINT('Ctrl Pts',(210.439385837966,5.5417116830592,133.497735776206));
#209504=CARTESIAN_POINT('Ctrl Pts',(210.253744162458,6.40049231640402,129.500124813146));
#209505=CARTESIAN_POINT('Ctrl Pts',(210.021704475947,3.49988613106459,124.739836436729));
#209506=CARTESIAN_POINT('Ctrl Pts',(209.743256852134,-3.22132718841443,
124.582443963435));
#209507=CARTESIAN_POINT('Ctrl Pts',(209.464809228321,-6.97029916743427,
130.151104711613));
#209508=CARTESIAN_POINT('Ctrl Pts',(209.186361604508,-4.320155850937,136.315756482887));
#209509=CARTESIAN_POINT('Ctrl Pts',(208.907913980696,2.30329626696544,137.417975354914));
#209510=CARTESIAN_POINT('Ctrl Pts',(208.629466356883,6.80838731381026,132.441404887444));
#209511=CARTESIAN_POINT('Ctrl Pts',(208.35101873307,5.05782663488002,125.961106241921));
#209512=CARTESIAN_POINT('Ctrl Pts',(208.072571109257,-1.34111875541754,
123.931185212061));
#209513=CARTESIAN_POINT('Ctrl Pts',(207.794123485444,-6.50738248846785,
128.217554840719));
#209514=CARTESIAN_POINT('Ctrl Pts',(207.515675861631,-5.69381680528821,
134.880978212762));
#209515=CARTESIAN_POINT('Ctrl Pts',(207.237228237818,0.352161018465804,
137.798239159538));
#209516=CARTESIAN_POINT('Ctrl Pts',(206.958780614005,6.07448159193836,134.288440920842));
#209517=CARTESIAN_POINT('Ctrl Pts',(206.680332990192,6.21467071562046,127.576957111676));
#209518=CARTESIAN_POINT('Ctrl Pts',(206.40188536638,0.643870262773591,123.831292031177));
#209519=CARTESIAN_POINT('Ctrl Pts',(206.123437742567,-5.51860979104455,
126.493540260974));
#209520=CARTESIAN_POINT('Ctrl Pts',(205.844990118754,-6.60976007302988,
133.117219720399));
#209521=CARTESIAN_POINT('Ctrl Pts',(205.566542494941,-1.62686214948821,
137.615495756827));
#209522=CARTESIAN_POINT('Ctrl Pts',(205.288094871128,4.8510417637676,135.85467075854));
#209523=CARTESIAN_POINT('Ctrl Pts',(205.009647247315,6.87107573233629,129.452857771449));
#209524=CARTESIAN_POINT('Ctrl Pts',(204.731199623502,2.57692653546199,124.293009711503));
#209525=CARTESIAN_POINT('Ctrl Pts',(204.452751999689,-4.08529213152394,
125.116775123829));
#209526=CARTESIAN_POINT('Ctrl Pts',(204.174304375876,-6.9933269740478,131.167153704944));
#209527=CARTESIAN_POINT('Ctrl Pts',(203.895856752063,-3.47483593506387,
136.884143186524));
#209528=CARTESIAN_POINT('Ctrl Pts',(203.617409128251,3.23685955433703,137.014109488232));
#209529=CARTESIAN_POINT('Ctrl Pts',(203.338961504438,6.97403925260401,131.437619947721));
#209530=CARTESIAN_POINT('Ctrl Pts',(203.060513880625,4.30241757323156,125.27919601562));
#209531=CARTESIAN_POINT('Ctrl Pts',(202.782066256812,-2.32291566837452,
124.198128435325));
#209532=CARTESIAN_POINT('Ctrl Pts',(202.503618632999,-6.81360289295739,
129.18786549711));
#209533=CARTESIAN_POINT('Ctrl Pts',(202.225171009186,-5.0429219211382,135.663082604955));
#209534=CARTESIAN_POINT('Ctrl Pts',(201.946723385373,1.36195793536179,137.673371567868));
#209535=CARTESIAN_POINT('Ctrl Pts',(201.66827576156,6.51526498482727,133.371375037445));
#209536=CARTESIAN_POINT('Ctrl Pts',(201.389828137747,5.6813618015098,126.710417660699));
#209537=CARTESIAN_POINT('Ctrl Pts',(201.111380513935,-0.373435327379839,
123.811593861123));
#209538=CARTESIAN_POINT('Ctrl Pts',(200.832932890122,-6.08506363376988,
127.338781095048));
#209539=CARTESIAN_POINT('Ctrl Pts',(200.554485266309,-6.20481573259303,
134.050666607207));
#209540=CARTESIAN_POINT('Ctrl Pts',(200.276037642496,-0.622645295272457,
137.779355505743));
#209541=CARTESIAN_POINT('Ctrl Pts',(199.997590018683,5.53170575049466,135.098364849491));
#209542=CARTESIAN_POINT('Ctrl Pts',(199.71914239487,6.60268945040398,128.471394077867));
#209543=CARTESIAN_POINT('Ctrl Pts',(199.440694771057,1.60612410470526,123.988305584475));
#209544=CARTESIAN_POINT('Ctrl Pts',(199.162247147244,-4.86639082969376,
125.768838683693));
#209545=CARTESIAN_POINT('Ctrl Pts',(198.883799523432,-6.86693032801245,
132.176770441218));
#209546=CARTESIAN_POINT('Ctrl Pts',(198.605351899619,-2.5570963230842,137.323524616753));
#209547=CARTESIAN_POINT('Ctrl Pts',(198.326904275806,4.10258428165832,136.479485555902));
#209548=CARTESIAN_POINT('Ctrl Pts',(198.048456651993,6.99219035394115,130.420283921986));
#209549=CARTESIAN_POINT('Ctrl Pts',(197.77000902818,3.45631507844086,124.714030008118));
#209550=CARTESIAN_POINT('Ctrl Pts',(197.491561404367,-3.25574490376804,
124.604492395141));
#209551=CARTESIAN_POINT('Ctrl Pts',(197.213113780554,-6.97593437139489,
130.192330798173));
#209552=CARTESIAN_POINT('Ctrl Pts',(196.934666156741,-4.28558094504976,
136.342594705906));
#209553=CARTESIAN_POINT('Ctrl Pts',(196.656218532928,2.3430120075278,137.403492044232));
#209554=CARTESIAN_POINT('Ctrl Pts',(196.377770909115,6.81849138768721,132.400109986944));
#209555=CARTESIAN_POINT('Ctrl Pts',(196.099323285303,5.02811028438465,125.930312215887));
#209556=CARTESIAN_POINT('Ctrl Pts',(195.82087566149,-1.38285853342424,123.939526815472));
#209557=CARTESIAN_POINT('Ctrl Pts',(195.542428037677,-6.5230479154113,128.257188313404));
#209558=CARTESIAN_POINT('Ctrl Pts',(195.263980413864,-5.66887493174189,
134.915576722577));
#209559=CARTESIAN_POINT('Ctrl Pts',(194.985532790051,0.394717174261835,
137.795958375315));
#209560=CARTESIAN_POINT('Ctrl Pts',(194.707085166238,6.09558348012494,134.251403247221));
#209561=CARTESIAN_POINT('Ctrl Pts',(194.428637542425,6.19490635356113,127.539184339867));
#209562=CARTESIAN_POINT('Ctrl Pts',(194.150189918612,0.601412926074683,
123.827502918989));
#209563=CARTESIAN_POINT('Ctrl Pts',(193.871742294799,-5.54474959981957,
126.527212884656));
#209564=CARTESIAN_POINT('Ctrl Pts',(193.593294670987,-6.59555811955654,
133.157412666584));
#209565=CARTESIAN_POINT('Ctrl Pts',(193.314847047174,-1.58537093834796,
137.625272568447));
#209566=CARTESIAN_POINT('Ctrl Pts',(193.036399423361,4.88169468552635,135.825047607524));
#209567=CARTESIAN_POINT('Ctrl Pts',(192.757951799548,6.86272137744547,129.411056577024));
#209568=CARTESIAN_POINT('Ctrl Pts',(192.479504175735,2.53724238606986,124.277443893095));
#209569=CARTESIAN_POINT('Ctrl Pts',(192.201056551922,-4.11983840692253,
125.141748821346));
#209570=CARTESIAN_POINT('Ctrl Pts',(191.922608928109,-6.99098896924831,
131.209717356357));
#209571=CARTESIAN_POINT('Ctrl Pts',(191.644161304296,-3.43776219763276,
136.905182851196));
#209572=CARTESIAN_POINT('Ctrl Pts',(191.365713680483,3.27460008958736,136.994290755064));
#209573=CARTESIAN_POINT('Ctrl Pts',(191.08726605667,6.9777648675845,131.395155257469));
#209574=CARTESIAN_POINT('Ctrl Pts',(190.808818432858,4.26870461503614,125.253108347726));
#209575=CARTESIAN_POINT('Ctrl Pts',(190.530370809044,-2.36308664091672,
124.212391080215));
#209576=CARTESIAN_POINT('Ctrl Pts',(190.251923185232,-6.82331671706736,
129.229371781915));
#209577=CARTESIAN_POINT('Ctrl Pts',(189.973475561419,-5.01325206778612,
135.693690281095));
#209578=CARTESIAN_POINT('Ctrl Pts',(189.695027937606,1.40374632081163,137.664953676525));
#209579=CARTESIAN_POINT('Ctrl Pts',(189.416580313793,6.53077041740369,133.331667209374));
#209580=CARTESIAN_POINT('Ctrl Pts',(189.13813268998,5.65633554627347,126.675909450142));
#209581=CARTESIAN_POINT('Ctrl Pts',(188.859685066167,-0.41599536452862,
123.81399662772));
#209582=CARTESIAN_POINT('Ctrl Pts',(188.581237442354,-6.10604685783229,
127.375886813701));
#209583=CARTESIAN_POINT('Ctrl Pts',(188.302789818542,-6.18493958576042,
134.088376935175));
#209584=CARTESIAN_POINT('Ctrl Pts',(188.024342194729,-0.580174985471077,
137.783016493883));
#209585=CARTESIAN_POINT('Ctrl Pts',(187.745894570916,5.55774208334242,135.064612228548));
#209586=CARTESIAN_POINT('Ctrl Pts',(187.467446947103,6.58836568835925,128.431244857581));
#209587=CARTESIAN_POINT('Ctrl Pts',(187.18899932329,1.56460308533104,123.97865493689));
#209588=CARTESIAN_POINT('Ctrl Pts',(186.910551699478,-4.89695331800637,
125.798555082479));
#209589=CARTESIAN_POINT('Ctrl Pts',(186.632104075664,-6.85844885156509,
132.218545967617));
#209590=CARTESIAN_POINT('Ctrl Pts',(186.353656451852,-2.51736494438869,
137.338969602853));
#209591=CARTESIAN_POINT('Ctrl Pts',(186.075208828038,4.13705436656654,136.454406814005));
#209592=CARTESIAN_POINT('Ctrl Pts',(185.796761204226,6.98972282098866,130.377727590732));
#209593=CARTESIAN_POINT('Ctrl Pts',(185.518313580413,3.41917746986535,124.693103276936));
#209594=CARTESIAN_POINT('Ctrl Pts',(185.2398659566,-3.29342493995873,124.62442590766));
#209595=CARTESIAN_POINT('Ctrl Pts',(184.961418332787,-6.97953072271363,
130.234806630193));
#209596=CARTESIAN_POINT('Ctrl Pts',(184.682970708974,-4.25178874032612,
136.368579642862));
#209597=CARTESIAN_POINT('Ctrl Pts',(184.404523085161,2.38313938299372,137.389107198495));
#209598=CARTESIAN_POINT('Ctrl Pts',(184.126075461348,6.82807883617355,132.358574329007));
#209599=CARTESIAN_POINT('Ctrl Pts',(183.847627837535,4.99834740910532,125.899794986266));
#209600=CARTESIAN_POINT('Ctrl Pts',(183.569180213722,-1.42462110408482,
123.948071857337));
#209601=CARTESIAN_POINT('Ctrl Pts',(183.290732589909,-6.53843241923107,
128.296943150732));
#209602=CARTESIAN_POINT('Ctrl Pts',(183.012284966097,-5.64374376128527,
134.950008601993));
#209603=CARTESIAN_POINT('Ctrl Pts',(182.733837342284,0.437269701071178,
137.793426081729));
#209604=CARTESIAN_POINT('Ctrl Pts',(182.455389718471,6.11645366995566,134.214233834728));
#209605=CARTESIAN_POINT('Ctrl Pts',(182.176942094658,6.17491552152431,127.501534682722));
#209606=CARTESIAN_POINT('Ctrl Pts',(181.898494470845,0.558931670205695,
123.82397121282));
#209607=CARTESIAN_POINT('Ctrl Pts',(181.620046847032,-5.57068308070185,
126.561044594899));
#209608=CARTESIAN_POINT('Ctrl Pts',(181.341599223219,-6.58111222344223,
133.197518104296));
#209609=CARTESIAN_POINT('Ctrl Pts',(181.063151599407,-1.54382073804491,
137.634796795631));
#209610=CARTESIAN_POINT('Ctrl Pts',(180.784703975594,4.91216658577983,135.795238324681));
#209611=CARTESIAN_POINT('Ctrl Pts',(180.506256351781,6.85411278995147,129.369307058824));
#209612=CARTESIAN_POINT('Ctrl Pts',(180.227808727968,2.49746418218255,124.262119907186));
#209613=CARTESIAN_POINT('Ctrl Pts',(179.949361104155,-4.15423200110403,
125.16693236216));
#209614=CARTESIAN_POINT('Ctrl Pts',(179.670913480342,-6.98839192089168,
131.252265980172));
#209615=CARTESIAN_POINT('Ctrl Pts',(179.392465856529,-3.40056106730489,
136.925996451342));
#209616=CARTESIAN_POINT('Ctrl Pts',(179.114018232716,3.31221928049139,136.974242649806));
#209617=CARTESIAN_POINT('Ctrl Pts',(178.835570608904,6.98123192042358,131.352668676138));
#209618=CARTESIAN_POINT('Ctrl Pts',(178.55712298509,4.23483347762603,125.227226382977));
#209619=CARTESIAN_POINT('Ctrl Pts',(178.278675361277,-2.40317004799311,
124.22689799325));
#209620=CARTESIAN_POINT('Ctrl Pts',(178.000227737465,-6.83277770089014,
129.270936428355));
#209621=CARTESIAN_POINT('Ctrl Pts',(177.721780113652,-4.98339644641697,
135.724116781409));
#209622=CARTESIAN_POINT('Ctrl Pts',(177.443332489839,1.44548268986267,137.65628156334));
#209623=CARTESIAN_POINT('Ctrl Pts',(177.164884866026,6.54603384991367,133.291865731052));
#209624=CARTESIAN_POINT('Ctrl Pts',(176.886437242213,5.63109969342586,126.64155422085));
#209625=CARTESIAN_POINT('Ctrl Pts',(176.6079896184,-0.458539986806858,123.816658424832));
#209626=CARTESIAN_POINT('Ctrl Pts',(176.329541994587,-6.12680382008778,
127.413119575705));
#209627=CARTESIAN_POINT('Ctrl Pts',(176.051094370774,-6.16483425371434,
134.125965572714));
#209628=CARTESIAN_POINT('Ctrl Pts',(175.772646746962,-0.537683177073775,
137.786418885364));
#209629=CARTESIAN_POINT('Ctrl Pts',(175.494199123148,5.58357247201413,135.030701742416));
#209630=CARTESIAN_POINT('Ctrl Pts',(175.215751499336,6.57379779200069,128.391183573973));
#209631=CARTESIAN_POINT('Ctrl Pts',(174.937303875523,1.5230240890144,123.969257218339));
#209632=CARTESIAN_POINT('Ctrl Pts',(174.65885625171,-4.92733434791298,125.82845697323));
#209633=CARTESIAN_POINT('Ctrl Pts',(174.380408627897,-6.84971323277332,
132.260269090858));
#209634=CARTESIAN_POINT('Ctrl Pts',(174.101961004084,-2.4775402838095,137.354172446613));
#209635=CARTESIAN_POINT('Ctrl Pts',(173.823513380271,4.1713711514037,136.429118707571));
#209636=CARTESIAN_POINT('Ctrl Pts',(173.545065756458,6.98699628128659,130.335187068521));
#209637=CARTESIAN_POINT('Ctrl Pts',(173.266618132645,3.38191316241135,124.672403000642));
#209638=CARTESIAN_POINT('Ctrl Pts',(172.988170508833,-3.33098293707706,
124.644588419932));
#209639=CARTESIAN_POINT('Ctrl Pts',(172.709722885019,-6.98286844495469,
130.277303567246));
#209640=CARTESIAN_POINT('Ctrl Pts',(172.431275261207,-4.21783898400718,
136.394358395635));
#209641=CARTESIAN_POINT('Ctrl Pts',(172.152827637394,2.42317845035331,137.374478352552));
#209642=CARTESIAN_POINT('Ctrl Pts',(171.874380013581,6.83741326768756,132.316981079111));
#209643=CARTESIAN_POINT('Ctrl Pts',(171.595932389768,4.96839931822471,125.869459497128));
#209644=CARTESIAN_POINT('Ctrl Pts',(171.317484765955,-1.46633088488636,
123.956870961504));
#209645=CARTESIAN_POINT('Ctrl Pts',(171.039037142142,-6.55357463903296,
128.336790901335));
#209646=CARTESIAN_POINT('Ctrl Pts',(170.760589518329,-5.61840345982816,
134.984286862899));
#209647=CARTESIAN_POINT('Ctrl Pts',(170.482141894517,0.479806024690783,
137.79063480575));
#209648=CARTESIAN_POINT('Ctrl Pts',(170.203694270703,6.13709721234627,134.176938068128));
#209649=CARTESIAN_POINT('Ctrl Pts',(169.925246646891,6.15469587572206,127.464007413007));
#209650=CARTESIAN_POINT('Ctrl Pts',(169.646799023078,0.51642970291829,123.820698167548));
#209651=CARTESIAN_POINT('Ctrl Pts',(169.368351399265,-5.59641013787386,
126.595033542778));
#209652=CARTESIAN_POINT('Ctrl Pts',(169.089903775452,-6.56642246179436,
133.237534862678));
#209653=CARTESIAN_POINT('Ctrl Pts',(168.811456151639,-1.50221333089678,
137.644067918489));
#209654=CARTESIAN_POINT('Ctrl Pts',(168.533008527826,4.94245646389391,135.76524410303));
#209655=CARTESIAN_POINT('Ctrl Pts',(168.254560904013,6.84525022078748,129.32761071706));
#209656=CARTESIAN_POINT('Ctrl Pts',(167.976113280201,2.45759343384159,124.247038346411));
#209657=CARTESIAN_POINT('Ctrl Pts',(167.697665656387,-4.1884716586909,125.192324799951));
#209658=CARTESIAN_POINT('Ctrl Pts',(167.419218032575,-6.98553591510243,
131.294798006688));
#209659=CARTESIAN_POINT('Ctrl Pts',(167.140770408762,-3.36323392793624,
136.946583212019));
#209660=CARTESIAN_POINT('Ctrl Pts',(166.862322784949,3.34971573589186,136.953965917302));
#209661=CARTESIAN_POINT('Ctrl Pts',(166.583875161136,6.98444028114645,131.310161777048));
#209662=CARTESIAN_POINT('Ctrl Pts',(166.305427537323,4.20080541690416,125.20155108099));
#209663=CARTESIAN_POINT('Ctrl Pts',(166.02697991351,-2.44316440471955,124.241648636582));
#209664=CARTESIAN_POINT('Ctrl Pts',(165.748532289697,-6.84198549362249,
129.312557896394));
#209665=CARTESIAN_POINT('Ctrl Pts',(165.470084665885,-4.95335616345982,
135.754360978348));
#209666=CARTESIAN_POINT('Ctrl Pts',(165.191637042072,1.48716549602113,137.647355549705));
#209667=CARTESIAN_POINT('Ctrl Pts',(164.913189418259,6.56105471673207,133.251972077313));
#209668=CARTESIAN_POINT('Ctrl Pts',(164.634741794446,5.60565517810829,126.60735324588));
#209669=CARTESIAN_POINT('Ctrl Pts',(164.356294170633,-0.501067617717217,
123.819579153818));
#209670=CARTESIAN_POINT('Ctrl Pts',(164.07784654682,-6.1473337513746,127.450478001396));
#209671=CARTESIAN_POINT('Ctrl Pts',(163.799398923007,-6.14450048146789,
134.163431126959));
#209672=CARTESIAN_POINT('Ctrl Pts',(163.520951299194,-0.495171444628521,
137.789562554107));
#209673=CARTESIAN_POINT('Ctrl Pts',(163.242503675381,5.60919595935461,134.996634647659));
#209674=CARTESIAN_POINT('Ctrl Pts',(162.964056051569,6.55898630114736,128.351211711527));
#209675=CARTESIAN_POINT('Ctrl Pts',(162.685608427755,1.48138865648,123.960112777059));
#209676=CARTESIAN_POINT('Ctrl Pts',(162.407160803943,-4.95753279363329,
125.85854324792));
#209677=CARTESIAN_POINT('Ctrl Pts',(162.12871318013,-6.84072379533872,132.301938264875));
#209678=CARTESIAN_POINT('Ctrl Pts',(161.850265556317,-2.4376238170639,137.369132584688));
#209679=CARTESIAN_POINT('Ctrl Pts',(161.571817932504,4.20553336454888,136.403622173655));
#209680=CARTESIAN_POINT('Ctrl Pts',(161.293370308691,6.98401083586784,130.292663931709));
#209681=CARTESIAN_POINT('Ctrl Pts',(161.014922684878,3.34452353692138,124.651929946293));
#209682=CARTESIAN_POINT('Ctrl Pts',(160.736475061065,-3.36841750339773,
124.664979184829));
#209683=CARTESIAN_POINT('Ctrl Pts',(160.458027437253,-6.98594741443756,
130.319820034592));
#209684=CARTESIAN_POINT('Ctrl Pts',(160.179579813439,-4.18373293411359,
136.419930008985));
#209685=CARTESIAN_POINT('Ctrl Pts',(159.901132189627,2.46312772594441,137.35960604848));
#209686=CARTESIAN_POINT('Ctrl Pts',(159.622684565814,6.84649433633851,132.275331778507));
#209687=CARTESIAN_POINT('Ctrl Pts',(159.344236942001,4.93826712148011,125.839306872565));
#209688=CARTESIAN_POINT('Ctrl Pts',(159.065789318188,-1.50798633025781,
123.965923801919));
#209689=CARTESIAN_POINT('Ctrl Pts',(158.787341694375,-6.56847401371661,
128.376730088641));
#209690=CARTESIAN_POINT('Ctrl Pts',(158.508894070562,-5.59285496636459,
135.018410235101));
#209691=CARTESIAN_POINT('Ctrl Pts',(158.230446446749,0.522324568921774,
137.787584650814));
#209692=CARTESIAN_POINT('Ctrl Pts',(157.951998822937,6.15751334234277,134.139517329431));
#209693=CARTESIAN_POINT('Ctrl Pts',(157.673551199123,6.13424816540071,127.426603921307));
#209694=CARTESIAN_POINT('Ctrl Pts',(157.395103575311,0.473908599138188,
123.817683904457));
#209695=CARTESIAN_POINT('Ctrl Pts',(157.116655951498,-5.62192981801017,
126.62917846882));
#209696=CARTESIAN_POINT('Ctrl Pts',(156.838208327685,-6.55148937894732,
133.277461458893));
#209697=CARTESIAN_POINT('Ctrl Pts',(156.559760703872,-1.46055025868114,
137.653085593479));
#209698=CARTESIAN_POINT('Ctrl Pts',(156.281313080059,4.97256319746619,135.735066054016));
#209699=CARTESIAN_POINT('Ctrl Pts',(156.002865456246,6.83613399835919,129.285969096806));
#209700=CARTESIAN_POINT('Ctrl Pts',(155.724417832433,2.4176316184721,124.232199769625));
#209701=CARTESIAN_POINT('Ctrl Pts',(155.44597020862,-4.2225561109203,125.217925193794));
#209702=CARTESIAN_POINT('Ctrl Pts',(155.167522584808,-6.98242105771092,
131.337311859867));
#209703=CARTESIAN_POINT('Ctrl Pts',(154.889074960995,-3.3257821626974,136.96694237038));
#209704=CARTESIAN_POINT('Ctrl Pts',(154.610627337182,3.38708806634394,136.933461308912));
#209705=CARTESIAN_POINT('Ctrl Pts',(154.332179713369,6.98738983086623,131.267636135312));
#209706=CARTESIAN_POINT('Ctrl Pts',(154.053732089556,4.1666216937926,125.17608339317));
#209707=CARTESIAN_POINT('Ctrl Pts',(153.775284465743,-2.48306822909056,
124.256642463619));
#209708=CARTESIAN_POINT('Ctrl Pts',(153.49683684193,-6.85093975406627,129.354234643731));
#209709=CARTESIAN_POINT('Ctrl Pts',(153.218389218117,-4.92313233206838,
135.784421751204));
#209710=CARTESIAN_POINT('Ctrl Pts',(152.939941594304,1.52879319471521,137.638175966376));
#209711=CARTESIAN_POINT('Ctrl Pts',(152.661493970491,6.57583246125511,133.21198772643));
#209712=CARTESIAN_POINT('Ctrl Pts',(152.383046346679,5.58000294317656,126.573307792561));
#209713=CARTESIAN_POINT('Ctrl Pts',(152.104598722866,-0.543576681382813,
123.822758706449));
#209714=CARTESIAN_POINT('Ctrl Pts',(151.826151099053,-6.16763589094857,
127.487960706439));
#209715=CARTESIAN_POINT('Ctrl Pts',(151.54770347524,-6.12393902249645,134.200772209611));
#209716=CARTESIAN_POINT('Ctrl Pts',(151.269255851427,-0.452641363423277,
137.792447383624));
#209717=CARTESIAN_POINT('Ctrl Pts',(150.990808227614,5.63461159587598,134.962412206646));
#209718=CARTESIAN_POINT('Ctrl Pts',(150.712360603801,6.54393176464461,128.311330751416));
#209719=CARTESIAN_POINT('Ctrl Pts',(150.433912979988,1.4396983305442,123.951221951899));
#209720=CARTESIAN_POINT('Ctrl Pts',(150.155465356176,-4.98754753615285,
125.888812791691));
#209721=CARTESIAN_POINT('Ctrl Pts',(149.877017732362,-6.83148087236823,
132.343551945603));
#209722=CARTESIAN_POINT('Ctrl Pts',(149.59857010855,-2.39761702327129,137.383849462723));
#209723=CARTESIAN_POINT('Ctrl Pts',(149.320122484737,4.23953974010866,136.377918157044));
#209724=CARTESIAN_POINT('Ctrl Pts',(149.041674860924,6.98076659535922,130.250159756006));
#209725=CARTESIAN_POINT('Ctrl Pts',(148.763227237111,3.30700997888175,124.631684872525));
#209726=CARTESIAN_POINT('Ctrl Pts',(148.484779613298,-3.40572725176907,
124.685597446761));
#209727=CARTESIAN_POINT('Ctrl Pts',(148.206331989485,-6.98876751706998,
130.362354456768));
#209728=CARTESIAN_POINT('Ctrl Pts',(147.927884365672,-4.14947185445744,
136.445293535346));
#209729=CARTESIAN_POINT('Ctrl Pts',(147.649436741859,2.50298572943186,137.344490837378));
#209730=CARTESIAN_POINT('Ctrl Pts',(147.370989118047,6.85532170562399,132.233627970525));
#209731=CARTESIAN_POINT('Ctrl Pts',(147.092541494233,4.90795193543132,125.809338229895));
#209732=CARTESIAN_POINT('Ctrl Pts',(146.814093870421,-1.54958589664124,
123.975230043125));
#209733=CARTESIAN_POINT('Ctrl Pts',(146.535646246608,-6.58312999118006,
128.41675923269));
#209734=CARTESIAN_POINT('Ctrl Pts',(146.257198622795,-5.56709922760349,
135.052377454143));
#209735=CARTESIAN_POINT('Ctrl Pts',(145.978750998982,0.564823758223794,
137.784275729942));
#209736=CARTESIAN_POINT('Ctrl Pts',(145.700303375169,6.17770130341801,134.101973005276));
#209737=CARTESIAN_POINT('Ctrl Pts',(145.421855751356,6.11357314825767,127.389325593625));
#209738=CARTESIAN_POINT('Ctrl Pts',(145.143408127543,0.431369934500661,
123.81492853524));
#209739=CARTESIAN_POINT('Ctrl Pts',(144.864960503731,-5.64724117546963,
126.663478107772));
#209740=CARTESIAN_POINT('Ctrl Pts',(144.586512879918,-6.53631352825206,
133.317296413447));
#209741=CARTESIAN_POINT('Ctrl Pts',(144.308065256105,-1.41883306523854,
137.661849486446));
#209742=CARTESIAN_POINT('Ctrl Pts',(144.029617632292,5.00248567088053,135.704705295899));
#209743=CARTESIAN_POINT('Ctrl Pts',(143.751170008479,6.82676446047164,129.244383741109));
#209744=CARTESIAN_POINT('Ctrl Pts',(143.472722384666,2.37758021687388,124.217604726676));
#209745=CARTESIAN_POINT('Ctrl Pts',(143.194274760853,-4.25648409478009,
125.243732595056));
#209746=CARTESIAN_POINT('Ctrl Pts',(142.91582713704,-6.97904746413934,131.379805964341));
#209747=CARTESIAN_POINT('Ctrl Pts',(142.637379513228,-3.28820715937746,
136.987073172008));
#209748=CARTESIAN_POINT('Ctrl Pts',(142.358931889414,3.42433488700229,136.912729584442));
#209749=CARTESIAN_POINT('Ctrl Pts',(142.080484265602,6.99008046028611,131.225093326731));
#209750=CARTESIAN_POINT('Ctrl Pts',(141.802036641788,4.13228357498186,125.150824263232));
#209751=CARTESIAN_POINT('Ctrl Pts',(141.523589017976,-2.52288004245522,
124.271878918761));
#209752=CARTESIAN_POINT('Ctrl Pts',(141.245141394163,-6.859640150418,129.395965126019));
#209753=CARTESIAN_POINT('Ctrl Pts',(140.96669377035,-4.89272607219785,135.814297986063));
#209754=CARTESIAN_POINT('Ctrl Pts',(140.688246146537,1.57036424341533,137.628743153505));
#209755=CARTESIAN_POINT('Ctrl Pts',(140.409798522724,6.59036653588803,133.17191416004));
#209756=CARTESIAN_POINT('Ctrl Pts',(140.131350898911,5.55414393918375,126.539419122461));
#209757=CARTESIAN_POINT('Ctrl Pts',(139.852903275098,-0.586065602614643,
123.826196964908));
#209758=CARTESIAN_POINT('Ctrl Pts',(139.574455651286,-6.18770948650656,
127.525566301902));
#209759=CARTESIAN_POINT('Ctrl Pts',(139.296008027473,-6.10315063871238,
134.237987436982));
#209760=CARTESIAN_POINT('Ctrl Pts',(139.01756040366,-0.410094509425858,
137.795073267016));
#209761=CARTESIAN_POINT('Ctrl Pts',(138.739112779847,5.65981843979252,134.928035687503));
#209762=CARTESIAN_POINT('Ctrl Pts',(138.460665156034,6.52863474034383,128.271542171445));
#209763=CARTESIAN_POINT('Ctrl Pts',(138.182217532221,1.39795465605713,123.942585072312));
#209764=CARTESIAN_POINT('Ctrl Pts',(137.903769908408,-5.01737746326431,
125.919264482896));
#209765=CARTESIAN_POINT('Ctrl Pts',(137.625322284595,-6.82198480636163,
132.385108591028));
#209766=CARTESIAN_POINT('Ctrl Pts',(137.346874660782,-2.35752138489827,
137.39832253538));
#209767=CARTESIAN_POINT('Ctrl Pts',(137.06842703697,4.27338901796432,136.352007610208));
#209768=CARTESIAN_POINT('Ctrl Pts',(136.789979413157,6.9772636799772,130.20767611642));
#209769=CARTESIAN_POINT('Ctrl Pts',(136.511531789344,3.26937387837121,124.611668529527));
#209770=CARTESIAN_POINT('Ctrl Pts',(136.233084165531,-3.44291079966457,
124.706442441713));
#209771=CARTESIAN_POINT('Ctrl Pts',(135.954636541718,-6.99132864835187,
130.404905257644));
#209772=CARTESIAN_POINT('Ctrl Pts',(135.676188917905,-4.1150570145959,136.470448034864));
#209773=CARTESIAN_POINT('Ctrl Pts',(135.397741294092,2.54275098386259,137.329133279345));
#209774=CARTESIAN_POINT('Ctrl Pts',(135.11929367028,6.8638950484427,132.191871200516));
#209775=CARTESIAN_POINT('Ctrl Pts',(134.840846046466,4.87745488341857,125.779554679616));
#209776=CARTESIAN_POINT('Ctrl Pts',(134.562398422654,-1.59112804254939,
123.984789340275));
#209777=CARTESIAN_POINT('Ctrl Pts',(134.283950798841,-6.59754202834077,
128.456876850186));
#209778=CARTESIAN_POINT('Ctrl Pts',(134.005503175028,-5.54113719793324,
135.086187261361));
#209779=CARTESIAN_POINT('Ctrl Pts',(133.727055551215,0.607302017773813,
137.780708165749));
#209780=CARTESIAN_POINT('Ctrl Pts',(133.448607927402,6.19766034749954,134.064306486881));
#209781=CARTESIAN_POINT('Ctrl Pts',(133.170160303589,6.09267159041341,127.352173811322));
#209782=CARTESIAN_POINT('Ctrl Pts',(132.891712679776,0.388815285291658,
123.812432161999));
#209783=CARTESIAN_POINT('Ctrl Pts',(132.613265055963,-5.67234327233058,
126.697931188648));
#209784=CARTESIAN_POINT('Ctrl Pts',(132.334817432151,-6.52089547205522,
133.357038250242));
#209785=CARTESIAN_POINT('Ctrl Pts',(132.056369808337,-1.37706329641493,
137.670359272641));
#209786=CARTESIAN_POINT('Ctrl Pts',(131.777922184525,5.0322227753486,135.674162953708));
#209787=CARTESIAN_POINT('Ctrl Pts',(131.499474560712,6.81714195431646,129.20285619093));
#209788=CARTESIAN_POINT('Ctrl Pts',(131.221026936899,2.33744071316646,124.203253758389));
#209789=CARTESIAN_POINT('Ctrl Pts',(130.942579313086,-4.29025435305649,
125.269746047434));
#209790=CARTESIAN_POINT('Ctrl Pts',(130.664131689273,-6.97541525939744,
131.422278745477));
#209791=CARTESIAN_POINT('Ctrl Pts',(130.38568406546,-3.25051031033198,137.006974870947));
#209792=CARTESIAN_POINT('Ctrl Pts',(130.107236441647,3.46145481767177,136.891771512113));
#209793=CARTESIAN_POINT('Ctrl Pts',(129.828788817834,6.99251206970404,131.182534927744));
#209794=CARTESIAN_POINT('Ctrl Pts',(129.550341194022,4.09779233288376,125.125774627163));
#209795=CARTESIAN_POINT('Ctrl Pts',(129.271893570209,-2.5625983695722,124.287357437414));
#209796=CARTESIAN_POINT('Ctrl Pts',(128.993445946396,-6.86808636028122,
129.43774779692));
#209797=CARTESIAN_POINT('Ctrl Pts',(128.714998322583,-4.86213851056362,
135.84398857585));
#209798=CARTESIAN_POINT('Ctrl Pts',(128.43655069877,1.61187710169066,137.61905746063));
#209799=CARTESIAN_POINT('Ctrl Pts',(128.158103074957,6.60465640206541,133.131752863082));
#209800=CARTESIAN_POINT('Ctrl Pts',(127.879655451144,5.52807912434469,126.505688491336));
#209801=CARTESIAN_POINT('Ctrl Pts',(127.601207827331,-0.628532806970051,
123.829893801787));
#209802=CARTESIAN_POINT('Ctrl Pts',(127.322760203518,-6.20755379421381,
127.563293394292));
#209803=CARTESIAN_POINT('Ctrl Pts',(127.044312579706,-6.08213610043705,
134.275075430049));
#209804=CARTESIAN_POINT('Ctrl Pts',(126.765864955893,-0.367532459225645,
137.797440106979));
#209805=CARTESIAN_POINT('Ctrl Pts',(126.48741733208,5.68481555705546,134.893506364063));
#209806=CARTESIAN_POINT('Ctrl Pts',(126.208969708267,6.51309579508176,128.231847445991));
#209807=CARTESIAN_POINT('Ctrl Pts',(125.930522084454,1.35615917984635,123.934202458341));
#209808=CARTESIAN_POINT('Ctrl Pts',(125.652074460641,-5.04702146960864,
125.949897193134));
#209809=CARTESIAN_POINT('Ctrl Pts',(125.373626836828,-6.81223594919939,
132.426606661257));
#209810=CARTESIAN_POINT('Ctrl Pts',(125.095179213015,-2.3173383877032,137.412551266352));
#209811=CARTESIAN_POINT('Ctrl Pts',(124.816731589202,4.3070799438184,136.325891493273));
#209812=CARTESIAN_POINT('Ctrl Pts',(124.538283965389,6.97350221952356,130.165214587198));
#209813=CARTESIAN_POINT('Ctrl Pts',(124.259836341577,3.2316166300094,124.591881659011));
#209814=CARTESIAN_POINT('Ctrl Pts',(123.981388717764,-3.47996676923432,
124.727513397266));
#209815=CARTESIAN_POINT('Ctrl Pts',(123.702941093951,-6.99363071337966,
130.447470860486));
#209816=CARTESIAN_POINT('Ctrl Pts',(123.424493470138,-4.08048968978323,
136.495392575427));
#209817=CARTESIAN_POINT('Ctrl Pts',(123.146045846325,2.58242201572056,137.313533943462));
#209818=CARTESIAN_POINT('Ctrl Pts',(122.867598222512,6.87221404710605,132.150063015792));
#209819=CARTESIAN_POINT('Ctrl Pts',(122.589150598699,4.84677709552158,125.749957325369));
#209820=CARTESIAN_POINT('Ctrl Pts',(122.310702974886,-1.63261122862275,
123.994601339147));
#209821=CARTESIAN_POINT('Ctrl Pts',(122.032255351073,-6.6117095911554,128.497081454556));
#209822=CARTESIAN_POINT('Ctrl Pts',(121.753807727261,-5.51496983938628,
135.119838403918));
#209823=CARTESIAN_POINT('Ctrl Pts',(121.475360103447,0.649757773524084,
137.776882090432));
#209824=CARTESIAN_POINT('Ctrl Pts',(121.196912479635,6.21738973499768,134.026519169992));
#209825=CARTESIAN_POINT('Ctrl Pts',(120.918464855822,6.07154426638285,127.315149951069));
#209826=CARTESIAN_POINT('Ctrl Pts',(120.640017232009,0.346246228389124,
123.810194877238));
#209827=CARTESIAN_POINT('Ctrl Pts',(120.361569608196,-5.69723517842559,
126.732536434776));
#209828=CARTESIAN_POINT('Ctrl Pts',(120.083121984383,-6.50523578167861,
133.396685496627));
#209829=CARTESIAN_POINT('Ctrl Pts',(119.80467436057,-1.3352425000044,137.678614636731));
#209830=CARTESIAN_POINT('Ctrl Pts',(119.526226736757,5.06177340895125,135.6434401592));
#209831=CARTESIAN_POINT('Ctrl Pts',(119.247779112945,6.8072668364591,129.161387985085));
#209832=CARTESIAN_POINT('Ctrl Pts',(118.969331489131,2.29721459473369,124.189147396544));
#209833=CARTESIAN_POINT('Ctrl Pts',(118.690883865319,-4.32386563438011,
125.29596458699));
#209834=CARTESIAN_POINT('Ctrl Pts',(118.412436241506,-6.97152457807781,
131.464728629428));
#209835=CARTESIAN_POINT('Ctrl Pts',(118.133988617693,-3.21269301243169,
137.026646729736));
#209836=CARTESIAN_POINT('Ctrl Pts',(117.85554099388,3.49844648286018,136.870587868534));
#209837=CARTESIAN_POINT('Ctrl Pts',(117.577093370067,6.99468456901571,131.139962515369));
#209838=CARTESIAN_POINT('Ctrl Pts',(117.298645746254,4.06314924558364,125.100935413187));
#209839=CARTESIAN_POINT('Ctrl Pts',(117.020198122441,-2.60222173866402,
124.303077446017));
#209840=CARTESIAN_POINT('Ctrl Pts',(116.741750498628,-6.8762780706787,129.479581108162));
#209841=CARTESIAN_POINT('Ctrl Pts',(116.463302874816,-4.83137078059878,
135.873492420371));
#209842=CARTESIAN_POINT('Ctrl Pts',(116.184855251003,1.65333023126747,137.609119246659));
#209843=CARTESIAN_POINT('Ctrl Pts',(115.90640762719,6.61870153027093,133.09150532375));
#209844=CARTESIAN_POINT('Ctrl Pts',(115.627960003377,5.5018094645007,126.472117149089));
#209845=CARTESIAN_POINT('Ctrl Pts',(115.349512379564,-0.670976720811003,
123.833849080098));
#209846=CARTESIAN_POINT('Ctrl Pts',(115.071064755751,-6.22716807873245,
127.601140585621));
#209847=CARTESIAN_POINT('Ctrl Pts',(114.792617131938,-6.06089618637186,
134.312034814502));
#209848=CARTESIAN_POINT('Ctrl Pts',(114.514169508125,-0.324956789974863,
137.79954781581));
#209849=CARTESIAN_POINT('Ctrl Pts',(114.235721884312,5.70960202138734,134.858825515823));
#209850=CARTESIAN_POINT('Ctrl Pts',(113.957274260499,6.4973155046598,128.192248045959));
#209851=CARTESIAN_POINT('Ctrl Pts',(113.678826636687,1.31431345065849,123.926074420608));
#209852=CARTESIAN_POINT('Ctrl Pts',(113.400379012874,-5.07647845671644,
125.980709787299));
#209853=CARTESIAN_POINT('Ctrl Pts',(113.121931389061,-6.80223466212876,
132.468044618562));
#209854=CARTESIAN_POINT('Ctrl Pts',(112.843483765248,-2.27706952068197,
137.42653512839));
#209855=CARTESIAN_POINT('Ctrl Pts',(112.565036141435,4.34061126924124,136.299570773982));
#209856=CARTESIAN_POINT('Ctrl Pts',(112.286588517622,6.96948235338073,130.122776741767));
#209857=CARTESIAN_POINT('Ctrl Pts',(112.008140893809,3.1937396329048,124.572324994188));
#209858=CARTESIAN_POINT('Ctrl Pts',(111.729693269996,-3.51689378735575,
124.748809532627));
#209859=CARTESIAN_POINT('Ctrl Pts',(111.451245646184,-6.99567362684944,
130.490049688009));
#209860=CARTESIAN_POINT('Ctrl Pts',(111.172798022371,-4.0457711609245,136.52012623271));
#209861=CARTESIAN_POINT('Ctrl Pts',(110.894350398558,2.62199735498092,137.297693407768));
#209862=CARTESIAN_POINT('Ctrl Pts',(110.615902774745,6.88027839335069,132.108204965571));
#209863=CARTESIAN_POINT('Ctrl Pts',(110.337455150932,4.81591970851693,125.720547263895));
#209864=CARTESIAN_POINT('Ctrl Pts',(110.059007527119,-1.67403391768677,
124.004665676154));
#209865=CARTESIAN_POINT('Ctrl Pts',(109.780559903306,-6.62563215463966,
128.537371556004));
#209866=CARTESIAN_POINT('Ctrl Pts',(109.502112279493,-5.48859812160383,
135.153329634858));
#209867=CARTESIAN_POINT('Ctrl Pts',(109.22366465568,0.692189452261082,137.772797645767));
#209868=CARTESIAN_POINT('Ctrl Pts',(108.945217031867,6.23688873483282,133.988612454835));
#209869=CARTESIAN_POINT('Ctrl Pts',(108.666769408055,6.05019195904657,127.278255384801));
#209870=CARTESIAN_POINT('Ctrl Pts',(108.388321784241,0.303664341205276,
123.808216763862));
#209871=CARTESIAN_POINT('Ctrl Pts',(108.109874160429,-5.72191597137591,
126.767292563848));
#209872=CARTESIAN_POINT('Ctrl Pts',(107.831426536616,-6.48933503739778,
133.436236683461));
#209873=CARTESIAN_POINT('Ctrl Pts',(107.552978912803,-1.29337222569216,
137.68661527281));
#209874=CARTESIAN_POINT('Ctrl Pts',(107.27453128899,5.09113647667873,135.612538050821));
#209875=CARTESIAN_POINT('Ctrl Pts',(106.996083665177,6.79713947282576,129.119980660195));
#209876=CARTESIAN_POINT('Ctrl Pts',(106.717636041364,2.25690335216928,124.175286163858));
#209877=CARTESIAN_POINT('Ctrl Pts',(106.439188417551,-4.35731669327239,
125.322387242187));
#209878=CARTESIAN_POINT('Ctrl Pts',(106.160740793739,-6.96737556435125,
131.5071540432));
#209879=CARTESIAN_POINT('Ctrl Pts',(105.882293169926,-3.17475666701035,
137.046088019424));
#209880=CARTESIAN_POINT('Ctrl Pts',(105.603845546113,3.53530851182771,136.849179438675));
#209881=CARTESIAN_POINT('Ctrl Pts',(105.3253979223,6.99659787771835,131.097377667143));
#209882=CARTESIAN_POINT('Ctrl Pts',(105.046950298487,4.02835559679407,125.076307541727));
#209883=CARTESIAN_POINT('Ctrl Pts',(104.768502674674,-2.64174868147234,
124.319038362058));
#209884=CARTESIAN_POINT('Ctrl Pts',(104.490055050861,-6.88421497806359,
129.521463509594));
#209885=CARTESIAN_POINT('Ctrl Pts',(104.211607427049,-4.80042402241278,
135.902808426348));
#209886=CARTESIAN_POINT('Ctrl Pts',(103.933159803235,1.69472209608453,137.598928879852));
#209887=CARTESIAN_POINT('Ctrl Pts',(103.654712179423,6.63250140005722,133.051173033428));
#209888=CARTESIAN_POINT('Ctrl Pts',(103.37626455561,5.47533593308374,126.438706339714));
#209889=CARTESIAN_POINT('Ctrl Pts',(103.097816931797,-0.713395771362793,
123.838062653278));
#209890=CARTESIAN_POINT('Ctrl Pts',(102.819369307984,-6.24655161324796,
127.639106473447));
#209891=CARTESIAN_POINT('Ctrl Pts',(102.540921684171,-6.03943168356949,
134.348864220799));
#209892=CARTESIAN_POINT('Ctrl Pts',(102.262474060358,-0.282369079330704,
137.801396315408));
#209893=CARTESIAN_POINT('Ctrl Pts',(101.984026436545,5.73417691431645,134.823994427897));
#209894=CARTESIAN_POINT('Ctrl Pts',(101.705578812732,6.48129445382252,128.15274543872));
#209895=CARTESIAN_POINT('Ctrl Pts',(101.427131188919,1.27241901910234,123.9182012603));
#209896=CARTESIAN_POINT('Ctrl Pts',(101.148683565106,-5.1057473330482,126.01170112362));
#209897=CARTESIAN_POINT('Ctrl Pts',(100.870235941294,-6.7919813157512,132.509420927444));
#209898=CARTESIAN_POINT('Ctrl Pts',(100.591788317481,-2.23671627601227,
137.440273603317));
#209899=CARTESIAN_POINT('Ctrl Pts',(100.313340693668,4.37398175171709,136.273046427655));
#209900=CARTESIAN_POINT('Ctrl Pts',(100.034893069855,6.96520423050629,130.080364152676));
#209901=CARTESIAN_POINT('Ctrl Pts',(99.7564454460421,3.15574429060373,124.552999259737));
#209902=CARTESIAN_POINT('Ctrl Pts',(99.4779978222292,-3.55369048568456,
124.770330058661));
#209903=CARTESIAN_POINT('Ctrl Pts',(99.1995501984162,-6.99745731306031,
130.532640162439));
#209904=CARTESIAN_POINT('Ctrl Pts',(98.9211025746034,-4.01090271452764,
136.544648090195));
#209905=CARTESIAN_POINT('Ctrl Pts',(98.6426549507905,2.66147553516503,137.281612259238));
#209906=CARTESIAN_POINT('Ctrl Pts',(98.3642073269776,6.88808778834931,132.066298600918));
#209907=CARTESIAN_POINT('Ctrl Pts',(98.0857597031646,4.78488386583629,125.691325584995));
#209908=CARTESIAN_POINT('Ctrl Pts',(97.8073120793519,-1.71539457480834,
124.014981978356));
#209909=CARTESIAN_POINT('Ctrl Pts',(97.5288644555388,-6.63930920288774,
128.577745661565));
#209910=CARTESIAN_POINT('Ctrl Pts',(97.2504168317261,-5.46202302179963,
135.186659713151));
#209911=CARTESIAN_POINT('Ctrl Pts',(96.9719692079131,0.734595481663425,
137.768454983106));
#209912=CARTESIAN_POINT('Ctrl Pts',(96.6935215841003,6.25615662446226,133.950587746053));
#209913=CARTESIAN_POINT('Ctrl Pts',(96.4150739602873,6.0286154596223,127.24149147966));
#209914=CARTESIAN_POINT('Ctrl Pts',(96.1366263364746,0.26107120162757,123.806497895168));
#209915=CARTESIAN_POINT('Ctrl Pts',(95.8581787126614,-5.74638473662552,
126.80219828796));
#209916=CARTESIAN_POINT('Ctrl Pts',(95.5797310888487,-6.47319382842077,
133.47569034516));
#209917=CARTESIAN_POINT('Ctrl Pts',(95.3012834650358,-1.25145402499642,
137.694360884412));
#209918=CARTESIAN_POINT('Ctrl Pts',(95.0228358412229,5.12031089047184,135.581457773658));
#209919=CARTESIAN_POINT('Ctrl Pts',(94.7443882174101,6.78676023868958,129.078635750625));
#209920=CARTESIAN_POINT('Ctrl Pts',(94.465940593597,2.21650847922131,124.161670573963));
#209921=CARTESIAN_POINT('Ctrl Pts',(94.1874929697842,-4.39060629019222,
125.349013033923));
#209922=CARTESIAN_POINT('Ctrl Pts',(93.9090453459715,-6.96296837196094,
131.549553414704));
#209923=CARTESIAN_POINT('Ctrl Pts',(93.6305977221583,-3.13670267981308,
137.065298019608));
#209924=CARTESIAN_POINT('Ctrl Pts',(93.3521500983456,3.5720395386382,136.82754701583));
#209925=CARTESIAN_POINT('Ctrl Pts',(93.0737024745325,6.99825192491364,131.054781961061));
#209926=CARTESIAN_POINT('Ctrl Pts',(92.7952548507199,3.99341267580637,125.051891925383));
#209927=CARTESIAN_POINT('Ctrl Pts',(92.5168072269068,-2.68117773331193,
124.335239594101));
#209928=CARTESIAN_POINT('Ctrl Pts',(92.238359603094,-6.89189678833074,129.563393449252));
#209929=CARTESIAN_POINT('Ctrl Pts',(91.959911979281,-4.7692993827493,135.931935507467));
#209930=CARTESIAN_POINT('Ctrl Pts',(91.6814643554683,1.73605116235111,137.588486737821));
#209931=CARTESIAN_POINT('Ctrl Pts',(91.4030167316553,6.6460555000649,133.010757486647));
#209932=CARTESIAN_POINT('Ctrl Pts',(91.1245691078424,5.44865951108031,126.405457301267));
#209933=CARTESIAN_POINT('Ctrl Pts',(90.8461214840295,-0.755788386771977,
123.84253436519));
#209934=CARTESIAN_POINT('Ctrl Pts',(90.5676738602166,-6.26570367949625,
127.677189650927));
#209935=CARTESIAN_POINT('Ctrl Pts',(90.2892262364038,-6.01774338740505,
134.38556228421));
#209936=CARTESIAN_POINT('Ctrl Pts',(90.0107786125907,-0.239770905396614,
137.802985537273));
#209937=CARTESIAN_POINT('Ctrl Pts',(89.7323309887781,5.75853932521132,134.78901439096));
#209938=CARTESIAN_POINT('Ctrl Pts',(89.453883364965,6.46503323623579,128.113341088056));
#209939=CARTESIAN_POINT('Ctrl Pts',(89.1754357411521,1.23047743759138,123.910583269158));
#209940=CARTESIAN_POINT('Ctrl Pts',(88.8969881173393,-5.13482701403487,
126.042870053701));
#209941=CARTESIAN_POINT('Ctrl Pts',(88.6185404935264,-6.78147629000823,
132.550734054689));
#209942=CARTESIAN_POINT('Ctrl Pts',(88.3400928697134,-2.19628014899849,
137.453766182047));
#209943=CARTESIAN_POINT('Ctrl Pts',(88.0616452459006,4.4071901546906,136.246319437167));
#209944=CARTESIAN_POINT('Ctrl Pts',(87.7831976220877,6.96066800942769,130.037978391542));
#209945=CARTESIAN_POINT('Ctrl Pts',(87.5047499982748,3.1176320110373,124.533905171779));
#209946=CARTESIAN_POINT('Ctrl Pts',(87.2263023744621,-3.59035550070555,
124.792074177916));
#209947=CARTESIAN_POINT('Ctrl Pts',(86.9478547506488,-6.99898170591706,
130.57524070557));
#209948=CARTESIAN_POINT('Ctrl Pts',(86.6694071268362,-3.97588564265574,
136.568957239218));
#209949=CARTESIAN_POINT('Ctrl Pts',(86.3909595030232,2.70085509339449,137.265291093768));
#209950=CARTESIAN_POINT('Ctrl Pts',(86.1125118792103,6.89564194272181,132.024345474689));
#209951=CARTESIAN_POINT('Ctrl Pts',(85.8340642553976,4.75367071752436,125.662293371487));
#209952=CARTESIAN_POINT('Ctrl Pts',(85.5556166315845,-1.75669166735309,
124.025549863481));
#209953=CARTESIAN_POINT('Ctrl Pts',(85.2771690077717,-6.65274022909182,
128.618202275162));
#209954=CARTESIAN_POINT('Ctrl Pts',(84.9987213839588,-5.4352455247236,135.21982740374));
#209955=CARTESIAN_POINT('Ctrl Pts',(84.7202737601459,0.776974290360158,
137.763854263368));
#209956=CARTESIAN_POINT('Ctrl Pts',(84.4418261363329,6.27519268990729,133.912446452669));
#209957=CARTESIAN_POINT('Ctrl Pts',(84.1633785125202,6.00681556763514,127.204859597945));
#209958=CARTESIAN_POINT('Ctrl Pts',(83.8849308887072,0.218468387960617,
123.805038334852));
#209959=CARTESIAN_POINT('Ctrl Pts',(83.6064832648944,-5.77064056747553,
126.837252313669));
#209960=CARTESIAN_POINT('Ctrl Pts',(83.3280356410814,-6.45681275286598,
133.515045019753));
#209961=CARTESIAN_POINT('Ctrl Pts',(83.0495880172686,-1.20948945121144,
137.701851184522));
#209962=CARTESIAN_POINT('Ctrl Pts',(82.7711403934555,5.14929556926191,135.550200479404));
#209963=CARTESIAN_POINT('Ctrl Pts',(82.4926927696429,6.77612951865689,129.037354788424));
#209964=CARTESIAN_POINT('Ctrl Pts',(82.2142451458298,2.17603147273656,124.148301131391));
#209965=CARTESIAN_POINT('Ctrl Pts',(81.9357975220171,-4.42373319158141,
125.375840975569));
#209966=CARTESIAN_POINT('Ctrl Pts',(81.6573498982041,-6.95830316421689,
131.591925172815));
#209967=CARTESIAN_POINT('Ctrl Pts',(81.3789022743912,-3.09853246094448,
137.084276018453));
#209968=CARTESIAN_POINT('Ctrl Pts',(81.1004546505783,3.60863820220999,136.805691401599));
#209969=CARTESIAN_POINT('Ctrl Pts',(80.8220070267654,6.99964664931016,131.012176975526));
#209970=CARTESIAN_POINT('Ctrl Pts',(80.5435594029525,3.95832177744353,125.02768946888));
#209971=CARTESIAN_POINT('Ctrl Pts',(80.2651117791397,-2.72050743312451,
124.351680541802));
#209972=CARTESIAN_POINT('Ctrl Pts',(79.9866641553267,-6.89932321682792,
129.605369373404));
#209973=CARTESIAN_POINT('Ctrl Pts',(79.7082165315139,-4.73799801494326,
135.960872584412));
#209974=CARTESIAN_POINT('Ctrl Pts',(79.4297689077009,1.77731589860328,137.577793207502));
#209975=CARTESIAN_POINT('Ctrl Pts',(79.1513212838881,6.65936332804202,132.970260181018));
#209976=CARTESIAN_POINT('Ctrl Pts',(78.8728736600752,5.42178118699497,126.372371265798));
#209977=CARTESIAN_POINT('Ctrl Pts',(78.5944260362623,-0.798152996164653,
123.847264050135));
#209978=CARTESIAN_POINT('Ctrl Pts',(78.3159784124494,-6.28462356779051,
127.715388706879));
#209979=CARTESIAN_POINT('Ctrl Pts',(78.0375307886365,-5.99583210154638,
134.422127644877));
#209980=CARTESIAN_POINT('Ctrl Pts',(77.7590831648237,-0.197163846663491,
137.804315422519));
#209981=CARTESIAN_POINT('Ctrl Pts',(77.4806355410107,5.78268835131386,134.753886701214));
#209982=CARTESIAN_POINT('Ctrl Pts',(77.2021879171979,6.44853245446487,128.07403645411));
#209983=CARTESIAN_POINT('Ctrl Pts',(76.9237402933849,1.18849026028645,123.903220729472));
#209984=CARTESIAN_POINT('Ctrl Pts',(76.6452926695721,-5.16371642211823,
126.074215422566));
#209985=CARTESIAN_POINT('Ctrl Pts',(76.3668450457591,-6.77071997416741,
132.591982469425));
#209986=CARTESIAN_POINT('Ctrl Pts',(76.0883974219463,-2.15576263801617,
137.467012364608));
#209987=CARTESIAN_POINT('Ctrl Pts',(75.8099497981334,4.44023524761227,136.219390792892));
#209988=CARTESIAN_POINT('Ctrl Pts',(75.5315021743204,6.95587385823614,129.995621028982));
#209989=CARTESIAN_POINT('Ctrl Pts',(75.2530545505077,3.0794042064702,124.515043437855));
#209990=CARTESIAN_POINT('Ctrl Pts',(74.9746069266946,-3.62688747378295,
124.814041084656));
#209991=CARTESIAN_POINT('Ctrl Pts',(74.6961593028819,-7.0002467489329,130.617849738824));
#209992=CARTESIAN_POINT('Ctrl Pts',(74.4177116790688,-3.94072124287924,
136.593052778991));
#209993=CARTESIAN_POINT('Ctrl Pts',(74.1392640552561,2.74013457044532,137.248730516143));
#209994=CARTESIAN_POINT('Ctrl Pts',(73.860816431443,6.90294057654623,131.982347141473));
#209995=CARTESIAN_POINT('Ctrl Pts',(73.5823688076304,4.72228142019582,125.633451699173));
#209996=CARTESIAN_POINT('Ctrl Pts',(73.3039211838172,-1.79792366504193,
124.036368939932));
#209997=CARTESIAN_POINT('Ctrl Pts',(73.0254735600045,-6.66592473556012,
128.658739897661));
#209998=CARTESIAN_POINT('Ctrl Pts',(72.7470259361915,-5.40826662262595,
135.252831477583));
#209999=CARTESIAN_POINT('Ctrl Pts',(72.4685783123786,0.819324307988826,
137.758995657032));
#210000=CARTESIAN_POINT('Ctrl Pts',(72.1901306885658,6.2939962257795,133.87418998802));
#210001=CARTESIAN_POINT('Ctrl Pts',(71.9116830647529,5.98479309088811,127.168361097063));
#210002=CARTESIAN_POINT('Ctrl Pts',(71.63323544094,0.17585747886725,123.803838136996));
#210003=CARTESIAN_POINT('Ctrl Pts',(71.3547878171271,-5.79468256511725,
126.872453342036));
#210004=CARTESIAN_POINT('Ctrl Pts',(71.0763401933142,-6.44019241774003,
133.554299248939));
#210005=CARTESIAN_POINT('Ctrl Pts',(70.7978925695013,-1.16748005934989,
137.709085895581));
#210006=CARTESIAN_POINT('Ctrl Pts',(70.5194449456884,5.17808943901089,135.518767326308));
#210007=CARTESIAN_POINT('Ctrl Pts',(70.2409973218756,6.76524770665308,128.996139303274));
#210008=CARTESIAN_POINT('Ctrl Pts',(69.9625496980626,2.1354738326052,124.135178331551));
#210009=CARTESIAN_POINT('Ctrl Pts',(69.6841020742497,-4.45669616991057,
125.402870073008));
#210010=CARTESIAN_POINT('Ctrl Pts',(69.4056544504369,-6.95338011399016,
131.634267747431));
#210011=CARTESIAN_POINT('Ctrl Pts',(69.1272068266238,-3.06024742481583,
137.103021312725));
#210012=CARTESIAN_POINT('Ctrl Pts',(68.8487592028112,3.64510314636624,136.783613405848));
#210013=CARTESIAN_POINT('Ctrl Pts',(68.5703115789981,7.00078199922599,130.969564289278));
#210014=CARTESIAN_POINT('Ctrl Pts',(68.2918639551854,3.92308420201135,125.003701069051));
#210015=CARTESIAN_POINT('Ctrl Pts',(68.0134163313723,-2.75973632353393,
124.368360595937));
#210016=CARTESIAN_POINT('Ctrl Pts',(67.7349687075595,-6.90649398836592,
129.647389726619));
#210017=CARTESIAN_POINT('Ctrl Pts',(67.4565210837467,-4.70652107887851,
135.98961858491));
#210018=CARTESIAN_POINT('Ctrl Pts',(67.1780734599337,1.81851477576126,137.566848685147));
#210019=CARTESIAN_POINT('Ctrl Pts',(66.8996258361208,6.67242439086218,132.929682617185));
#210020=CARTESIAN_POINT('Ctrl Pts',(66.6211782123079,5.39470195681365,126.339449459324));
#210021=CARTESIAN_POINT('Ctrl Pts',(66.3427305884951,-0.840488029704522,
123.852251532852));
#210022=CARTESIAN_POINT('Ctrl Pts',(66.0642829646821,-6.30331057704718,
127.753702225821));
#210023=CARTESIAN_POINT('Ctrl Pts',(65.7858353408693,-5.97369863792435,
134.458558947856));
#210024=CARTESIAN_POINT('Ctrl Pts',(65.5073877170563,-0.154549481951222,
137.805385921867));
#210025=CARTESIAN_POINT('Ctrl Pts',(65.2289400932435,5.80662309777304,134.718612660325));
#210026=CARTESIAN_POINT('Ctrl Pts',(64.9504924694306,6.43179271995227,128.03483299333));
#210027=CARTESIAN_POINT('Ctrl Pts',(64.6720448456177,1.14645904303803,123.896113914062));
#210028=CARTESIAN_POINT('Ctrl Pts',(64.3935972218049,-5.19241448679041,
126.1057360687));
#210029=CARTESIAN_POINT('Ctrl Pts',(64.1151495979918,-6.75971276680813,
132.633164643176));
#210030=CARTESIAN_POINT('Ctrl Pts',(63.8367019741791,-2.11516524445634,
137.480011660159));
#210031=CARTESIAN_POINT('Ctrl Pts',(63.5582543503661,4.47311580598391,136.192261492683));
#210032=CARTESIAN_POINT('Ctrl Pts',(63.2798067265533,6.95082195458075,129.953293634565));
#210033=CARTESIAN_POINT('Ctrl Pts',(63.0013591027403,3.041062293448,124.496414756892));
#210034=CARTESIAN_POINT('Ctrl Pts',(62.7229114789275,-3.66328505121137,
124.836229964889));
#210035=CARTESIAN_POINT('Ctrl Pts',(62.4444638551145,-7.00125239523119,
130.660465683307));
#210036=CARTESIAN_POINT('Ctrl Pts',(62.1660162313017,-3.90541081822766,
136.616933816649));
#210037=CARTESIAN_POINT('Ctrl Pts',(61.8875686074887,2.77931251080179,137.231931140021));
#210038=CARTESIAN_POINT('Ctrl Pts',(61.609120983676,6.909983419369,131.940305157533));
#210039=CARTESIAN_POINT('Ctrl Pts',(61.3306733598629,4.69071713699276,125.604801636791));
#210040=CARTESIAN_POINT('Ctrl Pts',(61.0522257360502,-1.83908904000824,
124.047438806804));
#210041=CARTESIAN_POINT('Ctrl Pts',(60.7737781122372,-6.67886223373588,
128.699357026925));
#210042=CARTESIAN_POINT('Ctrl Pts',(60.4953304884244,-5.38108731521968,
135.285670711703));
#210043=CARTESIAN_POINT('Ctrl Pts',(60.2168828646114,0.861643965253713,
137.753879344138));
#210044=CARTESIAN_POINT('Ctrl Pts',(59.9384352407986,6.31256653530686,133.835819769716));
#210045=CARTESIAN_POINT('Ctrl Pts',(59.6599876169856,5.96254884543232,127.131997329482));
#210046=CARTESIAN_POINT('Ctrl Pts',(59.3815399931728,0.133240053310041,
123.802897346075));
#210047=CARTESIAN_POINT('Ctrl Pts',(59.1030923693598,-5.81850983866561,
126.907800068673));
#210048=CARTESIAN_POINT('Ctrl Pts',(58.824644745547,-6.42333343891552,133.593451578138));
#210049=CARTESIAN_POINT('Ctrl Pts',(58.5461971217341,-1.12542740608588,
137.716064749505));
#210050=CARTESIAN_POINT('Ctrl Pts',(58.2677494979212,5.20669143275151,135.487159479138));
#210051=CARTESIAN_POINT('Ctrl Pts',(57.9893018741083,6.75411520590753,128.954990822428));
#210052=CARTESIAN_POINT('Ctrl Pts',(57.7108542502954,2.09483706170563,124.122302660713));
#210053=CARTESIAN_POINT('Ctrl Pts',(57.4324066264825,-4.48949400372376,
125.430099324666));
#210054=CARTESIAN_POINT('Ctrl Pts',(57.1539590026696,-6.94819940370625,
131.676579569534));
#210055=CARTESIAN_POINT('Ctrl Pts',(56.8755113788568,-3.02184899009409,
137.121533207807));
#210056=CARTESIAN_POINT('Ctrl Pts',(56.5970637550437,3.68143301988451,136.761313846687));
#210057=CARTESIAN_POINT('Ctrl Pts',(56.318616131231,7.00165793259049,130.926945481348));
#210058=CARTESIAN_POINT('Ctrl Pts',(56.040168507418,3.88770125525153,124.979927614796));
#210059=CARTESIAN_POINT('Ctrl Pts',(55.7617208836052,-2.79886295089852,
124.385279138419));
#210060=CARTESIAN_POINT('Ctrl Pts',(55.4832732597923,-6.91340883722955,
129.689452951814));
#210061=CARTESIAN_POINT('Ctrl Pts',(55.2048256359794,-4.67486974094423,
136.018172443767));
#210062=CARTESIAN_POINT('Ctrl Pts',(54.9263780121665,1.85964626718557,137.555653576309));
#210063=CARTESIAN_POINT('Ctrl Pts',(54.6479303883536,6.68523820454244,132.889026298762));
#210064=CARTESIAN_POINT('Ctrl Pts',(54.3694827645407,5.36742282396772,126.306693101776));
#210065=CARTESIAN_POINT('Ctrl Pts',(54.0910351407278,-0.882791918651148,
123.857496628527));
#210066=CARTESIAN_POINT('Ctrl Pts',(53.8125875169149,-6.32176401481248,
127.792128788032));
#210067=CARTESIAN_POINT('Ctrl Pts',(53.534139893102,-5.95134381670231,134.494854843172));
#210068=CARTESIAN_POINT('Ctrl Pts',(53.2556922692892,-0.111929390351441,
137.806196995646));
#210069=CARTESIAN_POINT('Ctrl Pts',(52.9772446454762,5.83034267767769,134.683193575387));
#210070=CARTESIAN_POINT('Ctrl Pts',(52.6987970216634,6.41481465299549,127.995732158415));
#210071=CARTESIAN_POINT('Ctrl Pts',(52.4203493978505,1.10438534332797,123.889263086274));
#210072=CARTESIAN_POINT('Ctrl Pts',(52.1419017740376,-5.22092014463445,
126.137430824095));
#210073=CARTESIAN_POINT('Ctrl Pts',(51.8634541502246,-6.74845507580631,
132.674279049921));
#210074=CARTESIAN_POINT('Ctrl Pts',(51.5850065264118,-2.07448947267055,
137.492763587005));
#210075=CARTESIAN_POINT('Ctrl Pts',(51.3065589025989,4.50583061140446,136.164932541826));
#210076=CARTESIAN_POINT('Ctrl Pts',(51.028111278786,6.94551248566166,129.910997776748));
#210077=CARTESIAN_POINT('Ctrl Pts',(50.7496636549731,3.00260769274395,124.478019819181));
#210078=CARTESIAN_POINT('Ctrl Pts',(50.4712160311602,-3.69954688426507,
124.858639996399));
#210079=CARTESIAN_POINT('Ctrl Pts',(50.1927684073473,-7.00199860754717,
130.70308695987));
#210080=CARTESIAN_POINT('Ctrl Pts',(49.9143207835345,-3.86995567714208,
136.640599467269));
#210081=CARTESIAN_POINT('Ctrl Pts',(49.6358731597215,2.81838746271124,137.214893587909));
#210082=CARTESIAN_POINT('Ctrl Pts',(49.3574255359087,6.91677021021505,131.89822108075));
#210083=CARTESIAN_POINT('Ctrl Pts',(49.0789779120958,4.65897903754105,125.576344245977));
#210084=CARTESIAN_POINT('Ctrl Pts',(48.8005302882828,-1.88018626685394,
124.058759053897));
#210085=CARTESIAN_POINT('Ctrl Pts',(48.5220826644701,-6.69155224421552,
128.740052157871));
#210086=CARTESIAN_POINT('Ctrl Pts',(48.243635040657,-5.35370860964396,135.318343889229));
#210087=CARTESIAN_POINT('Ctrl Pts',(47.9651874168443,0.903931693984841,
137.748505514272));
#210088=CARTESIAN_POINT('Ctrl Pts',(47.6867397930313,6.33090293035988,133.797337219578));
#210089=CARTESIAN_POINT('Ctrl Pts',(47.4082921692184,5.94008365553619,127.095769642671));
#210090=CARTESIAN_POINT('Ctrl Pts',(47.1298445454056,0.0906176904940206,
123.80221599695));
#210091=CARTESIAN_POINT('Ctrl Pts',(46.8513969215926,-5.84212150519187,
126.943291183793));
#210092=CARTESIAN_POINT('Ctrl Pts',(46.5729492977799,-6.40623644110861,
133.632500556544));
#210093=CARTESIAN_POINT('Ctrl Pts',(46.2945016739667,-1.08333304969514,
137.722787487691));
#210094=CARTESIAN_POINT('Ctrl Pts',(46.016054050154,5.23510049062639,135.455378109134));
#210095=CARTESIAN_POINT('Ctrl Pts',(45.737606426341,6.7427324289391,128.913910870662));
#210096=CARTESIAN_POINT('Ctrl Pts',(45.4591588025282,2.0541226658487,124.10967459599));
#210097=CARTESIAN_POINT('Ctrl Pts',(45.1807111787153,-4.5221254776858,125.457527721552));
#210098=CARTESIAN_POINT('Ctrl Pts',(44.9022635549024,-6.94276122533821,
131.718859071242));
#210099=CARTESIAN_POINT('Ctrl Pts',(44.6238159310895,-2.98333857964632,
137.139811017737));
#210100=CARTESIAN_POINT('Ctrl Pts',(44.3453683072766,3.71762647654865,136.738793550433));
#210101=CARTESIAN_POINT('Ctrl Pts',(44.0669206834637,7.00227441694529,130.88432213099));
#210102=CARTESIAN_POINT('Ctrl Pts',(43.7884730596509,3.85217424829189,124.956369987047));
#210103=CARTESIAN_POINT('Ctrl Pts',(43.5100254358379,-2.8378858653675,124.402435542326));
#210104=CARTESIAN_POINT('Ctrl Pts',(43.2315778120251,-6.92006750718621,
129.731557490323));
#210105=CARTESIAN_POINT('Ctrl Pts',(42.9531301882121,-4.64304517399252,
136.04653310291));
#210106=CARTESIAN_POINT('Ctrl Pts',(42.6746825643993,1.90070884873357,137.544208295828));
#210107=CARTESIAN_POINT('Ctrl Pts',(42.3962349405864,6.69780429426274,132.848292732287));
#210108=CARTESIAN_POINT('Ctrl Pts',(42.1177873167735,5.33994479929498,126.274103406951));
#210109=CARTESIAN_POINT('Ctrl Pts',(41.8393396929606,-0.925063095418803,
123.862999142802));
#210110=CARTESIAN_POINT('Ctrl Pts',(41.5608920691476,-6.33998319728738,
127.8306669696));
#210111=CARTESIAN_POINT('Ctrl Pts',(41.2824444453348,-5.92876846624656,
134.531013985867));
#210112=CARTESIAN_POINT('Ctrl Pts',(41.0039968215219,-0.069305151166692,
137.806748613804));
#210113=CARTESIAN_POINT('Ctrl Pts',(40.725549197709,5.85384621209049,134.647630758868));
#210114=CARTESIAN_POINT('Ctrl Pts',(40.4471015738961,6.39759888272248,127.956735398261));
#210115=CARTESIAN_POINT('Ctrl Pts',(40.1686539500832,1.06227072021291,123.882668499967));
#210116=CARTESIAN_POINT('Ctrl Pts',(39.8902063262704,-5.24923233936253,
126.169298514289));
#210117=CARTESIAN_POINT('Ctrl Pts',(39.6117587024575,-6.73694731831984,
132.715324166149));
#210118=CARTESIAN_POINT('Ctrl Pts',(39.3333110786445,-2.03373682991476,
137.505267672621));
#210119=CARTESIAN_POINT('Ctrl Pts',(39.0548634548317,4.53837845161457,136.137404953004));
#210120=CARTESIAN_POINT('Ctrl Pts',(38.7764158310188,6.9399456482232,129.86873502282));
#210121=CARTESIAN_POINT('Ctrl Pts',(38.4979682072059,2.96404182930761,124.459859306355));
#210122=CARTESIAN_POINT('Ctrl Pts',(38.219520583393,-3.73567162924815,124.881270348773));
#210123=CARTESIAN_POINT('Ctrl Pts',(37.9410729595801,-7.00248535822977,
130.745711989165));
#210124=CARTESIAN_POINT('Ctrl Pts',(37.6626253357672,-3.83435713342598,
136.664048853912));
#210125=CARTESIAN_POINT('Ctrl Pts',(37.3841777119543,2.8573579782368,137.197618491141));
#210126=CARTESIAN_POINT('Ctrl Pts',(37.1057300881414,6.92330069759731,131.856096470565));
#210127=CARTESIAN_POINT('Ctrl Pts',(36.8272824643285,4.62706829790778,125.548080581235));
#210128=CARTESIAN_POINT('Ctrl Pts',(36.5488348405156,-1.92121382270608,
124.070329261737));
#210129=CARTESIAN_POINT('Ctrl Pts',(36.2703872167028,-6.70399429676593,
128.780823782526));
#210130=CARTESIAN_POINT('Ctrl Pts',(35.9919395928899,-5.32613152042688,
135.350849799446));
#210131=CARTESIAN_POINT('Ctrl Pts',(35.7134919690769,0.946185927194629,
137.742874366562));
#210132=CARTESIAN_POINT('Ctrl Pts',(35.4350443452641,6.34900473147662,133.758743763591));
#210133=CARTESIAN_POINT('Ctrl Pts',(35.1565967214512,5.91739835365575,127.059679379064));
#210134=CARTESIAN_POINT('Ctrl Pts',(34.8781490976383,0.0479919698059151,
123.80179411487));
#210135=CARTESIAN_POINT('Ctrl Pts',(34.5997014738253,-5.8655166897575,126.978925372262));
#210136=CARTESIAN_POINT('Ctrl Pts',(34.3212538500126,-6.38890205785425,
133.671444737187));
#210137=CARTESIAN_POINT('Ctrl Pts',(34.0428062261996,-1.04119854999986,
137.729253861025));
#210138=CARTESIAN_POINT('Ctrl Pts',(33.7643586023867,5.26331555992738,135.423424393967));
#210139=CARTESIAN_POINT('Ctrl Pts',(33.4859109785738,6.73109979754094,128.872900970206));
#210140=CARTESIAN_POINT('Ctrl Pts',(33.207463354761,2.01333215372067,124.097294605319));
#210141=CARTESIAN_POINT('Ctrl Pts',(32.9290157309481,-4.55458938262534,
125.485154247296));
#210142=CARTESIAN_POINT('Ctrl Pts',(32.6505681071352,-6.93706578039975,
131.761104685873));
#210143=CARTESIAN_POINT('Ctrl Pts',(32.3721204833222,-2.94471762049033,
137.157854065221));
#210144=CARTESIAN_POINT('Ctrl Pts',(32.0936728595094,3.75368217519627,136.716053351584));
#210145=CARTESIAN_POINT('Ctrl Pts',(31.8152252356965,7.00263142944649,130.84169581763));
#210146=CARTESIAN_POINT('Ctrl Pts',(31.5367776118836,3.8165044975991,124.933029058741));
#210147=CARTESIAN_POINT('Ctrl Pts',(31.2583299880707,-2.87680362093211,
124.41982917192));
#210148=CARTESIAN_POINT('Ctrl Pts',(30.9798823642578,-6.92646975149653,
129.773701781947));
#210149=CARTESIAN_POINT('Ctrl Pts',(30.7014347404449,-4.6110485572945,136.074699511423));
#210150=CARTESIAN_POINT('Ctrl Pts',(30.422987116632,1.94170099881587,137.532513267813));
#210151=CARTESIAN_POINT('Ctrl Pts',(30.1445394928192,6.71012219438185,132.807483427156));
#210152=CARTESIAN_POINT('Ctrl Pts',(29.8660918690062,5.31226890100394,126.241681582474));
#210153=CARTESIAN_POINT('Ctrl Pts',(29.5876442451933,-0.967299993633269,
123.868758871779));
#210154=CARTESIAN_POINT('Ctrl Pts',(29.3091966213805,-6.35796744935336,
127.869315342481));
#210155=CARTESIAN_POINT('Ctrl Pts',(29.0307489975676,-5.90597342309497,
134.567035036052));
#210156=CARTESIAN_POINT('Ctrl Pts',(28.7523013737546,-0.026678343854083,
137.807040755898));
#210157=CARTESIAN_POINT('Ctrl Pts',(28.4738537499418,5.87713283007914,134.611925528561));
#210158=CARTESIAN_POINT('Ctrl Pts',(28.1954061261289,6.38014604707014,127.917844157905));
#210159=CARTESIAN_POINT('Ctrl Pts',(27.916958502316,1.02011673426565,123.876330399509));
#210160=CARTESIAN_POINT('Ctrl Pts',(27.6385108785031,-5.27735002185588,
126.201337958415));
#210161=CARTESIAN_POINT('Ctrl Pts',(27.3600632546902,-6.72518992077305,
132.756298470923));
#210162=CARTESIAN_POINT('Ctrl Pts',(27.0816156308773,-1.99290882629253,
137.51752345366));
#210163=CARTESIAN_POINT('Ctrl Pts',(26.8031680070644,4.57075812054227,136.109679746264));
#210164=CARTESIAN_POINT('Ctrl Pts',(26.5247203832516,6.93412164854658,129.826506938842));
#210165=CARTESIAN_POINT('Ctrl Pts',(26.2462727594386,2.92536613221128,124.441933891359));
#210166=CARTESIAN_POINT('Ctrl Pts',(25.9678251356258,-3.7716579475455,124.904120183435));
#210167=CARTESIAN_POINT('Ctrl Pts',(25.6893775118128,-7.00271262924226,
130.788339191706));
#210168=CARTESIAN_POINT('Ctrl Pts',(25.410929888,-3.79861650619593,136.687281107654));
#210169=CARTESIAN_POINT('Ctrl Pts',(25.1324822641871,2.89622261331168,137.180106489852));
#210170=CARTESIAN_POINT('Ctrl Pts',(24.8540346403742,6.92957463952618,131.813932887921));
#210171=CARTESIAN_POINT('Ctrl Pts',(24.5755870165613,4.59498610055721,125.520011689881));
#210172=CARTESIAN_POINT('Ctrl Pts',(24.2971393927484,-1.96217018727317,
124.082149001586));
#210173=CARTESIAN_POINT('Ctrl Pts',(24.0186917689355,-6.71618793034234,
128.821670390082));
#210174=CARTESIAN_POINT('Ctrl Pts',(23.7402441451226,-5.29835706944761,
135.383187237832));
#210175=CARTESIAN_POINT('Ctrl Pts',(23.4617965213097,0.988405099136929,
137.736986109674));
#210176=CARTESIAN_POINT('Ctrl Pts',(23.1833488974968,6.36687126788796,133.720040831851));
#210177=CARTESIAN_POINT('Ctrl Pts',(22.9049012736839,5.89449378040337,127.023727875996));
#210178=CARTESIAN_POINT('Ctrl Pts',(22.6264536498711,0.00536447075796404,
123.801631715467));
#210179=CARTESIAN_POINT('Ctrl Pts',(22.3480060260581,-5.88869452544514,
127.01470131364));
#210180=CARTESIAN_POINT('Ctrl Pts',(22.0695584022453,-6.3713309314846,133.710282676972));
#210181=CARTESIAN_POINT('Ctrl Pts',(21.7911107784324,-0.999025468309402,
137.735463629893));
#210182=CARTESIAN_POINT('Ctrl Pts',(21.5126631546195,5.29133559513472,135.391299517692));
#210183=CARTESIAN_POINT('Ctrl Pts',(21.2342155308066,6.71921774276442,128.831962640697));
#210184=CARTESIAN_POINT('Ctrl Pts',(20.9557679069937,1.97246703682929,124.085163147446));
#210185=CARTESIAN_POINT('Ctrl Pts',(20.6773202831809,-4.58688451558038,
125.51297787819));
#210186=CARTESIAN_POINT('Ctrl Pts',(20.3988726593679,-6.93111327993769,
131.803314848003));
#210187=CARTESIAN_POINT('Ctrl Pts',(20.120425035555,-2.90598754374001,137.175661681671));
#210188=CARTESIAN_POINT('Ctrl Pts',(19.8419774117421,3.78959877977074,136.693094092787));
#210189=CARTESIAN_POINT('Ctrl Pts',(19.5635297879293,7.00272895686486,130.799068120799));
#210190=CARTESIAN_POINT('Ctrl Pts',(19.2850821641163,3.78069332492835,124.909905694786));
#210191=CARTESIAN_POINT('Ctrl Pts',(19.0066345403035,-2.91561477548059,
124.437459382677));
#210192=CARTESIAN_POINT('Ctrl Pts',(18.7281869164906,-6.932615332923,129.815884265012));
#210193=CARTESIAN_POINT('Ctrl Pts',(18.4497392926777,-4.57888107649638,
136.102670625591));
#210194=CARTESIAN_POINT('Ctrl Pts',(18.1712916688647,1.98262119845391,137.520568925627));
#210195=CARTESIAN_POINT('Ctrl Pts',(17.892844045052,6.72219144845534,132.766599895572));
#210196=CARTESIAN_POINT('Ctrl Pts',(17.614396421239,5.28439615463518,126.209428829746));
#210197=CARTESIAN_POINT('Ctrl Pts',(17.3359487974261,-1.00950104819076,
123.87477560203));
#210198=CARTESIAN_POINT('Ctrl Pts',(17.0575011736132,-6.37571610459714,
127.908072474542));
#210199=CARTESIAN_POINT('Ctrl Pts',(16.7790535498004,-5.88295953192644,
134.602916658952));
#210200=CARTESIAN_POINT('Ctrl Pts',(16.5006059259874,0.0159494520341194,
137.807073411106));
#210201=CARTESIAN_POINT('Ctrl Pts',(16.2221583021745,5.90020166874948,134.576079207535));
#210202=CARTESIAN_POINT('Ctrl Pts',(15.9437106783617,6.3624567927597,127.879059878479));
#210203=CARTESIAN_POINT('Ctrl Pts',(15.6652630545488,0.977924947517885,
123.870249019757));
#210204=CARTESIAN_POINT('Ctrl Pts',(15.3868154307359,-5.3052721502032,126.233547969238));
#210205=CARTESIAN_POINT('Ctrl Pts',(15.108367806923,-6.71318331884074,132.797200445919));
#210206=CARTESIAN_POINT('Ctrl Pts',(14.8299201831101,-1.95200697470083,
137.529530475982));
#210207=CARTESIAN_POINT('Ctrl Pts',(14.5514725592972,4.6029684183469,136.081757948972));
#210208=CARTESIAN_POINT('Ctrl Pts',(14.2730249354843,6.92804070244224,129.784315089592));
#210209=CARTESIAN_POINT('Ctrl Pts',(13.9945773116714,2.88658203459712,124.424244238425));
#210210=CARTESIAN_POINT('Ctrl Pts',(13.7161296878585,-3.80750450567058,
124.927188653676));
#210211=CARTESIAN_POINT('Ctrl Pts',(13.4376820640456,-7.00268041216303,
130.830966987928));
#210212=CARTESIAN_POINT('Ctrl Pts',(13.1592344402328,-3.7627351198343,136.710295367612));
#210213=CARTESIAN_POINT('Ctrl Pts',(12.8807868164199,2.93497992779253,137.162358232954));
#210214=CARTESIAN_POINT('Ctrl Pts',(12.602339192607,6.93559180351842,131.771731895206));
#210215=CARTESIAN_POINT('Ctrl Pts',(12.323891568794,4.56273363430679,125.49213861202));
#210216=CARTESIAN_POINT('Ctrl Pts',(12.0454439449812,-2.00305384290271,
124.094217835458));
#210217=CARTESIAN_POINT('Ctrl Pts',(11.7669963211683,-6.72813269310505,
128.862590466954));
#210218=CARTESIAN_POINT('Ctrl Pts',(11.4885486973554,-5.27038628589867,
135.415355006116));
#210219=CARTESIAN_POINT('Ctrl Pts',(11.2101010735425,1.03058764536478,137.730840961799));
#210220=CARTESIAN_POINT('Ctrl Pts',(10.9316534497296,6.38450187754329,133.681229858508));
#210221=CARTESIAN_POINT('Ctrl Pts',(10.6532058259167,5.87137078451608,126.987916465666));
#210222=CARTESIAN_POINT('Ctrl Pts',(10.3747582021038,-0.0372632270726686,
123.801728804758));
#210223=CARTESIAN_POINT('Ctrl Pts',(10.0963105782909,-5.91165415339157,
127.050617682238));
#210224=CARTESIAN_POINT('Ctrl Pts',(9.81786295447806,-6.35352371310424,
133.749012936746));
#210225=CARTESIAN_POINT('Ctrl Pts',(9.53941533066515,-0.956815367363035,
137.741416564191));
#210226=CARTESIAN_POINT('Ctrl Pts',(9.26096770685226,5.31915955795546,135.35900467071));
#210227=CARTESIAN_POINT('Ctrl Pts',(8.98252008303941,6.70708670490366,128.791097399121));
#210228=CARTESIAN_POINT('Ctrl Pts',(8.70407245922646,1.93152882944647,124.073280671906));
#210229=CARTESIAN_POINT('Ctrl Pts',(8.42562483541358,-4.61900967984285,
125.540997583217));
#210230=CARTESIAN_POINT('Ctrl Pts',(8.14717721160073,-6.92490394452403,
131.845487993513));
#210231=CARTESIAN_POINT('Ctrl Pts',(7.86872958778781,-2.86714978455288,
137.193233207215));
#210232=CARTESIAN_POINT('Ctrl Pts',(7.59028196397491,3.82537495936868,136.669916624805));
#210233=CARTESIAN_POINT('Ctrl Pts',(7.31183434016203,7.00256699558648,130.756440620084));
#210234=CARTESIAN_POINT('Ctrl Pts',(7.03338671634916,3.7447420572761,124.887000752025));
#210235=CARTESIAN_POINT('Ctrl Pts',(6.75493909253623,-2.95431789085107,
124.455325521299));
#210236=CARTESIAN_POINT('Ctrl Pts',(6.47649146872337,-6.9385040237388,129.858103376433));
#210237=CARTESIAN_POINT('Ctrl Pts',(6.19804384491048,-4.54654392357636,
136.130445408932));
#210238=CARTESIAN_POINT('Ctrl Pts',(5.91959622109758,2.02346793133434,137.508375711873));
#210239=CARTESIAN_POINT('Ctrl Pts',(5.64114859728465,6.73401160925262,132.725643652489));
#210240=CARTESIAN_POINT('Ctrl Pts',(5.36270097347181,5.25632759302358,126.177346343905));
#210241=CARTESIAN_POINT('Ctrl Pts',(5.08425334965889,-1.05166469531565,
123.881049110601));
#210242=CARTESIAN_POINT('Ctrl Pts',(4.80580572584599,-6.39322850533622,
127.946936929627));
#210243=CARTESIAN_POINT('Ctrl Pts',(4.5273581020331,-5.85972764552883,134.638657524961));
#210244=CARTESIAN_POINT('Ctrl Pts',(4.24891047822024,0.0585766569097649,
137.806846578216));
#210245=CARTESIAN_POINT('Ctrl Pts',(3.97046285440732,5.92305187327717,134.54009312409));
#210246=CARTESIAN_POINT('Ctrl Pts',(3.69201523059441,6.34453177527304,127.840383997147));
#210247=CARTESIAN_POINT('Ctrl Pts',(3.41356760678156,0.935696923401329,
123.864424586062));
#210248=CARTESIAN_POINT('Ctrl Pts',(3.13511998296867,-5.33299768974021,
126.265927353204));
#210249=CARTESIAN_POINT('Ctrl Pts',(2.85667235915575,-6.70092795743158,
132.838028575505));
#210250=CARTESIAN_POINT('Ctrl Pts',(2.57822473534285,-1.91103279077285,
137.541288294661));
#210251=CARTESIAN_POINT('Ctrl Pts',(2.29977711153,4.63500815146407,136.053640595781));
#210252=CARTESIAN_POINT('Ctrl Pts',(2.02132948771708,6.92170303524179,129.742161038504));
#210253=CARTESIAN_POINT('Ctrl Pts',(1.74288186390418,2.84769097362441,124.40679100305));
#210254=CARTESIAN_POINT('Ctrl Pts',(1.46443424009131,-3.84320997531586,
124.950474904685));
#210255=CARTESIAN_POINT('Ctrl Pts',(1.18598661627842,-7.00238870818588,
130.873593798241));
#210256=CARTESIAN_POINT('Ctrl Pts',(0.907538992465495,-3.72671430393905,
136.733090780986));
#210257=CARTESIAN_POINT('Ctrl Pts',(0.629091368652655,2.97362848551254,
137.144374378117));
#210258=CARTESIAN_POINT('Ctrl Pts',(0.350643744839755,6.94135196660579,
131.729495056193));
#210259=CARTESIAN_POINT('Ctrl Pts',(0.0721961210268491,4.53031209428387,
125.4644623805));
#210260=CARTESIAN_POINT('Ctrl Pts',(-0.206251502786054,-2.04386327463549,
124.106535316138));
#210261=CARTESIAN_POINT('Ctrl Pts',(-0.484699126598912,-6.73982814243653,
128.903582496833));
#210262=CARTESIAN_POINT('Ctrl Pts',(-0.763146750411823,-5.24222020624778,
135.447351912307));
#210263=CARTESIAN_POINT('Ctrl Pts',(-1.04159437422473,1.07273200278813,
137.724439150648));
#210264=CARTESIAN_POINT('Ctrl Pts',(-1.32004199803759,6.40189590713365,
133.642312281717));
#210265=CARTESIAN_POINT('Ctrl Pts',(-1.59848962185049,5.84803022282516,
126.952246475077));
#210266=CARTESIAN_POINT('Ctrl Pts',(-1.87693724566341,-0.0798895441007186,
123.802085379146));
#210267=CARTESIAN_POINT('Ctrl Pts',(-2.1553848694763,-5.93439472281934,
127.08667314716));
#210268=CARTESIAN_POINT('Ctrl Pts',(-2.43383249328916,-6.33548106256618,
133.787634081347));
#210269=CARTESIAN_POINT('Ctrl Pts',(-2.71228011710207,-0.914569811271147,
137.747112443329));
#210270=CARTESIAN_POINT('Ctrl Pts',(-2.99072774091498,5.34678641736288,
135.326541049718));
#210271=CARTESIAN_POINT('Ctrl Pts',(-3.26917536472784,6.6947071334783,128.750306759754));
#210272=CARTESIAN_POINT('Ctrl Pts',(-3.54762298854074,1.89051904855254,
124.061647619009));
#210273=CARTESIAN_POINT('Ctrl Pts',(-3.82607061235365,-4.65096368500298,
125.569212324096));
#210274=CARTESIAN_POINT('Ctrl Pts',(-4.10451823616654,-6.91843800424817,
131.887622559669));
#210275=CARTESIAN_POINT('Ctrl Pts',(-4.38296585997939,-2.82820578207579,
137.210567990736));
#210276=CARTESIAN_POINT('Ctrl Pts',(-4.66141348379231,3.86100938829084,
136.646521806489));
#210277=CARTESIAN_POINT('Ctrl Pts',(-4.93986110760522,7.00214555161287,
130.713814895061));
#210278=CARTESIAN_POINT('Ctrl Pts',(-5.21830873141809,3.70865202682979,
124.864315079211));
#210279=CARTESIAN_POINT('Ctrl Pts',(-5.49675635523098,-2.99291153288594,
124.473426925751));
#210280=CARTESIAN_POINT('Ctrl Pts',(-5.77520397904388,-6.9441356057364,
129.900357551763));
#210281=CARTESIAN_POINT('Ctrl Pts',(-6.05365160285679,-4.51403829679898,
136.158022832244));
#210282=CARTESIAN_POINT('Ctrl Pts',(-6.33209922666964,2.06423968386644,
137.495934078373));
#210283=CARTESIAN_POINT('Ctrl Pts',(-6.61054685048256,6.74558223877327,
132.684616215558));
#210284=CARTESIAN_POINT('Ctrl Pts',(-6.88899447429547,5.22806425626005,
126.145435313781));
#210285=CARTESIAN_POINT('Ctrl Pts',(-7.16744209810832,-1.09378937261818,
123.887579165027));
#210286=CARTESIAN_POINT('Ctrl Pts',(-7.44588972192122,-6.41050400264194,
127.985907267597));
#210287=CARTESIAN_POINT('Ctrl Pts',(-7.72433734573414,-5.8362786247684,
134.674256309687));
#210288=CARTESIAN_POINT('Ctrl Pts',(-8.002784969547,0.101201691205851,137.806360265633));
#210289=CARTESIAN_POINT('Ctrl Pts',(-8.28123259335988,5.94568259693924,
134.503968611703));
#210290=CARTESIAN_POINT('Ctrl Pts',(-8.55968021717279,6.32637165882838,
127.80181794706));
#210291=CARTESIAN_POINT('Ctrl Pts',(-8.8381278409857,0.893434226691435,
123.858857314246));
#210292=CARTESIAN_POINT('Ctrl Pts',(-9.11657546479855,-5.3605256130866,
126.298474910485));
#210293=CARTESIAN_POINT('Ctrl Pts',(-9.39502308861147,-6.68842429067269,
132.878781346775));
#210294=CARTESIAN_POINT('Ctrl Pts',(-9.67347071242438,-1.86998779282204,
137.552796474009));
#210295=CARTESIAN_POINT('Ctrl Pts',(-9.95191833623725,4.66687613264966,
136.025328728591));
#210296=CARTESIAN_POINT('Ctrl Pts',(-10.2303659600501,6.91510888178999,
129.700046347612));
#210297=CARTESIAN_POINT('Ctrl Pts',(-10.508813583863,2.80869439041515,124.389574831969));
#210298=CARTESIAN_POINT('Ctrl Pts',(-10.787261207676,-3.87877303340228,
124.973978073582));
#210299=CARTESIAN_POINT('Ctrl Pts',(-11.0657088314888,-7.00183752812002,
130.916218043094));
#210300=CARTESIAN_POINT('Ctrl Pts',(-11.3441564553017,-3.69055539327479,
136.755666503084));
#210301=CARTESIAN_POINT('Ctrl Pts',(-11.6226040791146,3.01216685433575,
137.126155591738));
#210302=CARTESIAN_POINT('Ctrl Pts',(-11.9010517029275,6.94685491534338,
131.687223935982));
#210303=CARTESIAN_POINT('Ctrl Pts',(-12.1794993267404,4.49772268187999,
125.436984020872));
#210304=CARTESIAN_POINT('Ctrl Pts',(-12.4579469505533,-2.08459697026297,
124.119100987199));
#210305=CARTESIAN_POINT('Ctrl Pts',(-12.7363945743662,-6.75127384495765,
128.944644960744));
#210306=CARTESIAN_POINT('Ctrl Pts',(-13.0148421981791,-5.21385987419926,
135.479176770748));
#210307=CARTESIAN_POINT('Ctrl Pts',(-13.2932898219919,1.11483660973293,
137.717780913442));
#210308=CARTESIAN_POINT('Ctrl Pts',(-13.5717374458049,6.41905271211686,
133.603289543584));
#210309=CARTESIAN_POINT('Ctrl Pts',(-13.8501850696177,5.82447296022373,
126.916719225995));
#210310=CARTESIAN_POINT('Ctrl Pts',(-14.1286326934306,-0.122512900792341,
123.802701425419));
#210311=CARTESIAN_POINT('Ctrl Pts',(-14.4070803172435,-5.95691539106803,
127.122866372359));
#210312=CARTESIAN_POINT('Ctrl Pts',(-14.6855279410564,-6.31720364844761,
133.826144679651));
#210313=CARTESIAN_POINT('Ctrl Pts',(-14.9639755648693,-0.872290365458834,
137.752551056246));
#210314=CARTESIAN_POINT('Ctrl Pts',(-15.2424231886822,5.37421514963333,
135.293909857666));
#210315=CARTESIAN_POINT('Ctrl Pts',(-15.5208708124951,6.68207948721813,
128.709592234107));
#210316=CARTESIAN_POINT('Ctrl Pts',(-15.799318436308,1.84943921378025,124.050264419823));
#210317=CARTESIAN_POINT('Ctrl Pts',(-16.0777660601209,-4.68274534699314,
125.59762105532));
#210318=CARTESIAN_POINT('Ctrl Pts',(-16.3562136839338,-6.91171569870797,
131.929716985153));
#210319=CARTESIAN_POINT('Ctrl Pts',(-16.6346613077467,-2.78915697939336,
137.227665389888));
#210320=CARTESIAN_POINT('Ctrl Pts',(-16.9131089315595,3.89650074609022,
136.622910504741));
#210321=CARTESIAN_POINT('Ctrl Pts',(-17.1915565553724,7.00146464056082,
130.671192525245));
#210322=CARTESIAN_POINT('Ctrl Pts',(-17.4700041791854,3.67242457091876,
124.841849516969));
#210323=CARTESIAN_POINT('Ctrl Pts',(-17.7484518029982,-3.0313942714833,
124.491762925279));
#210324=CARTESIAN_POINT('Ctrl Pts',(-18.0268994268111,-6.94950987023543,
129.942645225261));
#210325=CARTESIAN_POINT('Ctrl Pts',(-18.305347050624,-4.48136540067248,
136.185401873632));
#210326=CARTESIAN_POINT('Ctrl Pts',(-18.5837946744369,2.10493494523792,
137.483244486159));
#210327=CARTESIAN_POINT('Ctrl Pts',(-18.8622422982498,6.75690290826339,
132.643519105064));
#210328=CARTESIAN_POINT('Ctrl Pts',(-19.1406899220627,5.19960719165284,
126.113696921846));
#210329=CARTESIAN_POINT('Ctrl Pts',(-19.4191375458756,-1.1358735191536,
123.894365523333));
#210330=CARTESIAN_POINT('Ctrl Pts',(-19.6975851696885,-6.42754195636435,
128.024982044393));
#210331=CARTESIAN_POINT('Ctrl Pts',(-19.9760327935014,-5.81261333855723,
134.709711694007));
#210332=CARTESIAN_POINT('Ctrl Pts',(-20.2544804173143,0.143822975436045,
137.805614491377));
#210333=CARTESIAN_POINT('Ctrl Pts',(-20.5329280411272,5.96809300114641,
134.467707008981));
#210334=CARTESIAN_POINT('Ctrl Pts',(-20.81137566494,6.30797711635522,127.763363157294));
#210335=CARTESIAN_POINT('Ctrl Pts',(-21.089823288753,0.851138423447451,
123.853547410611));
#210336=CARTESIAN_POINT('Ctrl Pts',(-21.3682709125658,-5.38785490018508,
126.331189435016));
#210337=CARTESIAN_POINT('Ctrl Pts',(-21.6467185363787,-6.67567278189203,
132.919457249623));
#210338=CARTESIAN_POINT('Ctrl Pts',(-21.9251661601916,-1.82887350178604,
137.564054587584));
#210339=CARTESIAN_POINT('Ctrl Pts',(-22.2036137840045,4.69857118102365,
135.996823396506));
#210340=CARTESIAN_POINT('Ctrl Pts',(-22.4820614078173,6.90825848643574,
129.657972577492));
#210341=CARTESIAN_POINT('Ctrl Pts',(-22.7605090316303,2.76959373000234,
124.372596363135));
#210342=CARTESIAN_POINT('Ctrl Pts',(-23.0389566554432,-3.91419236212754,
124.997697289448));
#210343=CARTESIAN_POINT('Ctrl Pts',(-23.3174042792561,-7.0010268923895,
130.958838143028));
#210344=CARTESIAN_POINT('Ctrl Pts',(-23.5958519030689,-3.65425972772349,
136.778021697354));
#210345=CARTESIAN_POINT('Ctrl Pts',(-23.8742995268818,3.05059360620828,
137.107702548922));
#210346=CARTESIAN_POINT('Ctrl Pts',(-24.1527471506948,6.95210044581739,
131.644920100946));
#210347=CARTESIAN_POINT('Ctrl Pts',(-24.4311947745076,4.4649666047081,125.409704551357));
#210348=CARTESIAN_POINT('Ctrl Pts',(-24.7096423983205,-2.12525342038311,
124.131914383013));
#210349=CARTESIAN_POINT('Ctrl Pts',(-24.9880900221334,-6.76246937654364,
128.985776337104));
#210350=CARTESIAN_POINT('Ctrl Pts',(-25.2665376459463,-5.18530634065569,
135.510828402156));
#210351=CARTESIAN_POINT('Ctrl Pts',(-25.5449852697592,1.15689990599717,
137.710866496904));
#210352=CARTESIAN_POINT('Ctrl Pts',(-25.8234328935721,6.43597165674122,
133.564163090109));
#210353=CARTESIAN_POINT('Ctrl Pts',(-26.101880517385,5.8006998696348,126.881336034893));
#210354=CARTESIAN_POINT('Ctrl Pts',(-26.3803281411979,-0.165131717723356,
123.803576920747));
#210355=CARTESIAN_POINT('Ctrl Pts',(-26.6587757650107,-5.9792153236265,
127.15919601668));
#210356=CARTESIAN_POINT('Ctrl Pts',(-26.9372233888237,-6.29869214802456,
133.864543304637));
#210357=CARTESIAN_POINT('Ctrl Pts',(-27.2156710126366,-0.829978596605981,
137.75773220141));
#210358=CARTESIAN_POINT('Ctrl Pts',(-27.4941186364494,5.40144473838504,
135.261112303716));
#210359=CARTESIAN_POINT('Ctrl Pts',(-27.7725662602623,6.66920423404522,
128.668955330874));
#210360=CARTESIAN_POINT('Ctrl Pts',(-28.0510138840753,1.80829084735756,
124.039131496154));
#210361=CARTESIAN_POINT('Ctrl Pts',(-28.3294615078881,-4.71435348813263,
125.626222724194));
#210362=CARTESIAN_POINT('Ctrl Pts',(-28.607909131701,-6.9047372770006,131.971769710144));
#210363=CARTESIAN_POINT('Ctrl Pts',(-28.8863567555139,-2.75000482347336,
137.244524771118));
#210364=CARTESIAN_POINT('Ctrl Pts',(-29.1648043793268,3.93184771762154,
136.599083594488));
#210365=CARTESIAN_POINT('Ctrl Pts',(-29.4432520031397,7.00052428766157,
130.628575090021));
#210366=CARTESIAN_POINT('Ctrl Pts',(-29.7216996269525,3.63606103196502,
124.819604897767));
#210367=CARTESIAN_POINT('Ctrl Pts',(-30.0001472507655,-3.06976468065099,
124.510332840438));
#210368=CARTESIAN_POINT('Ctrl Pts',(-30.2785948745783,-6.95462661809053,
129.984964829937));
#210369=CARTESIAN_POINT('Ctrl Pts',(-30.5570424983912,-4.44852644590303,
136.212581518559));
#210370=CARTESIAN_POINT('Ctrl Pts',(-30.8354901222041,2.14555220747066,
137.470307405446));
#210371=CARTESIAN_POINT('Ctrl Pts',(-31.113937746017,6.7679731982313,132.602353843876));
#210372=CARTESIAN_POINT('Ctrl Pts',(-31.3923853698299,5.17095745368924,
126.082132344179));
#210373=CARTESIAN_POINT('Ctrl Pts',(-31.6708329936428,-1.17791557547805,
123.901407934047));
#210374=CARTESIAN_POINT('Ctrl Pts',(-31.9492806174558,-6.44434173515584,
128.064159812084));
#210375=CARTESIAN_POINT('Ctrl Pts',(-32.2277282412685,-5.78873266382121,
134.745022364106));
#210376=CARTESIAN_POINT('Ctrl Pts',(-32.5061758650815,0.186438930252996,
137.804609283086));
#210377=CARTESIAN_POINT('Ctrl Pts',(-32.7846234888944,5.99028225547263,
134.431309659613));
#210378=CARTESIAN_POINT('Ctrl Pts',(-33.0630711127073,6.28934882947028,
127.725021052809));
#210379=CARTESIAN_POINT('Ctrl Pts',(-33.3415187365202,0.808811080956172,
123.848495071916));
#210380=CARTESIAN_POINT('Ctrl Pts',(-33.619966360333,-5.41498453833882,
126.364069714552));
#210381=CARTESIAN_POINT('Ctrl Pts',(-33.898413984146,-6.66267390360147,
132.960054776787));
#210382=CARTESIAN_POINT('Ctrl Pts',(-34.1768616079588,-1.78769144116968,
137.575062218212));
#210383=CARTESIAN_POINT('Ctrl Pts',(-34.4553092317717,4.73009212211488,
135.968125655805));
#210384=CARTESIAN_POINT('Ctrl Pts',(-34.7337568555846,6.90115210302259,
129.615941287202));
#210385=CARTESIAN_POINT('Ctrl Pts',(-35.0122044793975,2.73039044127535,
124.355856225691));
#210386=CARTESIAN_POINT('Ctrl Pts',(-35.2906521032104,-3.94946664901538,
125.02163167336));
#210387=CARTESIAN_POINT('Ctrl Pts',(-35.5690997270233,-6.99995683103299,
131.00145251874));
#210388=CARTESIAN_POINT('Ctrl Pts',(-35.8475473508362,-3.61782865223385,
136.800155535415));
#210389=CARTESIAN_POINT('Ctrl Pts',(-36.125994974649,3.08890731721304,137.089015933453));
#210390=CARTESIAN_POINT('Ctrl Pts',(-36.404442598462,6.95708836365274,131.60258511867));
#210391=CARTESIAN_POINT('Ctrl Pts',(-36.6828902222748,4.43204507655667,
125.382624982808));
#210392=CARTESIAN_POINT('Ctrl Pts',(-36.9613378460878,-2.16583111845593,
124.144975028777));
#210393=CARTESIAN_POINT('Ctrl Pts',(-37.2397854699006,-6.7734143223399,
129.026975101771));
#210394=CARTESIAN_POINT('Ctrl Pts',(-37.5182330937135,-5.15656066367905,
135.54230563367));
#210395=CARTESIAN_POINT('Ctrl Pts',(-37.7966807175264,1.19892033290996,
137.703696157251));
#210396=CARTESIAN_POINT('Ctrl Pts',(-38.0751283413393,6.45265211406898,
133.524934371139));
#210397=CARTESIAN_POINT('Ctrl Pts',(-38.3535759651522,5.77671183197903,
126.846098212911));
#210398=CARTESIAN_POINT('Ctrl Pts',(-38.6320235889651,-0.207744415637528,
123.80471183269));
#210399=CARTESIAN_POINT('Ctrl Pts',(-38.910471212778,-6.00129369416227,
127.195660733917));
#210400=CARTESIAN_POINT('Ctrl Pts',(-39.1889188365908,-6.27994724724761,
133.902828533427));
#210401=CARTESIAN_POINT('Ctrl Pts',(-39.4673664604039,-0.787636072591,137.762655686833));
#210402=CARTESIAN_POINT('Ctrl Pts',(-39.7458140842166,5.42847417461558,
135.228149603194));
#210403=CARTESIAN_POINT('Ctrl Pts',(-40.0242617080296,6.65608185105682,
128.628397555869));
#210404=CARTESIAN_POINT('Ctrl Pts',(-40.3027093318424,1.76707547405252,
124.028249260538));
#210405=CARTESIAN_POINT('Ctrl Pts',(-40.5811569556554,-4.7457869371699,
125.655016270872));
#210406=CARTESIAN_POINT('Ctrl Pts',(-40.8596045794682,-6.89750299771422,
132.013779176361));
#210407=CARTESIAN_POINT('Ctrl Pts',(-41.1380522032811,-2.7107507651133,
137.261145509698));
#210408=CARTESIAN_POINT('Ctrl Pts',(-41.416499827094,3.96704899308973,136.575041958643));
#210409=CARTESIAN_POINT('Ctrl Pts',(-41.694947450907,6.99932452776054,130.585964168594));
#210410=CARTESIAN_POINT('Ctrl Pts',(-41.9733950747197,3.59956275743227,
124.79758204589));
#210411=CARTESIAN_POINT('Ctrl Pts',(-42.2518426985328,-3.10802133855968,
124.529135983109));
#210412=CARTESIAN_POINT('Ctrl Pts',(-42.5302903223456,-6.95948565969872,
130.027314797628));
#210413=CARTESIAN_POINT('Ctrl Pts',(-42.8087379461585,-4.41552264935019,
136.23956075987));
#210414=CARTESIAN_POINT('Ctrl Pts',(-43.0871855699714,2.18608996547759,
137.457123315624));
#210415=CARTESIAN_POINT('Ctrl Pts',(-43.3656331937842,6.77879269846351,
132.561121957388));
#210416=CARTESIAN_POINT('Ctrl Pts',(-43.6440808175972,5.14211610399531,
126.050742750417));
#210417=CARTESIAN_POINT('Ctrl Pts',(-43.92252844141,-1.21991398370768,123.908706136214));
#210418=CARTESIAN_POINT('Ctrl Pts',(-44.200976065223,-6.46090271649442,
128.103439118922));
#210419=CARTESIAN_POINT('Ctrl Pts',(-44.4794236890358,-5.76463748546755,
134.780187011534));
#210420=CARTESIAN_POINT('Ctrl Pts',(-44.7578713128487,0.229047976506494,
137.803344678006));
#210421=CARTESIAN_POINT('Ctrl Pts',(-45.0363189366615,6.01224953768695,
134.394777912313));
#210422=CARTESIAN_POINT('Ctrl Pts',(-45.3147665604746,6.27048748845154,
127.686793054383));
#210423=CARTESIAN_POINT('Ctrl Pts',(-45.5932141842873,0.766453767672844,
123.843700485376));
#210424=CARTESIAN_POINT('Ctrl Pts',(-45.8716618081003,-5.44191352224889,
126.397114530699));
#210425=CARTESIAN_POINT('Ctrl Pts',(-46.1501094319132,-6.6494281374793,
133.000572423912));
#210426=CARTESIAN_POINT('Ctrl Pts',(-46.4285570557261,-1.74644313698983,
137.585818958004));
#210427=CARTESIAN_POINT('Ctrl Pts',(-46.7070046795389,4.76143778790304,
135.93923656989));
#210428=CARTESIAN_POINT('Ctrl Pts',(-46.9854523033519,6.89378999488032,
129.573954034227));
#210429=CARTESIAN_POINT('Ctrl Pts',(-47.2638999271647,2.69108597692664,
124.339355039948));
#210430=CARTESIAN_POINT('Ctrl Pts',(-47.5423475509777,-3.98459458696386,
125.045780338419));
#210431=CARTESIAN_POINT('Ctrl Pts',(-47.8207951747905,-6.998627383702,131.044059591139));
#210432=CARTESIAN_POINT('Ctrl Pts',(-48.0992427986034,-3.58126351677304,
136.822067197091));
#210433=CARTESIAN_POINT('Ctrl Pts',(-48.3776904224163,3.1271065676212,137.070096437769));
#210434=CARTESIAN_POINT('Ctrl Pts',(-48.6561380462292,6.9618184840203,131.560220557891));
#210435=CARTESIAN_POINT('Ctrl Pts',(-48.9345856700421,4.39895931734504,
125.355746318666));
#210436=CARTESIAN_POINT('Ctrl Pts',(-49.213033293855,-2.20632856086043,
124.158282440523));
#210437=CARTESIAN_POINT('Ctrl Pts',(-49.4914809176678,-6.78410827677761,
129.068239728113));
#210438=CARTESIAN_POINT('Ctrl Pts',(-49.7699285414808,-5.12762390845042,
135.573607298891));
#210439=CARTESIAN_POINT('Ctrl Pts',(-50.0483761652936,1.2408963333889,137.696270160183));
#210440=CARTESIAN_POINT('Ctrl Pts',(-50.3268237891066,6.46909346599971,
133.485604840309));
#210441=CARTESIAN_POINT('Ctrl Pts',(-50.6052714129194,5.7525097361419,126.811007065796));
#210442=CARTESIAN_POINT('Ctrl Pts',(-50.8837190367324,-0.250349415506305,
123.806106119193));
#210443=CARTESIAN_POINT('Ctrl Pts',(-51.1621666605453,-6.02314968455324,
127.232259172855));
#210444=CARTESIAN_POINT('Ctrl Pts',(-51.4406142843581,-6.26096964071598,
133.94099894735));
#210445=CARTESIAN_POINT('Ctrl Pts',(-51.719061908171,-0.745264362431691,
137.767321330073));
#210446=CARTESIAN_POINT('Ctrl Pts',(-51.997509531984,5.45530245673899,135.195022977544));
#210447=CARTESIAN_POINT('Ctrl Pts',(-52.2759571557968,6.64271282450778,
128.587920411975));
#210448=CARTESIAN_POINT('Ctrl Pts',(-52.5544047796097,1.72579462111621,
124.01761811622));
#210449=CARTESIAN_POINT('Ctrl Pts',(-52.8328524034226,-4.77704452932697,
125.684000628399));
#210450=CARTESIAN_POINT('Ctrl Pts',(-53.1113000272355,-6.89001312891767,
132.05574382713));
#210451=CARTESIAN_POINT('Ctrl Pts',(-53.3897476510484,-2.67139625888694,
137.277526989739));
#210452=CARTESIAN_POINT('Ctrl Pts',(-53.6681952748612,4.00210326809833,
136.550786488079));
#210453=CARTESIAN_POINT('Ctrl Pts',(-53.9466428986742,6.99786540531528,
130.543361339928));
#210454=CARTESIAN_POINT('Ctrl Pts',(-54.225090522487,3.56293109977782,124.775781777402));
#210455=CARTESIAN_POINT('Ctrl Pts',(-54.5035381462999,-3.14616282759469,
124.548171656537));
#210456=CARTESIAN_POINT('Ctrl Pts',(-54.7819857701128,-6.9640868150063,
130.069693559035));
#210457=CARTESIAN_POINT('Ctrl Pts',(-55.0604333939257,-4.382355233982,136.266338597842));
#210458=CARTESIAN_POINT('Ctrl Pts',(-55.3388810177386,2.22654671711671,
137.443692705233));
#210459=CARTESIAN_POINT('Ctrl Pts',(-55.6173286415515,6.78936100803939,
132.519824973462));
#210460=CARTESIAN_POINT('Ctrl Pts',(-55.8957762653644,5.11308421129812,
126.019529303714));
#210461=CARTESIAN_POINT('Ctrl Pts',(-56.1742238891773,-1.26186718757599,
123.916259859391));
#210462=CARTESIAN_POINT('Ctrl Pts',(-56.4526715129901,-6.47722428670686,
128.142818509401));
#210463=CARTESIAN_POINT('Ctrl Pts',(-56.7311191368031,-5.74032869635189,
134.815204333253));
#210464=CARTESIAN_POINT('Ctrl Pts',(-57.0095667606159,0.271648535303317,
137.801820722997));
#210465=CARTESIAN_POINT('Ctrl Pts',(-57.2880143844289,6.03399403378365,
134.358113120779));
#210466=CARTESIAN_POINT('Ctrl Pts',(-57.5664620082417,6.25139379221294,
127.64868057857));
#210467=CARTESIAN_POINT('Ctrl Pts',(-57.8449096320546,0.724068053163303,
123.839163828657));
#210468=CARTESIAN_POINT('Ctrl Pts',(-58.1233572558676,-5.46864085405239,
126.430322658971));
#210469=CARTESIAN_POINT('Ctrl Pts',(-58.4018048796803,-6.63593597435208,
133.0410086896));
#210470=CARTESIAN_POINT('Ctrl Pts',(-58.6802525034934,-1.705130117717,137.596324408362));
#210471=CARTESIAN_POINT('Ctrl Pts',(-58.9587001273061,4.79260701686295,
135.910157209259));
#210472=CARTESIAN_POINT('Ctrl Pts',(-59.2371477511191,6.88617243481463,
129.532012374421));
#210473=CARTESIAN_POINT('Ctrl Pts',(-59.515595374932,2.65168179339722,124.323093417365));
#210474=CARTESIAN_POINT('Ctrl Pts',(-59.7940429987449,-4.01957487429483,
125.070142389788));
#210475=CARTESIAN_POINT('Ctrl Pts',(-60.0724906225578,-6.99703859965941,
131.086657781405));
#210476=CARTESIAN_POINT('Ctrl Pts',(-60.3509382463707,-3.5445656762756,
136.843755870437));
#210477=CARTESIAN_POINT('Ctrl Pts',(-60.6293858701835,3.16518994194552,
137.050944762941));
#210478=CARTESIAN_POINT('Ctrl Pts',(-60.9078334939965,6.96629063164357,
131.517827988445));
#210479=CARTESIAN_POINT('Ctrl Pts',(-61.1862811178092,4.36571055307847,
125.32906955493));
#210480=CARTESIAN_POINT('Ctrl Pts',(-61.4647287416223,-2.24674424694855,
124.171836125139));
#210481=CARTESIAN_POINT('Ctrl Pts',(-61.743176365435,-6.79455084358828,
129.109568687053));
#210482=CARTESIAN_POINT('Ctrl Pts',(-62.0216239892481,-5.09849714723216,
135.60473223792));
#210483=CARTESIAN_POINT('Ctrl Pts',(-62.3000716130609,1.2828263519976,137.688588780872));
#210484=CARTESIAN_POINT('Ctrl Pts',(-62.5785192368738,6.48529510329292,
133.446175954988));
#210485=CARTESIAN_POINT('Ctrl Pts',(-62.8569668606868,5.72809447894126,
126.776063893867));
#210486=CARTESIAN_POINT('Ctrl Pts',(-63.1354144844995,-0.292945138585431,
123.80775972859));
#210487=CARTESIAN_POINT('Ctrl Pts',(-63.4138621083125,-6.04478248491762,
127.268989977326));
#210488=CARTESIAN_POINT('Ctrl Pts',(-63.6923097321254,-6.24176003165182,
133.979053131985));
#210489=CARTESIAN_POINT('Ctrl Pts',(-63.9707573559382,-0.702865036227365,
137.771728958244));
#210490=CARTESIAN_POINT('Ctrl Pts',(-64.2492049797512,5.48192859062395,
135.161733654286));
#210491=CARTESIAN_POINT('Ctrl Pts',(-64.527652603564,6.62909764979204,128.547525399088));
#210492=CARTESIAN_POINT('Ctrl Pts',(-64.806100227377,1.68444981822529,124.007238457143));
#210493=CARTESIAN_POINT('Ctrl Pts',(-65.0845478511898,-4.80812510634223,
125.713174722747));
#210494=CARTESIAN_POINT('Ctrl Pts',(-65.3629954750027,-6.88226794815085,
132.097662107432));
#210495=CARTESIAN_POINT('Ctrl Pts',(-65.6414430988157,-2.63194276308962,
137.29366860422));
#210496=CARTESIAN_POINT('Ctrl Pts',(-65.9198907226284,4.03700924369883,
136.526318081592));
#210497=CARTESIAN_POINT('Ctrl Pts',(-66.1983383464414,6.99614697439381,
130.500768182686));
#210498=CARTESIAN_POINT('Ctrl Pts',(-66.4767859702543,3.5261674164012,124.75420490012));
#210499=CARTESIAN_POINT('Ctrl Pts',(-66.7552335940671,-3.18418773440913,
124.567439155348));
#210500=CARTESIAN_POINT('Ctrl Pts',(-67.0336812178801,-6.96842991351606,
130.112099543802));
#210501=CARTESIAN_POINT('Ctrl Pts',(-67.3121288416929,-4.34902542882876,
136.292914040211));
#210502=CARTESIAN_POINT('Ctrl Pts',(-67.5905764655059,2.26692096324861,
137.43001607195));
#210503=CARTESIAN_POINT('Ctrl Pts',(-67.8690240893187,6.79967773534632,
132.478464422373));
#210504=CARTESIAN_POINT('Ctrl Pts',(-68.1474717131316,5.08386285138514,
125.988493160695));
#210505=CARTESIAN_POINT('Ctrl Pts',(-68.4259193369445,-1.30377363249137,
123.924068823677));
#210506=CARTESIAN_POINT('Ctrl Pts',(-68.7043669607574,-6.49330584099122,
128.182296524302));
#210507=CARTESIAN_POINT('Ctrl Pts',(-68.9828145845703,-5.71580719724563,
134.850073031684));
#210508=CARTESIAN_POINT('Ctrl Pts',(-69.2612622083832,0.314239028063776,
137.800037474531));
#210509=CARTESIAN_POINT('Ctrl Pts',(-69.5397098321961,6.05551493801243,
134.32131664364));
#210510=CARTESIAN_POINT('Ctrl Pts',(-69.818157456009,6.23206844827842,127.610685037641));
#210511=CARTESIAN_POINT('Ctrl Pts',(-70.0966050798218,0.681655508046095,
123.834885269867));
#210512=CARTESIAN_POINT('Ctrl Pts',(-70.3750527036349,-5.49516554335789,
126.463692868828));
#210513=CARTESIAN_POINT('Ctrl Pts',(-70.6535003274475,-6.62219791417695,
133.081362075471));
#210514=CARTESIAN_POINT('Ctrl Pts',(-70.9319479512606,-1.66375391422059,
137.606578180005));
#210515=CARTESIAN_POINT('Ctrl Pts',(-71.2103955750734,4.82359865400735,
135.880888651457));
#210516=CARTESIAN_POINT('Ctrl Pts',(-71.4888431988863,6.87829970509706,
129.490117861946));
#210517=CARTESIAN_POINT('Ctrl Pts',(-71.7672908226993,2.6121793508235,124.307071960521));
#210518=CARTESIAN_POINT('Ctrl Pts',(-72.045738446512,-4.05440621480077,
125.094716924722));
#210519=CARTESIAN_POINT('Ctrl Pts',(-72.3241860703251,-6.99519053777849,
131.129245511046));
#210520=CARTESIAN_POINT('Ctrl Pts',(-72.6026336941378,-3.5077364905931,
136.865220751771));
#210521=CARTESIAN_POINT('Ctrl Pts',(-72.8810813179508,3.20315602899298,
137.031561618638));
#210522=CARTESIAN_POINT('Ctrl Pts',(-73.1595289417638,6.97050464080582,
131.475408981201));
#210523=CARTESIAN_POINT('Ctrl Pts',(-73.4379765655765,4.33230001580124,
125.302595680118));
#210524=CARTESIAN_POINT('Ctrl Pts',(-73.7164241893894,-2.28707667910305,
124.18563558039));
#210525=CARTESIAN_POINT('Ctrl Pts',(-73.9948718132024,-6.80474163581863,
129.150960447132));
#210526=CARTESIAN_POINT('Ctrl Pts',(-74.2733194370152,-5.0691814593271,
135.635679297414));
#210527=CARTESIAN_POINT('Ctrl Pts',(-74.5517670608282,1.32470883500465,
137.680652303954));
#210528=CARTESIAN_POINT('Ctrl Pts',(-74.830214684641,6.5012564255912,133.406649176227));
#210529=CARTESIAN_POINT('Ctrl Pts',(-75.108662308454,5.70346696509291,126.741269991954));
#210530=CARTESIAN_POINT('Ctrl Pts',(-75.3871099322667,-0.335530006474783,
123.809672599606));
#210531=CARTESIAN_POINT('Ctrl Pts',(-75.6655575560798,-6.06619129364391,
127.305851786256));
#210532=CARTESIAN_POINT('Ctrl Pts',(-75.9440051798925,-6.22231913187452,
134.016989677222));
#210533=CARTESIAN_POINT('Ctrl Pts',(-76.2224528037055,-0.66043966510086,
137.775878408018));
#210534=CARTESIAN_POINT('Ctrl Pts',(-76.5009004275184,5.50835158962877,
135.128282866967));
#210535=CARTESIAN_POINT('Ctrl Pts',(-76.7793480513312,6.61523683142527,
128.507214014061));
#210536=CARTESIAN_POINT('Ctrl Pts',(-77.0577956751442,1.64304259742666,
123.997110667925));
#210537=CARTESIAN_POINT('Ctrl Pts',(-77.336243298957,-4.83902751651344,
125.742537472861));
#210538=CARTESIAN_POINT('Ctrl Pts',(-77.6146909227699,-6.87426774241415,
132.139532463972));
#210539=CARTESIAN_POINT('Ctrl Pts',(-77.8931385465828,-2.59239173968542,
137.309569755007));
#210540=CARTESIAN_POINT('Ctrl Pts',(-78.1715861703958,4.07176562643718,
136.501637645866));
#210541=CARTESIAN_POINT('Ctrl Pts',(-78.4500337942086,6.99416929867323,
130.458186275174));
#210542=CARTESIAN_POINT('Ctrl Pts',(-78.7284814180215,3.48927306959449,
124.732852213582));
#210543=CARTESIAN_POINT('Ctrl Pts',(-79.0069290418344,-3.22209464997582,
124.586937765577));
#210544=CARTESIAN_POINT('Ctrl Pts',(-79.2853766656473,-6.97251479429268,
130.154531180556));
#210545=CARTESIAN_POINT('Ctrl Pts',(-79.5638242894601,-4.3155344689392,
136.319286102215));
#210546=CARTESIAN_POINT('Ctrl Pts',(-79.8422719132732,2.30721120779087,
137.416093922569));
#210547=CARTESIAN_POINT('Ctrl Pts',(-80.1207195370859,6.80974249809405,
132.437041836753));
#210548=CARTESIAN_POINT('Ctrl Pts',(-80.3991671608989,5.0544531070646,125.957635471416));
#210549=CARTESIAN_POINT('Ctrl Pts',(-80.6776147847117,-1.34563176559565,
123.932132739704));
#210550=CARTESIAN_POINT('Ctrl Pts',(-80.9560624085247,-6.50914678343976,
128.221871700751));
#210551=CARTESIAN_POINT('Ctrl Pts',(-81.2345100323374,-5.69107389680138,
134.884791814753));
#210552=CARTESIAN_POINT('Ctrl Pts',(-81.5129576561506,0.356817876581242,
137.797994998686));
#210553=CARTESIAN_POINT('Ctrl Pts',(-81.7914052799631,6.07681145290804,
134.284389844403));
#210554=CARTESIAN_POINT('Ctrl Pts',(-82.0698529037763,6.21251217275584,
127.572807839535));
#210555=CARTESIAN_POINT('Ctrl Pts',(-82.348300527589,0.639217703933302,
123.830864967548));
#210556=CARTESIAN_POINT('Ctrl Pts',(-82.626748151402,-5.52148660728364,
126.497223923725));
#210557=CARTESIAN_POINT('Ctrl Pts',(-82.9051957752149,-6.60821446602265,
133.121631086217));
#210558=CARTESIAN_POINT('Ctrl Pts',(-83.1836433990278,-1.62231605971109,
137.616579892973));
#210559=CARTESIAN_POINT('Ctrl Pts',(-83.4620910228406,4.85441155092967,
135.851431981043));
#210560=CARTESIAN_POINT('Ctrl Pts',(-83.7405386466535,6.87017209745416,
129.448272049221));
#210561=CARTESIAN_POINT('Ctrl Pts',(-84.0189862704665,2.57258011298421,
124.291291263097));
#210562=CARTESIAN_POINT('Ctrl Pts',(-84.2974338942792,-4.08908731779306,
125.119503032603));
#210563=CARTESIAN_POINT('Ctrl Pts',(-84.5758815180923,-6.99308326653956,
131.171821201958));
#210564=CARTESIAN_POINT('Ctrl Pts',(-84.8543291419051,-3.47077732444568,
136.886461045702));
#210565=CARTESIAN_POINT('Ctrl Pts',(-85.132776765718,3.2410034219148,137.011947723114));
#210566=CARTESIAN_POINT('Ctrl Pts',(-85.4112243895309,6.97446035535538,
131.432965108015));
#210567=CARTESIAN_POINT('Ctrl Pts',(-85.6896720133437,4.29872894355427,
125.27632567523));
#210568=CARTESIAN_POINT('Ctrl Pts',(-85.9681196371569,-2.327324362789,124.19968029493));
#210569=CARTESIAN_POINT('Ctrl Pts',(-86.2465672609694,-6.81468027584547,
129.192413474561));
#210570=CARTESIAN_POINT('Ctrl Pts',(-86.5250148847825,-5.03967793103904,
135.666447330617));
#210571=CARTESIAN_POINT('Ctrl Pts',(-86.8034625085954,1.36654223043768,
137.672461023519));
#210572=CARTESIAN_POINT('Ctrl Pts',(-87.0819101324082,6.51697684144191,
133.367025968708));
#210573=CARTESIAN_POINT('Ctrl Pts',(-87.3603577562212,5.67862810717874,
126.706626649358));
#210574=CARTESIAN_POINT('Ctrl Pts',(-87.638805380034,-0.378102441176264,
123.811844661359));
#210575=CARTESIAN_POINT('Ctrl Pts',(-87.917253003847,-6.08737531742114,
127.342843233717));
#210576=CARTESIAN_POINT('Ctrl Pts',(-88.1957006276599,-6.20264766177327,
134.054807177307));
#210577=CARTESIAN_POINT('Ctrl Pts',(-88.4741482514726,-0.617989821139493,
137.779769525637));
#210578=CARTESIAN_POINT('Ctrl Pts',(-88.7525958752857,5.53457047463998,
135.094671855119));
#210579=CARTESIAN_POINT('Ctrl Pts',(-89.0310434990984,6.6011308830247,128.466987750645));
#210580=CARTESIAN_POINT('Ctrl Pts',(-89.3094911229114,1.60157449308101,
123.987235123859));
#210581=CARTESIAN_POINT('Ctrl Pts',(-89.5879387467241,-4.86975061474005,
125.772087790693));
#210582=CARTESIAN_POINT('Ctrl Pts',(-89.8663863705374,-6.8660128081587,
132.181353345229));
#210583=CARTESIAN_POINT('Ctrl Pts',(-90.1448339943499,-2.55274465425183,
137.325229852876));
#210584=CARTESIAN_POINT('Ctrl Pts',(-90.4232816181632,4.10637112840284,
136.476746095445));
#210585=CARTESIAN_POINT('Ctrl Pts',(-90.7017292419757,6.99193245143733,
130.415617195278));
#210586=CARTESIAN_POINT('Ctrl Pts',(-90.9801768657889,3.45224942649073,
124.711724509022));
#210587=CARTESIAN_POINT('Ctrl Pts',(-91.2586244896016,-3.2598821696406,
124.606666764696));
#210588=CARTESIAN_POINT('Ctrl Pts',(-91.5370721134145,-6.97634130596949,
130.196986896981));
#210589=CARTESIAN_POINT('Ctrl Pts',(-91.8155197372274,-4.28188359533257,
136.345453806627));
#210590=CARTESIAN_POINT('Ctrl Pts',(-92.0939673610402,2.34741595777304,
137.401926772977));
#210591=CARTESIAN_POINT('Ctrl Pts',(-92.3724149848533,6.81955492332935,
132.395558751529));
#210592=CARTESIAN_POINT('Ctrl Pts',(-92.650862608666,5.02485606812542,125.926957379319));
#210593=CARTESIAN_POINT('Ctrl Pts',(-92.929310232479,-1.38744003581995,
123.940451308663));
#210594=CARTESIAN_POINT('Ctrl Pts',(-93.2077578562919,-6.52474652706058,
128.261542572277));
#210595=CARTESIAN_POINT('Ctrl Pts',(-93.4862054801047,-5.66612971152105,
134.919359395943));
#210596=CARTESIAN_POINT('Ctrl Pts',(-93.7646531039176,0.39938350308132,
137.795693371147));
#210597=CARTESIAN_POINT('Ctrl Pts',(-94.0431007277306,6.09788278932073,
134.247334091402));
#210598=CARTESIAN_POINT('Ctrl Pts',(-94.3215483515434,6.19272569030992,
127.535050387806));
#210599=CARTESIAN_POINT('Ctrl Pts',(-94.5999959753563,0.596756213373149,
123.827103070676));
#210600=CARTESIAN_POINT('Ctrl Pts',(-94.8784435991693,-5.54760307049237,
126.530914581157));
#210601=CARTESIAN_POINT('Ctrl Pts',(-95.1568912229821,-6.59398614805128,
133.161814229653));
#210602=CARTESIAN_POINT('Ctrl Pts',(-95.4353388467949,-1.58081808968337,
137.626329176652));
#210603=CARTESIAN_POINT('Ctrl Pts',(-95.7137864706081,4.88504456584684,
135.821788289543));
#210604=CARTESIAN_POINT('Ctrl Pts',(-95.9922340944205,6.86178991305786,
129.406476486855));
#210605=CARTESIAN_POINT('Ctrl Pts',(-96.2706817182339,2.53288554724217,
124.275751909854));
#210606=CARTESIAN_POINT('Ctrl Pts',(-96.5491293420464,-4.12361689815126,
125.144499794972));
#210607=CARTESIAN_POINT('Ctrl Pts',(-96.8275769658595,-6.99071686402826,
131.214383276482));
#210608=CARTESIAN_POINT('Ctrl Pts',(-97.1060245896722,-3.4336895473684,
136.907475965166));
#210609=CARTESIAN_POINT('Ctrl Pts',(-97.3844722134854,3.27873071826322,
136.992103803166));
#210610=CARTESIAN_POINT('Ctrl Pts',(-97.6629198372979,6.9781576287114,131.390497941658));
#210611=CARTESIAN_POINT('Ctrl Pts',(-97.9413674611112,4.26499858032525,
125.250260513709));
#210612=CARTESIAN_POINT('Ctrl Pts',(-98.2198150849237,-2.36748580661544,
124.21396974833));
#210613=CARTESIAN_POINT('Ctrl Pts',(-98.498262708737,-6.82436639538843,
129.233926233285));
#210614=CARTESIAN_POINT('Ctrl Pts',(-98.7767103325495,-5.00998765563179,
135.69703519741));
#210615=CARTESIAN_POINT('Ctrl Pts',(-99.0551579563628,1.40832498814648,
137.664015243098));
#210616=CARTESIAN_POINT('Ctrl Pts',(-99.3336055801754,6.53245576831905,
133.327307800681));
#210617=CARTESIAN_POINT('Ctrl Pts',(-99.6120532039884,5.65357882561176,
126.672135149802));
#210618=CARTESIAN_POINT('Ctrl Pts',(-99.8905008278013,-0.420660865152761,
123.814275833361));
#210619=CARTESIAN_POINT('Ctrl Pts',(-100.168948451614,-6.10833377126732,
127.379962948978));
#210620=CARTESIAN_POINT('Ctrl Pts',(-100.447396075427,-6.18274635028192,
134.092504230901));
#210621=CARTESIAN_POINT('Ctrl Pts',(-100.72584369924,-0.575517077338011,
137.783402166914));
#210622=CARTESIAN_POINT('Ctrl Pts',(-101.004291323053,5.56058427410689,
135.060901864211));
#210623=CARTESIAN_POINT('Ctrl Pts',(-101.282738946866,6.58678032729173,
128.426848099441));
#210624=CARTESIAN_POINT('Ctrl Pts',(-101.561186570679,1.56004704180311,
123.977612190885));
#210625=CARTESIAN_POINT('Ctrl Pts',(-101.839634194492,-4.90029326256724,
125.801824581246));
#210626=CARTESIAN_POINT('Ctrl Pts',(-102.118081818304,-6.85750345127332,
132.223123201514));
#210627=CARTESIAN_POINT('Ctrl Pts',(-102.396529442117,-2.51300297592632,
137.340648317539));
#210628=CARTESIAN_POINT('Ctrl Pts',(-102.67497706593,4.14082446727623,136.451644352694));
#210629=CARTESIAN_POINT('Ctrl Pts',(-102.953424689743,6.98943651557314,
130.373062520413));
#210630=CARTESIAN_POINT('Ctrl Pts',(-103.231872313556,3.41509785901489,
124.690822569333));
#210631=CARTESIAN_POINT('Ctrl Pts',(-103.510319937369,-3.29754889317273,
124.626625421641));
#210632=CARTESIAN_POINT('Ctrl Pts',(-103.788767561182,-6.97990930675369,
130.239465119861));
#210633=CARTESIAN_POINT('Ctrl Pts',(-104.067215184995,-4.24807405495459,
136.371416183792));
#210634=CARTESIAN_POINT('Ctrl Pts',(-104.345662808808,2.38753372339306,
137.387515148146));
#210635=CARTESIAN_POINT('Ctrl Pts',(-104.62411043262,6.82911464744894,132.354016703874));
#210636=CARTESIAN_POINT('Ctrl Pts',(-104.902558056433,4.99507283129728,
125.896460021193));
#210637=CARTESIAN_POINT('Ctrl Pts',(-105.181005680246,-1.42919689394351,
123.949024222305));
#210638=CARTESIAN_POINT('Ctrl Pts',(-105.459453304059,-6.54010449379936,
128.301307668861));
#210639=CARTESIAN_POINT('Ctrl Pts',(-105.737900927872,-5.64097556572054,
134.953774494342));
#210640=CARTESIAN_POINT('Ctrl Pts',(-106.016348551685,0.441934330278796,
137.793132677202));
#210641=CARTESIAN_POINT('Ctrl Pts',(-106.294796175498,6.11872816644418,
134.210150757753));
#210642=CARTESIAN_POINT('Ctrl Pts',(-106.573243799311,6.17270973413615,
127.49741408157));
#210643=CARTESIAN_POINT('Ctrl Pts',(-106.851691423124,0.554272609792058,
123.823599718647));
#210644=CARTESIAN_POINT('Ctrl Pts',(-107.130139046936,-5.57351396522919,
126.564763592701));
#210645=CARTESIAN_POINT('Ctrl Pts',(-107.40858667075,-6.57951348749827,
133.201910016778));
#210646=CARTESIAN_POINT('Ctrl Pts',(-107.687034294562,-1.53926154185996,
137.635825669776));
#210647=CARTESIAN_POINT('Ctrl Pts',(-107.965481918375,4.91549656364115,
135.791958675416));
#210648=CARTESIAN_POINT('Ctrl Pts',(-108.243929542188,6.85315346251289,
129.364732723601));
#210649=CARTESIAN_POINT('Ctrl Pts',(-108.522377166001,2.49309712449469,
124.260454476607));
#210650=CARTESIAN_POINT('Ctrl Pts',(-108.800824789814,-4.15799367636883,
125.169706285567));
#210651=CARTESIAN_POINT('Ctrl Pts',(-109.079272413627,-6.98809141793296,
131.256930157466));
#210652=CARTESIAN_POINT('Ctrl Pts',(-109.35772003744,-3.39647453366164,
136.928264731447));
#210653=CARTESIAN_POINT('Ctrl Pts',(-109.636167661252,3.31633652003941,
136.97203059412));
#210654=CARTESIAN_POINT('Ctrl Pts',(-109.914615285065,6.98159632387027,
131.348009055767));
#210655=CARTESIAN_POINT('Ctrl Pts',(-110.193062908878,4.23111017600536,
125.22440116141));
#210656=CARTESIAN_POINT('Ctrl Pts',(-110.471510532691,-2.40755952238467,
124.228503411086));
#210657=CARTESIAN_POINT('Ctrl Pts',(-110.749958156504,-6.83379963552497,
129.275497185033));
#210658=CARTESIAN_POINT('Ctrl Pts',(-111.028405780317,-4.98011173328953,
135.727441764346));
#210659=CARTESIAN_POINT('Ctrl Pts',(-111.30685340413,1.45005555985492,137.655315275653));
#210660=CARTESIAN_POINT('Ctrl Pts',(-111.585301027943,6.54769263264538,
133.287496143919));
#210661=CARTESIAN_POINT('Ctrl Pts',(-111.863748651756,5.62832004860235,
126.63779677138));
#210662=CARTESIAN_POINT('Ctrl Pts',(-112.142196275568,-0.463203701385527,
123.816966025527));
#210663=CARTESIAN_POINT('Ctrl Pts',(-112.420643899382,-6.12906587855929,
127.417209556553));
#210664=CARTESIAN_POINT('Ctrl Pts',(-112.699091523194,-6.16261593485082,
134.130079441122));
#210665=CARTESIAN_POINT('Ctrl Pts',(-112.977539147007,-0.533023007539609,
137.786776197239));
#210666=CARTESIAN_POINT('Ctrl Pts',(-113.25598677082,5.58639202407863,135.026974145601));
#210667=CARTESIAN_POINT('Ctrl Pts',(-113.534434394633,6.57218569599142,
128.386796547837));
#210668=CARTESIAN_POINT('Ctrl Pts',(-113.812882018446,1.5184617824084,123.968242225583));
#210669=CARTESIAN_POINT('Ctrl Pts',(-114.091329642259,-4.93065432822552,
125.831746742611));
#210670=CARTESIAN_POINT('Ctrl Pts',(-114.369777266072,-6.84873998707567,
132.26484048503));
#210671=CARTESIAN_POINT('Ctrl Pts',(-114.648224889884,-2.4731681773514,
137.355824577657));
#210672=CARTESIAN_POINT('Ctrl Pts',(-114.926672513697,4.17512436637621,
136.426333347767));
#210673=CARTESIAN_POINT('Ctrl Pts',(-115.20512013751,6.98668158356849,130.330523827459));
#210674=CARTESIAN_POINT('Ctrl Pts',(-115.483567761323,3.377819743832,124.670147169045));
#210675=CARTESIAN_POINT('Ctrl Pts',(-115.762015385136,-3.33509342481799,
124.646812996834));
#210676=CARTESIAN_POINT('Ctrl Pts',(-116.040463008949,-6.98321866443162,
130.281964275151));
#210677=CARTESIAN_POINT('Ctrl Pts',(-116.318910632762,-4.21410710063033,
136.397172271667));
#210678=CARTESIAN_POINT('Ctrl Pts',(-116.597358256575,2.42756301807353,
137.372859582102));
#210679=CARTESIAN_POINT('Ctrl Pts',(-116.875805880388,6.83842131621399,
132.312417233142));
#210680=CARTESIAN_POINT('Ctrl Pts',(-117.154253504201,4.96510450020791,
125.866144527128));
#210681=CARTESIAN_POINT('Ctrl Pts',(-117.432701128013,-1.47090079265054,
123.957851162959));
#210682=CARTESIAN_POINT('Ctrl Pts',(-117.711148751826,-6.55522011456102,
128.341165516992));
#210683=CARTESIAN_POINT('Ctrl Pts',(-117.989596375639,-5.61561239149597,
134.988035834682));
#210684=CARTESIAN_POINT('Ctrl Pts',(-118.268043999452,0.484468781437156,
137.790313011739));
#210685=CARTESIAN_POINT('Ctrl Pts',(-118.546491623265,6.13934681184524,
134.172841221298));
#210686=CARTESIAN_POINT('Ctrl Pts',(-118.824939247078,6.15246504593319,
127.459900315453));
#210687=CARTESIAN_POINT('Ctrl Pts',(-119.103386870891,0.511768467435545,
123.820355041281));
#210688=CARTESIAN_POINT('Ctrl Pts',(-119.381834494704,-5.59921833135585,
126.598769704074));
#210689=CARTESIAN_POINT('Ctrl Pts',(-119.660282118516,-6.56479702065358,
133.241916961827));
#210690=CARTESIAN_POINT('Ctrl Pts',(-119.93872974233,-1.49764795613459,
137.645069020452));
#210691=CARTESIAN_POINT('Ctrl Pts',(-120.217177366142,4.94576641590264,
135.761944244007));
#210692=CARTESIAN_POINT('Ctrl Pts',(-120.495624989955,6.84426306584611,
129.323042306287));
#210693=CARTESIAN_POINT('Ctrl Pts',(-120.774072613768,2.45321631911644,
124.245399530209));
#210694=CARTESIAN_POINT('Ctrl Pts',(-121.052520237581,-4.19221637860163,
125.195121570349));
#210695=CARTESIAN_POINT('Ctrl Pts',(-121.330967861394,-6.98520702554029,
131.299460268319));
#210696=CARTESIAN_POINT('Ctrl Pts',(-121.609415485207,-3.35913366234199,
136.948826574209));
#210697=CARTESIAN_POINT('Ctrl Pts',(-121.88786310902,3.3538194337463,136.951728839794));
#210698=CARTESIAN_POINT('Ctrl Pts',(-122.166310732833,6.98477631340985,
131.305500024783));
#210699=CARTESIAN_POINT('Ctrl Pts',(-122.444758356646,4.19706498634193,
125.198748576561));
#210700=CARTESIAN_POINT('Ctrl Pts',(-122.723205980458,-2.44754402515043,
124.24328074465));
#210701=CARTESIAN_POINT('Ctrl Pts',(-123.001653604271,-6.84297964670285,
129.317124789377));
#210702=CARTESIAN_POINT('Ctrl Pts',(-123.280101228084,-4.95005127107555,
135.7576659047));
#210703=CARTESIAN_POINT('Ctrl Pts',(-123.558548851897,1.49173239922134,
137.646361443563));
#210704=CARTESIAN_POINT('Ctrl Pts',(-123.83699647571,6.5626868698133,133.247592473656));
#210705=CARTESIAN_POINT('Ctrl Pts',(-124.115444099523,5.60285271212367,
126.603612786514));
#210706=CARTESIAN_POINT('Ctrl Pts',(-124.393891723336,-0.505729373435472,
123.819915138168));
#210707=CARTESIAN_POINT('Ctrl Pts',(-124.672339347149,-6.14957087106115,
127.454581676257));
#210708=CARTESIAN_POINT('Ctrl Pts',(-124.950786970961,-6.14225716141998,
134.167531415611));
#210709=CARTESIAN_POINT('Ctrl Pts',(-125.229234594775,-0.490509186377616,
137.789891491587));
#210710=CARTESIAN_POINT('Ctrl Pts',(-125.507682218587,5.6119927682395,134.992889956494));
#210711=CARTESIAN_POINT('Ctrl Pts',(-125.786129842401,6.55734752993325,
128.346834579959));
#210712=CARTESIAN_POINT('Ctrl Pts',(-126.064577466213,1.47682025585389,
123.959125575163));
#210713=CARTESIAN_POINT('Ctrl Pts',(-126.343025090026,-4.9608326866744,
125.861853166013));
#210714=CARTESIAN_POINT('Ctrl Pts',(-126.621472713839,-6.8397227402992,
132.306503649927));
#210715=CARTESIAN_POINT('Ctrl Pts',(-126.899920337652,-2.43324173462049,
137.370758070868));
#210716=CARTESIAN_POINT('Ctrl Pts',(-127.178367961465,4.20926955470684,
136.400814018573));
#210717=CARTESIAN_POINT('Ctrl Pts',(-127.456815585278,6.98366775750873,
130.288002692701));
#210718=CARTESIAN_POINT('Ctrl Pts',(-127.73526320909,3.34041646229627,124.649699074291));
#210719=CARTESIAN_POINT('Ctrl Pts',(-128.013710832904,-3.37251437334987,
124.66722874222));
#210720=CARTESIAN_POINT('Ctrl Pts',(-128.292158456716,-6.9862692563739,
130.324482788031));
#210721=CARTESIAN_POINT('Ctrl Pts',(-128.570606080529,-4.17998399101771,
136.422721115849));
#210722=CARTESIAN_POINT('Ctrl Pts',(-128.849053704342,2.46750235851359,
137.357960617914));
#210723=CARTESIAN_POINT('Ctrl Pts',(-129.127501328155,6.84747458476236,
132.270761880817));
#210724=CARTESIAN_POINT('Ctrl Pts',(-129.405948951968,4.93495218534535,
125.836012020477));
#210725=CARTESIAN_POINT('Ctrl Pts',(-129.684396575781,-1.51255018658779,
123.966931803538));
#210726=CARTESIAN_POINT('Ctrl Pts',(-129.962844199593,-6.57009282923063,
128.381114639724));
#210727=CARTESIAN_POINT('Ctrl Pts',(-130.241291823406,-5.59004112868908,
135.022142147398));
#210728=CARTESIAN_POINT('Ctrl Pts',(-130.519739447219,0.52698528042665,
137.78723447924));
#210729=CARTESIAN_POINT('Ctrl Pts',(-130.798187071032,6.15973796149245,
134.135406864555));
#210730=CARTESIAN_POINT('Ctrl Pts',(-131.076634694845,6.13199237587537,
127.422510479544));
#210731=CARTESIAN_POINT('Ctrl Pts',(-131.355082318658,0.4692453613103,123.81736915881));
#210732=CARTESIAN_POINT('Ctrl Pts',(-131.633529942471,-5.62471521638866,
126.632931655165));
#210733=CARTESIAN_POINT('Ctrl Pts',(-131.911977566284,-6.54983729284086,
133.281833582332));
#210734=CARTESIAN_POINT('Ctrl Pts',(-132.190425190097,-1.45597887451291,
137.654058886162));
#210735=CARTESIAN_POINT('Ctrl Pts',(-132.46887281391,4.97585300097076,135.731746107516));
#210736=CARTESIAN_POINT('Ctrl Pts',(-132.747320437723,6.83511905249447,
129.281406779768));
#210737=CARTESIAN_POINT('Ctrl Pts',(-133.025768061535,2.4132446089053,124.230587628526));
#210738=CARTESIAN_POINT('Ctrl Pts',(-133.304215685348,-4.22628373671482,
125.220744707546));
#210739=CARTESIAN_POINT('Ctrl Pts',(-133.582663309161,-6.98206379373247,
131.341972033073));
#210740=CARTESIAN_POINT('Ctrl Pts',(-133.861110932974,-3.32166831708915,
136.969160731525));
#210741=CARTESIAN_POINT('Ctrl Pts',(-134.139558556787,3.39117807044069,
136.931199292478));
#210742=CARTESIAN_POINT('Ctrl Pts',(-134.4180061806,6.98769747949419,131.262972423894));
#210743=CARTESIAN_POINT('Ctrl Pts',(-134.696453804413,4.16286427289247,
125.173303709728));
#210744=CARTESIAN_POINT('Ctrl Pts',(-134.974901428226,-2.48743783327188,
124.25830120144));
#210745=CARTESIAN_POINT('Ctrl Pts',(-135.253349052039,-6.85190608875344,
129.358807503792));
#210746=CARTESIAN_POINT('Ctrl Pts',(-135.531796675851,-4.91980738289134,
135.787706498505));
#210747=CARTESIAN_POINT('Ctrl Pts',(-135.810244299665,1.53335396189511,
137.637154078616));
#210748=CARTESIAN_POINT('Ctrl Pts',(-136.088691923477,6.57743792420584,
133.207598268539));
#210749=CARTESIAN_POINT('Ctrl Pts',(-136.36713954729,5.57717775987727,126.569584461903));
#210750=CARTESIAN_POINT('Ctrl Pts',(-136.645587171103,-0.548236305497475,
123.823123062006));
#210751=CARTESIAN_POINT('Ctrl Pts',(-136.924034794916,-6.1698479889529,
127.492077923251));
#210752=CARTESIAN_POINT('Ctrl Pts',(-137.202482418729,-6.12167078439119,
134.204858766568));
#210753=CARTESIAN_POINT('Ctrl Pts',(-137.480930042542,-0.447977189217358,
137.792747934521));
#210754=CARTESIAN_POINT('Ctrl Pts',(-137.759377666354,5.63738555794455,
134.958650559891));
#210755=CARTESIAN_POINT('Ctrl Pts',(-138.037825290167,6.54226637895086,
128.306963676612));
#210756=CARTESIAN_POINT('Ctrl Pts',(-138.31627291398,1.43512400518173,123.950262577445));
#210757=CARTESIAN_POINT('Ctrl Pts',(-138.594720537793,-4.99082721964375,
125.892142735845));
#210758=CARTESIAN_POINT('Ctrl Pts',(-138.873168161606,-6.83045204508126,
132.348111152362));
#210759=CARTESIAN_POINT('Ctrl Pts',(-139.151615785419,-2.39322512722196,
137.385448243807));
#210760=CARTESIAN_POINT('Ctrl Pts',(-139.430063409232,4.24325876700673,
136.375087310741));
#210761=CARTESIAN_POINT('Ctrl Pts',(-139.708511033045,6.98039514907165,
130.245500691775));
#210762=CARTESIAN_POINT('Ctrl Pts',(-139.986958656858,3.30288940040013,
124.629479042785));
#210763=CARTESIAN_POINT('Ctrl Pts',(-140.26540628067,-3.40981035212143,
124.687871901284));
#210764=CARTESIAN_POINT('Ctrl Pts',(-140.543853904484,-6.98906096953965,
130.36701908296));
#210765=CARTESIAN_POINT('Ctrl Pts',(-140.822301528296,-4.1457059905611,
136.448061769617));
#210766=CARTESIAN_POINT('Ctrl Pts',(-141.100749152109,2.50735026474636,
137.342818807668));
#210767=CARTESIAN_POINT('Ctrl Pts',(-141.379196775922,6.85627411762182,
132.229052190456));
#210768=CARTESIAN_POINT('Ctrl Pts',(-141.657644399735,4.90461700401472,
125.80606361781));
#210769=CARTESIAN_POINT('Ctrl Pts',(-141.936092023548,-1.5541435324211,
123.976265807557));
#210770=CARTESIAN_POINT('Ctrl Pts',(-142.214539647361,-6.58472208669408,
128.421153556726));
#210771=CARTESIAN_POINT('Ctrl Pts',(-142.492987271174,-5.56426272485295,
135.056092168669));
#210772=CARTESIAN_POINT('Ctrl Pts',(-142.771434894987,0.569482251782813,
137.783897193782));
#210773=CARTESIAN_POINT('Ctrl Pts',(-143.0498825188,6.17990085978423,134.097849074668));
#210774=CARTESIAN_POINT('Ctrl Pts',(-143.328330142612,6.11129248258502,
127.385245959334));
#210775=CARTESIAN_POINT('Ctrl Pts',(-143.606777766425,0.426704867125613,
123.814642181877));
#210776=CARTESIAN_POINT('Ctrl Pts',(-143.885225390238,-5.65000367553061,
126.667248180088));
#210777=CARTESIAN_POINT('Ctrl Pts',(-144.163673014051,-6.53463485839856,
133.321658399163));
#210778=CARTESIAN_POINT('Ctrl Pts',(-144.442120637864,-1.4142558410586,
137.662794933783));
#210779=CARTESIAN_POINT('Ctrl Pts',(-144.720568261677,5.00575520397605,
135.701365384942));
#210780=CARTESIAN_POINT('Ctrl Pts',(-144.99901588549,6.82572176129271,129.239827686864));
#210781=CARTESIAN_POINT('Ctrl Pts',(-145.277463509303,2.37318347502772,
124.216019320419));
#210782=CARTESIAN_POINT('Ctrl Pts',(-145.555911133116,-4.26019448832994,
125.246574747685));
#210783=CARTESIAN_POINT('Ctrl Pts',(-145.834358756928,-6.97866183898313,
131.384463876438));
#210784=CARTESIAN_POINT('Ctrl Pts',(-146.112806380741,-3.28407988619528,
136.989266449907));
#210785=CARTESIAN_POINT('Ctrl Pts',(-146.391254004554,3.42841104578457,
136.910442712901));
#210786=CARTESIAN_POINT('Ctrl Pts',(-146.669701628367,6.99035971387901,
131.220427828976));
#210787=CARTESIAN_POINT('Ctrl Pts',(-146.94814925218,4.12850930297597,125.148067503779));
#210788=CARTESIAN_POINT('Ctrl Pts',(-147.226596875993,-2.52723946847004,
124.27356422487));
#210789=CARTESIAN_POINT('Ctrl Pts',(-147.505044499806,-6.86057863090408,
129.400543783708));
#210790=CARTESIAN_POINT('Ctrl Pts',(-147.783492123619,-4.88938118943532,
135.817562432597));
#210791=CARTESIAN_POINT('Ctrl Pts',(-148.061939747432,1.57491870557395,
137.627693521995));
#210792=CARTESIAN_POINT('Ctrl Pts',(-148.340387371245,6.5919452492172,133.167515010566));
#210793=CARTESIAN_POINT('Ctrl Pts',(-148.618834995057,5.55129614325799,
126.535713058481));
#210794=CARTESIAN_POINT('Ctrl Pts',(-148.89728261887,-0.590722922461593,
123.826589678167));
#210795=CARTESIAN_POINT('Ctrl Pts',(-149.175730242683,-6.18989648085842,
127.529696908099));
#210796=CARTESIAN_POINT('Ctrl Pts',(-149.454177866496,-6.10085756660025,
134.242060110815));
#210797=CARTESIAN_POINT('Ctrl Pts',(-149.732625490309,-0.405428592098244,
137.795345420191));
#210798=CARTESIAN_POINT('Ctrl Pts',(-150.011073114122,5.66256945225453,
134.924257224548));
#210799=CARTESIAN_POINT('Ctrl Pts',(-150.289520737935,6.52694280188189,
128.267185315226));
#210800=CARTESIAN_POINT('Ctrl Pts',(-150.567968361748,1.39337457546175,
123.94165356085));
#210801=CARTESIAN_POINT('Ctrl Pts',(-150.84641598556,-5.02063681567507,
125.922614329717));
#210802=CARTESIAN_POINT('Ctrl Pts',(-151.124863609373,-6.8209282449509,
132.389661450552));
#210803=CARTESIAN_POINT('Ctrl Pts',(-151.403311233186,-2.35311983798619,
137.399894552124));
#210804=CARTESIAN_POINT('Ctrl Pts',(-151.681758856999,4.2770907437925,136.349154177582));
#210805=CARTESIAN_POINT('Ctrl Pts',(-151.960206480812,6.97686387952531,
130.20301939961));
#210806=CARTESIAN_POINT('Ctrl Pts',(-152.238654104625,3.26523994872261,
124.609487823786));
#210807=CARTESIAN_POINT('Ctrl Pts',(-152.517101728438,-3.44697997911642,
124.708741709087));
#210808=CARTESIAN_POINT('Ctrl Pts',(-152.795549352251,-6.99159370048095,
130.40957158374));
#210809=CARTESIAN_POINT('Ctrl Pts',(-153.073996976064,-4.11127436944443,
136.473193293963));
#210810=CARTESIAN_POINT('Ctrl Pts',(-153.352444599876,2.54710526019297,
137.327434712448));
#210811=CARTESIAN_POINT('Ctrl Pts',(-153.63089222369,6.86481958872245,132.187289707623));
#210812=CARTESIAN_POINT('Ctrl Pts',(-153.909339847502,4.87410008029735,
125.776300428876));
#210813=CARTESIAN_POINT('Ctrl Pts',(-154.187787471315,-1.5956792888948,
123.98585282914));
#210814=CARTESIAN_POINT('Ctrl Pts',(-154.466235095128,-6.5991073448593,
128.461280784342));
#210815=CARTESIAN_POINT('Ctrl Pts',(-154.744682718941,-5.53827813521478,
135.089884640464));
#210816=CARTESIAN_POINT('Ctrl Pts',(-155.023130342754,0.611958120764675,
137.78030127903));
#210817=CARTESIAN_POINT('Ctrl Pts',(-155.301577966567,6.19983475957701,
134.060169243357));
#210818=CARTESIAN_POINT('Ctrl Pts',(-155.58002559038,6.0903661331043,127.348108135675));
#210819=CARTESIAN_POINT('Ctrl Pts',(-155.858473214192,0.38414856123516,
123.812174211531));
#210820=CARTESIAN_POINT('Ctrl Pts',(-156.136920838005,-5.67508277170857,
126.701718007236));
#210821=CARTESIAN_POINT('Ctrl Pts',(-156.415368461818,-6.51919028065846,
133.3613899366));
#210822=CARTESIAN_POINT('Ctrl Pts',(-156.693816085631,-1.37248040183399,
137.671276839599));
#210823=CARTESIAN_POINT('Ctrl Pts',(-156.972263709444,5.03547191688086,
135.670803202055));
#210824=CARTESIAN_POINT('Ctrl Pts',(-157.250711333257,6.81607154046107,
129.198306568304));
#210825=CARTESIAN_POINT('Ctrl Pts',(-157.52915895707,2.33303440196427,124.201695145721));
#210826=CARTESIAN_POINT('Ctrl Pts',(-157.807606580883,-4.29394737687161,
125.272610733624));
#210827=CARTESIAN_POINT('Ctrl Pts',(-158.086054204696,-6.97500128735293,
131.426934223863));
#210828=CARTESIAN_POINT('Ctrl Pts',(-158.364501828508,-3.2463697625135,
137.009142984327));
#210829=CARTESIAN_POINT('Ctrl Pts',(-158.642949452322,3.46551698009634,
136.889459870208));
#210830=CARTESIAN_POINT('Ctrl Pts',(-158.921397076134,6.99276291791392,
131.177867816534));
#210831=CARTESIAN_POINT('Ctrl Pts',(-159.199844699947,4.09400134962899,
125.123040893851));
#210832=CARTESIAN_POINT('Ctrl Pts',(-159.47829232376,-2.56694745588028,
124.289069249361));
#210833=CARTESIAN_POINT('Ctrl Pts',(-159.756739947573,-6.86899695179061,
129.442332082575));
#210834=CARTESIAN_POINT('Ctrl Pts',(-160.035187571386,-4.85877381816122,
135.84723260065));
#210835=CARTESIAN_POINT('Ctrl Pts',(-160.313635195198,1.61642509006095,
137.617980124263));
#210836=CARTESIAN_POINT('Ctrl Pts',(-160.592082819012,6.60620830727321,
133.12734418504));
#210837=CARTESIAN_POINT('Ctrl Pts',(-160.870530442824,5.52520882131862,
126.501999831362));
#210838=CARTESIAN_POINT('Ctrl Pts',(-161.148978066638,-0.633187649970563,
123.830314858198));
#210839=CARTESIAN_POINT('Ctrl Pts',(-161.42742569045,-6.20971560387352,
127.567437236815));
#210840=CARTESIAN_POINT('Ctrl Pts',(-161.705873314263,-6.07981827928859,
134.279134069845));
#210841=CARTESIAN_POINT('Ctrl Pts',(-161.984320938076,-0.362864971672915,
137.79768385235));
#210842=CARTESIAN_POINT('Ctrl Pts',(-162.262768561889,5.68754351797111,
134.889711224922));
#210843=CARTESIAN_POINT('Ctrl Pts',(-162.541216185702,6.5113773665471,128.227500969805));
#210844=CARTESIAN_POINT('Ctrl Pts',(-162.819663809515,1.35157351373451,
123.93329884439));
#210845=CARTESIAN_POINT('Ctrl Pts',(-163.098111433328,-5.05026037016286,
125.953266818493));
#210846=CARTESIAN_POINT('Ctrl Pts',(-163.376559057141,-6.81115169281603,
132.431153004838));
#210847=CARTESIAN_POINT('Ctrl Pts',(-163.655006680953,-2.31292735302948,
137.414096460505));
#210848=CARTESIAN_POINT('Ctrl Pts',(-163.933454304766,4.31076423140788,
136.323015580059));
#210849=CARTESIAN_POINT('Ctrl Pts',(-164.211901928579,6.97307407972212,
130.160560390364));
#210850=CARTESIAN_POINT('Ctrl Pts',(-164.490349552392,3.2274695023783,124.589726158078));
#210851=CARTESIAN_POINT('Ctrl Pts',(-164.768797176205,-3.4840218770001,
124.729837392289));
#210852=CARTESIAN_POINT('Ctrl Pts',(-165.047244800018,-6.99386735534677,
130.452138713572));
#210853=CARTESIAN_POINT('Ctrl Pts',(-165.325692423831,-4.07669040354407,
136.498114757629));
#210854=CARTESIAN_POINT('Ctrl Pts',(-165.604140047644,2.58676587171747,
137.31180890232));
#210855=CARTESIAN_POINT('Ctrl Pts',(-165.882587671457,6.87311068140868,
132.145475979844));
#210856=CARTESIAN_POINT('Ctrl Pts',(-166.161035295269,4.84340254500906,
125.746723556562));
#210857=CARTESIAN_POINT('Ctrl Pts',(-166.439482919082,-1.63715591688565,
123.995692513036));
#210858=CARTESIAN_POINT('Ctrl Pts',(-166.717930542895,-6.61324807067504,
128.501494835643));
#210859=CARTESIAN_POINT('Ctrl Pts',(-166.996378166708,-5.5120883226436,
135.12351831059));
#210860=CARTESIAN_POINT('Ctrl Pts',(-167.274825790521,0.654411313413328,
137.776446868231));
#210861=CARTESIAN_POINT('Ctrl Pts',(-167.553273414334,6.21953892221278,
134.022368766858));
#210862=CARTESIAN_POINT('Ctrl Pts',(-167.831721038147,6.06921410286677,
127.311098384725));
#210863=CARTESIAN_POINT('Ctrl Pts',(-168.11016866196,0.3415780205785,123.809965339223));
#210864=CARTESIAN_POINT('Ctrl Pts',(-168.388616285773,-5.69995157560742,
126.736339859314));
#210865=CARTESIAN_POINT('Ctrl Pts',(-168.667063909585,-6.50350413192509,
133.401026722375));
#210866=CARTESIAN_POINT('Ctrl Pts',(-168.945511533399,-1.33065410484337,
137.679504289309));
#210867=CARTESIAN_POINT('Ctrl Pts',(-169.223959157211,5.06500203852252,
135.640060691349));
#210868=CARTESIAN_POINT('Ctrl Pts',(-169.502406781024,6.80616874759175,
129.156844962666));
#210869=CARTESIAN_POINT('Ctrl Pts',(-169.780854404837,2.29279887745254,
124.18761563522));
#210870=CARTESIAN_POINT('Ctrl Pts',(-170.05930202865,-4.32754115161411,
125.298851700587));
#210871=CARTESIAN_POINT('Ctrl Pts',(-170.337749652463,-6.97108227448498,
131.469381501595));
#210872=CARTESIAN_POINT('Ctrl Pts',(-170.616197276276,-3.20853934340632,
137.028789598255));
#210873=CARTESIAN_POINT('Ctrl Pts',(-170.894644900089,3.50249449840198,
136.868251541923));
#210874=CARTESIAN_POINT('Ctrl Pts',(-171.173092523901,6.99490700254731,
131.135293963646));
#210875=CARTESIAN_POINT('Ctrl Pts',(-171.451540147715,4.05934169155642,
125.098224807315));
#210876=CARTESIAN_POINT('Ctrl Pts',(-171.729987771527,-2.60656032410858,
124.304815700371));
#210877=CARTESIAN_POINT('Ctrl Pts',(-172.00843539534,-6.87716073946864,
129.484170851909));
#210878=CARTESIAN_POINT('Ctrl Pts',(-172.286883019153,-4.82798640323697,
135.876715903229));
#210879=CARTESIAN_POINT('Ctrl Pts',(-172.565330642966,1.65787157732142,
137.608014245356));
#210880=CARTESIAN_POINT('Ctrl Pts',(-172.843778266779,6.62022656985093,
133.087087280501));
#210881=CARTESIAN_POINT('Ctrl Pts',(-173.122225890592,5.49891676073447,
126.468446029806));
#210882=CARTESIAN_POINT('Ctrl Pts',(-173.400673514405,-0.675628914478315,
123.834298464058));
#210883=CARTESIAN_POINT('Ctrl Pts',(-173.679121138218,-6.22930462359329,
127.605297510917));
#210884=CARTESIAN_POINT('Ctrl Pts',(-173.95756876203,-6.05855370207473,
134.316079269865));
#210885=CARTESIAN_POINT('Ctrl Pts',(-174.236016385844,-0.320287905152608,
137.799763144343));
#210886=CARTESIAN_POINT('Ctrl Pts',(-174.514464009656,5.71230682967103,
134.855013841124));
#210887=CARTESIAN_POINT('Ctrl Pts',(-174.792911633469,6.49557064972945,
128.187912110866));
#210888=CARTESIAN_POINT('Ctrl Pts',(-175.071359257282,1.30972236895365,
123.925198737649));
#210889=CARTESIAN_POINT('Ctrl Pts',(-175.349806881095,-5.07969678539539,
125.984099066334));
#210890=CARTESIAN_POINT('Ctrl Pts',(-175.628254504908,-6.80112275095037,
132.472584277733));
#210891=CARTESIAN_POINT('Ctrl Pts',(-175.906702128721,-2.27264916169912,
137.428053442694));
#210892=CARTESIAN_POINT('Ctrl Pts',(-176.185149752534,4.34427798206938,
136.296672486746));
#210893=CARTESIAN_POINT('Ctrl Pts',(-176.463597376347,6.96902589009458,
130.118125237372));
#210894=CARTESIAN_POINT('Ctrl Pts',(-176.742045000159,3.18957946096438,
124.570194777934));
#210895=CARTESIAN_POINT('Ctrl Pts',(-177.020492623972,-3.52093467317244,
124.751158169184));
#210896=CARTESIAN_POINT('Ctrl Pts',(-177.298940247785,-6.99588184988549,
130.494718895118));
#210897=CARTESIAN_POINT('Ctrl Pts',(-177.577387871598,-4.04195537438161,
136.522825237142));
#210898=CARTESIAN_POINT('Ctrl Pts',(-177.855835495411,2.62633062968132,
137.295941956302));
#210899=CARTESIAN_POINT('Ctrl Pts',(-178.134283119224,6.88114708845103,
132.103612556543));
#210900=CARTESIAN_POINT('Ctrl Pts',(-178.412730743037,4.81252553565828,
125.717334096849));
#210901=CARTESIAN_POINT('Ctrl Pts',(-178.69117836685,-1.67857187946192,
124.005784494632));
#210902=CARTESIAN_POINT('Ctrl Pts',(-178.969625990663,-6.62714374015151,
128.541794220484));
#210903=CARTESIAN_POINT('Ctrl Pts',(-179.248073614475,-5.48569425761253,
135.15699193274));
#210904=CARTESIAN_POINT('Ctrl Pts',(-179.526521238288,0.696840256609583,
137.772334104211));
#210905=CARTESIAN_POINT('Ctrl Pts',(-179.804968862101,6.23901261754625,
133.984449045885));
#210906=CARTESIAN_POINT('Ctrl Pts',(-180.083416485914,6.0478371756692,127.27421807789));
#210907=CARTESIAN_POINT('Ctrl Pts',(-180.361864109727,0.298994822622653,
123.808015646805));
#210908=CARTESIAN_POINT('Ctrl Pts',(-180.64031173354,-5.72460916570447,
126.771112453397));
#210909=CARTESIAN_POINT('Ctrl Pts',(-180.918759357353,-6.48757699345442,
133.440567287733));
#210910=CARTESIAN_POINT('Ctrl Pts',(-181.197206981166,-1.28877849997557,
137.687476978041));
#210911=CARTESIAN_POINT('Ctrl Pts',(-181.475654604978,5.094344474651,135.609138992));
#210912=CARTESIAN_POINT('Ctrl Pts',(-181.754102228792,6.79601374963652,
129.115444406326));
#210913=CARTESIAN_POINT('Ctrl Pts',(-182.032549852604,2.25247839243521,
124.173781310638));
#210914=CARTESIAN_POINT('Ctrl Pts',(-182.310997476417,-4.36097456772779,
125.32529667621));
#210915=CARTESIAN_POINT('Ctrl Pts',(-182.58944510023,-6.96690494559973,
131.511804136733));
#210916=CARTESIAN_POINT('Ctrl Pts',(-182.867892724043,-3.17059003069381,
137.048205563678));
#210917=CARTESIAN_POINT('Ctrl Pts',(-183.146340347856,3.53934223048593,
136.84681851393));
#210918=CARTESIAN_POINT('Ctrl Pts',(-183.424787971669,6.99679188832936,
131.092707847901));
#210919=CARTESIAN_POINT('Ctrl Pts',(-183.703235595482,4.02453161308464,
125.07362016374));
#210920=CARTESIAN_POINT('Ctrl Pts',(-183.981683219295,-2.64607660528548,
124.320802994409));
#210921=CARTESIAN_POINT('Ctrl Pts',(-184.260130843107,-6.88506969142675,
129.52605854136));
#210922=CARTESIAN_POINT('Ctrl Pts',(-184.53857846692,-4.79702008550057,
135.906011247817));
#210923=CARTESIAN_POINT('Ctrl Pts',(-184.817026090733,1.6992566315413,137.597796254561));
#210924=CARTESIAN_POINT('Ctrl Pts',(-185.095473714546,6.63399951749853,
133.046745788687));
#210925=CARTESIAN_POINT('Ctrl Pts',(-185.373921338359,5.47242093576752,
126.435052897159));
#210926=CARTESIAN_POINT('Ctrl Pts',(-185.652368962172,-0.718045143308166,
123.838540348135));
#210927=CARTESIAN_POINT('Ctrl Pts',(-185.930816585985,-6.24866281413942,
127.64327632748));
#210928=CARTESIAN_POINT('Ctrl Pts',(-186.209264209798,-6.03706462292539,
134.35289434186));
#210929=CARTESIAN_POINT('Ctrl Pts',(-186.487711833611,-0.277698970246197,
137.801583219124));
#210930=CARTESIAN_POINT('Ctrl Pts',(-186.766159457423,5.73685846974069,
134.820166358884));
#210931=CARTESIAN_POINT('Ctrl Pts',(-187.044607081237,6.47952323715255,
128.148420205389));
#210932=CARTESIAN_POINT('Ctrl Pts',(-187.323054705049,1.2678226919294,123.917353540782));
#210933=CARTESIAN_POINT('Ctrl Pts',(-187.601502328862,-5.10894497059535,
126.01510993074));
#210934=CARTESIAN_POINT('Ctrl Pts',(-187.879949952675,-6.79084179098006,
132.513953733987));
#210935=CARTESIAN_POINT('Ctrl Pts',(-188.158397576488,-2.23228675651833,
137.44176498151));
#210936=CARTESIAN_POINT('Ctrl Pts',(-188.436845200301,4.37763075391265,
136.270125873797));
#210937=CARTESIAN_POINT('Ctrl Pts',(-188.715292824114,6.96471946064982,
130.075715513085));
#210938=CARTESIAN_POINT('Ctrl Pts',(-188.993740447926,3.15157122851057,
124.550894407098));
#210939=CARTESIAN_POINT('Ctrl Pts',(-189.27218807174,-3.55771699981564,
124.772703249722));
#210940=CARTESIAN_POINT('Ctrl Pts',(-189.550635695553,-6.99763710944952,
130.53731055055));
#210941=CARTESIAN_POINT('Ctrl Pts',(-189.829083319365,-4.00707056907658,
136.547323816845));
#210942=CARTESIAN_POINT('Ctrl Pts',(-190.107530943179,2.66579806799723,
137.279834462351));
#210943=CARTESIAN_POINT('Ctrl Pts',(-190.385978566991,6.88892851205765,
132.061700988983));
#210944=CARTESIAN_POINT('Ctrl Pts',(-190.664426190804,4.78147019640398,
125.688133138775));
#210945=CARTESIAN_POINT('Ctrl Pts',(-190.942873814617,-1.71992564193992,
124.016128399968));
#210946=CARTESIAN_POINT('Ctrl Pts',(-191.22132143843,-6.64079383837953,
128.582177445553));
#210947=CARTESIAN_POINT('Ctrl Pts',(-191.499769062243,-5.45909691816341,
135.190304266535));
#210948=CARTESIAN_POINT('Ctrl Pts',(-191.778216686055,0.739243378134395,
137.767963139373));
#210949=CARTESIAN_POINT('Ctrl Pts',(-192.056664309869,6.25825512397307,
133.946411485565));
#210950=CARTESIAN_POINT('Ctrl Pts',(-192.335111933681,6.0262361436405,127.237468581785));
#210951=CARTESIAN_POINT('Ctrl Pts',(-192.613559557494,0.256400545303713,
123.806325206523));
#210952=CARTESIAN_POINT('Ctrl Pts',(-192.892007181307,-5.74905462830365,
126.806034500975));
#210953=CARTESIAN_POINT('Ctrl Pts',(-193.17045480512,-6.47140945543246,
133.480010167483));
#210954=CARTESIAN_POINT('Ctrl Pts',(-193.448902428933,-1.24685513894648,
137.695194610365));
#210955=CARTESIAN_POINT('Ctrl Pts',(-193.727350052746,5.12349813797151,
135.578039249819));
#210956=CARTESIAN_POINT('Ctrl Pts',(-194.005797676559,6.78560692289256,
129.074106433399));
#210957=CARTESIAN_POINT('Ctrl Pts',(-194.284245300372,2.2120744410027,124.160192684611));
#210958=CARTESIAN_POINT('Ctrl Pts',(-194.562692924184,-4.39424638632456,
125.35194468056));
#210959=CARTESIAN_POINT('Ctrl Pts',(-194.841140547997,-6.9624694554897,
131.554200557291));
#210960=CARTESIAN_POINT('Ctrl Pts',(-195.11958817181,-3.13252323060231,
137.067390161131));
#210961=CARTESIAN_POINT('Ctrl Pts',(-195.398035795623,3.57605881094196,
136.825161580438));
#210962=CARTESIAN_POINT('Ctrl Pts',(-195.676483419436,6.99841750541489,
131.050111047343));
#210963=CARTESIAN_POINT('Ctrl Pts',(-195.954931043249,3.98957240411393,
125.04922787486));
#210964=CARTESIAN_POINT('Ctrl Pts',(-196.233378667062,-2.68549483512068,
124.337030539057));
#210965=CARTESIAN_POINT('Ctrl Pts',(-196.511826290875,-6.89272351459547,
129.567993598765));
#210966=CARTESIAN_POINT('Ctrl Pts',(-196.790273914688,-4.76587601242081,
135.935117548864));
#210967=CARTESIAN_POINT('Ctrl Pts',(-197.0687215385,1.74057871918182,137.58732653051));
#210968=CARTESIAN_POINT('Ctrl Pts',(-197.347169162313,6.64752663985393,
133.006321204467));
#210969=CARTESIAN_POINT('Ctrl Pts',(-197.625616786126,5.44572232823074,
126.401821670817));
#210970=CARTESIAN_POINT('Ctrl Pts',(-197.904064409939,-0.760434764710735,
123.843040353244));
#210971=CARTESIAN_POINT('Ctrl Pts',(-198.182512033752,-6.26778945818702,
127.681372279183));
#210972=CARTESIAN_POINT('Ctrl Pts',(-198.460959657565,-6.01535183812634,
134.389577921633));
#210973=CARTESIAN_POINT('Ctrl Pts',(-198.739407281378,-0.235099745102313,
137.803144009248));
#210974=CARTESIAN_POINT('Ctrl Pts',(-199.017854905191,5.76119752841001,
134.785170069484));
#210975=CARTESIAN_POINT('Ctrl Pts',(-199.296302529004,6.46323572345932,
128.10902671676));
#210976=CARTESIAN_POINT('Ctrl Pts',(-199.574750152817,1.22587603526843,
123.909763544495));
#210977=CARTESIAN_POINT('Ctrl Pts',(-199.853197776629,-5.13800384196074,
126.04629826259));
#210978=CARTESIAN_POINT('Ctrl Pts',(-200.131645400443,-6.78030919386985,
132.555259840639));
#210979=CARTESIAN_POINT('Ctrl Pts',(-200.410093024255,-2.19184163313082,
137.455230568865));
#210980=CARTESIAN_POINT('Ctrl Pts',(-200.688540648069,4.41082131103843,
136.243376724908));
#210981=CARTESIAN_POINT('Ctrl Pts',(-200.96698827188,6.96015495096418,130.03333278901));
#210982=CARTESIAN_POINT('Ctrl Pts',(-201.245435895694,3.11344621342587,
124.531825760752));
#210983=CARTESIAN_POINT('Ctrl Pts',(-201.523883519507,-3.59436749394705,
124.794471835542));
#210984=CARTESIAN_POINT('Ctrl Pts',(-201.80233114332,-6.99913306899709,
130.579912101622));
#210985=CARTESIAN_POINT('Ctrl Pts',(-202.080778767133,-3.97203728029775,
136.571609588935));
#210986=CARTESIAN_POINT('Ctrl Pts',(-202.359226390945,2.705166724186,137.263487017335));
#210987=CARTESIAN_POINT('Ctrl Pts',(-202.637674014758,6.89645466388467,
132.019742830214));
#210988=CARTESIAN_POINT('Ctrl Pts',(-202.916121638571,4.75023767801316,
125.659121764391));
#210989=CARTESIAN_POINT('Ctrl Pts',(-203.194569262384,-1.76121567194074,
124.026723845744));
#210990=CARTESIAN_POINT('Ctrl Pts',(-203.473016886197,-6.65419785954973,
128.622643014438));
#210991=CARTESIAN_POINT('Ctrl Pts',(-203.75146451001,-5.43229728987039,
135.223454077576));
#210992=CARTESIAN_POINT('Ctrl Pts',(-204.029912133822,0.781619106723946,
137.763334135682));
#210993=CARTESIAN_POINT('Ctrl Pts',(-204.308359757636,6.27726572845484,
133.908257495395));
#210994=CARTESIAN_POINT('Ctrl Pts',(-204.586807381448,6.00441180721532,
127.200851258176));
#210995=CARTESIAN_POINT('Ctrl Pts',(-204.865255005262,0.213796766968775,
123.804894081017));
#210996=CARTESIAN_POINT('Ctrl Pts',(-205.143702629074,-5.77328705756903,
126.841104707996));
#210997=CARTESIAN_POINT('Ctrl Pts',(-205.422150252887,-6.4550021169537,
133.519353900054));
#210998=CARTESIAN_POINT('Ctrl Pts',(-205.7005978767,-1.20488557524167,137.702656900301));
#210999=CARTESIAN_POINT('Ctrl Pts',(-205.979045500513,5.15246194818434,
135.546762617222));
#211000=CARTESIAN_POINT('Ctrl Pts',(-206.257493124326,6.77494865298866,
129.032832575676));
#211001=CARTESIAN_POINT('Ctrl Pts',(-206.535940748139,2.17158852033829,
124.14685026067));
#211002=CARTESIAN_POINT('Ctrl Pts',(-206.814388371952,-4.42735537450605,
125.378794726189));
#211003=CARTESIAN_POINT('Ctrl Pts',(-207.092835995765,-6.9577759685135,
131.596569192254));
#211004=CARTESIAN_POINT('Ctrl Pts',(-207.371283619578,-3.09434035370993,
137.086342679721));
#211005=CARTESIAN_POINT('Ctrl Pts',(-207.64973124339,3.61264287922363,136.803281543952));
#211006=CARTESIAN_POINT('Ctrl Pts',(-207.928178867203,6.99978379356611,
131.007505140413));
#211007=CARTESIAN_POINT('Ctrl Pts',(-208.206626491016,3.95446536007061,
125.025048844539));
#211008=CARTESIAN_POINT('Ctrl Pts',(-208.485074114829,-2.72481355295718,
124.353497733001));
#211009=CARTESIAN_POINT('Ctrl Pts',(-208.763521738642,-6.90012192535954,
129.609974470206));
#211010=CARTESIAN_POINT('Ctrl Pts',(-209.041969362455,-4.73455533805275,
135.964033727826));
#211011=CARTESIAN_POINT('Ctrl Pts',(-209.320416986268,1.78183630903778,
137.576605461163));
#211012=CARTESIAN_POINT('Ctrl Pts',(-209.598864610081,6.66080743566547,
132.965815025787));
#211013=CARTESIAN_POINT('Ctrl Pts',(-209.877312233893,5.41882192745001,
126.368753582173));
#211014=CARTESIAN_POINT('Ctrl Pts',(-210.155759857706,-0.802796207923886,
123.847798312635));
#211015=CARTESIAN_POINT('Ctrl Pts',(-210.434207481519,-6.28668384699127,
127.719583954367));
#211016=CARTESIAN_POINT('Ctrl Pts',(-210.712655105332,-5.99341615225276,
134.42612864986));
#211017=CARTESIAN_POINT('Ctrl Pts',(-210.991102729145,-0.19249180825093,
137.804445456879));
#211018=CARTESIAN_POINT('Ctrl Pts',(-211.269550352958,5.78532310378624,
134.750026269725));
#211019=CARTESIAN_POINT('Ctrl Pts',(-211.547997976771,6.44670871218949,
128.069733104719));
#211020=CARTESIAN_POINT('Ctrl Pts',(-211.826445600584,1.18388395332015,
123.902429030038));
#211021=CARTESIAN_POINT('Ctrl Pts',(-212.104893224396,-5.16687232270428,
126.077662906191));
#211022=CARTESIAN_POINT('Ctrl Pts',(-212.38334084821,-6.76952534990887,
132.596501067076));
#211023=CARTESIAN_POINT('Ctrl Pts',(-212.661788472022,-2.15131529024619,
137.468449705789));
#211024=CARTESIAN_POINT('Ctrl Pts',(-212.940236095835,4.44384842355829,
136.216426031276));
#211025=CARTESIAN_POINT('Ctrl Pts',(-213.218683719648,6.95533253017721,
129.990978635656));
#211026=CARTESIAN_POINT('Ctrl Pts',(-213.497131343461,3.0752058284468,124.512989545492));
#211027=CARTESIAN_POINT('Ctrl Pts',(-213.775578967274,-3.63088479746918,
124.81646312));
#211028=CARTESIAN_POINT('Ctrl Pts',(-214.054026591087,-7.00036967309483,
130.622521969716));
#211029=CARTESIAN_POINT('Ctrl Pts',(-214.3324742149,-3.93685680621679,136.595681653493));
#211030=CARTESIAN_POINT('Ctrl Pts',(-214.610921838713,2.74443513942699,
137.246900227015));
#211031=CARTESIAN_POINT('Ctrl Pts',(-214.889369462525,6.90372526504794,
131.977739635008));
#211032=CARTESIAN_POINT('Ctrl Pts',(-215.167817086339,4.71882913781829,
125.630301048724));
#211033=CARTESIAN_POINT('Ctrl Pts',(-215.446264710151,-1.80244043944716,
124.037570439344));
#211034=CARTESIAN_POINT('Ctrl Pts',(-215.724712333964,-6.66735530697114,
128.66318942767));
#211035=CARTESIAN_POINT('Ctrl Pts',(-216.003159957777,-5.40529636580357,
135.256440137483));
#211036=CARTESIAN_POINT('Ctrl Pts',(-216.28160758159,0.823965872130078,
137.758447264668));
#211037=CARTESIAN_POINT('Ctrl Pts',(-216.560055205403,6.29604372654653,
133.869988489185));
#211038=CARTESIAN_POINT('Ctrl Pts',(-216.838502829216,5.98236497510254,
127.164367463932));
#211039=CARTESIAN_POINT('Ctrl Pts',(-217.116950453029,0.171185066315507,
123.803722323317));
#211040=CARTESIAN_POINT('Ctrl Pts',(-217.395398076842,-5.79730555555969,
126.876321774922));
#211041=CARTESIAN_POINT('Ctrl Pts',(-217.673845700654,-6.43835558599724,
133.558597027552));
#211042=CARTESIAN_POINT('Ctrl Pts',(-217.952293324468,-1.16287136405879,
137.709863571333));
#211043=CARTESIAN_POINT('Ctrl Pts',(-218.23074094828,5.18123483202488,135.515310253174));
#211044=CARTESIAN_POINT('Ctrl Pts',(-218.509188572093,6.76403933487094,
128.991624362576));
#211045=CARTESIAN_POINT('Ctrl Pts',(-218.787636195906,2.13102213066266,
124.133754533223));
#211046=CARTESIAN_POINT('Ctrl Pts',(-219.066083819719,-4.46030030540597,
125.405845818157));
#211047=CARTESIAN_POINT('Ctrl Pts',(-219.344531443532,-6.95282465859006,
131.638908471637));
#211048=CARTESIAN_POINT('Ctrl Pts',(-219.622979067345,-3.0560428148978,
137.105062417155));
#211049=CARTESIAN_POINT('Ctrl Pts',(-219.901426691158,3.6490930796943,136.781179215245));
#211050=CARTESIAN_POINT('Ctrl Pts',(-220.179874314971,7.00089070215466,
130.964891705888));
#211051=CARTESIAN_POINT('Ctrl Pts',(-220.458321938783,3.91921178185968,
125.001083968743));
#211052=CARTESIAN_POINT('Ctrl Pts',(-220.736769562596,-2.76403130182543,
124.370203966041));
#211053=CARTESIAN_POINT('Ctrl Pts',(-221.015217186409,-6.90726464956813,
129.651999600063));
#211054=CARTESIAN_POINT('Ctrl Pts',(-221.293664810222,-4.7030592229955,
135.992758713204));
#211055=CARTESIAN_POINT('Ctrl Pts',(-221.572112434035,1.82302787229404,
137.565633443793));
#211056=CARTESIAN_POINT('Ctrl Pts',(-221.850560057848,6.67384141280798,
132.925228753618));
#211057=CARTESIAN_POINT('Ctrl Pts',(-222.129007681661,5.39172073022998,
126.33584985658));
#211058=CARTESIAN_POINT('Ctrl Pts',(-222.407455305474,-0.845127903228338,
123.85281405));
#211059=CARTESIAN_POINT('Ctrl Pts',(-222.685902929286,-6.30534528041361,
127.757909937084));
#211060=CARTESIAN_POINT('Ctrl Pts',(-222.964350553099,-5.9712583781396,
134.462545172141));
#211061=CARTESIAN_POINT('Ctrl Pts',(-223.242798176912,-0.14987673854478,
137.805487513793));
#211062=CARTESIAN_POINT('Ctrl Pts',(-223.521245800725,5.80923430188729,
134.714736261875));
#211063=CARTESIAN_POINT('Ctrl Pts',(-223.799693424538,6.42994281575757,
128.030540825308));
#211064=CARTESIAN_POINT('Ctrl Pts',(-224.078141048351,1.1418480021166,123.895350269195));
#211065=CARTESIAN_POINT('Ctrl Pts',(-224.356588672164,-5.19554934309376,
126.109202699315));
#211066=CARTESIAN_POINT('Ctrl Pts',(-224.635036295977,-6.75849065869668,
132.637675885092));
#211067=CARTESIAN_POINT('Ctrl Pts',(-224.913483919789,-2.11070922958169,
137.481421902441));
#211068=CARTESIAN_POINT('Ctrl Pts',(-225.191931543603,4.47671086764076,
136.189274791569));
#211069=CARTESIAN_POINT('Ctrl Pts',(-225.470379167415,6.95025237698553,
129.948654622468));
#211070=CARTESIAN_POINT('Ctrl Pts',(-225.748826791228,3.03685149058481,
124.494386459301));
#211071=CARTESIAN_POINT('Ctrl Pts',(-226.027274415041,-3.66726755721984,
124.838676288203));
#211072=CARTESIAN_POINT('Ctrl Pts',(-226.305722038854,-7.00134687591997,
130.665138575908));
#211073=CARTESIAN_POINT('Ctrl Pts',(-226.584169662667,-3.9015304504591,
136.619539118521));
#211074=CARTESIAN_POINT('Ctrl Pts',(-226.86261728648,2.78360185861461,137.230074706019));
#211075=CARTESIAN_POINT('Ctrl Pts',(-227.141064910293,6.91074004613266,
131.935692959814));
#211076=CARTESIAN_POINT('Ctrl Pts',(-227.419512534106,4.68724573967455,
125.601672059739));
#211077=CARTESIAN_POINT('Ctrl Pts',(-227.697960157918,-1.8435984168596,
124.048667778841));
#211078=CARTESIAN_POINT('Ctrl Pts',(-227.976407781732,-6.68026569308986,
128.703815182788));
#211079=CARTESIAN_POINT('Ctrl Pts',(-228.254855405544,-5.37809514649209,
135.289261223946));
#211080=CARTESIAN_POINT('Ctrl Pts',(-228.533303029357,0.86628210517778,
137.753302707416));
#211081=CARTESIAN_POINT('Ctrl Pts',(-228.81175065317,6.31458842242258,133.831605885006));
#211082=CARTESIAN_POINT('Ctrl Pts',(-229.090198276983,5.96009646425557,
127.128018550972));
#211083=CARTESIAN_POINT('Ctrl Pts',(-229.368645900796,0.128567022336676,
123.802809976843));
#211084=CARTESIAN_POINT('Ctrl Pts',(-229.647093524609,-5.82110923226107,
126.911684396774));
#211085=CARTESIAN_POINT('Ctrl Pts',(-229.925541148421,-6.42147047940683,
133.597738095807));
#211086=CARTESIAN_POINT('Ctrl Pts',(-230.203988772235,-1.12081406224988,
137.716814356412));
#211087=CARTESIAN_POINT('Ctrl Pts',(-230.482436396047,5.20981572330331,
135.483683323156));
#211088=CARTESIAN_POINT('Ctrl Pts',(-230.76088401986,6.75287937278817,128.950483321085));
#211089=CARTESIAN_POINT('Ctrl Pts',(-231.039331643673,2.0903767751783,124.120905987538));
#211090=CARTESIAN_POINT('Ctrl Pts',(-231.317779267486,-4.49307995823781,
125.433096954076));
#211091=CARTESIAN_POINT('Ctrl Pts',(-231.596226891299,-6.94761570919197,
131.681216826544));
#211092=CARTESIAN_POINT('Ctrl Pts',(-231.874674515112,-3.01763203329532,
137.123548679767));
#211093=CARTESIAN_POINT('Ctrl Pts',(-232.153122138925,3.68540806167951,
136.758855413326));
#211094=CARTESIAN_POINT('Ctrl Pts',(-232.431569762738,7.00173819016367,
130.922272322824));
#211095=CARTESIAN_POINT('Ctrl Pts',(-232.71001738655,3.88381297581431,124.977334135496));
#211096=CARTESIAN_POINT('Ctrl Pts',(-232.988465010364,-2.80314662849731,
124.38714861912));
#211097=CARTESIAN_POINT('Ctrl Pts',(-233.266912634176,-6.914151422545,129.694067431082));
#211098=CARTESIAN_POINT('Ctrl Pts',(-233.545360257989,-4.67138883434919,
136.021291440583));
#211099=CARTESIAN_POINT('Ctrl Pts',(-233.823807881803,1.86415188258208,
137.554410884971));
#211100=CARTESIAN_POINT('Ctrl Pts',(-234.102255505615,6.68662808830262,
132.884563891901));
#211101=CARTESIAN_POINT('Ctrl Pts',(-234.380703129428,5.36441974081549,
126.303111713297));
#211102=CARTESIAN_POINT('Ctrl Pts',(-234.659150753241,-0.887428282007554,
123.858087379481));
#211103=CARTESIAN_POINT('Ctrl Pts',(-234.937598377053,-6.32377306694735,
127.796348807152));
#211104=CARTESIAN_POINT('Ctrl Pts',(-235.216046000867,-5.94887933685163,
134.498826139047));
#211105=CARTESIAN_POINT('Ctrl Pts',(-235.494493624679,-0.107256115101469,
137.806270141374));
#211106=CARTESIAN_POINT('Ctrl Pts',(-235.772941248493,5.83293023667497,
134.679301353618));
#211107=CARTESIAN_POINT('Ctrl Pts',(-236.051388872305,6.41293865542997,
127.991451330808));
#211108=CARTESIAN_POINT('Ctrl Pts',(-236.329836496118,1.09976973931543,
123.88852752427));
#211109=CARTESIAN_POINT('Ctrl Pts',(-236.608284119931,-5.22403384049169,
126.140916473241));
#211110=CARTESIAN_POINT('Ctrl Pts',(-236.886731743744,-6.7472055291277,
132.678782768935));
#211111=CARTESIAN_POINT('Ctrl Pts',(-237.165179367557,-2.07002495581049,
137.494146678133));
#211112=CARTESIAN_POINT('Ctrl Pts',(-237.44362699137,4.50940742555574,136.161924011888));
#211113=CARTESIAN_POINT('Ctrl Pts',(-237.722074615182,6.94491467963605,
129.906362317783));
#211114=CARTESIAN_POINT('Ctrl Pts',(-238.000522238996,2.99838462107406,
124.476017191522));
#211115=CARTESIAN_POINT('Ctrl Pts',(-238.278969862808,-3.70351442502255,
124.861110517033));
#211116=CARTESIAN_POINT('Ctrl Pts',(-238.557417486622,-7.00206464126185,
130.707760341024));
#211117=CARTESIAN_POINT('Ctrl Pts',(-238.835865110434,-3.86605952205578,
136.64318109997));
#211118=CARTESIAN_POINT('Ctrl Pts',(-239.114312734247,2.82266543041169,
137.213011077826));
#211119=CARTESIAN_POINT('Ctrl Pts',(-239.39276035806,6.91749874720356,131.893604362681));
#211120=CARTESIAN_POINT('Ctrl Pts',(-239.671207981873,4.655488653916,125.573235858291));
#211121=CARTESIAN_POINT('Ctrl Pts',(-239.949655605686,-1.88468807905538,
124.060015453022));
#211122=CARTESIAN_POINT('Ctrl Pts',(-240.228103229498,-6.69292853950653,
128.74451877439));
#211123=CARTESIAN_POINT('Ctrl Pts',(-240.506550853312,-5.35069463988719,
135.321916120768));
#211124=CARTESIAN_POINT('Ctrl Pts',(-240.784998477124,0.908566237823527,
137.747900654559));
#211125=CARTESIAN_POINT('Ctrl Pts',(-241.063446100938,6.33289912890243,
133.79311110514));
#211126=CARTESIAN_POINT('Ctrl Pts',(-241.34189372475,5.9376070998423,127.091805866219));
#211127=CARTESIAN_POINT('Ctrl Pts',(-241.620341348563,0.0859442142595387,
123.802157075403));
#211128=CARTESIAN_POINT('Ctrl Pts',(-241.898788972376,-5.84469720561911,
126.947191263173));
#211129=CARTESIAN_POINT('Ctrl Pts',(-242.177236596189,-6.40434742286629,
133.636775654432));
#211130=CARTESIAN_POINT('Ctrl Pts',(-242.455684220002,-1.07871522826414,
137.723508997977));
#211131=CARTESIAN_POINT('Ctrl Pts',(-242.734131843815,5.23820356294377,
135.451882999115));
#211132=CARTESIAN_POINT('Ctrl Pts',(-243.012579467628,6.74146918027728,
128.909410975699));
#211133=CARTESIAN_POINT('Ctrl Pts',(-243.29102709144,2.04965396001378,124.108305099723));
#211134=CARTESIAN_POINT('Ctrl Pts',(-243.569474715254,-4.52569311833944,
125.460547124147));
#211135=CARTESIAN_POINT('Ctrl Pts',(-243.847922339066,-6.94214931333881,
131.72349268922));
#211136=CARTESIAN_POINT('Ctrl Pts',(-244.12636996288,-2.9791094322281,137.141800782542));
#211137=CARTESIAN_POINT('Ctrl Pts',(-244.404817586691,3.72158647951367,
136.736310965414));
#211138=CARTESIAN_POINT('Ctrl Pts',(-244.683265210505,7.00232622618917,
130.879648570499));
#211139=CARTESIAN_POINT('Ctrl Pts',(-244.961712834317,3.84827025365086,
124.953800224859));
#211140=CARTESIAN_POINT('Ctrl Pts',(-245.240160458131,-2.84215808354001,
124.404331064352));
#211141=CARTESIAN_POINT('Ctrl Pts',(-245.518608081943,-6.92078198909823,
129.736176404423));
#211142=CARTESIAN_POINT('Ctrl Pts',(-245.797055705757,-4.63954534567172,
136.049630852671));
#211143=CARTESIAN_POINT('Ctrl Pts',(-246.075503329569,1.90520681603656,
137.542938200555));
#211144=CARTESIAN_POINT('Ctrl Pts',(-246.353950953382,6.69916698833444,
132.843821947487));
#211145=CARTESIAN_POINT('Ctrl Pts',(-246.632398577195,5.33691997085474,
126.270540365447));
#211146=CARTESIAN_POINT('Ctrl Pts',(-246.910846201008,-0.929695776805409,
123.86361810567));
#211147=CARTESIAN_POINT('Ctrl Pts',(-247.189293824821,-6.34196652374499,
127.834899140205));
#211148=CARTESIAN_POINT('Ctrl Pts',(-247.467741448634,-5.9262798576518,
134.534970206175));
#211149=CARTESIAN_POINT('Ctrl Pts',(-247.746189072447,-0.0646315172428821,
137.806793310625));
#211150=CARTESIAN_POINT('Ctrl Pts',(-248.024636696259,5.85641003008765,
134.643722858007));
#211151=CARTESIAN_POINT('Ctrl Pts',(-248.303084320073,6.39569686130214,
127.952466069697));
#211152=CARTESIAN_POINT('Ctrl Pts',(-248.581531943885,1.05765072414216,
123.881961048084));
#211153=CARTESIAN_POINT('Ctrl Pts',(-248.859979567699,-5.25232475939459,
126.172803052805));
#211154=CARTESIAN_POINT('Ctrl Pts',(-249.138427191511,-6.73567037937639,
132.719820195375));
#211155=CARTESIAN_POINT('Ctrl Pts',(-249.416874815324,-2.02926397650361,
137.506623561341));
#211156=CARTESIAN_POINT('Ctrl Pts',(-249.695322439137,4.54193688572079,
136.134374705723));
#211157=CARTESIAN_POINT('Ctrl Pts',(-249.97377006295,6.93931963591783,129.864103288757));
#211158=CARTESIAN_POINT('Ctrl Pts',(-250.252217686763,2.95980664532115,
124.457882422832));
#211159=CARTESIAN_POINT('Ctrl Pts',(-250.530665310576,-3.73962405773988,
124.883764975191));
#211160=CARTESIAN_POINT('Ctrl Pts',(-250.809112934388,-7.00252294251614,
130.750385685678));
#211161=CARTESIAN_POINT('Ctrl Pts',(-251.087560558202,-3.83044533540895,
136.666606721818));
#211162=CARTESIAN_POINT('Ctrl Pts',(-251.366008182014,2.86162440732935,
137.195709974661));
#211163=CARTESIAN_POINT('Ctrl Pts',(-251.644455805827,6.9240011177651,131.851475403357));
#211164=CARTESIAN_POINT('Ctrl Pts',(-251.92290342964,4.62355905740654,125.54499349784));
#211165=CARTESIAN_POINT('Ctrl Pts',(-252.201351053453,-1.92570790361727,
124.071613041873));
#211166=CARTESIAN_POINT('Ctrl Pts',(-252.479798677266,-6.70534337666252,
128.785298693283));
#211167=CARTESIAN_POINT('Ctrl Pts',(-252.758246301079,-5.3230958619522,
135.354403619622));
#211168=CARTESIAN_POINT('Ctrl Pts',(-253.036693924892,0.950816704398073,
137.74224130304));
#211169=CARTESIAN_POINT('Ctrl Pts',(-253.315141548704,6.35097516523885,
133.754505582129));
#211170=CARTESIAN_POINT('Ctrl Pts',(-253.593589172518,5.91489771943887,
127.055730740027));
#211171=CARTESIAN_POINT('Ctrl Pts',(-253.87203679633,0.0433182135112656,
123.801763664947));
#211172=CARTESIAN_POINT('Ctrl Pts',(-254.150484420143,-5.86806858651122,
126.982841017323));
#211173=CARTESIAN_POINT('Ctrl Pts',(-254.428932043956,-6.38698707931617,
133.675708334441));
#211174=CARTESIAN_POINT('Ctrl Pts',(-254.707379667769,-1.03657636838919,
137.729947101491));
#211175=CARTESIAN_POINT('Ctrl Pts',(-254.985827291582,5.26639719763008,
135.41991073597));
#211176=CARTESIAN_POINT('Ctrl Pts',(-255.264274915395,6.72980937160111,
128.868408326187));
#211177=CARTESIAN_POINT('Ctrl Pts',(-255.542722539208,2.00885483266244,
124.095953322692));
#211178=CARTESIAN_POINT('Ctrl Pts',(-255.821170163021,-4.5581378946222,
125.488193449449));
#211179=CARTESIAN_POINT('Ctrl Pts',(-256.099617786833,-6.93642696247006,
131.765738008466));
#211180=CARTESIAN_POINT('Ctrl Pts',(-256.378065410647,-2.94047400549736,
137.159811411449));
#211181=CARTESIAN_POINT('Ctrl Pts',(-256.656513034459,3.7576223973322,136.713559240208));
#211182=CARTESIAN_POINT('Ctrl Pts',(-256.934960658272,7.0026634652268,130.836998362911));
#211183=CARTESIAN_POINT('Ctrl Pts',(-257.213408282085,3.81256854888166,
124.930527794066));
#211184=CARTESIAN_POINT('Ctrl Pts',(-257.491855905898,-2.88103328591622,
124.421666290213));
#211185=CARTESIAN_POINT('Ctrl Pts',(-257.770303529711,-6.92721451599304,
129.778484277494));
#211186=CARTESIAN_POINT('Ctrl Pts',(-258.048751153524,-4.60741964202412,
136.077475067175));
#211187=CARTESIAN_POINT('Ctrl Pts',(-258.327198777336,1.94598288966397,
137.53178391186));
#211188=CARTESIAN_POINT('Ctrl Pts',(-258.60564640115,6.71185090883407,132.801931226644));
#211189=CARTESIAN_POINT('Ctrl Pts',(-258.884094024962,5.30847971878909,
126.240167716581));
#211190=CARTESIAN_POINT('Ctrl Pts',(-259.162541648776,-0.970525071554103,
123.86553674091));
#211191=CARTESIAN_POINT('Ctrl Pts',(-259.440989272588,-6.36258613651914,
127.881151058581));
#211192=CARTESIAN_POINT('Ctrl Pts',(-259.673028959099,-5.97575359986218,
133.442106215535));
#211193=CARTESIAN_POINT('Ctrl Pts',(-259.858689921174,-2.9628379271774,
136.206922793942));
#211194=CARTESIAN_POINT('Ctrl Pts',(-259.951535008647,-1.00384119663989,
136.721969923993));
#211195=CARTESIAN_POINT('Ctrl Pts',(-259.997972158816,-0.016740685831905,
136.724751058381));
#211196=CARTESIAN_POINT('Ctrl Pts',(210.384788400103,3.2437100417032,135.350446923363));
#211197=CARTESIAN_POINT('Ctrl Pts',(210.338370536501,4.00135710969089,134.809856772425));
#211198=CARTESIAN_POINT('Ctrl Pts',(210.245544735596,5.2274450014198,133.344996311945));
#211199=CARTESIAN_POINT('Ctrl Pts',(210.059903060087,6.03752477204218,129.574087134129));
#211200=CARTESIAN_POINT('Ctrl Pts',(209.827863373576,3.30140998082846,125.08375145776));
#211201=CARTESIAN_POINT('Ctrl Pts',(209.549415749763,-3.03864792542705,
124.935284604053));
#211202=CARTESIAN_POINT('Ctrl Pts',(209.27096812595,-6.57501826603042,130.18815040753));
#211203=CARTESIAN_POINT('Ctrl Pts',(208.992520502138,-4.0751627655632,136.003208990552));
#211204=CARTESIAN_POINT('Ctrl Pts',(208.714072878324,2.17267791003586,137.042921783734));
#211205=CARTESIAN_POINT('Ctrl Pts',(208.435625254512,6.42228832295553,132.348569225854));
#211206=CARTESIAN_POINT('Ctrl Pts',(208.157177630698,4.77100074356668,126.235763887068));
#211207=CARTESIAN_POINT('Ctrl Pts',(207.878730006886,-1.26506482749479,
124.320958291314));
#211208=CARTESIAN_POINT('Ctrl Pts',(207.600282383073,-6.13835327551471,
128.364250828182));
#211209=CARTESIAN_POINT('Ctrl Pts',(207.32183475926,-5.37092434612766,134.649796015418));
#211210=CARTESIAN_POINT('Ctrl Pts',(207.043387135447,0.332190207827403,
137.40162108792));
#211211=CARTESIAN_POINT('Ctrl Pts',(206.764939511634,5.73000189292936,134.090861108297));
#211212=CARTESIAN_POINT('Ctrl Pts',(206.486491887821,5.86224098722307,127.759980958474));
#211213=CARTESIAN_POINT('Ctrl Pts',(206.208044264008,0.607356820266201,
124.226729984437));
#211214=CARTESIAN_POINT('Ctrl Pts',(205.929596640195,-5.20565320191231,
126.738003936844));
#211215=CARTESIAN_POINT('Ctrl Pts',(205.651149016382,-6.23492509722864,
132.986059061584));
#211216=CARTESIAN_POINT('Ctrl Pts',(205.37270139257,-1.53460390898592,137.229240938669));
#211217=CARTESIAN_POINT('Ctrl Pts',(205.094253768756,4.57594250116295,135.568271122458));
#211218=CARTESIAN_POINT('Ctrl Pts',(204.815806144944,6.48142172411287,129.529500574057));
#211219=CARTESIAN_POINT('Ctrl Pts',(204.537358521131,2.43079079302514,124.662263970705));
#211220=CARTESIAN_POINT('Ctrl Pts',(204.258910897318,-3.85361800715474,
125.439314209572));
#211221=CARTESIAN_POINT('Ctrl Pts',(203.980463273505,-6.5967401814699,131.146579956944));
#211222=CARTESIAN_POINT('Ctrl Pts',(203.702015649692,-3.27778036432047,
136.539362872731));
#211223=CARTESIAN_POINT('Ctrl Pts',(203.42356802588,3.05329946149495,136.661958874297));
#211224=CARTESIAN_POINT('Ctrl Pts',(203.145120402066,6.5785462535266,131.40170824395));
#211225=CARTESIAN_POINT('Ctrl Pts',(202.866672778254,4.05843041346184,125.592524323598));
#211226=CARTESIAN_POINT('Ctrl Pts',(202.58822515444,-2.19118470860141,124.572763346851));
#211227=CARTESIAN_POINT('Ctrl Pts',(202.309777530628,-6.42720813017419,
129.279535830482));
#211228=CARTESIAN_POINT('Ctrl Pts',(202.031329906815,-4.75694126595338,
135.387547802118));
#211229=CARTESIAN_POINT('Ctrl Pts',(201.752882283002,1.28472223178851,137.283834652022));
#211230=CARTESIAN_POINT('Ctrl Pts',(201.474434659189,6.14578876089344,133.225801404307));
#211231=CARTESIAN_POINT('Ctrl Pts',(201.195987035376,5.35917565710019,126.94258236746));
#211232=CARTESIAN_POINT('Ctrl Pts',(200.917539411563,-0.352258065224466,
124.208148884143));
#211233=CARTESIAN_POINT('Ctrl Pts',(200.63909178775,-5.73998383440169,127.535311740963));
#211234=CARTESIAN_POINT('Ctrl Pts',(200.360644163938,-5.85294487354697,
133.866570813476));
#211235=CARTESIAN_POINT('Ctrl Pts',(200.082196540124,-0.587335506164227,
137.383808313225));
#211236=CARTESIAN_POINT('Ctrl Pts',(199.803748916312,5.2180064984534,134.854854804556));
#211237=CARTESIAN_POINT('Ctrl Pts',(199.525301292498,6.22825544477889,128.603695015683));
#211238=CARTESIAN_POINT('Ctrl Pts',(199.246853668687,1.51504190454761,124.374839406449));
#211239=CARTESIAN_POINT('Ctrl Pts',(198.968406044873,-4.5904211320519,126.054399690658));
#211240=CARTESIAN_POINT('Ctrl Pts',(198.689958421061,-6.47751140283473,
132.098942018204));
#211241=CARTESIAN_POINT('Ctrl Pts',(198.411510797247,-2.41208513843682,
136.95382728238));
#211242=CARTESIAN_POINT('Ctrl Pts',(198.133063173434,3.86992953127461,136.15765309974));
#211243=CARTESIAN_POINT('Ctrl Pts',(197.854615549622,6.59566801831256,130.442064648858));
#211244=CARTESIAN_POINT('Ctrl Pts',(197.576167925809,3.26030981281707,125.059408494076));
#211245=CARTESIAN_POINT('Ctrl Pts',(197.297720301996,-3.07111383566833,
124.956082684267));
#211246=CARTESIAN_POINT('Ctrl Pts',(197.019272678183,-6.58033390142619,
130.227038590899));
#211247=CARTESIAN_POINT('Ctrl Pts',(196.74082505437,-4.04254857895594,136.028525236289));
#211248=CARTESIAN_POINT('Ctrl Pts',(196.462377430557,2.21014139809766,137.029259811701));
#211249=CARTESIAN_POINT('Ctrl Pts',(196.183929806745,6.43181940170927,132.309616130935));
#211250=CARTESIAN_POINT('Ctrl Pts',(195.905482182931,4.74296958699597,126.206716169203));
#211251=CARTESIAN_POINT('Ctrl Pts',(195.627034559119,-1.30443757122094,
124.328826848098));
#211252=CARTESIAN_POINT('Ctrl Pts',(195.348586935305,-6.15313032680387,
128.401636713722));
#211253=CARTESIAN_POINT('Ctrl Pts',(195.070139311493,-5.34739690918169,
134.682432467391));
#211254=CARTESIAN_POINT('Ctrl Pts',(194.791691687679,0.372333033116476,
137.399469645412));
#211255=CARTESIAN_POINT('Ctrl Pts',(194.513244063867,5.74990710746052,134.055923815831));
#211256=CARTESIAN_POINT('Ctrl Pts',(194.234796440054,5.84359744862664,127.724350254736));
#211257=CARTESIAN_POINT('Ctrl Pts',(193.956348816241,0.567307210110782,
124.223155750211));
#211258=CARTESIAN_POINT('Ctrl Pts',(193.677901192428,-5.23031063999889,
126.769767009054));
#211259=CARTESIAN_POINT('Ctrl Pts',(193.399453568615,-6.22152852682933,
133.023972693263));
#211260=CARTESIAN_POINT('Ctrl Pts',(193.121005944802,-1.49546563606909,
137.238463313985));
#211261=CARTESIAN_POINT('Ctrl Pts',(192.84255832099,4.60485711668079,135.540327880088));
#211262=CARTESIAN_POINT('Ctrl Pts',(192.564110697177,6.47354113897745,129.490069896797));
#211263=CARTESIAN_POINT('Ctrl Pts',(192.285663073364,2.39335710461987,124.64758087922));
#211264=CARTESIAN_POINT('Ctrl Pts',(192.007215449551,-3.88620518688872,
125.462871665772));
#211265=CARTESIAN_POINT('Ctrl Pts',(191.728767825738,-6.59453476332446,
131.18672985278));
#211266=CARTESIAN_POINT('Ctrl Pts',(191.450320201925,-3.24280905319821,
136.559209392401));
#211267=CARTESIAN_POINT('Ctrl Pts',(191.171872578112,3.08889975678785,136.643264047941));
#211268=CARTESIAN_POINT('Ctrl Pts',(190.893424954299,6.58206059142805,131.361651697256));
#211269=CARTESIAN_POINT('Ctrl Pts',(190.614977330486,4.02662929408197,125.567916069518));
#211270=CARTESIAN_POINT('Ctrl Pts',(190.336529706674,-2.22907761274862,
124.586217166899));
#211271=CARTESIAN_POINT('Ctrl Pts',(190.05808208286,-6.43637108995848,129.318688322246));
#211272=CARTESIAN_POINT('Ctrl Pts',(189.779634459048,-4.72895396970476,
135.416419737866));
#211273=CARTESIAN_POINT('Ctrl Pts',(189.501186835235,1.32414082646293,137.275894133543));
#211274=CARTESIAN_POINT('Ctrl Pts',(189.222739211422,6.16041489098677,133.188345380025));
#211275=CARTESIAN_POINT('Ctrl Pts',(188.944291587609,5.33556862369218,126.910031093937));
#211276=CARTESIAN_POINT('Ctrl Pts',(188.665843963796,-0.392404551757433,
124.210415391489));
#211277=CARTESIAN_POINT('Ctrl Pts',(188.387396339983,-5.75977711417006,
127.570313219673));
#211278=CARTESIAN_POINT('Ctrl Pts',(188.10894871617,-5.83419588941534,133.902142614521));
#211279=CARTESIAN_POINT('Ctrl Pts',(187.830501092358,-0.547273658602122,
137.387261689231));
#211280=CARTESIAN_POINT('Ctrl Pts',(187.552053468544,5.24256632866185,134.823016271676));
#211281=CARTESIAN_POINT('Ctrl Pts',(187.273605844732,6.214743973489,128.565822630237));
#211282=CARTESIAN_POINT('Ctrl Pts',(186.995158220918,1.47587551380139,124.365736040492));
#211283=CARTESIAN_POINT('Ctrl Pts',(186.716710597106,-4.61925044254253,
126.082430892781));
#211284=CARTESIAN_POINT('Ctrl Pts',(186.438262973293,-6.46951090511933,
132.138348483055));
#211285=CARTESIAN_POINT('Ctrl Pts',(186.15981534948,-2.37460689906969,136.968396393875));
#211286=CARTESIAN_POINT('Ctrl Pts',(185.881367725667,3.90244484122886,136.133996556155));
#211287=CARTESIAN_POINT('Ctrl Pts',(185.602920101854,6.59334041746713,130.401921658061));
#211288=CARTESIAN_POINT('Ctrl Pts',(185.324472478041,3.22527825263932,125.039668503516));
#211289=CARTESIAN_POINT('Ctrl Pts',(185.046024854228,-3.10665706276191,
124.974885780916));
#211290=CARTESIAN_POINT('Ctrl Pts',(184.767577230416,-6.5837263061198,130.26710564752));
#211291=CARTESIAN_POINT('Ctrl Pts',(184.489129606603,-4.01067270706429,
136.05303658523));
#211292=CARTESIAN_POINT('Ctrl Pts',(184.21068198279,2.247993177529,137.015690720733));
#211293=CARTESIAN_POINT('Ctrl Pts',(183.932234358977,6.44086315254518,132.270435931769));
#211294=CARTESIAN_POINT('Ctrl Pts',(183.653786735164,4.71489454403,126.177929550814));
#211295=CARTESIAN_POINT('Ctrl Pts',(183.375339111351,-1.34383181504516,
124.33688730648));
#211296=CARTESIAN_POINT('Ctrl Pts',(183.096891487538,-6.16764238592767,
128.439137081397));
#211297=CARTESIAN_POINT('Ctrl Pts',(182.818443863726,-5.32369091022383,
134.71491173846));
#211298=CARTESIAN_POINT('Ctrl Pts',(182.539996239912,0.412472435216218,
137.397080956463));
#211299=CARTESIAN_POINT('Ctrl Pts',(182.2615486161,5.76959376309122,134.020862255314));
#211300=CARTESIAN_POINT('Ctrl Pts',(181.983100992287,5.82474028301032,127.688835683913));
#211301=CARTESIAN_POINT('Ctrl Pts',(181.704653368474,0.527235037225083,
124.219824324685));
#211302=CARTESIAN_POINT('Ctrl Pts',(181.426205744661,-5.25477345090652,
126.801680146133));
#211303=CARTESIAN_POINT('Ctrl Pts',(181.147758120848,-6.20790184760947,
133.061803779016));
#211304=CARTESIAN_POINT('Ctrl Pts',(180.869310497035,-1.45627171922457,
137.247447428754));
#211305=CARTESIAN_POINT('Ctrl Pts',(180.590862873222,4.63360097629919,135.5122090613));
#211306=CARTESIAN_POINT('Ctrl Pts',(180.31241524941,6.46542073859599,129.450687965235));
#211307=CARTESIAN_POINT('Ctrl Pts',(180.033967625596,2.35583469548556,124.633125906077));
#211308=CARTESIAN_POINT('Ctrl Pts',(179.755520001784,-3.91864834385308,
125.4866270652));
#211309=CARTESIAN_POINT('Ctrl Pts',(179.477072377971,-6.59208499180493,
131.226865573221));
#211310=CARTESIAN_POINT('Ctrl Pts',(179.198624754158,-3.20771757354326,
136.578842667508));
#211311=CARTESIAN_POINT('Ctrl Pts',(178.920177130345,3.12438558908937,136.62435285703));
#211312=CARTESIAN_POINT('Ctrl Pts',(178.641729506532,6.58533103007041,131.32157450091));
#211313=CARTESIAN_POINT('Ctrl Pts',(178.363281882719,3.99467896572256,125.5435018533));
#211314=CARTESIAN_POINT('Ctrl Pts',(178.084834258906,-2.26688791720775,
124.599901402811));
#211315=CARTESIAN_POINT('Ctrl Pts',(177.806386635093,-6.44529554785546,
129.357895865998));
#211316=CARTESIAN_POINT('Ctrl Pts',(177.527939011281,-4.70079144021631,
135.445120772143));
#211317=CARTESIAN_POINT('Ctrl Pts',(177.249491387467,1.36351035455298,137.26771380997));
#211318=CARTESIAN_POINT('Ctrl Pts',(176.971043763655,6.17481274467203,133.150801016333));
#211319=CARTESIAN_POINT('Ctrl Pts',(176.692596139842,5.31176387881016,126.877624126216));
#211320=CARTESIAN_POINT('Ctrl Pts',(176.414148516029,-0.432536497586617,
124.212926239906));
#211321=CARTESIAN_POINT('Ctrl Pts',(176.135700892216,-5.77935696328393,
127.605434537195));
#211322=CARTESIAN_POINT('Ctrl Pts',(175.857253268403,-5.81523071700703,
133.937599626117));
#211323=CARTESIAN_POINT('Ctrl Pts',(175.57880564459,-0.50719153161477,137.390471133416));
#211324=CARTESIAN_POINT('Ctrl Pts',(175.300358020777,5.2669318936477,134.791028826034));
#211325=CARTESIAN_POINT('Ctrl Pts',(175.021910396965,6.20100221257536,128.528033194638));
#211326=CARTESIAN_POINT('Ctrl Pts',(174.743462773151,1.43665443394553,124.356871260137));
#211327=CARTESIAN_POINT('Ctrl Pts',(174.465015149339,-4.64790858500931,
126.110637067746));
#211328=CARTESIAN_POINT('Ctrl Pts',(174.186567525525,-6.46127067729819,
132.177705516496));
#211329=CARTESIAN_POINT('Ctrl Pts',(173.908119901713,-2.33704066777073,
136.982737094758));
#211330=CARTESIAN_POINT('Ctrl Pts',(173.6296722779,3.93481554465429,136.11014252095));
#211331=CARTESIAN_POINT('Ctrl Pts',(173.351224654087,6.59076849796787,130.361793579788));
#211332=CARTESIAN_POINT('Ctrl Pts',(173.072777030274,3.1901271785899,125.020142125741));
#211333=CARTESIAN_POINT('Ctrl Pts',(172.794329406461,-3.14208517153551,
124.993904890899));
#211334=CARTESIAN_POINT('Ctrl Pts',(172.515881782648,-6.58687474841394,
130.30719261232));
#211335=CARTESIAN_POINT('Ctrl Pts',(172.237434158836,-3.97864821822065,
136.077353442554));
#211336=CARTESIAN_POINT('Ctrl Pts',(171.958986535022,2.28576165674636,137.001891466644));
#211337=CARTESIAN_POINT('Ctrl Pts',(171.68053891121,6.44966823482829,132.231201406644));
#211338=CARTESIAN_POINT('Ctrl Pts',(171.402091287397,4.68664478891289,126.149314366529));
#211339=CARTESIAN_POINT('Ctrl Pts',(171.123643663584,-1.38317626268716,
124.345187419464));
#211340=CARTESIAN_POINT('Ctrl Pts',(170.845196039771,-6.18192590079466,
128.476725093301));
#211341=CARTESIAN_POINT('Ctrl Pts',(170.566748415958,-5.29978763994156,
134.747246102621));
#211342=CARTESIAN_POINT('Ctrl Pts',(170.288300792145,0.452596552998033,
137.394447971839));
#211343=CARTESIAN_POINT('Ctrl Pts',(170.009853168332,5.78906662430322,133.985681506144));
#211344=CARTESIAN_POINT('Ctrl Pts',(169.73140554452,5.80566727950083,127.653436560012));
#211345=CARTESIAN_POINT('Ctrl Pts',(169.452957920706,0.487143327451347,
124.216736891574));
#211346=CARTESIAN_POINT('Ctrl Pts',(169.174510296894,-5.27904154425138,
126.833741604011));
#211347=CARTESIAN_POINT('Ctrl Pts',(168.896062673081,-6.19404513230377,
133.099551214382));
#211348=CARTESIAN_POINT('Ctrl Pts',(168.617615049268,-1.41702383969606,
137.256192792574));
#211349=CARTESIAN_POINT('Ctrl Pts',(168.339167425455,4.66217313612931,135.483915791456));
#211350=CARTESIAN_POINT('Ctrl Pts',(168.060719801642,6.45706075967145,129.411356194513));
#211351=CARTESIAN_POINT('Ctrl Pts',(167.782272177829,2.3182249900303,124.618899610305));
#211352=CARTESIAN_POINT('Ctrl Pts',(167.503824554016,-3.95094629386185,
125.510579515201));
#211353=CARTESIAN_POINT('Ctrl Pts',(167.225376930203,-6.58939094815179,
131.266985637585));
#211354=CARTESIAN_POINT('Ctrl Pts',(166.946929306391,-3.1725072307341,136.59826196706));
#211355=CARTESIAN_POINT('Ctrl Pts',(166.668481682578,3.15975564613386,136.605226004165));
#211356=CARTESIAN_POINT('Ctrl Pts',(166.390034058765,6.58835744684964,131.281478139015));
#211357=CARTESIAN_POINT('Ctrl Pts',(166.111586434952,3.96258061306513,125.519282580138));
#211358=CARTESIAN_POINT('Ctrl Pts',(165.833138811139,-2.30461422130139,
124.613815547242));
#211359=CARTESIAN_POINT('Ctrl Pts',(165.554691187326,-6.45398117295568,
129.397157009033));
#211360=CARTESIAN_POINT('Ctrl Pts',(165.276243563513,-4.67245472117232,
135.473649841348));
#211361=CARTESIAN_POINT('Ctrl Pts',(164.9977959397,1.40282935726546,137.259293984466));
#211362=CARTESIAN_POINT('Ctrl Pts',(164.719348315888,6.18898178840028,133.11316970443));
#211363=CARTESIAN_POINT('Ctrl Pts',(164.440900692075,5.2877623045642,126.845362665158));
#211364=CARTESIAN_POINT('Ctrl Pts',(164.162453068262,-0.472652415616787,
124.215681336348));
#211365=CARTESIAN_POINT('Ctrl Pts',(163.884005444449,-5.79872265620017,
127.640674392099));
#211366=CARTESIAN_POINT('Ctrl Pts',(163.605557820636,-5.79605005908598,
133.97294053439));
#211367=CARTESIAN_POINT('Ctrl Pts',(163.327110196823,-0.467090610458611,
137.393436526853));
#211368=CARTESIAN_POINT('Ctrl Pts',(163.04866257301,5.29110229053537,134.758893652935));
#211369=CARTESIAN_POINT('Ctrl Pts',(162.770214949197,6.18703067124424,128.49032810919));
#211370=CARTESIAN_POINT('Ctrl Pts',(162.491767325384,1.39738011833125,124.34824539387));
#211371=CARTESIAN_POINT('Ctrl Pts',(162.213319701571,-4.67639449751423,
126.139017170363));
#211372=CARTESIAN_POINT('Ctrl Pts',(161.934872077759,-6.45279102471594,
132.217011660137));
#211373=CARTESIAN_POINT('Ctrl Pts',(161.656424453946,-2.29938783657033,
136.996848853628));
#211374=CARTESIAN_POINT('Ctrl Pts',(161.377976830133,3.96704044204275,136.086091878046));
#211375=CARTESIAN_POINT('Ctrl Pts',(161.09952920632,6.58795235511813,130.321681900999));
#211376=CARTESIAN_POINT('Ctrl Pts',(160.821081582507,3.15485789320466,125.000830084311));
#211377=CARTESIAN_POINT('Ctrl Pts',(160.542633958694,-3.17739684918762,
125.013139309456));
#211378=CARTESIAN_POINT('Ctrl Pts',(160.264186334881,-6.58977911164196,
130.347297999864));
#211379=CARTESIAN_POINT('Ctrl Pts',(159.985738711068,-3.94647629910411,
136.10147490719));
#211380=CARTESIAN_POINT('Ctrl Pts',(159.707291087255,2.32344543622502,136.98786256077));
#211381=CARTESIAN_POINT('Ctrl Pts',(159.428843463442,6.45823432228318,132.191914009409));
#211382=CARTESIAN_POINT('Ctrl Pts',(159.15039583963,4.65822136844951,126.120871676696));
#211383=CARTESIAN_POINT('Ctrl Pts',(158.871948215817,-1.42246945622416,
124.353726879487));
#211384=CARTESIAN_POINT('Ctrl Pts',(158.593500592004,-6.19598034212407,
128.514399356595));
#211385=CARTESIAN_POINT('Ctrl Pts',(158.315052968191,-5.2756879840792,134.779434361708));
#211386=CARTESIAN_POINT('Ctrl Pts',(158.036605344378,0.49270389964821,137.391570789103));
#211387=CARTESIAN_POINT('Ctrl Pts',(157.758157720565,5.80832496952254,133.950382871961));
#211388=CARTESIAN_POINT('Ctrl Pts',(157.479710096752,5.78637914485521,127.618154194761));
#211389=CARTESIAN_POINT('Ctrl Pts',(157.201262472939,0.447033566402335,
124.213893565282));
#211390=CARTESIAN_POINT('Ctrl Pts',(156.922814849126,-5.3031140207705,126.865950194636));
#211391=CARTESIAN_POINT('Ctrl Pts',(156.644367225313,-6.17995889437779,
133.137213600617));
#211392=CARTESIAN_POINT('Ctrl Pts',(156.365919601501,-1.37772345182797,
137.264699081378));
#211393=CARTESIAN_POINT('Ctrl Pts',(156.087471977688,4.69057253741941,135.455449118975));
#211394=CARTESIAN_POINT('Ctrl Pts',(155.809024353875,6.44846151198586,129.372076042081));
#211395=CARTESIAN_POINT('Ctrl Pts',(155.530576730062,2.28052938189546,124.604902519066));
#211396=CARTESIAN_POINT('Ctrl Pts',(155.252129106249,-3.98309784010292,
125.534728128207));
#211397=CARTESIAN_POINT('Ctrl Pts',(154.973681482436,-6.58645273219382,
131.307088559209));
#211398=CARTESIAN_POINT('Ctrl Pts',(154.695233858623,-3.13717932950269,
136.617466571466));
#211399=CARTESIAN_POINT('Ctrl Pts',(154.41678623481,3.19500861727094,136.585884198101));
#211400=CARTESIAN_POINT('Ctrl Pts',(154.138338610998,6.59113972962085,131.241364097354));
#211401=CARTESIAN_POINT('Ctrl Pts',(153.859890987185,3.93033542552574,125.495259147487));
#211402=CARTESIAN_POINT('Ctrl Pts',(153.581443363372,-2.3422551270676,124.627959084596));
#211403=CARTESIAN_POINT('Ctrl Pts',(153.302995739559,-6.46242764341012,
129.436470296516));
#211404=CARTESIAN_POINT('Ctrl Pts',(153.024548115746,-4.64394486260028,
135.502005888322));
#211405=CARTESIAN_POINT('Ctrl Pts',(152.746100491933,1.44209637762021,137.250634969033));
#211406=CARTESIAN_POINT('Ctrl Pts',(152.46765286812,6.20292149713234,133.075452838754));
#211407=CARTESIAN_POINT('Ctrl Pts',(152.189205244307,5.26356479034146,126.813247906226));
#211408=CARTESIAN_POINT('Ctrl Pts',(151.910757620494,-0.512750819337957,
124.218680578724));
#211409=CARTESIAN_POINT('Ctrl Pts',(151.632309996682,-5.8178734753159,127.676031478561));
#211410=CARTESIAN_POINT('Ctrl Pts',(151.353862372869,-5.77665462639848,
134.008164029768));
#211411=CARTESIAN_POINT('Ctrl Pts',(151.075414749056,-0.4269723810881,137.39615775966));
#211412=CARTESIAN_POINT('Ctrl Pts',(150.796967125243,5.31507662368183,134.72661194316));
#211413=CARTESIAN_POINT('Ctrl Pts',(150.51851950143,6.17282986721635,128.452708771068));
#211414=CARTESIAN_POINT('Ctrl Pts',(150.240071877617,1.35805402228283,124.339858761329));
#211415=CARTESIAN_POINT('Ctrl Pts',(149.961624253804,-4.70470712450132,
126.167570148998));
#211416=CARTESIAN_POINT('Ctrl Pts',(149.683176629991,-6.44407226158927,
132.256265457474));
#211417=CARTESIAN_POINT('Ctrl Pts',(149.404729006178,-2.26164980070799,
137.010731147569));
#211418=CARTESIAN_POINT('Ctrl Pts',(149.126281382365,3.99911833928874,136.061845518646));
#211419=CARTESIAN_POINT('Ctrl Pts',(148.847833758553,6.58489209327119,130.281588108047));
#211420=CARTESIAN_POINT('Ctrl Pts',(148.56938613474,3.11947170339994,124.981733094838));
#211421=CARTESIAN_POINT('Ctrl Pts',(148.290938510927,-3.21259078723097,
125.032588323847));
#211422=CARTESIAN_POINT('Ctrl Pts',(148.012490887114,-6.59243928818165,
130.387420324031));
#211423=CARTESIAN_POINT('Ctrl Pts',(147.734043263301,-3.91415814185689,
136.125400085308));
#211424=CARTESIAN_POINT('Ctrl Pts',(147.455595639488,2.36104311957866,136.973604522958));
#211425=CARTESIAN_POINT('Ctrl Pts',(147.177148015675,6.46656109749016,132.152575195872));
#211426=CARTESIAN_POINT('Ctrl Pts',(146.898700391862,4.6296253358803,126.092602535266));
#211427=CARTESIAN_POINT('Ctrl Pts',(146.62025276805,-1.46170993963237,124.362505370115));
#211428=CARTESIAN_POINT('Ctrl Pts',(146.341805144237,-6.20980518912327,
128.552158475246));
#211429=CARTESIAN_POINT('Ctrl Pts',(146.063357520424,-5.2513928356585,134.811475322978));
#211430=CARTESIAN_POINT('Ctrl Pts',(145.784909896611,0.532792988974217,
137.388449514872));
#211431=CARTESIAN_POINT('Ctrl Pts',(145.506462272798,5.82736808512415,133.914967660766));
#211432=CARTESIAN_POINT('Ctrl Pts',(145.228014648985,5.76687659380242,127.582989895561));
#211433=CARTESIAN_POINT('Ctrl Pts',(144.949567025172,0.406907240360106,
124.211294451169));
#211434=CARTESIAN_POINT('Ctrl Pts',(144.671119401359,-5.32698998844935,
126.898304724507));
#211435=CARTESIAN_POINT('Ctrl Pts',(144.392671777546,-6.16564365580234,
133.174789542127));
#211436=CARTESIAN_POINT('Ctrl Pts',(144.114224153734,-1.33837201191069,
137.272965979966));
#211437=CARTESIAN_POINT('Ctrl Pts',(143.83577652992,4.71879812781917,135.426810098699));
#211438=CARTESIAN_POINT('Ctrl Pts',(143.557328906108,6.43962331418753,129.332848963481));
#211439=CARTESIAN_POINT('Ctrl Pts',(143.278881282295,2.24274926790569,124.591135151027));
#211440=CARTESIAN_POINT('Ctrl Pts',(143.000433658482,-4.01510179118866,
125.559072009383));
#211441=CARTESIAN_POINT('Ctrl Pts',(142.721986034669,-6.58327045280769,
131.347172852065));
#211442=CARTESIAN_POINT('Ctrl Pts',(142.443538410856,-3.10173517893752,
136.636455769093));
#211443=CARTESIAN_POINT('Ctrl Pts',(142.165090787043,3.23014319618891,136.566328155556));
#211444=CARTESIAN_POINT('Ctrl Pts',(141.886643163231,6.5936777752854,131.201233862367));
#211445=CARTESIAN_POINT('Ctrl Pts',(141.608195539417,3.89794459796173,125.471432445543));
#211446=CARTESIAN_POINT('Ctrl Pts',(141.329747915605,-2.37980923970876,
124.642331490782));
#211447=CARTESIAN_POINT('Ctrl Pts',(141.051300291792,-6.47063464623165,
129.475834271677));
#211448=CARTESIAN_POINT('Ctrl Pts',(140.772852667979,-4.61526292094352,
135.530187862324));
#211449=CARTESIAN_POINT('Ctrl Pts',(140.494405044166,1.48130996056343,137.241737084533));
#211450=CARTESIAN_POINT('Ctrl Pts',(140.215957420353,6.21663135432719,133.037651816923));
#211451=CARTESIAN_POINT('Ctrl Pts',(139.93750979654,5.23917223278974,126.781281039444));
#211452=CARTESIAN_POINT('Ctrl Pts',(139.659062172727,-0.552830222889001,
124.221923855894));
#211453=CARTESIAN_POINT('Ctrl Pts',(139.380614548914,-5.83680871099059,
127.711504486408));
#211454=CARTESIAN_POINT('Ctrl Pts',(139.102166925101,-5.75704513764935,
134.043268807033));
#211455=CARTESIAN_POINT('Ctrl Pts',(138.823719301288,-0.386838330098996,
137.398634730999));
#211456=CARTESIAN_POINT('Ctrl Pts',(138.545271677476,5.33885400470937,134.694184892919));
#211457=CARTESIAN_POINT('Ctrl Pts',(138.266824053663,6.15840032670771,128.41517657427));
#211458=CARTESIAN_POINT('Ctrl Pts',(137.98837642985,1.31867760304303,124.331711673279));
#211459=CARTESIAN_POINT('Ctrl Pts',(137.709928806037,-4.7328454168358,126.196294945608));
#211460=CARTESIAN_POINT('Ctrl Pts',(137.431481182224,-6.43511471099507,
132.295465453942));
#211461=CARTESIAN_POINT('Ctrl Pts',(137.153033558411,-2.22382795858067,
137.024383462168));
#211462=CARTESIAN_POINT('Ctrl Pts',(136.874585934598,4.03104804773404,136.037404341212));
#211463=CARTESIAN_POINT('Ctrl Pts',(136.596138310785,6.5815878258261,130.241513686623));
#211464=CARTESIAN_POINT('Ctrl Pts',(136.317690686972,3.08396992042408,124.96285186497));
#211465=CARTESIAN_POINT('Ctrl Pts',(136.03924306316,-3.24766568154122,125.052251213384));
#211466=CARTESIAN_POINT('Ctrl Pts',(135.760795439346,-6.5948551794591,130.427558098075));
#211467=CARTESIAN_POINT('Ctrl Pts',(135.482347815534,-3.88169494404043,
136.149128090351));
#211468=CARTESIAN_POINT('Ctrl Pts',(135.203900191721,2.3985533136112,136.959117881544));
#211469=CARTESIAN_POINT('Ctrl Pts',(134.925452567908,6.47464825189767,132.113186423748));
#211470=CARTESIAN_POINT('Ctrl Pts',(134.647004944095,4.60085775084163,126.064507989766));
#211471=CARTESIAN_POINT('Ctrl Pts',(134.368557320282,-1.50089625884118,
124.371522566057));
#211472=CARTESIAN_POINT('Ctrl Pts',(134.090109696469,-6.22339992950755,
128.590001050074));
#211473=CARTESIAN_POINT('Ctrl Pts',(133.811662072656,-5.22690309494509,
134.843367799137));
#211474=CARTESIAN_POINT('Ctrl Pts',(133.533214448844,0.572862335460145,
137.385084264805));
#211475=CARTESIAN_POINT('Ctrl Pts',(133.25476682503,5.84619526545829,133.879437184883));
#211476=CARTESIAN_POINT('Ctrl Pts',(132.976319201218,5.7471603490167,127.547944965438));
#211477=CARTESIAN_POINT('Ctrl Pts',(132.697871577405,0.366765836220533,
124.208939645549));
#211478=CARTESIAN_POINT('Ctrl Pts',(132.419423953592,-5.35066856255522,
126.930803994717));
#211479=CARTESIAN_POINT('Ctrl Pts',(132.140976329779,-6.15109994703373,
133.212277646521));
#211480=CARTESIAN_POINT('Ctrl Pts',(131.862528705966,-1.29897097812634,
137.280993182001));
#211481=CARTESIAN_POINT('Ctrl Pts',(131.584081082153,4.74684886141891,135.397999791857));
#211482=CARTESIAN_POINT('Ctrl Pts',(131.30563345834,6.43054649377913,129.293676412286));
#211483=CARTESIAN_POINT('Ctrl Pts',(131.027185834528,2.20488604801711,124.577598016342));
#211484=CARTESIAN_POINT('Ctrl Pts',(130.748738210715,-4.04695696120101,
125.583610256657));
#211485=CARTESIAN_POINT('Ctrl Pts',(130.470290586902,-6.57984422791396,
131.387237030814));
#211486=CARTESIAN_POINT('Ctrl Pts',(130.191842963089,-3.06617609243459,
136.65522885629));
#211487=CARTESIAN_POINT('Ctrl Pts',(129.913395339276,3.26515808096253,136.546558601182));
#211488=CARTESIAN_POINT('Ctrl Pts',(129.634947715463,6.59597148979528,131.161088921098));
#211489=CARTESIAN_POINT('Ctrl Pts',(129.35650009165,3.86540933062731,125.447803357213));
#211490=CARTESIAN_POINT('Ctrl Pts',(129.078052467837,-2.41727516764341,
124.656932233223));
#211491=CARTESIAN_POINT('Ctrl Pts',(128.799604844024,-6.47860187730669,
129.515247475871));
#211492=CARTESIAN_POINT('Ctrl Pts',(128.521157220212,-4.58640995902212,
135.558194719059));
#211493=CARTESIAN_POINT('Ctrl Pts',(128.242709596398,1.52046865302106,137.232600660681));
#211494=CARTESIAN_POINT('Ctrl Pts',(127.964261972586,6.23011085196111,132.999768039666));
#211495=CARTESIAN_POINT('Ctrl Pts',(127.685814348773,5.2145855357842,126.749463249355));
#211496=CARTESIAN_POINT('Ctrl Pts',(127.40736672496,-0.592889141112855,
124.225411047681));
#211497=CARTESIAN_POINT('Ctrl Pts',(127.128919101147,-5.85552766157182,
127.747092101177));
#211498=CARTESIAN_POINT('Ctrl Pts',(126.850471477334,-5.7372223194756,134.078253565364));
#211499=CARTESIAN_POINT('Ctrl Pts',(126.572023853521,-0.346689944673359,
137.400867349086));
#211500=CARTESIAN_POINT('Ctrl Pts',(126.293576229708,5.36243355253846,134.66161370381));
#211501=CARTESIAN_POINT('Ctrl Pts',(126.015128605896,6.14374258441013,128.377732909565));
#211502=CARTESIAN_POINT('Ctrl Pts',(125.736680982083,1.27925231971985,124.323804431618));
#211503=CARTESIAN_POINT('Ctrl Pts',(125.45823335827,-4.76080833184274,126.225190495787));
#211504=CARTESIAN_POINT('Ctrl Pts',(125.179785734457,-6.42591870485886,
132.334610196974));
#211505=CARTESIAN_POINT('Ctrl Pts',(124.901338110644,-2.1859237116904,137.037805291532));
#211506=CARTESIAN_POINT('Ctrl Pts',(124.622890486831,4.06282838421153,136.012769251418));
#211507=CARTESIAN_POINT('Ctrl Pts',(124.344442863018,6.5780396752237,130.201460121699));
#211508=CARTESIAN_POINT('Ctrl Pts',(124.065995239205,3.04835385980878,124.944187094356));
#211509=CARTESIAN_POINT('Ctrl Pts',(123.787547615392,-3.28262023240536,
125.07212724945));
#211510=CARTESIAN_POINT('Ctrl Pts',(123.509099991579,-6.59702669595264,
130.467709834674));
#211511=CARTESIAN_POINT('Ctrl Pts',(123.230652367767,-3.84908790859021,
136.17265804307));
#211512=CARTESIAN_POINT('Ctrl Pts',(122.952204743954,2.43597462836867,136.944403173336));
#211513=CARTESIAN_POINT('Ctrl Pts',(122.673757120141,6.48249548583303,132.073749152604));
#211514=CARTESIAN_POINT('Ctrl Pts',(122.395309496328,4.57191967932717,126.036589081248));
#211515=CARTESIAN_POINT('Ctrl Pts',(122.116861872515,-1.54002696178715,
124.380778133181));
#211516=CARTESIAN_POINT('Ctrl Pts',(121.838414248702,-6.23676405951882,
128.627925678811));
#211517=CARTESIAN_POINT('Ctrl Pts',(121.559966624889,-5.20221966941523,
134.8751106084));
#211518=CARTESIAN_POINT('Ctrl Pts',(121.281519001076,0.612910454321425,
137.381475163605));
#211519=CARTESIAN_POINT('Ctrl Pts',(121.003071377263,5.86480581287692,133.843792760907));
#211520=CARTESIAN_POINT('Ctrl Pts',(120.724623753451,5.72723114109079,127.513020702994));
#211521=CARTESIAN_POINT('Ctrl Pts',(120.446176129638,0.326610841437887,
124.206829235678));
#211522=CARTESIAN_POINT('Ctrl Pts',(120.167728505825,-5.3741488656698,126.963446800991));
#211523=CARTESIAN_POINT('Ctrl Pts',(119.889280882012,-6.13632830699453,
133.249676524665));
#211524=CARTESIAN_POINT('Ctrl Pts',(119.610833258199,-1.25952181049465,
137.288780390037));
#211525=CARTESIAN_POINT('Ctrl Pts',(119.332385634386,4.77472369878856,135.369019266025));
#211526=CARTESIAN_POINT('Ctrl Pts',(119.053938010573,6.42123138710552,129.254559840052));
#211527=CARTESIAN_POINT('Ctrl Pts',(118.77549038676,2.16694112526505,124.564291616636));
#211528=CARTESIAN_POINT('Ctrl Pts',(118.497042762948,-4.07866216973492,
125.608341960757));
#211529=CARTESIAN_POINT('Ctrl Pts',(118.218595139134,-6.57617418447253,
131.427279610862));
#211530=CARTESIAN_POINT('Ctrl Pts',(117.940147515322,-3.03050338764912,
136.673785137412));
#211531=CARTESIAN_POINT('Ctrl Pts',(117.661699891509,3.30005197410286,136.526576267552));
#211532=CARTESIAN_POINT('Ctrl Pts',(117.383252267696,6.59802078815589,131.120930761129));
#211533=CARTESIAN_POINT('Ctrl Pts',(117.104804643883,3.83273082912851,125.424372758082));
#211534=CARTESIAN_POINT('Ctrl Pts',(116.82635702007,-2.45465152255762,124.671760770883));
#211535=CARTESIAN_POINT('Ctrl Pts',(116.547909396257,-6.48632904140672,
129.554708448625));
#211536=CARTESIAN_POINT('Ctrl Pts',(116.269461772444,-4.55738704599302,
135.586025420722));
#211537=CARTESIAN_POINT('Ctrl Pts',(115.991014148631,1.55957100395386,137.223226036031));
#211538=CARTESIAN_POINT('Ctrl Pts',(115.712566524818,6.24335949054626,132.961802910777));
#211539=CARTESIAN_POINT('Ctrl Pts',(115.434118901006,5.18980561039392,126.717795714978));
#211540=CARTESIAN_POINT('Ctrl Pts',(115.155671277193,-0.632926089611396,
124.229142024863));
#211541=CARTESIAN_POINT('Ctrl Pts',(114.87722365338,-5.87402963342224,127.782793004156));
#211542=CARTESIAN_POINT('Ctrl Pts',(114.598776029567,-5.71718690641897,
134.113117008387));
#211543=CARTESIAN_POINT('Ctrl Pts',(114.320328405754,-0.306528712524212,
137.40285553119));
#211544=CARTESIAN_POINT('Ctrl Pts',(114.041880781941,5.38581439342023,134.628899582769));
#211545=CARTESIAN_POINT('Ctrl Pts',(113.763433158128,6.12885718347172,128.340379164441));
#211546=CARTESIAN_POINT('Ctrl Pts',(113.484985534315,1.23977963323159,124.316137329349));
#211547=CARTESIAN_POINT('Ctrl Pts',(113.206537910502,-4.78859483334625,
126.254255728798));
#211548=CARTESIAN_POINT('Ctrl Pts',(112.92809028669,-6.41648458394181,132.373698236044));
#211549=CARTESIAN_POINT('Ctrl Pts',(112.649642662877,-2.14793846459313,
137.050996138312));
#211550=CARTESIAN_POINT('Ctrl Pts',(112.371195039064,4.09445817108915,135.987941162125));
#211551=CARTESIAN_POINT('Ctrl Pts',(112.092747415251,6.57424777294209,130.161428897475));
#211552=CARTESIAN_POINT('Ctrl Pts',(111.814299791438,3.01262484132005,124.925739474628));
#211553=CARTESIAN_POINT('Ctrl Pts',(111.535852167625,-3.31745314456969,
125.092215695531));
#211554=CARTESIAN_POINT('Ctrl Pts',(111.257404543812,-6.59895375719588,
130.507874045991));
#211555=CARTESIAN_POINT('Ctrl Pts',(110.978956919999,-3.816338243772,136.195989071554));
#211556=CARTESIAN_POINT('Ctrl Pts',(110.700509296186,2.47330567719032,136.929460943594));
#211557=CARTESIAN_POINT('Ctrl Pts',(110.422061672374,6.49010250851429,132.0342648438));
#211558=CARTESIAN_POINT('Ctrl Pts',(110.143614048561,4.54281219364771,126.008846844259));
#211559=CARTESIAN_POINT('Ctrl Pts',(109.865166424748,-1.57910059846782,
124.390271728514));
#211560=CARTESIAN_POINT('Ctrl Pts',(109.586718800935,-6.24989708394428,
128.665930956147));
#211561=CARTESIAN_POINT('Ctrl Pts',(109.308271177122,-5.17734347372243,
134.906702574525));
#211562=CARTESIAN_POINT('Ctrl Pts',(109.029823553309,0.652935861560398,
137.377622345005));
#211563=CARTESIAN_POINT('Ctrl Pts',(108.751375929496,5.88319903775945,133.808035709655));
#211564=CARTESIAN_POINT('Ctrl Pts',(108.472928305683,5.70708970850866,127.478218402361));
#211565=CARTESIAN_POINT('Ctrl Pts',(108.19448068187,0.286443743970404,124.204963299759));
#211566=CARTESIAN_POINT('Ctrl Pts',(107.916033058058,-5.39743002772183,
126.996231933739));
#211567=CARTESIAN_POINT('Ctrl Pts',(107.637585434244,-6.12132928305326,
133.286984790727));
#211568=CARTESIAN_POINT('Ctrl Pts',(107.359137810432,-1.22002597081922,
137.296327315513));
#211569=CARTESIAN_POINT('Ctrl Pts',(107.080690186619,4.80242160701559,135.339869595089));
#211570=CARTESIAN_POINT('Ctrl Pts',(106.802242562806,6.41167833934146,129.215500696253));
#211571=CARTESIAN_POINT('Ctrl Pts',(106.523794938993,2.12891590571267,124.551216444981));
#211572=CARTESIAN_POINT('Ctrl Pts',(106.24534731518,-4.11021624194206,125.633266205238));
#211573=CARTESIAN_POINT('Ctrl Pts',(105.966899691367,-6.57226045847839,
131.467299108419));
#211574=CARTESIAN_POINT('Ctrl Pts',(105.688452067554,-2.99471838644612,
136.692123924851));
#211575=CARTESIAN_POINT('Ctrl Pts',(105.410004443742,3.33482358260376,136.506381895117));
#211576=CARTESIAN_POINT('Ctrl Pts',(105.131556819929,6.59982559442975,131.080760870538));
#211577=CARTESIAN_POINT('Ctrl Pts',(104.853109196116,3.79991030437941,125.401141516381));
#211578=CARTESIAN_POINT('Ctrl Pts',(104.574661572303,-2.49193691945696,
124.686816554284));
#211579=CARTESIAN_POINT('Ctrl Pts',(104.29621394849,-6.49381585219884,129.594215727701));
#211580=CARTESIAN_POINT('Ctrl Pts',(104.017766324677,-4.52819525731082,
135.613678936038));
#211581=CARTESIAN_POINT('Ctrl Pts',(103.739318700864,1.59861556440955,137.213613557961));
#211582=CARTESIAN_POINT('Ctrl Pts',(103.460871077051,6.25637677914949,132.923757837073));
#211583=CARTESIAN_POINT('Ctrl Pts',(103.182423453238,5.16483337484823,126.686279609768));
#211584=CARTESIAN_POINT('Ctrl Pts',(102.903975829425,-0.672939584800916,
124.233116649188));
#211585=CARTESIAN_POINT('Ctrl Pts',(102.625528205613,-5.89231394094447,
127.818605872432));
#211586=CARTESIAN_POINT('Ctrl Pts',(102.347080581799,-5.69693964089892,
134.147857844226));
#211587=CARTESIAN_POINT('Ctrl Pts',(102.068632957987,-0.266356121840884,
137.40459920364));
#211588=CARTESIAN_POINT('Ctrl Pts',(101.790185334174,5.40899566096888,134.59604374203));
#211589=CARTESIAN_POINT('Ctrl Pts',(101.511737710361,6.11374467547657,128.303116723058));
#211590=CARTESIAN_POINT('Ctrl Pts',(101.233290086548,1.20026100625305,124.308710650579));
#211591=CARTESIAN_POINT('Ctrl Pts',(100.954842462735,-4.81620389170723,
126.28348956762));
#211592=CARTESIAN_POINT('Ctrl Pts',(100.676394838922,-6.40681269782886,
132.412728122731));
#211593=CARTESIAN_POINT('Ctrl Pts',(100.397947215109,-2.10987362484612,
137.063955513716));
#211594=CARTESIAN_POINT('Ctrl Pts',(100.119499591297,4.12593623631335,135.962920993349));
#211595=CARTESIAN_POINT('Ctrl Pts',(99.8410519674839,6.5702122594916,130.121421497322));
#211596=CARTESIAN_POINT('Ctrl Pts',(99.5626043436712,2.97678418891005,124.907509689368));
#211597=CARTESIAN_POINT('Ctrl Pts',(99.2841567198582,-3.35216312728773,
125.112515807244));
#211598=CARTESIAN_POINT('Ctrl Pts',(99.0057090960455,-6.6006362917809,130.548049243728));
#211599=CARTESIAN_POINT('Ctrl Pts',(98.7272614722323,-3.78344716313679,
136.219120311263));
#211600=CARTESIAN_POINT('Ctrl Pts',(98.4488138484198,2.51054507676055,136.914291746006));
#211601=CARTESIAN_POINT('Ctrl Pts',(98.1703662246066,6.49746903806041,131.994734960442));
#211602=CARTESIAN_POINT('Ctrl Pts',(97.8919186007939,4.51353637239165,125.981282306795));
#211603=CARTESIAN_POINT('Ctrl Pts',(97.6134709769809,-1.61811572099509,
124.400003000271));
#211604=CARTESIAN_POINT('Ctrl Pts',(97.335023353168,-6.26279851613479,128.704015473778));
#211605=CARTESIAN_POINT('Ctrl Pts',(97.0565757293552,-5.15227542966332,
134.938142526861));
#211606=CARTESIAN_POINT('Ctrl Pts',(96.7781281055422,0.692937074020952,
137.373525951775));
#211607=CARTESIAN_POINT('Ctrl Pts',(96.4996804817294,5.90137425853808,133.772167356118));
#211608=CARTESIAN_POINT('Ctrl Pts',(96.2212328579164,5.6867367976186,127.443539353151));
#211609=CARTESIAN_POINT('Ctrl Pts',(95.9427852341037,0.246266032224636,
124.203341906934));
#211610=CARTESIAN_POINT('Ctrl Pts',(95.6643376102905,-5.42051118601915,
127.029158178097));
#211611=CARTESIAN_POINT('Ctrl Pts',(95.3858899864779,-6.10610343100435,
133.324201062238));
#211612=CARTESIAN_POINT('Ctrl Pts',(95.1074423626648,-1.18048492263276,
137.303633678775));
#211613=CARTESIAN_POINT('Ctrl Pts',(94.828994738852,4.82994155974394,135.3105518592));
#211614=CARTESIAN_POINT('Ctrl Pts',(94.5505471150391,6.40188770447863,129.176500428244));
#211615=CARTESIAN_POINT('Ctrl Pts',(94.2720994912261,2.09081179839861,124.538372985881));
#211616=CARTESIAN_POINT('Ctrl Pts',(93.9936518674133,-4.14161800857485,
125.658382066524));
#211617=CARTESIAN_POINT('Ctrl Pts',(93.7152042436005,-6.56810319495607,
131.507294040545));
#211618=CARTESIAN_POINT('Ctrl Pts',(93.4367566197874,-2.95882241485189,
136.710244539055));
#211619=CARTESIAN_POINT('Ctrl Pts',(93.1583089959747,3.36947161799043,136.485976232185));
#211620=CARTESIAN_POINT('Ctrl Pts',(92.8798613721617,6.60138584173913,131.040580737834));
#211621=CARTESIAN_POINT('Ctrl Pts',(92.6014137483489,3.76694897255651,125.37811049295));
#211622=CARTESIAN_POINT('Ctrl Pts',(92.3229661245359,-2.5291299767175,124.702099025532));
#211623=CARTESIAN_POINT('Ctrl Pts',(92.044518500723,-6.50106203225643,129.633767849141));
#211624=CARTESIAN_POINT('Ctrl Pts',(91.7660708769102,-4.49883567468812,
135.641154240296));
#211625=CARTESIAN_POINT('Ctrl Pts',(91.4876232530973,1.63760088757763,137.203763582666));
#211626=CARTESIAN_POINT('Ctrl Pts',(91.2091756292845,6.26916223541028,132.885634228324));
#211627=CARTESIAN_POINT('Ctrl Pts',(90.9307280054714,5.13966975450256,126.654916101563));
#211628=CARTESIAN_POINT('Ctrl Pts',(90.6522803816587,-0.71292814396669,
124.237334773374));
#211629=CARTESIAN_POINT('Ctrl Pts',(90.3738327578456,-5.91037990660673,
127.85452937895));
#211630=CARTESIAN_POINT('Ctrl Pts',(90.0953851340328,-5.67648127318543,
134.182474785545));
#211631=CARTESIAN_POINT('Ctrl Pts',(89.8169375102199,-0.226173661233629,
137.406098301819));
#211632=CARTESIAN_POINT('Ctrl Pts',(89.5384898864071,5.43197649619419,134.563047399079));
#211633=CARTESIAN_POINT('Ctrl Pts',(89.260042262594,6.09840562042418,128.265946966186));
#211634=CARTESIAN_POINT('Ctrl Pts',(88.9815946387814,1.1606979031614,124.301524670509));
#211635=CARTESIAN_POINT('Ctrl Pts',(88.7031470149683,-4.84363448386183,
126.312890928981));
#211636=CARTESIAN_POINT('Ctrl Pts',(88.4246993911556,-6.39690340491527,
132.45169841077));
#211637=CARTESIAN_POINT('Ctrl Pts',(88.1462517673426,-2.07173060295614,
137.076682937528));
#211638=CARTESIAN_POINT('Ctrl Pts',(87.8678041435297,4.15726141345302,135.937709672222));
#211639=CARTESIAN_POINT('Ctrl Pts',(87.5893565197169,6.5659332844097,130.081439403729));
#211640=CARTESIAN_POINT('Ctrl Pts',(87.3109088959039,2.94083323066708,124.889498414087));
#211641=CARTESIAN_POINT('Ctrl Pts',(87.032461272091,-3.38674889436835,125.133026832359));
#211642=CARTESIAN_POINT('Ctrl Pts',(86.7540136482781,-6.60207423736065,
130.588233939178));
#211643=CARTESIAN_POINT('Ctrl Pts',(86.4755660244652,-3.75041588547566,
136.242050905059));
#211644=CARTESIAN_POINT('Ctrl Pts',(86.1971184006524,2.54769144715974,136.898896142674));
#211645=CARTESIAN_POINT('Ctrl Pts',(85.9186707768394,6.50459480150186,131.955160967326));
#211646=CARTESIAN_POINT('Ctrl Pts',(85.6402231530266,4.48409330038545,125.953896490271));
#211647=CARTESIAN_POINT('Ctrl Pts',(85.3617755292137,-1.65707088364924,
124.409971587854));
#211648=CARTESIAN_POINT('Ctrl Pts',(85.0833279054008,-6.27546787802325,
128.742177820471));
#211649=CARTESIAN_POINT('Ctrl Pts',(84.8048802815879,-5.12701646614329,
134.969429300388));
#211650=CARTESIAN_POINT('Ctrl Pts',(84.526432657775,0.732912609443495,137.369186135708));
#211651=CARTESIAN_POINT('Ctrl Pts',(84.2479850339622,5.91933080172332,133.73618902941));
#211652=CARTESIAN_POINT('Ctrl Pts',(83.9695374101491,5.6661731626052,127.408984840408));
#211653=CARTESIAN_POINT('Ctrl Pts',(83.6910897863363,0.206079195000604,
124.201965117285));
#211654=CARTESIAN_POINT('Ctrl Pts',(83.4126421625234,-5.44339148528112,
127.062224313968));
#211655=CARTESIAN_POINT('Ctrl Pts',(83.1341945387106,-6.09065131504733,
133.361323960135));
#211656=CARTESIAN_POINT('Ctrl Pts',(82.8557469148977,-1.14090013114324,
137.310699209084));
#211657=CARTESIAN_POINT('Ctrl Pts',(82.5772992910847,4.85728253721157,135.281067144739));
#211658=CARTESIAN_POINT('Ctrl Pts',(82.2988516672719,6.39185984531258,129.137560481192));
#211659=CARTESIAN_POINT('Ctrl Pts',(82.0204040434589,2.05263021528453,124.52576171526));
#211660=CARTESIAN_POINT('Ctrl Pts',(81.7419564196462,-4.17286630602932,
125.683688613938));
#211661=CARTESIAN_POINT('Ctrl Pts',(81.4635087958331,-6.56370254795435,
131.547262925216));
#211662=CARTESIAN_POINT('Ctrl Pts',(81.1850611720204,-2.92281680300497,
136.728146308557));
#211663=CARTESIAN_POINT('Ctrl Pts',(80.9066135482074,3.40399479636718,136.465360034899));
#211664=CARTESIAN_POINT('Ctrl Pts',(80.6281659243945,6.60270147226842,131.000391851905));
#211665=CARTESIAN_POINT('Ctrl Pts',(80.3497183005816,3.73384805505426,125.355280541214));
#211666=CARTESIAN_POINT('Ctrl Pts',(80.0712706767688,-2.56622931613655,
124.717607618327));
#211667=CARTESIAN_POINT('Ctrl Pts',(79.7928230529558,-6.50806731306963,
129.673363347327));
#211668=CARTESIAN_POINT('Ctrl Pts',(79.514375429143,-4.46930938605503,135.668450315387));
#211669=CARTESIAN_POINT('Ctrl Pts',(79.23592780533,1.67652552884245,137.193676475141));
#211670=CARTESIAN_POINT('Ctrl Pts',(78.9574801815173,6.28171538555901,132.847433497217));
#211671=CARTESIAN_POINT('Ctrl Pts',(78.6790325577042,5.11431568180404,126.62370635255));
#211672=CARTESIAN_POINT('Ctrl Pts',(78.4005849338915,-0.752890285318027,
124.241796241119));
#211673=CARTESIAN_POINT('Ctrl Pts',(78.1221373100785,-5.92822686096799,
127.890562192549));
#211674=CARTESIAN_POINT('Ctrl Pts',(77.8436896862655,-5.65581256137084,
134.216966549603));
#211675=CARTESIAN_POINT('Ctrl Pts',(77.5652420624528,-0.185982819678218,
137.407352770183));
#211676=CARTESIAN_POINT('Ctrl Pts',(77.2867944386398,5.45475604753291,134.529911776607));
#211677=CARTESIAN_POINT('Ctrl Pts',(77.008346814827,6.08284058670873,128.228871271165));
#211678=CARTESIAN_POINT('Ctrl Pts',(76.729899191014,1.12109178998211,124.294579655415));
#211679=CARTESIAN_POINT('Ctrl Pts',(76.4514515672013,-4.8708855933594,126.342458723402));
#211680=CARTESIAN_POINT('Ctrl Pts',(76.1730039433881,-6.38675707239351,
132.4906076561));
#211681=CARTESIAN_POINT('Ctrl Pts',(75.8945563195755,-2.03351081232684,
137.089177938131));
#211682=CARTESIAN_POINT('Ctrl Pts',(75.6161086957625,4.18843254174224,135.912308132958));
#211683=CARTESIAN_POINT('Ctrl Pts',(75.3376610719495,6.56141100625526,130.041484098248));
#211684=CARTESIAN_POINT('Ctrl Pts',(75.0592134481368,2.90477329876725,124.871706316201));
#211685=CARTESIAN_POINT('Ctrl Pts',(74.7807658243238,-3.42120916422307,
125.153748010832));
#211686=CARTESIAN_POINT('Ctrl Pts',(74.5023182005109,-6.60326754065171,
130.628426643279));
#211687=CARTESIAN_POINT('Ctrl Pts',(74.223870576698,-3.71724563477466,136.264780003243));
#211688=CARTESIAN_POINT('Ctrl Pts',(73.9454229528852,2.58474341191554,136.883274704086));
#211689=CARTESIAN_POINT('Ctrl Pts',(73.6669753290721,6.51147953479087,131.915544330879));
#211690=CARTESIAN_POINT('Ctrl Pts',(73.3885277052595,4.45448406865298,125.926690409479));
#211691=CARTESIAN_POINT('Ctrl Pts',(73.1100800814464,-1.6959646429323,124.420177121874));
#211692=CARTESIAN_POINT('Ctrl Pts',(72.8316324576336,-6.28790470014163,
128.780416582107));
#211693=CARTESIAN_POINT('Ctrl Pts',(72.5531848338207,-5.1015675191428,135.000561735763));
#211694=CARTESIAN_POINT('Ctrl Pts',(72.2747372100078,0.772860986519783,
137.364603057617));
#211695=CARTESIAN_POINT('Ctrl Pts',(71.996289586195,5.93706800192887,133.700102062723));
#211696=CARTESIAN_POINT('Ctrl Pts',(71.7178419623819,5.64539956546153,127.374556144564));
#211697=CARTESIAN_POINT('Ctrl Pts',(71.4393943385692,0.165884721436248,
124.20083298183));
#211698=CARTESIAN_POINT('Ctrl Pts',(71.1609467147562,-5.46607007766984,
127.095429116077));
#211699=CARTESIAN_POINT('Ctrl Pts',(70.8824990909434,-6.07497350776591,
133.398352108815));
#211700=CARTESIAN_POINT('Ctrl Pts',(70.6040514671303,-1.10127306317963,
137.317523644624));
#211701=CARTESIAN_POINT('Ctrl Pts',(70.3256038433176,4.88444352628841,135.251416544269));
#211702=CARTESIAN_POINT('Ctrl Pts',(70.0471562195047,6.38159513342946,129.098682298033));
#211703=CARTESIAN_POINT('Ctrl Pts',(69.7687085956917,2.01437257120279,124.513383100429));
#211704=CARTESIAN_POINT('Ctrl Pts',(69.4902609718789,-4.20395997638847,
125.709184909736));
#211705=CARTESIAN_POINT('Ctrl Pts',(69.211813348066,-6.5590586805409,131.587204281367));
#211706=CARTESIAN_POINT('Ctrl Pts',(68.9333657242531,-2.88670288510633,
136.745828570004));
#211707=CARTESIAN_POINT('Ctrl Pts',(68.6549181004402,3.43839183846502,136.444534067195));
#211708=CARTESIAN_POINT('Ctrl Pts',(68.3764704766273,6.60377243726651,130.960195701968));
#211709=CARTESIAN_POINT('Ctrl Pts',(68.0980228528144,3.70060877843901,125.332652507142));
#211710=CARTESIAN_POINT('Ctrl Pts',(67.8195752290015,-2.6032335629848,124.733341757993));
#211711=CARTESIAN_POINT('Ctrl Pts',(67.5411276051886,-6.51483143505509,
129.713000755032));
#211712=CARTESIAN_POINT('Ctrl Pts',(67.2626799813758,-4.43961748551916,
135.695566149845));
#211713=CARTESIAN_POINT('Ctrl Pts',(66.9842323575627,1.71538804583728,137.183352609169));
#211714=CARTESIAN_POINT('Ctrl Pts',(66.7057847337499,6.29403576443417,132.809157059292));
#211715=CARTESIAN_POINT('Ctrl Pts',(66.4273371099371,5.08877209625689,126.592651519219));
#211716=CARTESIAN_POINT('Ctrl Pts',(66.1488894861241,-0.792824528042931,
124.246500887099));
#211717=CARTESIAN_POINT('Ctrl Pts',(65.8704418623113,-5.94585414270274,
127.92670297802));
#211718=CARTESIAN_POINT('Ctrl Pts',(65.5919942384984,-5.63493427134196,
134.251331858291));
#211719=CARTESIAN_POINT('Ctrl Pts',(65.3135466146855,-0.145785086460763,
137.408362562243));
#211720=CARTESIAN_POINT('Ctrl Pts',(65.0350989908726,5.47733347088038,134.496638102466));
#211721=CARTESIAN_POINT('Ctrl Pts',(64.7566513670597,6.06705015109826,128.191891011849));
#211722=CARTESIAN_POINT('Ctrl Pts',(64.4782037432468,1.0814441343344,124.28787586265));
#211723=CARTESIAN_POINT('Ctrl Pts',(64.199756119434,-4.89795621039988,126.37219185524));
#211724=CARTESIAN_POINT('Ctrl Pts',(63.921308495621,-6.37637407623982,132.529454416925));
#211725=CARTESIAN_POINT('Ctrl Pts',(63.6428608718081,-1.99521566920641,
137.101440052517));
#211726=CARTESIAN_POINT('Ctrl Pts',(63.3644132479953,4.21944846612332,135.886717316821));
#211727=CARTESIAN_POINT('Ctrl Pts',(63.0859656241823,6.556645592603,130.001557061437));
#211728=CARTESIAN_POINT('Ctrl Pts',(62.8075180003696,2.86860572942485,124.854134055001));
#211729=CARTESIAN_POINT('Ctrl Pts',(62.5290703765565,-3.4555426599142,125.174678574835));
#211730=CARTESIAN_POINT('Ctrl Pts',(62.2506227527437,-6.60421615743575,
130.66862586668));
#211731=CARTESIAN_POINT('Ctrl Pts',(61.9721751289308,-3.68393764016947,
136.287306763578));
#211732=CARTESIAN_POINT('Ctrl Pts',(61.6937275051179,2.62169959805353,136.867428009101));
#211733=CARTESIAN_POINT('Ctrl Pts',(61.415279881305,6.51812298281107,131.875886519111));
#211734=CARTESIAN_POINT('Ctrl Pts',(61.1368322574921,4.42470977437533,125.899665072552));
#211735=CARTESIAN_POINT('Ctrl Pts',(60.8583846336791,-1.73479555762186,
124.430619224162));
#211736=CARTESIAN_POINT('Ctrl Pts',(60.5799370098664,-6.30010852163892,
128.818730341733));
#211737=CARTESIAN_POINT('Ctrl Pts',(60.3014893860534,-5.07592953168175,
135.031538679362));
#211738=CARTESIAN_POINT('Ctrl Pts',(60.0230417622406,0.81278072494776,137.35977688733));
#211739=CARTESIAN_POINT('Ctrl Pts',(59.7445941384276,5.95458520189618,133.663907793273));
#211740=CARTESIAN_POINT('Ctrl Pts',(59.4661465146148,5.62441677596096,127.340254541386));
#211741=CARTESIAN_POINT('Ctrl Pts',(59.1876988908018,0.125684100952275,
124.199945542519));
#211742=CARTESIAN_POINT('Ctrl Pts',(58.909251266989,-5.48854612282181,127.128771354006));
#211743=CARTESIAN_POINT('Ctrl Pts',(58.6308036431761,-6.05907059010694,
133.435284136186));
#211744=CARTESIAN_POINT('Ctrl Pts',(58.3523560193632,-1.06160518713815,
137.324106732513));
#211745=CARTESIAN_POINT('Ctrl Pts',(58.0739083955504,4.91142352051418,135.221601156507));
#211746=CARTESIAN_POINT('Ctrl Pts',(57.7954607717374,6.37109394919177,129.059867319411));
#211747=CARTESIAN_POINT('Ctrl Pts',(57.5170131479246,1.97604028380464,124.501237600083));
#211748=CARTESIAN_POINT('Ctrl Pts',(57.2385655241116,-4.23489786746425,
125.734870009144));
#211749=CARTESIAN_POINT('Ctrl Pts',(56.9601179002987,-6.554171764796,131.627116628959));
#211750=CARTESIAN_POINT('Ctrl Pts',(56.6816702764859,-2.85048199937133,
136.76329066817));
#211751=CARTESIAN_POINT('Ctrl Pts',(56.4032226526729,3.47266146968847,136.423499100792));
#211752=CARTESIAN_POINT('Ctrl Pts',(56.1247750288601,6.60459869704857,130.919993777505));
#211753=CARTESIAN_POINT('Ctrl Pts',(55.8463274050471,3.66723237440476,125.310227229228));
#211754=CARTESIAN_POINT('Ctrl Pts',(55.5678797812343,-2.6401413460556,124.749300861495));
#211755=CARTESIAN_POINT('Ctrl Pts',(55.2894321574214,-6.5213541475661,129.752678603477));
#211756=CARTESIAN_POINT('Ctrl Pts',(55.0109845336085,-4.40976107332459,
135.722500738884));
#211757=CARTESIAN_POINT('Ctrl Pts',(54.7325369097956,1.75418699849736,137.172792367301));
#211758=CARTESIAN_POINT('Ctrl Pts',(54.4540892859827,6.30612291549916,132.770806332897));
#211759=CARTESIAN_POINT('Ctrl Pts',(54.1756416621698,5.06303994438864,126.561752752318));
#211760=CARTESIAN_POINT('Ctrl Pts',(53.897194038357,-0.832729392363195,
124.251448536985));
#211761=CARTESIAN_POINT('Ctrl Pts',(53.618746414544,-5.96326109862574,127.962950396153));
#211762=CARTESIAN_POINT('Ctrl Pts',(53.3402987907312,-5.61384717675129,
134.285569438194));
#211763=CARTESIAN_POINT('Ctrl Pts',(53.0618511669183,-0.105581951123662,
137.409127640582));
#211764=CARTESIAN_POINT('Ctrl Pts',(52.7834035431054,5.49970792962155,134.463227609627));
#211765=CARTESIAN_POINT('Ctrl Pts',(52.5049559192925,6.05103489871361,128.155007558556));
#211766=CARTESIAN_POINT('Ctrl Pts',(52.2265082954796,1.04175640537643,124.281413540623));
#211767=CARTESIAN_POINT('Ctrl Pts',(51.9480606716666,-4.9248453318719,126.402089222721));
#211768=CARTESIAN_POINT('Ctrl Pts',(51.6696130478539,-6.36575480119974,
132.568237253767));
#211769=CARTESIAN_POINT('Ctrl Pts',(51.3911654240409,-1.95684659263562,
137.113468826308));
#211770=CARTESIAN_POINT('Ctrl Pts',(51.112717800228,4.25030803728985,135.860938172086));
#211771=CARTESIAN_POINT('Ctrl Pts',(50.8342701764151,6.55163722003711,129.961659772806));
#211772=CARTESIAN_POINT('Ctrl Pts',(50.5558225526023,2.83233186284197,124.836782281636));
#211773=CARTESIAN_POINT('Ctrl Pts',(50.2773749287893,-3.48974810920128,
125.195817748775));
#211774=CARTESIAN_POINT('Ctrl Pts',(49.9989273049765,-6.60492005256131,
130.708830119782));
#211775=CARTESIAN_POINT('Ctrl Pts',(49.7204796811635,-3.65049313590031,
136.309630351328));
#211776=CARTESIAN_POINT('Ctrl Pts',(49.4420320573507,2.65855863614892,136.851356644924));
#211777=CARTESIAN_POINT('Ctrl Pts',(49.1635844335378,6.52452489938715,131.836189001557));
#211778=CARTESIAN_POINT('Ctrl Pts',(48.8851368097249,4.39477152084969,125.87282148092));
#211779=CARTESIAN_POINT('Ctrl Pts',(48.606689185912,-1.77356218882415,124.441297507781));
#211780=CARTESIAN_POINT('Ctrl Pts',(48.3282415620992,-6.31207889029818,
128.857117679619));
#211781=CARTESIAN_POINT('Ctrl Pts',(48.0497939382862,-5.05010345378512,
135.062358983324));
#211782=CARTESIAN_POINT('Ctrl Pts',(47.7713463144734,0.852670345487299,
137.354707803682));
#211783=CARTESIAN_POINT('Ctrl Pts',(47.4928986906604,5.97188175251911,133.627607562248));
#211784=CARTESIAN_POINT('Ctrl Pts',(47.2144510668476,5.60322557162828,127.306081301933));
#211785=CARTESIAN_POINT('Ctrl Pts',(46.9360034430346,0.0854788231980546,
124.199302832238));
#211786=CARTESIAN_POINT('Ctrl Pts',(46.6575558192218,-5.5108187878785,127.162249792247));
#211787=CARTESIAN_POINT('Ctrl Pts',(46.3791081954089,-6.04294315135938,
133.47211867372));
#211788=CARTESIAN_POINT('Ctrl Pts',(46.100660571596,-1.02189797292572,137.330448228811));
#211789=CARTESIAN_POINT('Ctrl Pts',(45.822212947783,4.93822152013526,135.191622086273));
#211790=CARTESIAN_POINT('Ctrl Pts',(45.5437653239702,6.36035668172477,129.02111698363));
#211791=CARTESIAN_POINT('Ctrl Pts',(45.2653177001572,1.9376347735074,124.489325664279));
#211792=CARTESIAN_POINT('Ctrl Pts',(44.9868700763445,-4.26567883284234,
125.76074296039));
#211793=CARTESIAN_POINT('Ctrl Pts',(44.7084224525315,-6.54904198180601,
131.666998489025));
#211794=CARTESIAN_POINT('Ctrl Pts',(44.4299748287186,-2.81415548797717,
136.780531955991));
#211795=CARTESIAN_POINT('Ctrl Pts',(44.1515272049057,3.50680242016433,136.402255915145));
#211796=CARTESIAN_POINT('Ctrl Pts',(43.8730795810928,6.60518022099696,130.879787568212));
#211797=CARTESIAN_POINT('Ctrl Pts',(43.59463195728,3.63372007972613,125.288005538446));
#211798=CARTESIAN_POINT('Ctrl Pts',(43.316184333467,-2.6769512977182,124.765484337463));
#211799=CARTESIAN_POINT('Ctrl Pts',(43.0377367096542,-6.52763520890084,
129.792395422388));
#211800=CARTESIAN_POINT('Ctrl Pts',(42.7592890858413,-4.37974125581177,
135.749253084432));
#211801=CARTESIAN_POINT('Ctrl Pts',(42.4808414620283,1.79292094911309,137.161996140853));
#211802=CARTESIAN_POINT('Ctrl Pts',(42.2023938382155,6.31797639086063,132.732382739134));
#211803=CARTESIAN_POINT('Ctrl Pts',(41.9239462144025,5.0371201797131,126.531011196811));
#211804=CARTESIAN_POINT('Ctrl Pts',(41.6454985905898,-0.872603399589798,
124.256639007436));
#211805=CARTESIAN_POINT('Ctrl Pts',(41.3670509667768,-5.98044708371573,
127.999303103786));
#211806=CARTESIAN_POINT('Ctrl Pts',(41.0886033429639,-5.592552058989,134.319678020622));
#211807=CARTESIAN_POINT('Ctrl Pts',(40.810155719151,-0.0653749034083074,
137.409647976851));
#211808=CARTESIAN_POINT('Ctrl Pts',(40.5317080953382,5.52187859466303,134.429681536124));
#211809=CARTESIAN_POINT('Ctrl Pts',(40.2532604715252,6.03479542300531,128.118222278014));
#211810=CARTESIAN_POINT('Ctrl Pts',(39.9748128477124,1.00203007375177,124.275192928799));
#211811=CARTESIAN_POINT('Ctrl Pts',(39.6963652238994,-4.95155196138904,
126.432149717987));
#211812=CARTESIAN_POINT('Ctrl Pts',(39.4179176000866,-6.35489964077443,
132.60695472951));
#211813=CARTESIAN_POINT('Ctrl Pts',(39.1394699762736,-1.91840500439501,
137.125263813774));
#211814=CARTESIAN_POINT('Ctrl Pts',(38.8610223524608,4.28101011172891,135.834971654011));
#211815=CARTESIAN_POINT('Ctrl Pts',(38.5825747286478,6.54638607414467,129.921793710766));
#211816=CARTESIAN_POINT('Ctrl Pts',(38.304127104835,2.79595304316033,124.819651639079));
#211817=CARTESIAN_POINT('Ctrl Pts',(38.0256794810221,-3.52382424458856,
125.217164749334));
#211818=CARTESIAN_POINT('Ctrl Pts',(37.7472318572093,-6.60537919994535,
130.749037912801));
#211819=CARTESIAN_POINT('Ctrl Pts',(37.4687842333963,-3.61691336126579,
136.331749939282));
#211820=CARTESIAN_POINT('Ctrl Pts',(37.1903366095834,2.69531916037638,136.835061207086));
#211821=CARTESIAN_POINT('Ctrl Pts',(36.9118889857706,6.53068504729366,131.796453249222));
#211822=CARTESIAN_POINT('Ctrl Pts',(36.6334413619576,4.36467041744916,125.846160629286));
#211823=CARTESIAN_POINT('Ctrl Pts',(36.3549937381448,-1.8122631000273,124.452211577043));
#211824=CARTESIAN_POINT('Ctrl Pts',(36.0765461143319,-6.32381536255287,
128.895577173308));
#211825=CARTESIAN_POINT('Ctrl Pts',(35.798098490519,-5.02409024244786,135.093021505591));
#211826=CARTESIAN_POINT('Ctrl Pts',(35.5196508667061,0.892528370013623,
137.34939599451));
#211827=CARTESIAN_POINT('Ctrl Pts',(35.2412032428932,5.98895701286753,133.591202714771));
#211828=CARTESIAN_POINT('Ctrl Pts',(34.9627556190803,5.58182673771145,127.272037692505));
#211829=CARTESIAN_POINT('Ctrl Pts',(34.6843079952674,0.0452703779943793,
124.198904874802));
#211830=CARTESIAN_POINT('Ctrl Pts',(34.4058603714545,-5.53288724751859,
127.195863190245));
#211831=CARTESIAN_POINT('Ctrl Pts',(34.1274127476417,-6.02659178913083,
133.508854356496));
#211832=CARTESIAN_POINT('Ctrl Pts',(33.8489651238287,-0.982152891908117,
137.336547898535));
#211833=CARTESIAN_POINT('Ctrl Pts',(33.5705175000158,4.96483653214189,135.161480444452));
#211834=CARTESIAN_POINT('Ctrl Pts',(33.292069876203,6.34938372890195,128.982432726597));
#211835=CARTESIAN_POINT('Ctrl Pts',(33.0136222523901,1.89915746344075,124.477647734417));
#211836=CARTESIAN_POINT('Ctrl Pts',(32.7351746285772,-4.29630173192265,
125.786802804744));
#211837=CARTESIAN_POINT('Ctrl Pts',(32.4567270047643,-6.543669521657,131.706848383727));
#211838=CARTESIAN_POINT('Ctrl Pts',(32.1782793809514,-2.77772469701646,
136.797551794587));
#211839=CARTESIAN_POINT('Ctrl Pts',(31.8998317571386,3.54081342478663,136.380805297429));
#211840=CARTESIAN_POINT('Ctrl Pts',(31.6213841333256,6.60551698756319,130.839578563946));
#211841=CARTESIAN_POINT('Ctrl Pts',(31.3429365095127,3.6000731362139,125.26598825823));
#211842=CARTESIAN_POINT('Ctrl Pts',(31.0644888856998,-2.71366205396602,
124.781891586214));
#211843=CARTESIAN_POINT('Ctrl Pts',(30.7860412618869,-6.53367438631237,
129.83214974004));
#211844=CARTESIAN_POINT('Ctrl Pts',(30.507593638074,-4.34955914537615,135.775822195171));
#211845=CARTESIAN_POINT('Ctrl Pts',(30.2291460142612,1.83158846238341,137.150964329883));
#211846=CARTESIAN_POINT('Ctrl Pts',(29.9506983904483,6.32959575128355,132.693887701803));
#211847=CARTESIAN_POINT('Ctrl Pts',(29.6722507666353,5.01101376269691,126.500427991838));
#211848=CARTESIAN_POINT('Ctrl Pts',(29.3938031428225,-0.912445072176531,
124.26207210612));
#211849=CARTESIAN_POINT('Ctrl Pts',(29.1153555190096,-5.99741146113971,
128.035759753857));
#211850=CARTESIAN_POINT('Ctrl Pts',(28.8369078951967,-5.57104970715349,
134.353656341672));
#211851=CARTESIAN_POINT('Ctrl Pts',(28.5584602713837,-0.0251654332018655,
137.409923551768));
#211852=CARTESIAN_POINT('Ctrl Pts',(28.280012647571,5.54384464446253,134.396001125022));
#211853=CARTESIAN_POINT('Ctrl Pts',(28.001565023758,6.0183323257333,128.081536533317));
#211854=CARTESIAN_POINT('Ctrl Pts',(27.7231173999451,0.962266611534229,
124.269214257685));
#211855=CARTESIAN_POINT('Ctrl Pts',(27.4446697761322,-4.97807510932732,
126.462372227135));
#211856=CARTESIAN_POINT('Ctrl Pts',(27.1662221523194,-6.34380899720599,
132.645605409466));
#211857=CARTESIAN_POINT('Ctrl Pts',(26.8877745285064,-1.87989232895117,
137.136824577849));
#211858=CARTESIAN_POINT('Ctrl Pts',(26.6093269046936,4.31155355176403,135.808818724794));
#211859=CARTESIAN_POINT('Ctrl Pts',(26.3308792808807,6.5408923495088,129.881960352566));
#211860=CARTESIAN_POINT('Ctrl Pts',(26.0524316570678,2.75947061841045,124.802742762115));
#211861=CARTESIAN_POINT('Ctrl Pts',(25.7739840332549,-3.55776980337282,
125.238718785491));
#211862=CARTESIAN_POINT('Ctrl Pts',(25.4955364094419,-6.60559358257403,
130.789247755823));
#211863=CARTESIAN_POINT('Ctrl Pts',(25.2170887856292,-3.58319956057628,
136.353664707793));
#211864=CARTESIAN_POINT('Ctrl Pts',(24.9386411618162,2.73197980856112,136.81854229942));
#211865=CARTESIAN_POINT('Ctrl Pts',(24.6601935380033,6.5366031982641,131.756680734531));
#211866=CARTESIAN_POINT('Ctrl Pts',(24.3817459141905,4.3344075795813,125.819683505575));
#211867=CARTESIAN_POINT('Ctrl Pts',(24.1032982903775,-1.85089685715453,
124.463361027524));
#211868=CARTESIAN_POINT('Ctrl Pts',(23.8248506665647,-6.33531750350378,
128.934107397669));
#211869=CARTESIAN_POINT('Ctrl Pts',(23.5464030427517,-4.99789086159903,
135.123525109951));
#211870=CARTESIAN_POINT('Ctrl Pts',(23.2679554189389,0.932353321572971,
137.343841656646));
#211871=CARTESIAN_POINT('Ctrl Pts',(22.9895077951259,6.00581035021119,133.554694599836));
#211872=CARTESIAN_POINT('Ctrl Pts',(22.7110601713131,5.56022106715229,127.238124974604));
#211873=CARTESIAN_POINT('Ctrl Pts',(22.4326125475002,0.00506025528043594,
124.198751684957));
#211874=CARTESIAN_POINT('Ctrl Pts',(22.1541649236873,-5.554750683987,127.229610302442));
#211875=CARTESIAN_POINT('Ctrl Pts',(21.8757172998744,-6.01001710932725,
133.545489823263));
#211876=CARTESIAN_POINT('Ctrl Pts',(21.5972696760615,-0.942371416853923,
137.342405515655));
#211877=CARTESIAN_POINT('Ctrl Pts',(21.3188220522486,4.99126757030501,135.131177347952));
#211878=CARTESIAN_POINT('Ctrl Pts',(21.0403744284357,6.33817549733007,128.943815981773));
#211879=CARTESIAN_POINT('Ctrl Pts',(20.7619268046228,1.86060977939589,124.466204243228));
#211880=CARTESIAN_POINT('Ctrl Pts',(20.48347918081,-4.32676542996233,125.813048576547));
#211881=CARTESIAN_POINT('Ctrl Pts',(20.205031556997,-6.5380545834274,131.746664836412));
#211882=CARTESIAN_POINT('Ctrl Pts',(19.9265839331841,-2.74119097644563,
136.814349553278));
#211883=CARTESIAN_POINT('Ctrl Pts',(19.6481363093713,3.57469322326559,136.359148042506));
#211884=CARTESIAN_POINT('Ctrl Pts',(19.3696886855584,6.60560898426828,130.799368254665));
#211885=CARTESIAN_POINT('Ctrl Pts',(19.0912410617455,3.56629279066743,125.244176204439));
#211886=CARTESIAN_POINT('Ctrl Pts',(18.8127934379326,-2.75027225446848,
124.798521999768));
#211887=CARTESIAN_POINT('Ctrl Pts',(18.5343458141197,-6.53947145601676,
129.871940083324));
#211888=CARTESIAN_POINT('Ctrl Pts',(18.2558981903068,-4.31921586042675,
135.802207086573));
#211889=CARTESIAN_POINT('Ctrl Pts',(17.9774505664939,1.87018810546999,137.139697343177));
#211890=CARTESIAN_POINT('Ctrl Pts',(17.6990029426811,6.34098056620813,132.65532264735));
#211891=CARTESIAN_POINT('Ctrl Pts',(17.4205553188681,4.98472166072295,126.470004270672));
#211892=CARTESIAN_POINT('Ctrl Pts',(17.1421076950552,-0.95225293377558,
124.26774763171));
#211893=CARTESIAN_POINT('Ctrl Pts',(16.8636600712423,-6.01415360227624,
128.072318995452));
#211894=CARTESIAN_POINT('Ctrl Pts',(16.5852124474295,-5.54934091802252,
134.387503142263));
#211895=CARTESIAN_POINT('Ctrl Pts',(16.3067648236166,0.0150449695187284,
137.409954355121));
#211896=CARTESIAN_POINT('Ctrl Pts',(16.0283171998036,5.56560526505998,134.362187624359));
#211897=CARTESIAN_POINT('Ctrl Pts',(15.7498695759908,6.00164621694371,128.044951683866));
#211898=CARTESIAN_POINT('Ctrl Pts',(15.4714219521779,0.922467492173741,
124.263477748823));
#211899=CARTESIAN_POINT('Ctrl Pts',(15.192974328365,-5.00441379286154,126.492755630261));
#211900=CARTESIAN_POINT('Ctrl Pts',(14.9145267045521,-6.33248328146239,
132.684187861418));
#211901=CARTESIAN_POINT('Ctrl Pts',(14.6360790807393,-1.84130999340576,
137.148150690142));
#211902=CARTESIAN_POINT('Ctrl Pts',(14.3576314569263,4.34193722559672,135.782480353541));
#211903=CARTESIAN_POINT('Ctrl Pts',(14.0791838331134,6.53515624970152,129.842161174248));
#211904=CARTESIAN_POINT('Ctrl Pts',(13.8007362093005,2.72288594046203,124.786056277307));
#211905=CARTESIAN_POINT('Ctrl Pts',(13.5222885854877,-3.59158352768866,
125.260479058552));
#211906=CARTESIAN_POINT('Ctrl Pts',(13.2438409616747,-6.60556319250329,
130.829458158858));
#211907=CARTESIAN_POINT('Ctrl Pts',(12.9653933378619,-3.54935298310934,
136.375373844801));
#211908=CARTESIAN_POINT('Ctrl Pts',(12.686945714049,2.76853922222938,136.801800534039));
#211909=CARTESIAN_POINT('Ctrl Pts',(12.4084980902361,6.5422791329992,131.716872931266));
#211910=CARTESIAN_POINT('Ctrl Pts',(12.1300504664232,4.30398412864651,125.793391090908));
#211911=CARTESIAN_POINT('Ctrl Pts',(11.8516028426103,-1.88946202861834,
124.474745446076));
#211912=CARTESIAN_POINT('Ctrl Pts',(11.5731552187974,-6.34658488693473,
128.972706924952));
#211913=CARTESIAN_POINT('Ctrl Pts',(11.2947075949845,-4.97150628206636,
135.153868666082));
#211914=CARTESIAN_POINT('Ctrl Pts',(11.0162599711716,0.972143724437105,
137.338044995907));
#211915=CARTESIAN_POINT('Ctrl Pts',(10.7378123473587,6.0224411400439,133.518084570262));
#211916=CARTESIAN_POINT('Ctrl Pts',(10.4593647235458,5.53840936055655,127.204344404875));
#211917=CARTESIAN_POINT('Ctrl Pts',(10.1809170997329,-0.0351500549433496,
124.198843268382));
#211918=CARTESIAN_POINT('Ctrl Pts',(9.90246947592002,-5.57640828712608,
127.263489878326));
#211919=CARTESIAN_POINT('Ctrl Pts',(9.62402185210712,-5.99321972612948,
133.582023716479));
#211920=CARTESIAN_POINT('Ctrl Pts',(9.34557422829421,-0.902555021880531,
137.348020863117));
#211921=CARTESIAN_POINT('Ctrl Pts',(9.06712660448133,5.01751365521256,135.100713919668));
#211922=CARTESIAN_POINT('Ctrl Pts',(8.78867898066847,6.32673240233446,128.905268180115));
#211923=CARTESIAN_POINT('Ctrl Pts',(8.51023135685555,1.82199314977141,124.454995614755));
#211924=CARTESIAN_POINT('Ctrl Pts',(8.23178373304265,-4.35706879811783,
125.839479303254));
#211925=CARTESIAN_POINT('Ctrl Pts',(7.9533361092298,-6.53219737518076,131.786446371669));
#211926=CARTESIAN_POINT('Ctrl Pts',(7.67488848541689,-2.70455568003535,
136.83092460962));
#211927=CARTESIAN_POINT('Ctrl Pts',(7.39644086160398,3.60844056017245,136.337284952891));
#211928=CARTESIAN_POINT('Ctrl Pts',(7.1179932377911,6.60545620770325,130.759158130379));
#211929=CARTESIAN_POINT('Ctrl Pts',(6.83954561397822,3.53238029483008,125.222570185327));
#211930=CARTESIAN_POINT('Ctrl Pts',(6.5610979901653,-2.78678054262086,124.815374961881));
#211931=CARTESIAN_POINT('Ctrl Pts',(6.28265036635242,-6.54502620320144,
129.911764977794));
#211932=CARTESIAN_POINT('Ctrl Pts',(6.00420274253956,-4.28871252534551,
135.828406780936));
#211933=CARTESIAN_POINT('Ctrl Pts',(5.72575511872663,1.90871844804856,137.128195598241));
#211934=CARTESIAN_POINT('Ctrl Pts',(5.44730749491374,6.35213041376593,132.616689004818));
#211935=CARTESIAN_POINT('Ctrl Pts',(5.16885987110085,4.95824484805471,126.439741160674));
#211936=CARTESIAN_POINT('Ctrl Pts',(4.89041224728798,-0.992025509291961,
124.273665373899));
#211937=CARTESIAN_POINT('Ctrl Pts',(4.61196462347505,-6.03067288673954,
128.108979473854));
#211938=CARTESIAN_POINT('Ctrl Pts',(4.33351699966218,-5.52742649602286,
134.421217168191));
#211939=CARTESIAN_POINT('Ctrl Pts',(4.05506937584931,0.0552548147426717,
137.409740385768));
#211940=CARTESIAN_POINT('Ctrl Pts',(3.77662175203639,5.58715965010757,134.328242287108));
#211941=CARTESIAN_POINT('Ctrl Pts',(3.49817412822347,5.98473771494644,128.008469085329));
#211942=CARTESIAN_POINT('Ctrl Pts',(3.21972650441063,0.882634190440881,
124.25798361478));
#211943=CARTESIAN_POINT('Ctrl Pts',(2.94127888059773,-5.03056703600248,
126.523298801495));
#211944=CARTESIAN_POINT('Ctrl Pts',(2.66283125678483,-6.32092291322184,
132.722700655682));
#211945=CARTESIAN_POINT('Ctrl Pts',(2.38438363297192,-1.80265942744139,
137.159241730961));
#211946=CARTESIAN_POINT('Ctrl Pts',(2.10593600915906,4.37216000734877,135.755957516231));
#211947=CARTESIAN_POINT('Ctrl Pts',(1.82748838534615,6.529177987276,129.802397650584));
#211948=CARTESIAN_POINT('Ctrl Pts',(1.54904076153325,2.68620036497402,124.769592802981));
#211949=CARTESIAN_POINT('Ctrl Pts',(1.27059313772038,-3.62526416455594,
125.282444762183));
#211950=CARTESIAN_POINT('Ctrl Pts',(0.992145513907496,-6.60528803085927,
130.869667631896));
#211951=CARTESIAN_POINT('Ctrl Pts',(0.713697890094564,-3.51537488306232,
136.396876545864));
#211952=CARTESIAN_POINT('Ctrl Pts',(0.435250266281723,2.80499604665836,
136.784836531317));
#211953=CARTESIAN_POINT('Ctrl Pts',(0.156802642468823,6.54771264117505,
131.677031314524));
#211954=CARTESIAN_POINT('Ctrl Pts',(-0.121644981344083,4.27340119199728,
125.767284359559));
#211955=CARTESIAN_POINT('Ctrl Pts',(-0.400092605156985,-1.92795718537184,
124.486364410847));
#211956=CARTESIAN_POINT('Ctrl Pts',(-0.678540228969845,-6.35761709532873,
129.011374324836));
#211957=CARTESIAN_POINT('Ctrl Pts',(-0.956987852782752,-4.94493748154019,
135.184051049593));
#211958=CARTESIAN_POINT('Ctrl Pts',(-1.23543547659566,1.01189810415772,
137.332006227089));
#211959=CARTESIAN_POINT('Ctrl Pts',(-1.51388310040852,6.03884876610542,
133.48137398265));
#211960=CARTESIAN_POINT('Ctrl Pts',(-1.79233072422142,5.51639242616521,
127.170697235071));
#211961=CARTESIAN_POINT('Ctrl Pts',(-2.07077834803434,-0.0753590626689394,
124.19917962168));
#211962=CARTESIAN_POINT('Ctrl Pts',(-2.34922597184723,-5.59785925440532,
127.297500662476));
#211963=CARTESIAN_POINT('Ctrl Pts',(-2.6276735956601,-5.97620026197078,
133.618454682368));
#211964=CARTESIAN_POINT('Ctrl Pts',(-2.906121219473,-0.862705182398668,
137.353393732843));
#211965=CARTESIAN_POINT('Ctrl Pts',(-3.18456884328591,5.04357381430661,
135.070091288433));
#211966=CARTESIAN_POINT('Ctrl Pts',(-3.46301646709877,6.31505486794284,
128.866790750024));
#211967=CARTESIAN_POINT('Ctrl Pts',(-3.74146409091167,1.78330900552073,
124.444022264336));
#211968=CARTESIAN_POINT('Ctrl Pts',(-4.01991171472458,-4.38721071348669,
125.866094005463));
#211969=CARTESIAN_POINT('Ctrl Pts',(-4.29835933853748,-6.52609811395827,
131.826191515377));
#211970=CARTESIAN_POINT('Ctrl Pts',(-4.57680696235032,-2.66782016531947,
136.847276349416));
#211971=CARTESIAN_POINT('Ctrl Pts',(-4.85525458616324,3.64205418498746,
136.31521683873));
#211972=CARTESIAN_POINT('Ctrl Pts',(-5.13370220997616,6.60505866352928,
130.718949681087));
#211973=CARTESIAN_POINT('Ctrl Pts',(-5.41214983378902,3.49833690534187,
125.201171001511));
#211974=CARTESIAN_POINT('Ctrl Pts',(-5.69059745760191,-2.82318556559566,
124.832449848059));
#211975=CARTESIAN_POINT('Ctrl Pts',(-5.96904508141481,-6.55033842203324,
129.951622947723));
#211976=CARTESIAN_POINT('Ctrl Pts',(-6.24749270522772,-4.2580502704442,
135.854420307421));
#211977=CARTESIAN_POINT('Ctrl Pts',(-6.52594032904057,1.9471780623631,137.116459521273));
#211978=CARTESIAN_POINT('Ctrl Pts',(-6.80438795285348,6.36304488079526,
132.577988205793));
#211979=CARTESIAN_POINT('Ctrl Pts',(-7.0828355766664,4.93158430580029,126.409639783256));
#211980=CARTESIAN_POINT('Ctrl Pts',(-7.36128320047925,-1.03176132493798,
124.279825113401));
#211981=CARTESIAN_POINT('Ctrl Pts',(-7.63973082429214,-6.04696870240127,
128.145739830595));
#211982=CARTESIAN_POINT('Ctrl Pts',(-7.91817844810507,-5.50530725320171,
134.454797170168));
#211983=CARTESIAN_POINT('Ctrl Pts',(-8.19662607191793,0.09546261247915,
137.40928165164));
#211984=CARTESIAN_POINT('Ctrl Pts',(-8.47507369573082,5.60850700089942,
134.294166371127));
#211985=CARTESIAN_POINT('Ctrl Pts',(-8.75352131954372,5.96760744629241,
127.972090089581));
#211986=CARTESIAN_POINT('Ctrl Pts',(-9.03196894335663,0.842768182373745,
124.252732059145));
#211987=CARTESIAN_POINT('Ctrl Pts',(-9.31041656716948,-5.05653386963193,
126.554000609049));
#211988=CARTESIAN_POINT('Ctrl Pts',(-9.5888641909824,-6.30912832085822,
132.76114236515));
#211989=CARTESIAN_POINT('Ctrl Pts',(-9.86731181479532,-1.76394206326903,
137.170097289323));
#211990=CARTESIAN_POINT('Ctrl Pts',(-10.1457594386081,4.40222077710389,
135.729251195677));
#211991=CARTESIAN_POINT('Ctrl Pts',(-10.424207062421,6.52295778375913,129.762671255026));
#211992=CARTESIAN_POINT('Ctrl Pts',(-10.7026546862339,2.64941525134336,
124.753352949195));
#211993=CARTESIAN_POINT('Ctrl Pts',(-10.9811023100469,-3.65881046592654,
125.304615082438));
#211994=CARTESIAN_POINT('Ctrl Pts',(-11.2595499338597,-6.60476810783814,
130.909874684957));
#211995=CARTESIAN_POINT('Ctrl Pts',(-11.5379975576726,-3.48126651950624,
136.418172014193));
#211996=CARTESIAN_POINT('Ctrl Pts',(-11.8164451814855,2.84134893092756,
136.767650919861));
#211997=CARTESIAN_POINT('Ctrl Pts',(-12.0948928052984,6.5529035214511,131.637157360647));
#211998=CARTESIAN_POINT('Ctrl Pts',(-12.3733404291112,4.2426599028951,125.741364278924));
#211999=CARTESIAN_POINT('Ctrl Pts',(-12.6517880529242,-1.96638090096281,
124.498217491291));
#212000=CARTESIAN_POINT('Ctrl Pts',(-12.9302356767371,-6.36841371988325,
129.050108164486));
#212001=CARTESIAN_POINT('Ctrl Pts',(-13.2086833005499,-4.91818544453708,
135.214071142064));
#212002=CARTESIAN_POINT('Ctrl Pts',(-13.4871309243628,1.05161498762227,
137.325725573964));
#212003=CARTESIAN_POINT('Ctrl Pts',(-13.7655785481758,6.05503262040511,
133.444564197323));
#212004=CARTESIAN_POINT('Ctrl Pts',(-14.0440261719886,5.49417107982388,
127.137184712));
#212005=CARTESIAN_POINT('Ctrl Pts',(-14.3224737958015,-0.115565277936756,
124.199760732389));
#212006=CARTESIAN_POINT('Ctrl Pts',(-14.6009214196144,-5.61910279095105,
127.331641394614));
#212007=CARTESIAN_POINT('Ctrl Pts',(-14.8793690434273,-5.95895934751375,
133.654781370965));
#212008=CARTESIAN_POINT('Ctrl Pts',(-15.1578166672402,-0.822823375059262,
137.358523925738));
#212009=CARTESIAN_POINT('Ctrl Pts',(-15.4362642910531,5.06944708191823,
135.039310588977));
#212010=CARTESIAN_POINT('Ctrl Pts',(-15.714711914866,6.3031433268707,128.828385117298));
#212011=CARTESIAN_POINT('Ctrl Pts',(-15.9931595386788,1.74455878009922,
124.433284598595));
#212012=CARTESIAN_POINT('Ctrl Pts',(-16.2716071624918,-4.41719005914895,
125.892891696959));
#212013=CARTESIAN_POINT('Ctrl Pts',(-16.5500547863046,-6.51975702577033,
131.865898794765));
#212014=CARTESIAN_POINT('Ctrl Pts',(-16.8285024101176,-2.63098579354628,
136.863404166748));
#212015=CARTESIAN_POINT('Ctrl Pts',(-17.1069500339304,3.67553285214529,
136.292944517765));
#212016=CARTESIAN_POINT('Ctrl Pts',(-17.3853976577434,6.60441636647752,
130.678744396729));
#212017=CARTESIAN_POINT('Ctrl Pts',(-17.6638452815562,3.46416388369313,
125.179979445948));
#212018=CARTESIAN_POINT('Ctrl Pts',(-17.9422929053691,-2.8594859743911,
124.849746025587));
#212019=CARTESIAN_POINT('Ctrl Pts',(-18.220740529182,-6.55540791566593,
129.991512516161));
#212020=CARTESIAN_POINT('Ctrl Pts',(-18.4991881529949,-4.22723023192423,
135.880246702087));
#212021=CARTESIAN_POINT('Ctrl Pts',(-18.7776357768078,1.98556552327847,
137.104489547159));
#212022=CARTESIAN_POINT('Ctrl Pts',(-19.0560834006207,6.37372356285652,
132.539221684343));
#212023=CARTESIAN_POINT('Ctrl Pts',(-19.3345310244336,4.90474102187576,
126.379701253833));
#212024=CARTESIAN_POINT('Ctrl Pts',(-19.6129786482465,-1.07145890828896,
124.286226621967));
#212025=CARTESIAN_POINT('Ctrl Pts',(-19.8914262720594,-6.06304044541393,
128.182598703507));
#212026=CARTESIAN_POINT('Ctrl Pts',(-20.1698738958722,-5.48298400919569,
134.488241903877));
#212027=CARTESIAN_POINT('Ctrl Pts',(-20.4483215196851,0.135666872813404,
137.408578169733));
#212028=CARTESIAN_POINT('Ctrl Pts',(-20.7267691434981,5.62964652640204,
134.25996113911));
#212029=CARTESIAN_POINT('Ctrl Pts',(-21.0052167673109,5.95025604574973,
127.935816044659));
#212030=CARTESIAN_POINT('Ctrl Pts',(-21.2836643911238,0.802870945221437,
124.247723276515));
#212031=CARTESIAN_POINT('Ctrl Pts',(-21.5621120149367,-5.08231333153929,
126.584859915257));
#212032=CARTESIAN_POINT('Ctrl Pts',(-21.8405596387496,-6.29709994142449,
132.79951156535));
#212033=CARTESIAN_POINT('Ctrl Pts',(-22.1190072625625,-1.725159335575,137.180716962973));
#212034=CARTESIAN_POINT('Ctrl Pts',(-22.3974548863754,4.43211842094896,
135.702362381491));
#212035=CARTESIAN_POINT('Ctrl Pts',(-22.6759025101882,6.51649586964294,
129.722983459651));
#212036=CARTESIAN_POINT('Ctrl Pts',(-22.9543501340012,2.61253196265622,
124.737337317723));
#212037=CARTESIAN_POINT('Ctrl Pts',(-23.232797757814,-3.6922211887298,125.326989197785));
#212038=CARTESIAN_POINT('Ctrl Pts',(-23.511245381627,-6.60400344270576,
130.950077828156));
#212039=CARTESIAN_POINT('Ctrl Pts',(-23.7896930054398,-3.4470291563393,
136.439259460675));
#212040=CARTESIAN_POINT('Ctrl Pts',(-24.0681406292527,2.87759652796706,
136.75024433649));
#212041=CARTESIAN_POINT('Ctrl Pts',(-24.3465882530656,6.55785158147733,
131.597252547181));
#212042=CARTESIAN_POINT('Ctrl Pts',(-24.6250358768785,4.21176140046998,
125.715631809479));
#212043=CARTESIAN_POINT('Ctrl Pts',(-24.9034835006914,-2.00473175158637,
124.510304248187));
#212044=CARTESIAN_POINT('Ctrl Pts',(-25.1819311245043,-6.3789743605254,
129.088907008606));
#212045=CARTESIAN_POINT('Ctrl Pts',(-25.4603787483172,-4.89125116236366,
135.24392783109));
#212046=CARTESIAN_POINT('Ctrl Pts',(-25.73882637213,1.09129290310671,137.319203269261));
#212047=CARTESIAN_POINT('Ctrl Pts',(-26.017273995943,6.07099210324431,133.407656578282));
#212048=CARTESIAN_POINT('Ctrl Pts',(-26.2957216197559,5.47174614495268,
127.103808077481));
#212049=CARTESIAN_POINT('Ctrl Pts',(-26.5741692435687,-0.155767210890682,
124.200586578976));
#212050=CARTESIAN_POINT('Ctrl Pts',(-26.8526168673816,-5.64013810957666,
127.365910809639));
#212051=CARTESIAN_POINT('Ctrl Pts',(-27.1310644911945,-5.94149762162655,
133.691002436174));
#212052=CARTESIAN_POINT('Ctrl Pts',(-27.4095121150075,-0.782911077696857,
137.363411251701));
#212053=CARTESIAN_POINT('Ctrl Pts',(-27.6879597388203,5.09513249930392,
135.008372961895));
#212054=CARTESIAN_POINT('Ctrl Pts',(-27.9664073626332,6.29099822050462,
128.79005270507));
#212055=CARTESIAN_POINT('Ctrl Pts',(-28.2448549864461,1.70574390941038,
124.422783015417));
#212056=CARTESIAN_POINT('Ctrl Pts',(-28.523302610259,-4.44700572420938,
125.919871384741));
#212057=CARTESIAN_POINT('Ctrl Pts',(-28.8017502340719,-6.51317434558802,
131.905566738465));
#212058=CARTESIAN_POINT('Ctrl Pts',(-29.0801978578848,-2.59405392962697,
136.879307463993));
#212059=CARTESIAN_POINT('Ctrl Pts',(-29.3586454816977,3.7088753210816,136.270468815306));
#212060=CARTESIAN_POINT('Ctrl Pts',(-29.6370931055106,6.6035293403484,130.638543767126));
#212061=CARTESIAN_POINT('Ctrl Pts',(-29.9155407293234,3.42986249617799,
125.158996303897));
#212062=CARTESIAN_POINT('Ctrl Pts',(-30.1939883531365,-2.89568042388203,
124.86726285355));
#212063=CARTESIAN_POINT('Ctrl Pts',(-30.4724359769491,-6.56023449624756,
130.031432204983));
#212064=CARTESIAN_POINT('Ctrl Pts',(-30.7508836007622,-4.19625355183344,
135.905885007927));
#212065=CARTESIAN_POINT('Ctrl Pts',(-31.029331224575,2.02387940833292,137.092286119451));
#212066=CARTESIAN_POINT('Ctrl Pts',(-31.3077788483879,6.38416606424714,
132.50039087698));
#212067=CARTESIAN_POINT('Ctrl Pts',(-31.5862264722008,4.8777159909692,126.349926681791));
#212068=CARTESIAN_POINT('Ctrl Pts',(-31.8646740960137,-1.11111678833609,
124.292869662384));
#212069=CARTESIAN_POINT('Ctrl Pts',(-32.1431217198266,-6.07888752023319,
128.219554726771));
#212070=CARTESIAN_POINT('Ctrl Pts',(-32.4215693436394,-5.46045759120085,
134.52155013001));
#212071=CARTESIAN_POINT('Ctrl Pts',(-32.7000169674524,0.175866105961793,
137.407629966116));
#212072=CARTESIAN_POINT('Ctrl Pts',(-32.9784645912652,5.65057744328232,
134.225627858545));
#212073=CARTESIAN_POINT('Ctrl Pts',(-33.2569122150782,5.93268415628106,
127.89964829471));
#212074=CARTESIAN_POINT('Ctrl Pts',(-33.535359838891,0.762943957391,124.242957452493));
#212075=CARTESIAN_POINT('Ctrl Pts',(-33.813807462704,-5.10790446645711,
126.615875576613));
#212076=CARTESIAN_POINT('Ctrl Pts',(-34.0922550865168,-6.28483822063666,
132.837806834499));
#212077=CARTESIAN_POINT('Ctrl Pts',(-34.3707027103298,-1.68631268146717,
137.191100358392));
#212078=CARTESIAN_POINT('Ctrl Pts',(-34.6491503341426,4.46185183101625,
135.675292070049));
#212079=CARTESIAN_POINT('Ctrl Pts',(-34.9275979579556,6.5097924843757,129.683335735103));
#212080=CARTESIAN_POINT('Ctrl Pts',(-35.2060455817684,2.57555186563646,
124.721546502031));
#212081=CARTESIAN_POINT('Ctrl Pts',(-35.4844932055813,-3.72549509491909,
125.349566279145));
#212082=CARTESIAN_POINT('Ctrl Pts',(-35.7629408293942,-6.60299406379731,
130.990275571749));
#212083=CARTESIAN_POINT('Ctrl Pts',(-36.0413884532071,-3.41266406223907,
136.460138103909));
#212084=CARTESIAN_POINT('Ctrl Pts',(-36.3198360770199,2.91373749460914,
136.73261742621));
#212085=CARTESIAN_POINT('Ctrl Pts',(-36.5982837008328,6.56255663790157,
131.557318352812));
#212086=CARTESIAN_POINT('Ctrl Pts',(-36.8767313246458,4.18070682967726,
125.690087904753));
#212087=CARTESIAN_POINT('Ctrl Pts',(-37.1551789484586,-2.04300831613737,
124.522624233657));
#212088=CARTESIAN_POINT('Ctrl Pts',(-37.4336265722715,-6.38929862592666,
129.12776941949));
#212089=CARTESIAN_POINT('Ctrl Pts',(-37.7120741960844,-4.86413563307991,
135.273620010322));
#212090=CARTESIAN_POINT('Ctrl Pts',(-37.9905218198973,1.13093038033133,
137.312439554669));
#212091=CARTESIAN_POINT('Ctrl Pts',(-38.2689694437102,6.0867266232385,133.370652493151));
#212092=CARTESIAN_POINT('Ctrl Pts',(-38.5474170675231,5.44911845251588,
127.070568568297));
#212093=CARTESIAN_POINT('Ctrl Pts',(-38.825864691336,-0.195963371833029,
124.201657130839));
#212094=CARTESIAN_POINT('Ctrl Pts',(-39.1043123151489,-5.66096443081045,
127.400307637685));
#212095=CARTESIAN_POINT('Ctrl Pts',(-39.3827599389617,-5.92381573136,133.727116535809));
#212096=CARTESIAN_POINT('Ctrl Pts',(-39.6612075627747,-0.742969769276543,
137.368055529631));
#212097=CARTESIAN_POINT('Ctrl Pts',(-39.9396551865875,5.12062911468111,
134.977279553588));
#212098=CARTESIAN_POINT('Ctrl Pts',(-40.2181028104005,6.27861999888597,
128.751794933764));
#212099=CARTESIAN_POINT('Ctrl Pts',(-40.4965504342133,1.66686583175366,
124.412517903944));
#212100=CARTESIAN_POINT('Ctrl Pts',(-40.7749980580263,-4.47665660383728,
125.947032069068));
#212101=CARTESIAN_POINT('Ctrl Pts',(-41.0534456818391,-6.5063503173351,
131.945193876568));
#212102=CARTESIAN_POINT('Ctrl Pts',(-41.3318933056519,-2.55702594208532,
136.894985651848));
#212103=CARTESIAN_POINT('Ctrl Pts',(-41.6103409294649,3.74208035627896,
136.247790564197));
#212104=CARTESIAN_POINT('Ctrl Pts',(-41.8887885532778,6.60239761801125,
130.598349281928));
#212105=CARTESIAN_POINT('Ctrl Pts',(-42.1672361770906,3.39543401384647,
125.138222352896));
#212106=CARTESIAN_POINT('Ctrl Pts',(-42.4456838009036,-2.93176757287012,
124.884999682853));
#212107=CARTESIAN_POINT('Ctrl Pts',(-42.7241314247165,-6.56481798492739,
130.071380534953));
#212108=CARTESIAN_POINT('Ctrl Pts',(-43.0025790485293,-4.16512137802412,
135.931334274905));
#212109=CARTESIAN_POINT('Ctrl Pts',(-43.2810266723423,2.06211829779186,
137.079849690351));
#212110=CARTESIAN_POINT('Ctrl Pts',(-43.5594742961552,6.39437199801655,
132.461497222591));
#212111=CARTESIAN_POINT('Ctrl Pts',(-43.837921919968,4.85051021450257,126.320317170437));
#212112=CARTESIAN_POINT('Ctrl Pts',(-44.116369543781,-1.150733495542,124.299753988494));
#212113=CARTESIAN_POINT('Ctrl Pts',(-44.3948171675938,-6.09450933963988,
128.256606530968));
#212114=CARTESIAN_POINT('Ctrl Pts',(-44.6732647914067,-5.43772883394191,
134.554720614319));
#212115=CARTESIAN_POINT('Ctrl Pts',(-44.9517124152196,0.216058822326645,
137.406437075925));
#212116=CARTESIAN_POINT('Ctrl Pts',(-45.2301600390324,5.67129897593744,
134.191167801664));
#212117=CARTESIAN_POINT('Ctrl Pts',(-45.5086076628454,5.91489242901924,
127.863588179946));
#212118=CARTESIAN_POINT('Ctrl Pts',(-45.7870552866582,0.722988698391639,
124.238434763679));
#212119=CARTESIAN_POINT('Ctrl Pts',(-46.0655029104712,-5.13330632609627,
126.647046443824));
#212120=CARTESIAN_POINT('Ctrl Pts',(-46.343950534284,-6.27234361285742,
132.876026753548));
#212121=CARTESIAN_POINT('Ctrl Pts',(-46.622398158097,-1.64740354042306,
137.201247090823));
#212122=CARTESIAN_POINT('Ctrl Pts',(-46.9008457819097,4.49141990552312,
135.64804126445));
#212123=CARTESIAN_POINT('Ctrl Pts',(-47.1792934057228,6.50284787635396,
129.643729550545));
#212124=CARTESIAN_POINT('Ctrl Pts',(-47.4577410295356,2.53847633059532,
124.705981087252));
#212125=CARTESIAN_POINT('Ctrl Pts',(-47.7361886533485,-3.75863095151733,
125.372345489915));
#212126=CARTESIAN_POINT('Ctrl Pts',(-48.0146362771614,-6.60174000851572,
131.030466426196));
#212127=CARTESIAN_POINT('Ctrl Pts',(-48.2930839009743,-3.37817251061699,
136.480807170229));
#212128=CARTESIAN_POINT('Ctrl Pts',(-48.5715315247872,2.94977049163681,
136.714770842195));
#212129=CARTESIAN_POINT('Ctrl Pts',(-48.8499791486,6.56701851637621,131.517356257317));
#212130=CARTESIAN_POINT('Ctrl Pts',(-49.128426772413,4.14949734125552,125.664733511282));
#212131=CARTESIAN_POINT('Ctrl Pts',(-49.4068743962258,-2.08120917626415,
124.535176991179));
#212132=CARTESIAN_POINT('Ctrl Pts',(-49.6853220200388,-6.39938613351776,
129.166693957078));
#212133=CARTESIAN_POINT('Ctrl Pts',(-49.9637696438516,-4.83683986146123,
135.303146579501));
#212134=CARTESIAN_POINT('Ctrl Pts',(-50.2422172676646,1.17052595051479,
137.305434680818));
#212135=CARTESIAN_POINT('Ctrl Pts',(-50.5206648914774,6.10223559733929,
133.333553313131));
#212136=CARTESIAN_POINT('Ctrl Pts',(-50.7991125152903,5.42628884099088,
127.03746741615));
#212137=CARTESIAN_POINT('Ctrl Pts',(-51.0775601391032,-0.236152271280866,
124.202972348307));
#212138=CARTESIAN_POINT('Ctrl Pts',(-51.3560077629162,-5.68158098292544,
127.434830604167));
#212139=CARTESIAN_POINT('Ctrl Pts',(-51.634455386729,-5.90591433192304,
133.763122331648));
#212140=CARTESIAN_POINT('Ctrl Pts',(-51.9129030105419,-0.703000929838195,
137.372456587432));
#212141=CARTESIAN_POINT('Ctrl Pts',(-52.1913506343548,5.14593598326309,
134.946031516236));
#212142=CARTESIAN_POINT('Ctrl Pts',(-52.4697982581677,6.26600912069438,
128.713613221033));
#212143=CARTESIAN_POINT('Ctrl Pts',(-52.7482458819806,1.62792598777083,
124.402489644555));
#212144=CARTESIAN_POINT('Ctrl Pts',(-53.0266935057934,-4.50614159930848,
125.97437274349));
#212145=CARTESIAN_POINT('Ctrl Pts',(-53.3051411296064,-6.49928519387843,
131.984778740675));
#212146=CARTESIAN_POINT('Ctrl Pts',(-53.5835887534191,-2.51990320300721,
136.910438149353));
#212147=CARTESIAN_POINT('Ctrl Pts',(-53.8620363772322,3.7751467273123,136.22491060479));
#212148=CARTESIAN_POINT('Ctrl Pts',(-54.140484001045,6.60102124140245,130.558162430556));
#212149=CARTESIAN_POINT('Ctrl Pts',(-54.418931624858,3.36087971245889,125.117658362733));
#212150=CARTESIAN_POINT('Ctrl Pts',(-54.6973792486707,-2.96774608413265,
124.902955856252));
#212151=CARTESIAN_POINT('Ctrl Pts',(-54.9758268724838,-6.56915821186243,
130.111356025769));
#212152=CARTESIAN_POINT('Ctrl Pts',(-55.2542744962966,-4.13383486411065,
135.956593559989));
#212153=CARTESIAN_POINT('Ctrl Pts',(-55.5327221201095,2.10028077469877,
137.067180720695));
#212154=CARTESIAN_POINT('Ctrl Pts',(-55.8111697439224,6.40434098598004,
132.422542162396));
#212155=CARTESIAN_POINT('Ctrl Pts',(-56.0896173677353,4.82312470059616,
126.29087381696));
#212156=CARTESIAN_POINT('Ctrl Pts',(-56.3680649915482,-1.19030756189505,
124.306879345194));
#212157=CARTESIAN_POINT('Ctrl Pts',(-56.646512615361,-6.10990532476174,
128.293752743129));
#212158=CARTESIAN_POINT('Ctrl Pts',(-56.924960239174,-5.41479857964128,
134.587752127659));
#212159=CARTESIAN_POINT('Ctrl Pts',(-57.2034078629868,0.256243532552689,
137.404999543363));
#212160=CARTESIAN_POINT('Ctrl Pts',(-57.4818554867998,5.69181035652338,
134.156582245398));
#212161=CARTESIAN_POINT('Ctrl Pts',(-57.7603031106126,5.89688152324325,
127.827637036585));
#212162=CARTESIAN_POINT('Ctrl Pts',(-58.0387507344255,0.683006648780185,
124.234155377662));
#212163=CARTESIAN_POINT('Ctrl Pts',(-58.3171983582384,-5.15851796918197,
126.67837136184));
#212164=CARTESIAN_POINT('Ctrl Pts',(-58.5956459820513,-6.25961658107885,
132.91416990625));
#212165=CARTESIAN_POINT('Ctrl Pts',(-58.8740936058642,-1.60843335423465,
137.211156784272));
#212166=CARTESIAN_POINT('Ctrl Pts',(-59.1525412296771,4.52082154881365,
135.620610974484));
#212167=CARTESIAN_POINT('Ctrl Pts',(-59.4309888534899,6.49566230291273,
129.604166373598));
#212168=CARTESIAN_POINT('Ctrl Pts',(-59.7094364773029,2.50130673138007,
124.69064165017));
#212169=CARTESIAN_POINT('Ctrl Pts',(-59.9878841011157,-3.79162753066369,
125.395325986002));
#212170=CARTESIAN_POINT('Ctrl Pts',(-60.2663317249287,-6.60024132333016,
131.070648902209));
#212171=CARTESIAN_POINT('Ctrl Pts',(-60.5447793487415,-3.34355577957023,
136.501265893734));
#212172=CARTESIAN_POINT('Ctrl Pts',(-60.8232269725544,2.98569418383416,
136.696705245755));
#212173=CARTESIAN_POINT('Ctrl Pts',(-61.1016745963673,6.57123705156454,
131.477367741508));
#212174=CARTESIAN_POINT('Ctrl Pts',(-61.3801222201802,4.11813409168408,
125.639569568584));
#212175=CARTESIAN_POINT('Ctrl Pts',(-61.6585698439931,-2.11933291641938,
124.547962055604));
#212176=CARTESIAN_POINT('Ctrl Pts',(-61.937017467806,-6.40923650950231,
129.205679179005));
#212177=CARTESIAN_POINT('Ctrl Pts',(-62.2154650916189,-4.80936485896274,
135.332506444514));
#212178=CARTESIAN_POINT('Ctrl Pts',(-62.4939127154318,1.21007814642843,
137.298188907278));
#212179=CARTESIAN_POINT('Ctrl Pts',(-62.7723603392447,6.1175184508558,133.296360412945));
#212180=CARTESIAN_POINT('Ctrl Pts',(-63.0508079630576,5.40325815633759,
127.004505847616));
#212181=CARTESIAN_POINT('Ctrl Pts',(-63.3292555868704,-0.276332420019459,
124.204532182646));
#212182=CARTESIAN_POINT('Ctrl Pts',(-63.6077032106833,-5.70198700196771,
127.469478429822));
#212183=CARTESIAN_POINT('Ctrl Pts',(-63.8861508344962,-5.8877940866586,
133.799018489484));
#212184=CARTESIAN_POINT('Ctrl Pts',(-64.1645984583092,-0.663006040441876,
137.376614262022));
#212185=CARTESIAN_POINT('Ctrl Pts',(-64.4430460821219,5.17105216729505,
134.914630007745));
#212186=CARTESIAN_POINT('Ctrl Pts',(-64.721493705935,6.25316605323042,128.675508981716));
#212187=CARTESIAN_POINT('Ctrl Pts',(-64.9999413297477,1.58892582039159,
124.392698608848));
#212188=CARTESIAN_POINT('Ctrl Pts',(-65.2783889535607,-4.53545961804555,
126.00189239489));
#212189=CARTESIAN_POINT('Ctrl Pts',(-65.5568365773735,-6.49197923701883,
132.024319863954));
#212190=CARTESIAN_POINT('Ctrl Pts',(-65.8352842011867,-2.48268708798906,
136.92566438391));
#212191=CARTESIAN_POINT('Ctrl Pts',(-66.1137318249993,3.80807320889562,
136.201829784909));
#212192=CARTESIAN_POINT('Ctrl Pts',(-66.3921794488124,6.59940026152389,
130.517984702147));
#212193=CARTESIAN_POINT('Ctrl Pts',(-66.6706270726251,3.3262008724376,125.097305095413));
#212194=CARTESIAN_POINT('Ctrl Pts',(-66.9490746964381,-3.00361462447264,
124.921130708376));
#212195=CARTESIAN_POINT('Ctrl Pts',(-67.227522320251,-6.57325501622426,
130.151357196124));
#212196=CARTESIAN_POINT('Ctrl Pts',(-67.5059699440638,-4.10239516942585,
135.981661927186));
#212197=CARTESIAN_POINT('Ctrl Pts',(-67.7844175678767,2.13836542492937,
137.054279679937));
#212198=CARTESIAN_POINT('Ctrl Pts',(-68.0628651916897,6.41407265873309,
132.383527139888));
#212199=CARTESIAN_POINT('Ctrl Pts',(-68.3413128155024,4.79556046403026,
126.261597712398));
#212200=CARTESIAN_POINT('Ctrl Pts',(-68.6197604393155,-1.22983752096341,
124.314245468451));
#212201=CARTESIAN_POINT('Ctrl Pts',(-68.8982080631282,-6.12507490509475,
128.330991986789));
#212202=CARTESIAN_POINT('Ctrl Pts',(-69.1766556869413,-5.39166767798822,
134.620643446035));
#212203=CARTESIAN_POINT('Ctrl Pts',(-69.455103310754,0.296418747580413,
137.403317421698));
#212204=CARTESIAN_POINT('Ctrl Pts',(-69.733550934567,5.7121108249834,134.121872471326));
#212205=CARTESIAN_POINT('Ctrl Pts',(-70.0119985583799,5.87865210635384,
127.791796196812));
#212206=CARTESIAN_POINT('Ctrl Pts',(-70.2904461821926,0.642999290106501,
124.230119453016));
#212207=CARTESIAN_POINT('Ctrl Pts',(-70.5688938060058,-5.18353846148724,
126.709849169906));
#212208=CARTESIAN_POINT('Ctrl Pts',(-70.8473414298183,-6.24665759690589,
132.95223487919));
#212209=CARTESIAN_POINT('Ctrl Pts',(-71.1257890536316,-1.56940356695681,
137.220829071533));
#212210=CARTESIAN_POINT('Ctrl Pts',(-71.4042366774442,4.55005567139915,
135.593002216589));
#212211=CARTESIAN_POINT('Ctrl Pts',(-71.6826843012574,6.48823603031619,
129.56464767029));
#212212=CARTESIAN_POINT('Ctrl Pts',(-71.9611319250699,2.46404444532374,
124.675528759193));
#212213=CARTESIAN_POINT('Ctrl Pts',(-72.2395795488831,-3.82448360965763,
125.418506915858));
#212214=CARTESIAN_POINT('Ctrl Pts',(-72.518027172696,-6.59849806377525,
131.110821510811));
#212215=CARTESIAN_POINT('Ctrl Pts',(-72.7964747965087,-3.30881515183405,
136.52151351632));
#212216=CARTESIAN_POINT('Ctrl Pts',(-73.0749224203217,3.02150724003593,
136.678421306317));
#212217=CARTESIAN_POINT('Ctrl Pts',(-73.3533700441346,6.57521208714753,
131.437354287172));
#212218=CARTESIAN_POINT('Ctrl Pts',(-73.6318176679474,4.08661824313884,
125.614597009117));
#212219=CARTESIAN_POINT('Ctrl Pts',(-73.9102652917603,-2.15737812391465,
124.56097895318));
#212220=CARTESIAN_POINT('Ctrl Pts',(-74.1887129155733,-6.41884938887091,
129.244723640663));
#212221=CARTESIAN_POINT('Ctrl Pts',(-74.4671605393861,-4.78171164368069,
135.361698517417));
#212222=CARTESIAN_POINT('Ctrl Pts',(-74.745608163199,1.24958550245192,137.290702502541));
#212223=CARTESIAN_POINT('Ctrl Pts',(-75.0240557870119,6.13257461747648,
133.25907517079));
#212224=CARTESIAN_POINT('Ctrl Pts',(-75.3025034108249,5.380027251966,126.971685084098));
#212225=CARTESIAN_POINT('Ctrl Pts',(-75.5809510346376,-0.31650232915867,
124.206336576053));
#212226=CARTESIAN_POINT('Ctrl Pts',(-75.8593986584506,-5.72218173178456,
127.504249830764));
#212227=CARTESIAN_POINT('Ctrl Pts',(-76.1378462822634,-5.86945566701928,
133.83480367917));
#212228=CARTESIAN_POINT('Ctrl Pts',(-76.4162939060764,-0.622986583113102,
137.380528399336));
#212229=CARTESIAN_POINT('Ctrl Pts',(-76.6947415298893,5.19597673608708,
134.88307619171));
#212230=CARTESIAN_POINT('Ctrl Pts',(-76.9731891537022,6.24009127239896,
128.637483627779));
#212231=CARTESIAN_POINT('Ctrl Pts',(-77.2516367775151,1.54986677478153,
124.383145159635));
#212232=CARTESIAN_POINT('Ctrl Pts',(-77.5300844013279,-4.56460957365852,
126.029590003516));
#212233=CARTESIAN_POINT('Ctrl Pts',(-77.8085320251407,-6.48443271748106,
132.063815781194));
#212234=CARTESIAN_POINT('Ctrl Pts',(-78.0869796489538,-2.44537897608793,
136.940663791305));
#212235=CARTESIAN_POINT('Ctrl Pts',(-78.3654272727665,3.84085858092573,
136.178548959823));
#212236=CARTESIAN_POINT('Ctrl Pts',(-78.6438748965796,6.5975347384416,130.477817585504));
#212237=CARTESIAN_POINT('Ctrl Pts',(-78.9223225203923,3.29139877882003,
125.077163305135));
#212238=CARTESIAN_POINT('Ctrl Pts',(-79.2007701442053,-3.03937186476788,
124.939523565746));
#212239=CARTESIAN_POINT('Ctrl Pts',(-79.4792177680182,-6.57710824620412,
130.191382563762));
#212240=CARTESIAN_POINT('Ctrl Pts',(-79.7576653918309,-4.07080345897965,
136.00653844758));
#212241=CARTESIAN_POINT('Ctrl Pts',(-80.036113015644,2.17637083724304,137.041147046131));
#212242=CARTESIAN_POINT('Ctrl Pts',(-80.314560639457,6.42356665566488,132.344453600785));
#212243=CARTESIAN_POINT('Ctrl Pts',(-80.5930082632696,4.76781852620778,
126.232489941585));
#212244=CARTESIAN_POINT('Ctrl Pts',(-80.8714558870828,-1.26932190795047,
124.321852085313));
#212245=CARTESIAN_POINT('Ctrl Pts',(-81.1499035108954,-6.14001751852468,
128.368322882032));
#212246=CARTESIAN_POINT('Ctrl Pts',(-81.4283511347085,-5.36833698610627,
134.653393350648));
#212247=CARTESIAN_POINT('Ctrl Pts',(-81.7067987585213,0.336582978702201,
137.401390773263));
#212248=CARTESIAN_POINT('Ctrl Pts',(-81.9852463823341,5.73219962907597,
134.087039765632));
#212249=CARTESIAN_POINT('Ctrl Pts',(-82.2636940061471,5.86020485384888,
127.756066988721));
#212250=CARTESIAN_POINT('Ctrl Pts',(-82.54214162996,0.602968104857597,124.226327139294));
#212251=CARTESIAN_POINT('Ctrl Pts',(-82.8205892537728,-5.20836687586887,
126.741478701599));
#212252=CARTESIAN_POINT('Ctrl Pts',(-83.0990368775859,-6.23346714053832,
132.990220261861));
#212253=CARTESIAN_POINT('Ctrl Pts',(-83.3774845013985,-1.53031562485268,
137.230263594196));
#212254=CARTESIAN_POINT('Ctrl Pts',(-83.6559321252116,4.57912118999838,
135.56521601382));
#212255=CARTESIAN_POINT('Ctrl Pts',(-83.9343797490243,6.48056933374724,
129.525174905002));
#212256=CARTESIAN_POINT('Ctrl Pts',(-84.2128273728376,2.42669085319518,
124.660642974335));
#212257=CARTESIAN_POINT('Ctrl Pts',(-84.4912749966499,-3.85719797100462,
125.441887420503));
#212258=CARTESIAN_POINT('Ctrl Pts',(-84.7697226204634,-6.59651029444787,
131.150982763393));
#212259=CARTESIAN_POINT('Ctrl Pts',(-85.0481702442759,-3.27395191473627,
136.541549287701));
#212260=CARTESIAN_POINT('Ctrl Pts',(-85.326617868089,3.05720833317481,136.659919701402));
#212261=CARTESIAN_POINT('Ctrl Pts',(-85.6050654919017,6.57894347582879,
131.397317377022));
#212262=CARTESIAN_POINT('Ctrl Pts',(-85.8835131157147,4.05495096345227,
125.58981675825));
#212263=CARTESIAN_POINT('Ctrl Pts',(-86.1619607395276,-2.19534338896908,
124.574227201559));
#212264=CARTESIAN_POINT('Ctrl Pts',(-86.4404083633404,-6.42822441541511,
129.283825895241));
#212265=CARTESIAN_POINT('Ctrl Pts',(-86.7188559871533,-4.75388124031539,
135.390721716488));
#212266=CARTESIAN_POINT('Ctrl Pts',(-86.9973036109663,1.28904655462414,
137.282975744021));
#212267=CARTESIAN_POINT('Ctrl Pts',(-87.2757512347791,6.14740353928957,
133.221698968287));
#212268=CARTESIAN_POINT('Ctrl Pts',(-87.554198858592,5.35659698870609,126.939006341782));
#212269=CARTESIAN_POINT('Ctrl Pts',(-87.8326464824051,-0.356660510187587,
124.208385461669));
#212270=CARTESIAN_POINT('Ctrl Pts',(-88.1110941062178,-5.74216442405318,
127.539143518524));
#212271=CARTESIAN_POINT('Ctrl Pts',(-88.3895417300309,-5.85089975254147,
133.870476574676));
#212272=CARTESIAN_POINT('Ctrl Pts',(-88.6679893538435,-0.582944040787213,
137.384198854334));
#212273=CARTESIAN_POINT('Ctrl Pts',(-88.9464369776566,5.22070876605056,
134.851371237371));
#212274=CARTESIAN_POINT('Ctrl Pts',(-89.2248846014694,6.22678526269035,
128.599538568266));
#212275=CARTESIAN_POINT('Ctrl Pts',(-89.5033322252823,1.51075029828878,
124.373829650922));
#212276=CARTESIAN_POINT('Ctrl Pts',(-89.7817798490951,-4.59359038598471,
126.057464543021));
#212277=CARTESIAN_POINT('Ctrl Pts',(-90.0602274729082,-6.47664591490472,
132.103265028861));
#212278=CARTESIAN_POINT('Ctrl Pts',(-90.338675096721,-2.40798024976945,
136.955435815729));
#212279=CARTESIAN_POINT('Ctrl Pts',(-90.6171227205338,3.87350162852866,
136.155068992212));
#212280=CARTESIAN_POINT('Ctrl Pts',(-90.8955703443469,6.59542474128344,
130.437662569033));
#212281=CARTESIAN_POINT('Ctrl Pts',(-91.1740179681596,3.25647472121003,
125.057233738258));
#212282=CARTESIAN_POINT('Ctrl Pts',(-91.4524655919725,-3.07501648002118,
124.958133746811));
#212283=CARTESIAN_POINT('Ctrl Pts',(-91.7309132157855,-6.58071775901922,
130.231430645527));
#212284=CARTESIAN_POINT('Ctrl Pts',(-92.0093608395982,-4.03906090341396,
136.031222199361));
#212285=CARTESIAN_POINT('Ctrl Pts',(-92.2878084634112,2.21429560333469,
137.027783305909));
#212286=CARTESIAN_POINT('Ctrl Pts',(-92.5662560872241,6.4328226249721,132.305322992969));
#212287=CARTESIAN_POINT('Ctrl Pts',(-92.844703711037,4.73989991511645,126.203551583122));
#212288=CARTESIAN_POINT('Ctrl Pts',(-93.1231513348499,-1.30875925974737,
124.329698913911));
#212289=CARTESIAN_POINT('Ctrl Pts',(-93.4015989586628,-6.15473261134757,
128.40574404555));
#212290=CARTESIAN_POINT('Ctrl Pts',(-93.6800465824757,-5.34480736852315,
134.686000627937));
#212291=CARTESIAN_POINT('Ctrl Pts',(-93.9584942062885,0.37673473761816,
137.399219669449));
#212292=CARTESIAN_POINT('Ctrl Pts',(-94.2369418301014,5.75207602440345,
134.052085419056));
#212293=CARTESIAN_POINT('Ctrl Pts',(-94.5153894539144,5.84154044929785,
127.720450736271));
#212294=CARTESIAN_POINT('Ctrl Pts',(-94.7938370777271,0.56291457640357,
124.222778577022));
#212295=CARTESIAN_POINT('Ctrl Pts',(-95.0722847015402,-5.23300229230026,
126.773258784876));
#212296=CARTESIAN_POINT('Ctrl Pts',(-95.350732325353,-6.22004570075364,
133.028124646699));
#212297=CARTESIAN_POINT('Ctrl Pts',(-95.6291799491659,-1.49117097634027,
137.239460002661));
#212298=CARTESIAN_POINT('Ctrl Pts',(-95.9076275729788,4.60801702757804,
135.537253395802));
#212299=CARTESIAN_POINT('Ctrl Pts',(-96.1860751967916,6.47266249729856,
129.48574954041));
#212300=CARTESIAN_POINT('Ctrl Pts',(-96.4645228206046,2.38924733914408,
124.645984847192));
#212301=CARTESIAN_POINT('Ctrl Pts',(-96.7429704444176,-3.88976940246256,
125.465466633565));
#212302=CARTESIAN_POINT('Ctrl Pts',(-97.0214180682302,-6.59427808900543,
131.191131171763));
#212303=CARTESIAN_POINT('Ctrl Pts',(-97.2998656920433,-3.23896736014657,
136.561372465446));
#212304=CARTESIAN_POINT('Ctrl Pts',(-97.5783133158561,3.09279614033489,
136.641201116591));
#212305=CARTESIAN_POINT('Ctrl Pts',(-97.856760939669,6.58243107933991,131.357258494642));
#212306=CARTESIAN_POINT('Ctrl Pts',(-98.135208563482,4.02313342606635,125.565229734223));
#212307=CARTESIAN_POINT('Ctrl Pts',(-98.4136561872948,-2.2332273047675,
124.587706309824));
#212308=CARTESIAN_POINT('Ctrl Pts',(-98.6921038111079,-6.43736124173946,
129.322984493793));
#212309=CARTESIAN_POINT('Ctrl Pts',(-98.9705514349205,-4.72587468013238,
135.419574966262));
#212310=CARTESIAN_POINT('Ctrl Pts',(-99.2489990587337,1.32845984070286,
137.275008918035));
#212311=CARTESIAN_POINT('Ctrl Pts',(-99.5274466825463,6.16200466680371,
133.184233190419));
#212312=CARTESIAN_POINT('Ctrl Pts',(-99.8058943063594,5.3329682347749,126.906470831589));
#212313=CARTESIAN_POINT('Ctrl Pts',(-100.084341930172,-0.396805475030165,
124.210678763569));
#212314=CARTESIAN_POINT('Ctrl Pts',(-100.362789553985,-5.76193433830736,
127.574158200105));
#212315=CARTESIAN_POINT('Ctrl Pts',(-100.641237177798,-5.83212703082168,
133.906035854126));
#212316=CARTESIAN_POINT('Ctrl Pts',(-100.919684801611,-0.542879897255484,
137.387625491007));
#212317=CARTESIAN_POINT('Ctrl Pts',(-101.198132425424,5.24524734073077,
134.819516319564));
#212318=CARTESIAN_POINT('Ctrl Pts',(-101.476580049237,6.21324851716398,
128.561675209245));
#212319=CARTESIAN_POINT('Ctrl Pts',(-101.75502767305,1.47157784038775,124.3647524279));
#212320=CARTESIAN_POINT('Ctrl Pts',(-102.033475296863,-4.62240098113028,
126.085514980508));
#212321=CARTESIAN_POINT('Ctrl Pts',(-102.311922920676,-6.4686191178319,
132.142666145147));
#212322=CARTESIAN_POINT('Ctrl Pts',(-102.590370544489,-2.3704922948573,
136.969979909799));
#212323=CARTESIAN_POINT('Ctrl Pts',(-102.868818168302,3.90600114210426,
136.131390752135));
#212324=CARTESIAN_POINT('Ctrl Pts',(-103.147265792114,6.59307034823604,
130.397521140692));
#212325=CARTESIAN_POINT('Ctrl Pts',(-103.425713415927,3.22142999373166,
125.037517133282));
#212326=CARTESIAN_POINT('Ctrl Pts',(-103.70416103974,-3.11054714940797,
124.976960561963));
#212327=CARTESIAN_POINT('Ctrl Pts',(-103.982608663553,-6.58408342091771,
130.271499957422));
#212328=CARTESIAN_POINT('Ctrl Pts',(-104.261056287366,-4.00716867896111,
136.055712267864));
#212329=CARTESIAN_POINT('Ctrl Pts',(-104.539503911179,2.25213831788793,
137.014188954471));
#212330=CARTESIAN_POINT('Ctrl Pts',(-104.817951534992,6.44184022367115,
132.266136766442));
#212331=CARTESIAN_POINT('Ctrl Pts',(-105.096399158805,4.71180566529118,
126.17478370933));
#212332=CARTESIAN_POINT('Ctrl Pts',(-105.374846782618,-1.34814811498862,
124.337785663482));
#212333=CARTESIAN_POINT('Ctrl Pts',(-105.65329440643,-6.16921963829011,
128.443254090687));
#212334=CARTESIAN_POINT('Ctrl Pts',(-105.931742030243,-5.32107969713743,
134.718464069627));
#212335=CARTESIAN_POINT('Ctrl Pts',(-106.210189654056,0.416872536489867,
137.396804190707));
#212336=CARTESIAN_POINT('Ctrl Pts',(-106.488637277869,5.77173927443855,
134.017010726842));
#212337=CARTESIAN_POINT('Ctrl Pts',(-106.767084901682,5.82265958431723,
127.684948759235));
#212338=CARTESIAN_POINT('Ctrl Pts',(-107.045532525495,0.52284018894291,
124.219473897692));
#212339=CARTESIAN_POINT('Ctrl Pts',(-107.323980149308,-5.25744379790729,
126.805188242113));
#212340=CARTESIAN_POINT('Ctrl Pts',(-107.602427773121,-6.20639377488812,
133.065946629143));
#212341=CARTESIAN_POINT('Ctrl Pts',(-107.880875396933,-1.45197107193893,
137.248417956151));
#212342=CARTESIAN_POINT('Ctrl Pts',(-108.159323020746,4.63674211339212,
135.509115398702));
#212343=CARTESIAN_POINT('Ctrl Pts',(-108.437770644559,6.46451581396073,
129.446373037437));
#212344=CARTESIAN_POINT('Ctrl Pts',(-108.716218268372,2.35171529065418,
124.631554920928));
#212345=CARTESIAN_POINT('Ctrl Pts',(-108.994665892185,-3.92219669708481,
125.489243681306));
#212346=CARTESIAN_POINT('Ctrl Pts',(-109.273113515998,-6.59180153016358,
131.231265248209));
#212347=CARTESIAN_POINT('Ctrl Pts',(-109.551561139811,-3.20386278442967,
136.580982315001));
#212348=CARTESIAN_POINT('Ctrl Pts',(-109.830008763624,3.12826934279688,
136.622266245509));
#212349=CARTESIAN_POINT('Ctrl Pts',(-110.108456387437,6.5856747684467,131.317179124427));
#212350=CARTESIAN_POINT('Ctrl Pts',(-110.38690401125,3.99116680999183,125.540836848117));
#212351=CARTESIAN_POINT('Ctrl Pts',(-110.665351635062,-2.27102846750687,
124.601415778499));
#212352=CARTESIAN_POINT('Ctrl Pts',(-110.943799258875,-6.44625952927566,
129.362197985281));
#212353=CARTESIAN_POINT('Ctrl Pts',(-111.222246882688,-4.69769300092514,
135.448257197571));
#212354=CARTESIAN_POINT('Ctrl Pts',(-111.500694506501,1.36782390021364,
137.266802319797));
#212355=CARTESIAN_POINT('Ctrl Pts',(-111.779142130314,6.17637745896884,
133.1466792255));
#212356=CARTESIAN_POINT('Ctrl Pts',(-112.057589754127,5.30914186574463,
126.874079759138));
#212357=CARTESIAN_POINT('Ctrl Pts',(-112.33603737794,-0.436935736099303,
124.213216396775));
#212358=CARTESIAN_POINT('Ctrl Pts',(-112.614485001753,-5.78149074196569,
127.609292578024));
#212359=CARTESIAN_POINT('Ctrl Pts',(-112.892932625565,-5.81313819748998,
133.94148019986));
#212360=CARTESIAN_POINT('Ctrl Pts',(-113.171380249379,-0.502795637109545,
137.390808182378));
#212361=CARTESIAN_POINT('Ctrl Pts',(-113.449827873191,5.26959155084185,
134.787512618686));
#212362=CARTESIAN_POINT('Ctrl Pts',(-113.728275497004,6.19948153742887,
128.523894953756));
#212363=CARTESIAN_POINT('Ctrl Pts',(-114.006723120817,1.43235085262869,
124.355913826926));
#212364=CARTESIAN_POINT('Ctrl Pts',(-114.28517074463,-4.65104029150761,
126.113740276555));
#212365=CARTESIAN_POINT('Ctrl Pts',(-114.563618368443,-6.46035262369882,
132.182017670029));
#212366=CARTESIAN_POINT('Ctrl Pts',(-114.842065992256,-2.33291650048142,
136.984295534578));
#212367=CARTESIAN_POINT('Ctrl Pts',(-115.120513616069,3.93835591737112,
136.107515116997));
#212368=CARTESIAN_POINT('Ctrl Pts',(-115.398961239881,6.59047164654225,
130.357394787938));
#212369=CARTESIAN_POINT('Ctrl Pts',(-115.677408863695,3.18626589498021,
125.018014220813));
#212370=CARTESIAN_POINT('Ctrl Pts',(-115.955856487507,-3.14596255632626,
124.996003313566));
#212371=CARTESIAN_POINT('Ctrl Pts',(-116.23430411132,-6.58720510718372,
130.311589014666));
#212372=CARTESIAN_POINT('Ctrl Pts',(-116.512751735133,-3.97512796739924,
136.0800077456));
#212373=CARTESIAN_POINT('Ctrl Pts',(-116.791199358946,2.28989757862811,
137.00036449556));
#212374=CARTESIAN_POINT('Ctrl Pts',(-117.069646982759,6.45061911761184,
132.226896373261));
#212375=CARTESIAN_POINT('Ctrl Pts',(-117.348094606572,4.68353681777373,
126.146187386213));
#212376=CARTESIAN_POINT('Ctrl Pts',(-117.626542230384,-1.38748701410568,
124.346112034364));
#212377=CARTESIAN_POINT('Ctrl Pts',(-117.904989854198,-6.18347806253024,
128.480851627495));
#212378=CARTESIAN_POINT('Ctrl Pts',(-118.18343747801,-5.29715485118671,
134.750782472776));
#212379=CARTESIAN_POINT('Ctrl Pts',(-118.461885101824,0.45699488799644,
137.394144426544));
#212380=CARTESIAN_POINT('Ctrl Pts',(-118.740332725636,5.79118865055225,
133.981816988697));
#212381=CARTESIAN_POINT('Ctrl Pts',(-119.018780349449,5.80356295854445,
127.649562373154));
#212382=CARTESIAN_POINT('Ctrl Pts',(-119.297227973262,0.482746427446748,
124.216413223762));
#212383=CARTESIAN_POINT('Ctrl Pts',(-119.575675597075,-5.28169048700048,
126.837265890154));
#212384=CARTESIAN_POINT('Ctrl Pts',(-119.854123220888,-6.19251186881905,
133.103684807684));
#212385=CARTESIAN_POINT('Ctrl Pts',(-120.132570844701,-1.41271736421608,
137.257137122728));
#212386=CARTESIAN_POINT('Ctrl Pts',(-120.411018468513,4.66529538302207,
135.480803065184));
#212387=CARTESIAN_POINT('Ctrl Pts',(-120.689466092327,6.45612958561205,
129.407046855192));
#212388=CARTESIAN_POINT('Ctrl Pts',(-120.967913716139,2.31409609848935,
124.61735373025));
#212389=CARTESIAN_POINT('Ctrl Pts',(-121.246361339953,-3.95447865326606,
125.51321768266));
#212390=CARTESIAN_POINT('Ctrl Pts',(-121.524808963765,-6.5890807096919,
131.271383505546));
#212391=CARTESIAN_POINT('Ctrl Pts',(-121.803256587578,-3.16863948839908,
136.600378109714));
#212392=CARTESIAN_POINT('Ctrl Pts',(-122.081704211391,3.16362662608795,
136.603115789794));
#212393=CARTESIAN_POINT('Ctrl Pts',(-122.360151835204,6.58867442295306,
131.277080751534));
#212394=CARTESIAN_POINT('Ctrl Pts',(-122.638599459017,3.9590522997634,125.51663900382));
#212395=CARTESIAN_POINT('Ctrl Pts',(-122.91704708283,-2.30874547645122,
124.615355099576));
#212396=CARTESIAN_POINT('Ctrl Pts',(-123.195494706643,-6.45491894829438,
129.401464916637));
#212397=CARTESIAN_POINT('Ctrl Pts',(-123.473942330455,-4.66933724697619,
135.476767347585));
#212398=CARTESIAN_POINT('Ctrl Pts',(-123.752389954268,1.40713727450679,
137.258356253404));
#212399=CARTESIAN_POINT('Ctrl Pts',(-124.030837578081,6.19052138319586,
133.109038465103));
#212400=CARTESIAN_POINT('Ctrl Pts',(-124.309285201894,5.28511876451003,
126.841834324687));
#212401=CARTESIAN_POINT('Ctrl Pts',(-124.587732825707,-0.477049806354697,
124.215998267256));
#212402=CARTESIAN_POINT('Ctrl Pts',(-124.86618044952,-5.80083291035842,
127.644545350364));
#212403=CARTESIAN_POINT('Ctrl Pts',(-125.144628073333,-5.79393395618462,
133.976808298475));
#212404=CARTESIAN_POINT('Ctrl Pts',(-125.423075697146,-0.462692745686338,
137.393746810514));
#212405=CARTESIAN_POINT('Ctrl Pts',(-125.701523320958,5.2937404943001,134.755361320645));
#212406=CARTESIAN_POINT('Ctrl Pts',(-125.979970944772,6.18548483362552,
128.486199201761));
#212407=CARTESIAN_POINT('Ctrl Pts',(-126.258418568584,1.39307078858202,
124.34731417552));
#212408=CARTESIAN_POINT('Ctrl Pts',(-126.536866192397,-4.67950725587653,
126.142139385264));
#212409=CARTESIAN_POINT('Ctrl Pts',(-126.81531381621,-6.45184673882346,
132.221318145323));
#212410=CARTESIAN_POINT('Ctrl Pts',(-127.093761440023,-2.29525425902701,
136.998382159598));
#212411=CARTESIAN_POINT('Ctrl Pts',(-127.372209063836,3.97056475541062,
136.083442971518));
#212412=CARTESIAN_POINT('Ctrl Pts',(-127.650656687649,6.58762873249828,
130.317284997668));
#212413=CARTESIAN_POINT('Ctrl Pts',(-127.929104311462,3.15098372797424,
124.998725723536));
#212414=CARTESIAN_POINT('Ctrl Pts',(-128.207551935275,-3.18126138844507,
125.015261295985));
#212415=CARTESIAN_POINT('Ctrl Pts',(-128.485999559087,-6.59008270214206,
130.351696331743));
#212416=CARTESIAN_POINT('Ctrl Pts',(-128.764447182901,-3.94293995600869,
136.104107732291));
#212417=CARTESIAN_POINT('Ctrl Pts',(-129.042894806713,2.32757198637139,
136.986310441447));
#212418=CARTESIAN_POINT('Ctrl Pts',(-129.321342430526,6.45915898148892,
132.187603267495));
#212419=CARTESIAN_POINT('Ctrl Pts',(-129.599790054339,4.6550944200771,126.117763673416));
#212420=CARTESIAN_POINT('Ctrl Pts',(-129.878237678152,-1.42677449938118,
124.354677718024));
#212421=CARTESIAN_POINT('Ctrl Pts',(-130.156685301965,-6.19750735571679,
128.518535262782));
#212422=CARTESIAN_POINT('Ctrl Pts',(-130.435132925778,-5.27303371721495,
134.782954639811));
#212423=CARTESIAN_POINT('Ctrl Pts',(-130.713580549591,0.497100305389368,
137.391240475519));
#212424=CARTESIAN_POINT('Ctrl Pts',(-130.992028173403,5.81042343204081,
133.946505508738));
#212425=CARTESIAN_POINT('Ctrl Pts',(-131.270475797217,5.78425127961196,
127.614292889281));
#212426=CARTESIAN_POINT('Ctrl Pts',(-131.548923421029,0.442634777604211,
124.213596668645));
#212427=CARTESIAN_POINT('Ctrl Pts',(-131.827371044842,-5.30574146111081,
126.869490540348));
#212428=CARTESIAN_POINT('Ctrl Pts',(-132.105818668655,-6.17840049694519,
133.141337783923));
#212429=CARTESIAN_POINT('Ctrl Pts',(-132.384266292468,-1.37341130773126,
137.265617179298));
#212430=CARTESIAN_POINT('Ctrl Pts',(-132.662713916281,4.69367577841589,
135.45231744437));
#212431=CARTESIAN_POINT('Ctrl Pts',(-132.941161540094,6.44750412300737,
129.367772450924));
#212432=CARTESIAN_POINT('Ctrl Pts',(-133.219609163907,2.27639115664257,
124.603381801387));
#212433=CARTESIAN_POINT('Ctrl Pts',(-133.49805678772,-3.98661407478655,
125.537387749261));
#212434=CARTESIAN_POINT('Ctrl Pts',(-133.776504411532,-6.58611572841139,
131.311484457178));
#212435=CARTESIAN_POINT('Ctrl Pts',(-134.054952035345,-3.13329877726696,
136.619559130867));
#212436=CARTESIAN_POINT('Ctrl Pts',(-134.333399659158,3.19886668003099,
136.583750459073));
#212437=CARTESIAN_POINT('Ctrl Pts',(-134.611847282971,6.59142993170542,
131.236964861823));
#212438=CARTESIAN_POINT('Ctrl Pts',(-134.890294906784,3.92679108539655,
125.492637097993));
#212439=CARTESIAN_POINT('Ctrl Pts',(-135.168742530597,-2.34637693398254,
124.629523756529));
#212440=CARTESIAN_POINT('Ctrl Pts',(-135.44719015441,-6.46333917791768,
129.440783832808));
#212441=CARTESIAN_POINT('Ctrl Pts',(-135.725637778223,-4.64080846901838,
135.505104359849));
#212442=CARTESIAN_POINT('Ctrl Pts',(-136.004085402036,1.44639850681073,
137.24967103183));
#212443=CARTESIAN_POINT('Ctrl Pts',(-136.282533025848,6.20443591537649,
133.07131230402));
#212444=CARTESIAN_POINT('Ctrl Pts',(-136.560980649661,5.26089982125598,
126.809735723105));
#212445=CARTESIAN_POINT('Ctrl Pts',(-136.839428273474,-0.517146199354053,
124.219024271924));
#212446=CARTESIAN_POINT('Ctrl Pts',(-137.117875897287,-5.81996012675442,
127.679915210822));
#212447=CARTESIAN_POINT('Ctrl Pts',(-137.3963235211,-5.77451501852576,134.012018840873));
#212448=CARTESIAN_POINT('Ctrl Pts',(-137.674771144913,-0.422572709013315,
137.396441266521));
#212449=CARTESIAN_POINT('Ctrl Pts',(-137.953218768726,5.31769327625758,
134.723063616821));
#212450=CARTESIAN_POINT('Ctrl Pts',(-138.231666392539,6.17125892440694,
128.448589350091));
#212451=CARTESIAN_POINT('Ctrl Pts',(-138.510114016352,1.35373910378499,
124.338953792345));
#212452=CARTESIAN_POINT('Ctrl Pts',(-138.788561640165,-4.70780081938319,
126.170711254294));
#212453=CARTESIAN_POINT('Ctrl Pts',(-139.067009263977,-6.44310177839452,
132.260566114734));
#212454=CARTESIAN_POINT('Ctrl Pts',(-139.34545688779,-2.25750696608163,
137.012239262869));
#212455=CARTESIAN_POINT('Ctrl Pts',(-139.623904511603,4.00262646271346,
136.059175207703));
#212456=CARTESIAN_POINT('Ctrl Pts',(-139.902352135416,6.5845417114487,130.277193256163));
#212457=CARTESIAN_POINT('Ctrl Pts',(-140.180799759229,3.11558480010749,
124.979652356196));
#212458=CARTESIAN_POINT('Ctrl Pts',(-140.459247383042,-3.21644233775325,
125.034733795609));
#212459=CARTESIAN_POINT('Ctrl Pts',(-140.737695006855,-6.59271609916233,
130.391820422461));
#212460=CARTESIAN_POINT('Ctrl Pts',(-141.016142630668,-3.91060583752806,
136.128011334905));
#212461=CARTESIAN_POINT('Ctrl Pts',(-141.294590254481,2.36516014507876,
136.97202731291));
#212462=CARTESIAN_POINT('Ctrl Pts',(-141.573037878293,6.46745949885459,
132.148258905163));
#212463=CARTESIAN_POINT('Ctrl Pts',(-141.851485502106,4.62647952614482,
126.089513624195));
#212464=CARTESIAN_POINT('Ctrl Pts',(-142.129933125919,-1.4660091150024,
124.363482397054));
#212465=CARTESIAN_POINT('Ctrl Pts',(-142.408380749732,-6.21130699798892,
128.556303600169));
#212466=CARTESIAN_POINT('Ctrl Pts',(-142.686828373545,-5.24871718904012,
134.814979378581));
#212467=CARTESIAN_POINT('Ctrl Pts',(-142.965275997358,0.537187302547703,
137.388092445238));
#212468=CARTESIAN_POINT('Ctrl Pts',(-143.243723621171,5.82944290615228,
133.911077595444));
#212469=CARTESIAN_POINT('Ctrl Pts',(-143.522171244983,5.76472526312116,
127.579141614542));
#212470=CARTESIAN_POINT('Ctrl Pts',(-143.800618868797,0.402506725767204,
124.21102433671));
#212471=CARTESIAN_POINT('Ctrl Pts',(-144.079066492609,-5.32959582902011,
126.901860998601));
#212472=CARTESIAN_POINT('Ctrl Pts',(-144.357514116423,-6.1640601821688,
133.178904162615));
#212473=CARTESIAN_POINT('Ctrl Pts',(-144.635961740235,-1.33405435898536,
137.27385781163));
#212474=CARTESIAN_POINT('Ctrl Pts',(-144.914409364048,4.72188224792766,
135.423659591808));
#212475=CARTESIAN_POINT('Ctrl Pts',(-145.192856987861,6.43863974576633,
129.328551279958));
#212476=CARTESIAN_POINT('Ctrl Pts',(-145.471304611674,2.23860186228433,
124.589639652074));
#212477=CARTESIAN_POINT('Ctrl Pts',(-145.749752235487,-4.01860177085642,
125.56175298548));
#212478=CARTESIAN_POINT('Ctrl Pts',(-146.0281998593,-6.58290669619051,131.35156661715));
#212479=CARTESIAN_POINT('Ctrl Pts',(-146.306647483113,-3.09784196059638,
136.638524667701));
#212480=CARTESIAN_POINT('Ctrl Pts',(-146.585095106925,3.2339881987928,136.564170970937));
#212481=CARTESIAN_POINT('Ctrl Pts',(-146.863542730738,6.59394119259793,
131.196832941802));
#212482=CARTESIAN_POINT('Ctrl Pts',(-147.141990354551,3.89438436234147,
125.468832020033));
#212483=CARTESIAN_POINT('Ctrl Pts',(-147.420437978364,-2.38392144565404,
124.643921224334));
#212484=CARTESIAN_POINT('Ctrl Pts',(-147.698885602177,-6.47151990613084,
129.480153276819));
#212485=CARTESIAN_POINT('Ctrl Pts',(-147.97733322599,-4.61210772419611,
135.533267184325));
#212486=CARTESIAN_POINT('Ctrl Pts',(-148.255780849803,1.48560614228611,
137.240746976909));
#212487=CARTESIAN_POINT('Ctrl Pts',(-148.534228473616,6.21812053990256,
133.033502140209));
#212488=CARTESIAN_POINT('Ctrl Pts',(-148.812676097428,5.23648593342438,
126.777785143819));
#212489=CARTESIAN_POINT('Ctrl Pts',(-149.091123721242,-0.557223429310831,
124.222294298654));
#212490=CARTESIAN_POINT('Ctrl Pts',(-149.369571345054,-5.83887168238761,
127.715400848752));
#212491=CARTESIAN_POINT('Ctrl Pts',(-149.648018968867,-5.75488210408933,
134.047110522317));
#212492=CARTESIAN_POINT('Ctrl Pts',(-149.92646659268,-0.382437013753756,
137.398891450554));
#212493=CARTESIAN_POINT('Ctrl Pts',(-150.204914216493,5.34144900913504,
134.690620704017));
#212494=CARTESIAN_POINT('Ctrl Pts',(-150.483361840306,6.15680433691945,
128.411066792389));
#212495=CARTESIAN_POINT('Ctrl Pts',(-150.761809464119,1.31435725568762,
124.330832987197));
#212496=CARTESIAN_POINT('Ctrl Pts',(-151.040257087932,-4.73591993359918,
126.199454824906));
#212497=CARTESIAN_POINT('Ctrl Pts',(-151.318704711745,-6.43411806645975,
132.299760123916));
#212498=CARTESIAN_POINT('Ctrl Pts',(-151.597152335558,-2.21967602038541,
137.025866330917));
#212499=CARTESIAN_POINT('Ctrl Pts',(-151.87559995937,4.03453985122072,136.034712724799));
#212500=CARTESIAN_POINT('Ctrl Pts',(-152.154047583183,6.58121069778455,
130.237121049039));
#212501=CARTESIAN_POINT('Ctrl Pts',(-152.432495206996,3.08007042310019,
124.960794825562));
#212502=CARTESIAN_POINT('Ctrl Pts',(-152.710942830809,-3.25150410060774,
125.054420090877));
#212503=CARTESIAN_POINT('Ctrl Pts',(-152.989390454622,-6.59510520066311,
130.431959800007));
#212504=CARTESIAN_POINT('Ctrl Pts',(-153.267838078435,-3.87812681010997,
136.151717667683));
#212505=CARTESIAN_POINT('Ctrl Pts',(-153.546285702248,2.40266066190714,
136.957515639215));
#212506=CARTESIAN_POINT('Ctrl Pts',(-153.824733326061,6.47552036213011,
132.108864744186));
#212507=CARTESIAN_POINT('Ctrl Pts',(-154.103180949873,4.59769319631231,
126.061438285362));
#212508=CARTESIAN_POINT('Ctrl Pts',(-154.381628573686,-1.50518940711724,
124.372525745196));
#212509=CARTESIAN_POINT('Ctrl Pts',(-154.660076197499,-6.22487647799626,
128.594155240135));
#212510=CARTESIAN_POINT('Ctrl Pts',(-154.938523821312,-5.22420616771914,
134.846855502398));
#212511=CARTESIAN_POINT('Ctrl Pts',(-155.216971445125,0.577254394032953,
137.384700452354));
#212512=CARTESIAN_POINT('Ctrl Pts',(-155.495419068938,5.84824636811312,
133.87553456161));
#212513=CARTESIAN_POINT('Ctrl Pts',(-155.773866692751,5.74498563261573,
127.544109851479));
#212514=CARTESIAN_POINT('Ctrl Pts',(-156.052314316564,0.362363758895462,
124.208696323275));
#212515=CARTESIAN_POINT('Ctrl Pts',(-156.330761940377,-5.353252706796,126.934376065411));
#212516=CARTESIAN_POINT('Ctrl Pts',(-156.60920956419,-6.14949145587554,
133.216382551721));
#212517=CARTESIAN_POINT('Ctrl Pts',(-156.887657188002,-1.29464797636456,
137.281858714364));
#212518=CARTESIAN_POINT('Ctrl Pts',(-157.166104811815,4.74991374635575,
135.394830569423));
#212519=CARTESIAN_POINT('Ctrl Pts',(-157.444552435628,6.42953678236183,
129.28938479565));
#212520=CARTESIAN_POINT('Ctrl Pts',(-157.723000059441,2.20072961571137,
124.576127791533));
#212521=CARTESIAN_POINT('Ctrl Pts',(-158.001447683254,-4.05044055615985,
125.586312488451));
#212522=CARTESIAN_POINT('Ctrl Pts',(-158.279895307067,-6.57945373194114,
131.391628500203));
#212523=CARTESIAN_POINT('Ctrl Pts',(-158.55834293088,-3.06227035225273,
136.657274017441));
#212524=CARTESIAN_POINT('Ctrl Pts',(-158.836790554693,3.2689898809326,136.54437805091));
#212525=CARTESIAN_POINT('Ctrl Pts',(-159.115238178505,6.59620811257463,
131.156686478575));
#212526=CARTESIAN_POINT('Ctrl Pts',(-159.393685802319,3.86183333144169,
125.445224652049));
#212527=CARTESIAN_POINT('Ctrl Pts',(-159.672133426131,-2.42137762023968,
124.658546969484));
#212528=CARTESIAN_POINT('Ctrl Pts',(-159.950581049944,-6.47946082979399,
129.519571789819));
#212529=CARTESIAN_POINT('Ctrl Pts',(-160.229028673757,-4.58323607602601,
135.56125477743));
#212530=CARTESIAN_POINT('Ctrl Pts',(-160.50747629757,1.52475872807955,137.231584419323));
#212531=CARTESIAN_POINT('Ctrl Pts',(-160.785923921383,6.23157474968534,
132.99560937474));
#212532=CARTESIAN_POINT('Ctrl Pts',(-161.064371545196,5.2118780056808,126.745983770767));
#212533=CARTESIAN_POINT('Ctrl Pts',(-161.342819169009,-0.597280011148509,
124.225808226271));
#212534=CARTESIAN_POINT('Ctrl Pts',(-161.621266792821,-5.85756687648338,
127.751000949223));
#212535=CARTESIAN_POINT('Ctrl Pts',(-161.899714416635,-5.73503594038016,
134.08208204247));
#212536=CARTESIAN_POINT('Ctrl Pts',(-162.178162040447,-0.342287147149402,
137.401097271823));
#212537=CARTESIAN_POINT('Ctrl Pts',(-162.45660966426,5.36500681265522,134.658033784415));
#212538=CARTESIAN_POINT('Ctrl Pts',(-162.735057288073,6.14212160678308,
128.373632919072));
#212539=CARTESIAN_POINT('Ctrl Pts',(-163.013504911886,1.27492670359879,
124.322952060995));
#212540=CARTESIAN_POINT('Ctrl Pts',(-163.291952535699,-4.76386355656041,
126.228369031995));
#212541=CARTESIAN_POINT('Ctrl Pts',(-163.570400159512,-6.42489593591386,
132.338898720518));
#212542=CARTESIAN_POINT('Ctrl Pts',(-163.848847783325,-2.18176282377798,
137.039262858781));
#212543=CARTESIAN_POINT('Ctrl Pts',(-164.127295407138,4.06630373837012,
136.010056429275));
#212544=CARTESIAN_POINT('Ctrl Pts',(-164.405743030951,6.57763581493773,
130.197069861187));
#212545=CARTESIAN_POINT('Ctrl Pts',(-164.684190654763,3.04444191295097,
124.942153830408));
#212546=CARTESIAN_POINT('Ctrl Pts',(-164.962638278576,-3.28644537778151,
125.074319452304));
#212547=CARTESIAN_POINT('Ctrl Pts',(-165.241085902389,-6.59724991811553,
130.472112977002));
#212548=CARTESIAN_POINT('Ctrl Pts',(-165.519533526202,-3.84550407727676,
136.175225852179));
#212549=CARTESIAN_POINT('Ctrl Pts',(-165.797981150015,2.44007214726114,
136.942775958099));
#212550=CARTESIAN_POINT('Ctrl Pts',(-166.076428773828,6.48334127261722,
132.069422244329));
#212551=CARTESIAN_POINT('Ctrl Pts',(-166.354876397641,4.56873649726763,
126.03353869726));
#212552=CARTESIAN_POINT('Ctrl Pts',(-166.633324021454,-1.54431392388507,
124.381807427344));
#212553=CARTESIAN_POINT('Ctrl Pts',(-166.911771645267,-6.23821529291649,
128.632088780075));
#212554=CARTESIAN_POINT('Ctrl Pts',(-167.19021926908,-5.19950156151742,
134.878581830081));
#212555=CARTESIAN_POINT('Ctrl Pts',(-167.468666892892,0.617300095144361,
137.381064622557));
#212556=CARTESIAN_POINT('Ctrl Pts',(-167.747114516705,5.86683312115408,
133.839877724298));
#212557=CARTESIAN_POINT('Ctrl Pts',(-168.025562140518,5.72503311955499,
127.509198898206));
#212558=CARTESIAN_POINT('Ctrl Pts',(-168.304009764331,0.32220736450136,
124.206612714607));
#212559=CARTESIAN_POINT('Ctrl Pts',(-168.582457388144,-5.37671121782417,
126.967034535923));
#212560=CARTESIAN_POINT('Ctrl Pts',(-168.860905011957,-6.1346948579149,
133.253771562468));
#212561=CARTESIAN_POINT('Ctrl Pts',(-169.13935263577,-1.25519362008691,
137.289619591024));
#212562=CARTESIAN_POINT('Ctrl Pts',(-169.417800259582,4.77776923498369,
135.365831445486));
#212563=CARTESIAN_POINT('Ctrl Pts',(-169.696247883396,6.42019557010726,
129.250274449328));
#212564=CARTESIAN_POINT('Ctrl Pts',(-169.974695507208,2.16277582029264,
124.562846720449));
#212565=CARTESIAN_POINT('Ctrl Pts',(-170.253143131021,-4.08212925089891,
125.611065348116));
#212566=CARTESIAN_POINT('Ctrl Pts',(-170.531590754834,-6.57575696361412,
131.431668621828));
#212567=CARTESIAN_POINT('Ctrl Pts',(-170.810038378647,-3.02658527035502,
136.675806485322));
#212568=CARTESIAN_POINT('Ctrl Pts',(-171.08848600246,3.30387042945021,136.524372432426));
#212569=CARTESIAN_POINT('Ctrl Pts',(-171.366933626273,6.59823060763395,
131.116526959784));
#212570=CARTESIAN_POINT('Ctrl Pts',(-171.645381250086,3.82913919888762,
125.421815868818));
#212571=CARTESIAN_POINT('Ctrl Pts',(-171.923828873899,-2.45874406978715,
124.673400450021));
#212572=CARTESIAN_POINT('Ctrl Pts',(-172.202276497711,-6.48716165465291,
129.559037911142));
#212573=CARTESIAN_POINT('Ctrl Pts',(-172.480724121525,-4.55419459435809,
135.589066102071));
#212574=CARTESIAN_POINT('Ctrl Pts',(-172.759171745337,1.5638548133772,137.222183698596));
#212575=CARTESIAN_POINT('Ctrl Pts',(-173.03761936915,6.24479804617409,132.957635411742));
#212576=CARTESIAN_POINT('Ctrl Pts',(-173.316066992963,5.18707694988104,
126.714332782362));
#212577=CARTESIAN_POINT('Ctrl Pts',(-173.594514616776,-0.637314460555731,
124.229565924566));
#212578=CARTESIAN_POINT('Ctrl Pts',(-173.872962240589,-5.8760450162844,
127.786714193059));
#212579=CARTESIAN_POINT('Ctrl Pts',(-174.151409864401,-5.71497726280517,
134.11693210545));
#212580=CARTESIAN_POINT('Ctrl Pts',(-174.429857488215,-0.302124596968923,
137.403058648589));
#212581=CARTESIAN_POINT('Ctrl Pts',(-174.708305112027,5.38836581387496,
134.625304065538));
#212582=CARTESIAN_POINT('Ctrl Pts',(-174.98675273584,6.1272112780718,128.336289117263));
#212583=CARTESIAN_POINT('Ctrl Pts',(-175.265200359654,1.2354489086321,124.315311305772));
#212584=CARTESIAN_POINT('Ctrl Pts',(-175.543647983466,-4.79163065280562,
126.257452804136));
#212585=CARTESIAN_POINT('Ctrl Pts',(-175.822095607279,-6.41543572848632,
132.377980454247));
#212586=CARTESIAN_POINT('Ctrl Pts',(-176.100543231092,-2.14376878114676,
137.05242835005));
#212587=CARTESIAN_POINT('Ctrl Pts',(-176.378990854905,4.09791694713909,
135.985207234778));
#212588=CARTESIAN_POINT('Ctrl Pts',(-176.657438478718,6.57381719537689,
130.157041176716));
#212589=CARTESIAN_POINT('Ctrl Pts',(-176.93588610253,3.00870058988678,124.923730061481));
#212590=CARTESIAN_POINT('Ctrl Pts',(-177.214333726344,-3.32126487451375,
125.094431142515));
#212591=CARTESIAN_POINT('Ctrl Pts',(-177.492781350156,-6.59915017204588,
130.512278465557));
#212592=CARTESIAN_POINT('Ctrl Pts',(-177.771228973969,-3.81273884787578,
136.198535017289));
#212593=CARTESIAN_POINT('Ctrl Pts',(-178.049676597782,2.47739321484437,
136.927808815745));
#212594=CARTESIAN_POINT('Ctrl Pts',(-178.328124221595,6.49092194050925,
132.029932867148));
#212595=CARTESIAN_POINT('Ctrl Pts',(-178.606571845408,4.53961050201187,
126.005815893719));
#212596=CARTESIAN_POINT('Ctrl Pts',(-178.885019469221,-1.58338121553252,
124.391327099562));
#212597=CARTESIAN_POINT('Ctrl Pts',(-179.163467093034,-6.25132294847495,
128.670102814346));
#212598=CARTESIAN_POINT('Ctrl Pts',(-179.441914716847,-5.1746042858732,
134.910157185999));
#212599=CARTESIAN_POINT('Ctrl Pts',(-179.72036234066,0.657322921973241,
137.377185090575));
#212600=CARTESIAN_POINT('Ctrl Pts',(-179.998809964472,5.88520247653593,
133.804108404782));
#212601=CARTESIAN_POINT('Ctrl Pts',(-180.277257588285,5.70486846328706,
127.474410048364));
#212602=CARTESIAN_POINT('Ctrl Pts',(-180.555705212098,0.282039030594865,
124.204773587913));
#212603=CARTESIAN_POINT('Ctrl Pts',(-180.834152835911,-5.39997049284089,
126.999835199963));
#212604=CARTESIAN_POINT('Ctrl Pts',(-181.112600459724,-6.11967093658025,
133.291069809391));
#212605=CARTESIAN_POINT('Ctrl Pts',(-181.391048083537,-1.21569275214809,
137.297140154028));
#212606=CARTESIAN_POINT('Ctrl Pts',(-181.669495707349,4.8054476816156,135.336663294571));
#212607=CARTESIAN_POINT('Ctrl Pts',(-181.947943331163,6.41061645514481,
129.21122169024));
#212608=CARTESIAN_POINT('Ctrl Pts',(-182.226390954976,2.12474188242055,
124.549796930959));
#212609=CARTESIAN_POINT('Ctrl Pts',(-182.504838578788,-4.11366668083735,
125.636010647245));
#212610=CARTESIAN_POINT('Ctrl Pts',(-182.783286202602,-6.5718165281946,
131.471685498325));
#212611=CARTESIAN_POINT('Ctrl Pts',(-183.061733826414,-2.99078803722709,
136.694121384618));
#212612=CARTESIAN_POINT('Ctrl Pts',(-183.340181450227,3.33862855183402,
136.5041548568));
#212613=CARTESIAN_POINT('Ctrl Pts',(-183.61862907404,6.60000860283161,131.076355873553));
#212614=CARTESIAN_POINT('Ctrl Pts',(-183.897076697853,3.79630317617236,
125.398606537762));
#212615=CARTESIAN_POINT('Ctrl Pts',(-184.175524321666,-2.49601940966891,
124.68848111554));
#212616=CARTESIAN_POINT('Ctrl Pts',(-184.453971945479,-6.49462209535141,
129.598550178357));
#212617=CARTESIAN_POINT('Ctrl Pts',(-184.732419569291,-4.52498435533419,
135.616700127691));
#212618=CARTESIAN_POINT('Ctrl Pts',(-185.010867193105,1.60289294946002,
137.212545163075));
#212619=CARTESIAN_POINT('Ctrl Pts',(-185.289314816917,6.25778993937471,
132.919581658354));
#212620=CARTESIAN_POINT('Ctrl Pts',(-185.56776244073,5.16208368503734,126.682833351442));
#212621=CARTESIAN_POINT('Ctrl Pts',(-185.846210064543,-0.677325294041226,
124.233567254297));
#212622=CARTESIAN_POINT('Ctrl Pts',(-186.124657688356,-5.89430541707644,
127.822539256894));
#212623=CARTESIAN_POINT('Ctrl Pts',(-186.403105312169,-5.69470681464601,
134.151659419877));
#212624=CARTESIAN_POINT('Ctrl Pts',(-186.681552935982,-0.261950851450417,
137.404775508174));
#212625=CARTESIAN_POINT('Ctrl Pts',(-186.960000559794,5.41152514721792,
134.592432760195));
#212626=CARTESIAN_POINT('Ctrl Pts',(-187.238448183608,6.11207390329327,
128.299036770752));
#212627=CARTESIAN_POINT('Ctrl Pts',(-187.51689580742,1.19592533365239,124.307911004657));
#212628=CARTESIAN_POINT('Ctrl Pts',(-187.795343431234,-4.81922019341476,
126.286705063617));
#212629=CARTESIAN_POINT('Ctrl Pts',(-188.073791055046,-6.40573779472858,
132.417003876913));
#212630=CARTESIAN_POINT('Ctrl Pts',(-188.352238678859,-2.10569530037498,
137.065362316871));
#212631=CARTESIAN_POINT('Ctrl Pts',(-188.630686302672,4.12937830608858,
135.960166062105));
#212632=CARTESIAN_POINT('Ctrl Pts',(-188.909133926485,6.56975498060235,
130.117036478904));
#212633=CARTESIAN_POINT('Ctrl Pts',(-189.187581550298,2.97284777831579,
124.905524201484));
#212634=CARTESIAN_POINT('Ctrl Pts',(-189.466029174111,-3.35596130055467,
125.114754416262));
#212635=CARTESIAN_POINT('Ctrl Pts',(-189.744476797923,-6.60080589203976,
130.552454777323));
#212636=CARTESIAN_POINT('Ctrl Pts',(-190.022924421737,-3.77983233603489,
136.221644299282));
#212637=CARTESIAN_POINT('Ctrl Pts',(-190.301372045549,2.5146224817104,136.912614766765));
#212638=CARTESIAN_POINT('Ctrl Pts',(-190.579819669362,6.49826208490189,
131.990398075938));
#212639=CARTESIAN_POINT('Ctrl Pts',(-190.858267293175,4.51031628981952,
125.978270902017));
#212640=CARTESIAN_POINT('Ctrl Pts',(-191.136714916988,-1.62238983440674,
124.401084409096));
#212641=CARTESIAN_POINT('Ctrl Pts',(-191.415162540801,-6.26419895896261,
128.708195934325));
#212642=CARTESIAN_POINT('Ctrl Pts',(-191.693610164614,-5.14951526336424,
134.941580400114));
#212643=CARTESIAN_POINT('Ctrl Pts',(-191.972057788427,0.697321391460013,
137.373062000163));
#212644=CARTESIAN_POINT('Ctrl Pts',(-192.25050541224,5.90335375357599,133.768227928508));
#212645=CARTESIAN_POINT('Ctrl Pts',(-192.528953036052,5.68449241101982,
127.439744591064));
#212646=CARTESIAN_POINT('Ctrl Pts',(-192.807400659866,0.241860245628379,
124.203179011344));
#212647=CARTESIAN_POINT('Ctrl Pts',(-193.085848283678,-5.42302966996514,
127.032776842093));
#212648=CARTESIAN_POINT('Ctrl Pts',(-193.364295907491,-6.10442024858855,
133.32827591039));
#212649=CARTESIAN_POINT('Ctrl Pts',(-193.642743531304,-1.17614683626724,
137.304420124699));
#212650=CARTESIAN_POINT('Ctrl Pts',(-193.921191155117,4.83294806061645,
135.307327197512));
#212651=CARTESIAN_POINT('Ctrl Pts',(-194.19963877893,6.40079979243214,129.172227965502));
#212652=CARTESIAN_POINT('Ctrl Pts',(-194.478086402743,2.08662921145659,
124.536978906625));
#212653=CARTESIAN_POINT('Ctrl Pts',(-194.756534026555,-4.14505167734362,
125.661147461485));
#212654=CARTESIAN_POINT('Ctrl Pts',(-195.034981650369,-6.5676325716969,
131.511677646851));
#212655=CARTESIAN_POINT('Ctrl Pts',(-195.313429274181,-2.95487997934909,
136.712218036662));
#212656=CARTESIAN_POINT('Ctrl Pts',(-195.591876897994,3.3732629601091,136.483726073203));
#212657=CARTESIAN_POINT('Ctrl Pts',(-195.870324521807,6.60154203228333,
131.03617470844));
#212658=CARTESIAN_POINT('Ctrl Pts',(-196.14877214562,3.76332648004682,125.375597518911));
#212659=CARTESIAN_POINT('Ctrl Pts',(-196.427219769433,-2.53320225863353,
124.703788407225));
#212660=CARTESIAN_POINT('Ctrl Pts',(-196.705667393246,-6.50184187543975,
129.63810712732));
#212661=CARTESIAN_POINT('Ctrl Pts',(-196.984115017059,-4.49560644135098,
135.644155830301));
#212662=CARTESIAN_POINT('Ctrl Pts',(-197.262562640871,1.64187168975517,
137.202669169918));
#212663=CARTESIAN_POINT('Ctrl Pts',(-197.541010264685,6.27054994786743,
132.881449524674));
#212664=CARTESIAN_POINT('Ctrl Pts',(-197.819457888497,5.13689913728475,
126.651486645231));
#212665=CARTESIAN_POINT('Ctrl Pts',(-198.097905512311,-0.717311028988463,
124.237812067191));
#212666=CARTESIAN_POINT('Ctrl Pts',(-198.376353136123,-5.91234740221361,
127.858474813215));
#212667=CARTESIAN_POINT('Ctrl Pts',(-198.654800759936,-5.67422534703162,
134.186262698915));
#212668=CARTESIAN_POINT('Ctrl Pts',(-198.933248383749,-0.221767399246752,
137.406247786956));
#212669=CARTESIAN_POINT('Ctrl Pts',(-199.211696007562,5.43448395450644,
134.559421086446));
#212670=CARTESIAN_POINT('Ctrl Pts',(-199.490143631375,6.09671004336861,
128.261877259937));
#212671=CARTESIAN_POINT('Ctrl Pts',(-199.768591255188,1.15635744321901,
124.300751431872));
#212672=CARTESIAN_POINT('Ctrl Pts',(-200.047038879001,-4.84663115604747,
126.316124726487));
#212673=CARTESIAN_POINT('Ctrl Pts',(-200.325486502814,-6.39580249400115,
132.455967542492));
#212674=CARTESIAN_POINT('Ctrl Pts',(-200.603934126626,-2.06754379228947,
137.078064279972));
#212675=CARTESIAN_POINT('Ctrl Pts',(-200.882381750439,4.16068664940635,
135.934933839164));
#212676=CARTESIAN_POINT('Ctrl Pts',(-201.160829374253,6.56544932114097,
130.077057250143));
#212677=CARTESIAN_POINT('Ctrl Pts',(-201.439276998065,2.9368848067771,124.887536925038));
#212678=CARTESIAN_POINT('Ctrl Pts',(-201.717724621878,-3.39053337021544,
125.13528852046));
#212679=CARTESIAN_POINT('Ctrl Pts',(-201.996172245691,-6.60221701674386,
130.592640423553));
#212680=CARTESIAN_POINT('Ctrl Pts',(-202.274619869504,-3.74678576111652,
136.244552841837));
#212681=CARTESIAN_POINT('Ctrl Pts',(-202.553067493317,2.55175856831618,
136.897194374181));
#212682=CARTESIAN_POINT('Ctrl Pts',(-202.83151511713,6.50536143380309,131.950819335672));
#212683=CARTESIAN_POINT('Ctrl Pts',(-203.109962740942,4.48085494619837,
125.950904742844));
#212684=CARTESIAN_POINT('Ctrl Pts',(-203.388410364755,-1.66133833502902,
124.411078994385));
#212685=CARTESIAN_POINT('Ctrl Pts',(-203.666857988568,-6.27684284725421,
128.746366728457));
#212686=CARTESIAN_POINT('Ctrl Pts',(-203.945305612381,-5.12423542367342,
134.97285030803));
#212687=CARTESIAN_POINT('Ctrl Pts',(-204.223753236194,0.737294021446153,
137.368695504108));
#212688=CARTESIAN_POINT('Ctrl Pts',(-204.502200860007,5.9212862796718,133.732237625041));
#212689=CARTESIAN_POINT('Ctrl Pts',(-204.78064848382,5.66390571779574,127.405203810847));
#212690=CARTESIAN_POINT('Ctrl Pts',(-205.059096107633,0.20167249844203,
124.201829043986));
#212691=CARTESIAN_POINT('Ctrl Pts',(-205.337543731446,-5.44588789473034,
127.065858241646));
#212692=CARTESIAN_POINT('Ctrl Pts',(-205.615991355258,-6.08894335906002,
133.36538848678));
#212693=CARTESIAN_POINT('Ctrl Pts',(-205.894438979071,-1.13655733783284,
137.311459233274));
#212694=CARTESIAN_POINT('Ctrl Pts',(-206.172886602884,4.86026935294961,
135.277824241371));
#212695=CARTESIAN_POINT('Ctrl Pts',(-206.451334226697,6.39074594572923,
129.133294720038));
#212696=CARTESIAN_POINT('Ctrl Pts',(-206.72978185051,2.04843921967989,124.524393122426));
#212697=CARTESIAN_POINT('Ctrl Pts',(-207.008229474323,-4.17628307743617,
125.686474859378));
#212698=CARTESIAN_POINT('Ctrl Pts',(-207.286677098136,-6.56320524915893,
131.551643585487));
#212699=CARTESIAN_POINT('Ctrl Pts',(-207.565124721949,-2.9188624273063,
136.730095770877));
#212700=CARTESIAN_POINT('Ctrl Pts',(-207.843572345762,3.40777237088467,
136.463086838631));
#212701=CARTESIAN_POINT('Ctrl Pts',(-208.122019969575,6.60283083916734,
130.995984953369));
#212702=CARTESIAN_POINT('Ctrl Pts',(-208.400467593387,3.73021033247459,
125.352789664874));
#212703=CARTESIAN_POINT('Ctrl Pts',(-208.678915217201,-2.57029123885685,
124.719321757855));
#212704=CARTESIAN_POINT('Ctrl Pts',(-208.957362841013,-6.50882072738636,
129.677707292235));
#212705=CARTESIAN_POINT('Ctrl Pts',(-209.235810464827,-4.4660619410178,
135.671432192519));
#212706=CARTESIAN_POINT('Ctrl Pts',(-209.514258088639,1.68078958989102,
137.192556085085));
#212707=CARTESIAN_POINT('Ctrl Pts',(-209.792705712452,6.28307759882623,
132.8432404237));
#212708=CARTESIAN_POINT('Ctrl Pts',(-210.071153336265,5.11152423984512,
126.620293825292));
#212709=CARTESIAN_POINT('Ctrl Pts',(-210.349600960078,-0.757270183712145,
124.242300205957));
#212710=CARTESIAN_POINT('Ctrl Pts',(-210.62804858389,-5.93017030314353,
127.894519530418));
#212711=CARTESIAN_POINT('Ctrl Pts',(-210.906496207704,-5.65353361891029,
134.220740660327));
#212712=CARTESIAN_POINT('Ctrl Pts',(-211.184943831516,-0.181575729370575,
137.407475430382));
#212713=CARTESIAN_POINT('Ctrl Pts',(-211.463391455329,5.4572413849935,134.52627026755));
#212714=CARTESIAN_POINT('Ctrl Pts',(-211.741839079142,6.08112026761121,
128.224811961777));
#212715=CARTESIAN_POINT('Ctrl Pts',(-212.020286702955,1.11674670353533,
124.293832852717));
#212716=CARTESIAN_POINT('Ctrl Pts',(-212.298734326768,-4.87386252498038,
126.345710702588));
#212717=CARTESIAN_POINT('Ctrl Pts',(-212.577181950581,-6.38563019446009,
132.494870007167));
#212718=CARTESIAN_POINT('Ctrl Pts',(-212.855629574394,-2.02931567060901,
137.090533768676));
#212719=CARTESIAN_POINT('Ctrl Pts',(-213.134077198207,4.19184081695006,
135.909511500946));
#212720=CARTESIAN_POINT('Ctrl Pts',(-213.412524822019,6.56090037654053,
130.037104971874));
#212721=CARTESIAN_POINT('Ctrl Pts',(-213.690972445832,2.90081300789186,
124.869768898671));
#212722=CARTESIAN_POINT('Ctrl Pts',(-213.969420069645,-3.42497980241531,
125.156032694208));
#212723=CARTESIAN_POINT('Ctrl Pts',(-214.247867693459,-6.60338349386843,
130.632833915152));
#212724=CARTESIAN_POINT('Ctrl Pts',(-214.52631531727,-3.71360034767391,
136.267259796069));
#212725=CARTESIAN_POINT('Ctrl Pts',(-214.804762941084,2.58880009856982,
136.881548209402));
#212726=CARTESIAN_POINT('Ctrl Pts',(-215.083210564897,6.51221972414398,
131.911198112957));
#212727=CARTESIAN_POINT('Ctrl Pts',(-215.36165818871,4.45122756284936,125.923718430264));
#212728=CARTESIAN_POINT('Ctrl Pts',(-215.640105812523,-1.70022527414834,
124.421310485075));
#212729=CARTESIAN_POINT('Ctrl Pts',(-215.918553436335,-6.28925414482577,
128.784613782311));
#212730=CARTESIAN_POINT('Ctrl Pts',(-216.197001060149,-5.09876570355457,
135.003965751026));
#212731=CARTESIAN_POINT('Ctrl Pts',(-216.475448683961,0.77723933073121,
137.364085764208));
#212732=CARTESIAN_POINT('Ctrl Pts',(-216.753896307774,5.93899939032692,
133.696138828015));
#212733=CARTESIAN_POINT('Ctrl Pts',(-217.032343931587,5.64310914646246,
127.370788987637));
#212734=CARTESIAN_POINT('Ctrl Pts',(-217.3107915554,0.161477278206604,124.200723735865));
#212735=CARTESIAN_POINT('Ctrl Pts',(-217.589239179213,-5.46854432011718,
127.099078172778));
#212736=CARTESIAN_POINT('Ctrl Pts',(-217.867686803026,-6.07324084149572,
133.402406163341));
#212737=CARTESIAN_POINT('Ctrl Pts',(-218.146134426838,-1.09692572384833,
137.318257218917));
#212738=CARTESIAN_POINT('Ctrl Pts',(-218.424582050652,4.88741054621452,
135.24815551939));
#212739=CARTESIAN_POINT('Ctrl Pts',(-218.703029674464,6.38045528758512,
129.094423396537));
#212740=CARTESIAN_POINT('Ctrl Pts',(-218.981477298277,2.01017332223456,
124.512040044732));
#212741=CARTESIAN_POINT('Ctrl Pts',(-219.25992492209,-4.20735972382344,
125.711991902411));
#212742=CARTESIAN_POINT('Ctrl Pts',(-219.538372545903,-6.55853472463687,
131.591581833275));
#212743=CARTESIAN_POINT('Ctrl Pts',(-219.816820169716,-2.8827367157428,
136.747753924796));
#212744=CARTESIAN_POINT('Ctrl Pts',(-220.095267793529,3.44215550540127,
136.442237917877));
#212745=CARTESIAN_POINT('Ctrl Pts',(-220.373715417342,6.60387497572639,
130.955788097589));
#212746=CARTESIAN_POINT('Ctrl Pts',(-220.652163041155,3.69695596058723,
125.330183820803));
#212747=CARTESIAN_POINT('Ctrl Pts',(-220.930610664968,-2.60728497599312,
124.735080591838));
#212748=CARTESIAN_POINT('Ctrl Pts',(-221.20905828878,-6.51555839258729,
129.717349205704));
#212749=CARTESIAN_POINT('Ctrl Pts',(-221.487505912593,-4.43635194911701,
135.698528203611));
#212750=CARTESIAN_POINT('Ctrl Pts',(-221.765953536406,1.71964520775051,
137.182206283321));
#212751=CARTESIAN_POINT('Ctrl Pts',(-222.044401160219,6.295372428034,132.804955771283));
#212752=CARTESIAN_POINT('Ctrl Pts',(-222.322848784032,5.08595993299503,
126.589256047487));
#212753=CARTESIAN_POINT('Ctrl Pts',(-222.601296407845,-0.797201277510683,
124.247031504286));
#212754=CARTESIAN_POINT('Ctrl Pts',(-222.879744031658,-5.94777345943203,
127.930672072853));
#212755=CARTESIAN_POINT('Ctrl Pts',(-223.158191655471,-5.63263239702162,
134.255092026522));
#212756=CARTESIAN_POINT('Ctrl Pts',(-223.436639279283,-0.141377331138957,
137.40845839296));
#212757=CARTESIAN_POINT('Ctrl Pts',(-223.715086903097,5.47979659539413,
134.492981531924));
#212758=CARTESIAN_POINT('Ctrl Pts',(-223.993534526909,6.06530515370598,
128.187842249741));
#212759=CARTESIAN_POINT('Ctrl Pts',(-224.271982150722,1.07709458239186,
124.287155523561));
#212760=CARTESIAN_POINT('Ctrl Pts',(-224.550429774535,-4.90091329114502,
126.375461895601));
#212761=CARTESIAN_POINT('Ctrl Pts',(-224.828877398348,-6.37522127304402,
132.533709829396));
#212762=CARTESIAN_POINT('Ctrl Pts',(-225.107325022161,-1.99101235188949,
137.102770320923));
#212763=CARTESIAN_POINT('Ctrl Pts',(-225.385772645974,4.22283965429091,
135.883899989486));
#212764=CARTESIAN_POINT('Ctrl Pts',(-225.664220269787,6.55610831536389,
129.997181124546));
#212765=CARTESIAN_POINT('Ctrl Pts',(-225.9426678936,2.86463371831382,124.852220780782));
#212766=CARTESIAN_POINT('Ctrl Pts',(-226.221115517412,-3.45929932072906,
125.176986168825));
#212767=CARTESIAN_POINT('Ctrl Pts',(-226.499563141226,-6.60430528018926,
130.673033762736));
#212768=CARTESIAN_POINT('Ctrl Pts',(-226.778010765038,-3.68027732540471,
136.289764320562));
#212769=CARTESIAN_POINT('Ctrl Pts',(-227.056458388851,2.62574569988376,
136.865676852203));
#212770=CARTESIAN_POINT('Ctrl Pts',(-227.334906012664,6.51883670178814,
131.871535875972));
#212771=CARTESIAN_POINT('Ctrl Pts',(-227.613353636477,4.42143523762624,
125.896712971676));
#212772=CARTESIAN_POINT('Ctrl Pts',(-227.89180126029,-1.73904921079426,
124.431778502036));
#212773=CARTESIAN_POINT('Ctrl Pts',(-228.170248884103,-6.30143239177224,
128.822935678624));
#212774=CARTESIAN_POINT('Ctrl Pts',(-228.448696507916,-5.07310704679746,
135.034925576111));
#212775=CARTESIAN_POINT('Ctrl Pts',(-228.727144131728,0.81715583912702,
137.359232951281));
#212776=CARTESIAN_POINT('Ctrl Pts',(-229.005591755541,5.95649242917557,
133.659932875084));
#212777=CARTESIAN_POINT('Ctrl Pts',(-229.284039379354,5.62210346764449,
127.336501396687));
#212778=CARTESIAN_POINT('Ctrl Pts',(-229.562487003167,0.121276074371264,
124.199863127936));
#212779=CARTESIAN_POINT('Ctrl Pts',(-229.84093462698,-5.4909981065832,127.132435404515));
#212780=CARTESIAN_POINT('Ctrl Pts',(-230.119382250793,-6.0573132777586,
133.439327568368));
#212781=CARTESIAN_POINT('Ctrl Pts',(-230.397829874606,-1.05725346287773,
137.324813829725));
#212782=CARTESIAN_POINT('Ctrl Pts',(-230.676277498418,4.91437063468431,
135.218322130955));
#212783=CARTESIAN_POINT('Ctrl Pts',(-230.954725122232,6.3699281993239,129.055615435388));
#212784=CARTESIAN_POINT('Ctrl Pts',(-231.233172746044,1.97183293707754,
124.49992013129));
#212785=CARTESIAN_POINT('Ctrl Pts',(-231.511620369858,-4.23828046494889,
125.73769764504));
#212786=CARTESIAN_POINT('Ctrl Pts',(-231.79006799367,-6.55362117119865,
131.631490910294));
#212787=CARTESIAN_POINT('Ctrl Pts',(-232.068515617483,-2.84650418331021,
136.765191844092));
#212788=CARTESIAN_POINT('Ctrl Pts',(-232.346963241296,3.47641108958031,
136.421180083507));
#212789=CARTESIAN_POINT('Ctrl Pts',(-232.625410865109,6.60467440326965,
130.915585630608));
#212790=CARTESIAN_POINT('Ctrl Pts',(-232.903858488922,3.66356459663667,
125.307780824367));
#212791=CARTESIAN_POINT('Ctrl Pts',(-233.182306112735,-2.64418209922576,
124.751064325225));
#212792=CARTESIAN_POINT('Ctrl Pts',(-233.460753736548,-6.52205462137589,
129.75703139878));
#212793=CARTESIAN_POINT('Ctrl Pts',(-233.73920136036,-4.40647756656326,
135.725442859523));
#212794=CARTESIAN_POINT('Ctrl Pts',(-234.017648984174,1.75843710352442,
137.17162014814));
#212795=CARTESIAN_POINT('Ctrl Pts',(-234.296096607986,6.30743397990132,
132.766596986079));
#212796=CARTESIAN_POINT('Ctrl Pts',(-234.574544231799,5.06020716402928,
126.558374461932));
#212797=CARTESIAN_POINT('Ctrl Pts',(-234.852991855612,-0.837102830722735,
124.252005786856));
#212798=CARTESIAN_POINT('Ctrl Pts',(-235.131439479425,-5.96515621878728,
127.966931100874));
#212799=CARTESIAN_POINT('Ctrl Pts',(-235.409887103238,-5.6115224558684,
134.289315524594));
#212800=CARTESIAN_POINT('Ctrl Pts',(-235.688334727051,-0.101173694118813,
137.409196638266));
#212801=CARTESIAN_POINT('Ctrl Pts',(-235.966782350864,5.50214874991674,
134.459556113093));
#212802=CARTESIAN_POINT('Ctrl Pts',(-236.245229974676,6.04926528768773,
128.150969493757));
#212803=CARTESIAN_POINT('Ctrl Pts',(-236.52367759849,1.03740254911254,124.280719691838));
#212804=CARTESIAN_POINT('Ctrl Pts',(-236.802125222302,-4.92778245216537,
126.405377203086));
#212805=CARTESIAN_POINT('Ctrl Pts',(-237.080572846115,-6.36457611545918,
132.572485569954));
#212806=CARTESIAN_POINT('Ctrl Pts',(-237.359020469928,-1.95263525547508,
137.114773483282));
#212807=CARTESIAN_POINT('Ctrl Pts',(-237.637468093741,4.25368201275546,
135.858100253825));
#212808=CARTESIAN_POINT('Ctrl Pts',(-237.915915717553,6.55107331518259,
129.957287187551));
#212809=CARTESIAN_POINT('Ctrl Pts',(-238.194363341367,2.8283482786799,124.834893221623));
#212810=CARTESIAN_POINT('Ctrl Pts',(-238.47281096518,-3.49349065343433,
125.198148167872));
#212811=CARTESIAN_POINT('Ctrl Pts',(-238.751258588993,-6.60498234154917,
130.713238476685));
#212812=CARTESIAN_POINT('Ctrl Pts',(-239.029706212805,-3.64681792910581,
136.312065581403));
#212813=CARTESIAN_POINT('Ctrl Pts',(-239.308153836619,2.66259400322518,
136.8495808907));
#212814=CARTESIAN_POINT('Ctrl Pts',(-239.586601460431,6.52521212154101,
131.831834094415));
#212815=CARTESIAN_POINT('Ctrl Pts',(-239.865049084244,4.39147907449425,
125.869889367774));
#212816=CARTESIAN_POINT('Ctrl Pts',(-240.143496708057,-1.77780870633274,
124.44248265737));
#212817=CARTESIAN_POINT('Ctrl Pts',(-240.42194433187,-6.31337713682396,
128.861330997368));
#212818=CARTESIAN_POINT('Ctrl Pts',(-240.700391955683,-5.04726040419313,
135.065728636055));
#212819=CARTESIAN_POINT('Ctrl Pts',(-240.978839579496,0.857042067512721,
137.354137245149));
#212820=CARTESIAN_POINT('Ctrl Pts',(-241.257287203309,5.97376474800676,
133.623621107872));
#212821=CARTESIAN_POINT('Ctrl Pts',(-241.535734827122,5.60088945971499,
127.302342308534));
#212822=CARTESIAN_POINT('Ctrl Pts',(-241.814182450934,0.0810703766063902,
124.199247252091));
#212823=CARTESIAN_POINT('Ctrl Pts',(-242.092630074747,-5.51324842209508,
127.165928700792));
#212824=CARTESIAN_POINT('Ctrl Pts',(-242.37107769856,-6.04116125805038,
133.476151333726));
#212825=CARTESIAN_POINT('Ctrl Pts',(-242.649525322373,-1.01754202499167,
137.331128822742));
#212826=CARTESIAN_POINT('Ctrl Pts',(-242.927972946186,4.94114861934255,
135.188325181553));
#212827=CARTESIAN_POINT('Ctrl Pts',(-243.206420569999,6.35916507103108,
129.016872274634));
#212828=CARTESIAN_POINT('Ctrl Pts',(-243.484868193812,1.93341948492588,
124.488033831209));
#212829=CARTESIAN_POINT('Ctrl Pts',(-243.763315817625,-4.26904415503308,
125.763591134728));
#212830=CARTESIAN_POINT('Ctrl Pts',(-244.041763441437,-6.54846477091785,
131.671369337695));
#212831=CARTESIAN_POINT('Ctrl Pts',(-244.320211065251,-2.8101661726183,
136.782408882594));
#212832=CARTESIAN_POINT('Ctrl Pts',(-244.598658689063,3.51053785406796,
136.399914115825));
#212833=CARTESIAN_POINT('Ctrl Pts',(-244.877106312876,6.60522909217403,
130.875379042142));
#212834=CARTESIAN_POINT('Ctrl Pts',(-245.155553936689,3.6300374779527,125.285581505715));
#212835=CARTESIAN_POINT('Ctrl Pts',(-245.434001560502,-2.68098124131831,
124.767272365732));
#212836=CARTESIAN_POINT('Ctrl Pts',(-245.712449184315,-6.528309173032,129.796752401026));
#212837=CARTESIAN_POINT('Ctrl Pts',(-245.990896808128,-4.37643990036281,
135.752175162922));
#212838=CARTESIAN_POINT('Ctrl Pts',(-246.269344431941,1.79716383976481,
137.160798071814));
#212839=CARTESIAN_POINT('Ctrl Pts',(-246.547792055753,6.31926180748295,
132.728165489484));
#212840=CARTESIAN_POINT('Ctrl Pts',(-246.826239679567,5.03426688722615,
126.527650212955));
#212841=CARTESIAN_POINT('Ctrl Pts',(-247.104687303379,-0.876973364781528,
124.257222869343));
#212842=CARTESIAN_POINT('Ctrl Pts',(-247.383134927193,-5.98231793708558,
128.003295270889));
#212843=CARTESIAN_POINT('Ctrl Pts',(-247.661582551005,-5.59020457768662,
134.32340988638));
#212844=CARTESIAN_POINT('Ctrl Pts',(-247.940030174818,-0.0609663080697638,
137.409690138946));
#212845=CARTESIAN_POINT('Ctrl Pts',(-248.218477798631,5.524297020294,134.425995249648));
#212846=CARTESIAN_POINT('Ctrl Pts',(-248.496925422444,6.03300126391963,
128.114195060156));
#212847=CARTESIAN_POINT('Ctrl Pts',(-248.775373046256,0.997672074500306,
124.274525596028));
#212848=CARTESIAN_POINT('Ctrl Pts',(-249.05382067007,-4.95446901239483,
126.435455516518));
#212849=CARTESIAN_POINT('Ctrl Pts',(-249.332268293882,-6.35369511616563,
132.611195791991));
#212850=CARTESIAN_POINT('Ctrl Pts',(-249.610715917695,-1.91418580344349,
137.126542810973));
#212851=CARTESIAN_POINT('Ctrl Pts',(-249.889163541508,4.28436674946925,
135.832113249982));
#212852=CARTESIAN_POINT('Ctrl Pts',(-250.167611165321,6.54579556256923,
129.917424639176));
#212853=CARTESIAN_POINT('Ctrl Pts',(-250.446058789134,2.79195803356287,
124.817786863269));
#212854=CARTESIAN_POINT('Ctrl Pts',(-250.724506412947,-3.52755253356211,
125.219517907192));
#212855=CARTESIAN_POINT('Ctrl Pts',(-251.00295403676,-6.60541465285253,
130.75344656718));
#212856=CARTESIAN_POINT('Ctrl Pts',(-251.281401660573,-3.61322339864049,
136.334162752248));
#212857=CARTESIAN_POINT('Ctrl Pts',(-251.559849284386,2.6993436431913,136.83326092127));
#212858=CARTESIAN_POINT('Ctrl Pts',(-251.838296908198,6.53134574711249,
131.792094239578));
#212859=CARTESIAN_POINT('Ctrl Pts',(-252.116744532012,4.3613601835781,125.843248612281));
#212860=CARTESIAN_POINT('Ctrl Pts',(-252.395192155824,-1.81650232468185,
124.453422554885));
#212861=CARTESIAN_POINT('Ctrl Pts',(-252.673639779637,-6.32508793705065,
128.899798314935));
#212862=CARTESIAN_POINT('Ctrl Pts',(-252.95208740345,-5.02122673409033,
135.096373791053));
#212863=CARTESIAN_POINT('Ctrl Pts',(-253.230535027263,0.896896539007115,
137.348798831588));
#212864=CARTESIAN_POINT('Ctrl Pts',(-253.508982651076,5.99081570467794,
133.587204877683));
#212865=CARTESIAN_POINT('Ctrl Pts',(-253.787430274889,5.57946791275175,
127.26831297809));
#212866=CARTESIAN_POINT('Ctrl Pts',(-254.065877898701,0.0408616672245685,
124.198876151673));
#212867=CARTESIAN_POINT('Ctrl Pts',(-254.344325522515,-5.53529442795169,
127.199556781751));
#212868=CARTESIAN_POINT('Ctrl Pts',(-254.622773146327,-6.0247854077167,
133.512876168065));
#212869=CARTESIAN_POINT('Ctrl Pts',(-254.90122077014,-0.977792831057213,
137.337201825807));
#212870=CARTESIAN_POINT('Ctrl Pts',(-255.179668393953,4.96774341227684,
135.158166043599));
#212871=CARTESIAN_POINT('Ctrl Pts',(-255.458116017766,6.34816648213513,
128.97819485735));
#212872=CARTESIAN_POINT('Ctrl Pts',(-255.736563641579,1.89493404819936,
124.476382515012));
#212873=CARTESIAN_POINT('Ctrl Pts',(-256.015011265392,-4.29964901022966,
125.789669655819));
#212874=CARTESIAN_POINT('Ctrl Pts',(-256.293458889205,-6.54306693065544,
131.711218953762));
#212875=CARTESIAN_POINT('Ctrl Pts',(-256.571906513018,-2.77372173452912,
136.799398141047));
#212876=CARTESIAN_POINT('Ctrl Pts',(-256.85035413683,3.54453019961847,136.378452625405));
#212877=CARTESIAN_POINT('Ctrl Pts',(-257.128801760644,6.60554720661629,
130.835147498674));
#212878=CARTESIAN_POINT('Ctrl Pts',(-257.407249384456,3.5963603924579,125.263628838565));
#212879=CARTESIAN_POINT('Ctrl Pts',(-257.685697008269,-2.71765185753996,
124.783624522784));
#212880=CARTESIAN_POINT('Ctrl Pts',(-257.964144632082,-6.53437691572335,
129.836661023534));
#212881=CARTESIAN_POINT('Ctrl Pts',(-258.242592255895,-4.34613602341029,
135.778440351053));
#212882=CARTESIAN_POINT('Ctrl Pts',(-258.521039879708,1.83562753012831,
137.150276335207));
#212883=CARTESIAN_POINT('Ctrl Pts',(-258.799487503521,6.33122643152078,
132.688650362788));
#212884=CARTESIAN_POINT('Ctrl Pts',(-259.077935127334,5.00743946241547,
126.498999976245));
#212885=CARTESIAN_POINT('Ctrl Pts',(-259.356382751147,-0.915487258132909,
124.259032700089));
#212886=CARTESIAN_POINT('Ctrl Pts',(-259.634830374959,-6.00176822571329,
128.046924274587));
#212887=CARTESIAN_POINT('Ctrl Pts',(-259.86687006147,-5.63687269779404,
133.292521465648));
#212888=CARTESIAN_POINT('Ctrl Pts',(-260.052531023546,-2.79481741349804,
135.900547185714));
#212889=CARTESIAN_POINT('Ctrl Pts',(-260.145376111017,-0.946914048523564,
136.386386345067));
#212890=CARTESIAN_POINT('Ctrl Pts',(-260.191813261187,-0.0157913329746497,
136.389009763222));
#212891=CARTESIAN_POINT('Ctrl Pts',(210.190947297731,3.04870273111253,135.077142573452));
#212892=CARTESIAN_POINT('Ctrl Pts',(210.144529434129,3.76080111712433,134.569051946243));
#212893=CARTESIAN_POINT('Ctrl Pts',(210.051703633225,4.91317831978039,133.192256847685));
#212894=CARTESIAN_POINT('Ctrl Pts',(209.866061957716,5.67455722768035,129.648049455111));
#212895=CARTESIAN_POINT('Ctrl Pts',(209.634022271206,3.10293383059235,125.427666478792));
#212896=CARTESIAN_POINT('Ctrl Pts',(209.355574647392,-2.85596866243967,
125.28812524467));
#212897=CARTESIAN_POINT('Ctrl Pts',(209.07712702358,-6.17973736462657,130.225196103446));
#212898=CARTESIAN_POINT('Ctrl Pts',(208.798679399767,-3.83016968018938,
135.690661498217));
#212899=CARTESIAN_POINT('Ctrl Pts',(208.520231775954,2.04205955310628,136.667868212554));
#212900=CARTESIAN_POINT('Ctrl Pts',(208.241784152142,6.03618933210081,132.255733564264));
#212901=CARTESIAN_POINT('Ctrl Pts',(207.963336528328,4.48417485225333,126.510421532214));
#212902=CARTESIAN_POINT('Ctrl Pts',(207.684888904515,-1.18901089957204,
124.710731370568));
#212903=CARTESIAN_POINT('Ctrl Pts',(207.406441280703,-5.76932406256156,
128.510946815645));
#212904=CARTESIAN_POINT('Ctrl Pts',(207.12799365689,-5.04803188696711,134.418613818075));
#212905=CARTESIAN_POINT('Ctrl Pts',(206.849546033077,0.312219397189005,
137.005003016302));
#212906=CARTESIAN_POINT('Ctrl Pts',(206.571098409264,5.38552219392035,133.893281295751));
#212907=CARTESIAN_POINT('Ctrl Pts',(206.292650785451,5.50981125882569,127.943004805273));
#212908=CARTESIAN_POINT('Ctrl Pts',(206.014203161638,0.570843377758803,
124.622167937696));
#212909=CARTESIAN_POINT('Ctrl Pts',(205.735755537825,-4.89269661278007,
126.982467612715));
#212910=CARTESIAN_POINT('Ctrl Pts',(205.457307914013,-5.86009012142741,
132.854898402769));
#212911=CARTESIAN_POINT('Ctrl Pts',(205.178860290199,-1.44234566848361,
136.842986120511));
#212912=CARTESIAN_POINT('Ctrl Pts',(204.900412666387,4.30084323855829,135.281871486376));
#212913=CARTESIAN_POINT('Ctrl Pts',(204.621965042573,6.09176771588946,129.606143376667));
#212914=CARTESIAN_POINT('Ctrl Pts',(204.343517418761,2.28465505058828,125.031518229909));
#212915=CARTESIAN_POINT('Ctrl Pts',(204.065069794948,-3.62194388278553,
125.761853295313));
#212916=CARTESIAN_POINT('Ctrl Pts',(203.786622171135,-6.20015338889199,
131.126006208945));
#212917=CARTESIAN_POINT('Ctrl Pts',(203.508174547322,-3.08072479357708,
136.194582558939));
#212918=CARTESIAN_POINT('Ctrl Pts',(203.229726923509,2.86973936865286,136.309808260363));
#212919=CARTESIAN_POINT('Ctrl Pts',(202.951279299696,6.1830532544492,131.365796540178));
#212920=CARTESIAN_POINT('Ctrl Pts',(202.672831675884,3.81444325369211,125.905852631576));
#212921=CARTESIAN_POINT('Ctrl Pts',(202.39438405207,-2.05945374882828,124.947398258377));
#212922=CARTESIAN_POINT('Ctrl Pts',(202.115936428258,-6.04081336739099,
129.371206163854));
#212923=CARTESIAN_POINT('Ctrl Pts',(201.837488804444,-4.47096061076856,
135.112012999282));
#212924=CARTESIAN_POINT('Ctrl Pts',(201.559041180632,1.20748652821524,136.894297736177));
#212925=CARTESIAN_POINT('Ctrl Pts',(201.280593556819,5.77631253695961,133.08022777117));
#212926=CARTESIAN_POINT('Ctrl Pts',(201.002145933006,5.03698951269057,127.174747074221));
#212927=CARTESIAN_POINT('Ctrl Pts',(200.723698309193,-0.331080803069094,
124.604703907164));
#212928=CARTESIAN_POINT('Ctrl Pts',(200.44525068538,-5.39490403503349,127.731842386878));
#212929=CARTESIAN_POINT('Ctrl Pts',(200.166803061567,-5.50107401450091,
133.682475019745));
#212930=CARTESIAN_POINT('Ctrl Pts',(199.888355437754,-0.552025717056,136.988261120707));
#212931=CARTESIAN_POINT('Ctrl Pts',(199.609907813942,4.90430724641216,134.611344759621));
#212932=CARTESIAN_POINT('Ctrl Pts',(199.331460190128,5.85382143915379,128.735995953499));
#212933=CARTESIAN_POINT('Ctrl Pts',(199.053012566316,1.42395970438994,124.761373228423));
#212934=CARTESIAN_POINT('Ctrl Pts',(198.774564942502,-4.31445143441004,
126.339960697623));
#212935=CARTESIAN_POINT('Ctrl Pts',(198.49611731869,-6.088092477657,132.02111359519));
#212936=CARTESIAN_POINT('Ctrl Pts',(198.217669694877,-2.26707395378944,
136.584129948007));
#212937=CARTESIAN_POINT('Ctrl Pts',(197.939222071064,3.6372747808909,135.835820643578));
#212938=CARTESIAN_POINT('Ctrl Pts',(197.660774447251,6.19914568268399,130.46384537573));
#212939=CARTESIAN_POINT('Ctrl Pts',(197.382326823438,3.06430454719326,125.404786980035));
#212940=CARTESIAN_POINT('Ctrl Pts',(197.103879199626,-2.88648276756863,
125.307672973393));
#212941=CARTESIAN_POINT('Ctrl Pts',(196.825431575812,-6.1847334314575,130.261746383626));
#212942=CARTESIAN_POINT('Ctrl Pts',(196.546983952,-3.79951621286212,135.71445576667));
#212943=CARTESIAN_POINT('Ctrl Pts',(196.268536328187,2.07727078866752,136.65502757917));
#212944=CARTESIAN_POINT('Ctrl Pts',(195.990088704374,6.04514741573133,132.219122274927));
#212945=CARTESIAN_POINT('Ctrl Pts',(195.711641080561,4.45782888960729,126.483120122517));
#212946=CARTESIAN_POINT('Ctrl Pts',(195.433193456748,-1.22601660901765,
124.718126880723));
#212947=CARTESIAN_POINT('Ctrl Pts',(195.154745832935,-5.78321273819644,
128.54608511404));
#212948=CARTESIAN_POINT('Ctrl Pts',(194.876298209123,-5.02591888662151,
134.449288212205));
#212949=CARTESIAN_POINT('Ctrl Pts',(194.597850585309,0.349948891971121,
137.002980915508));
#212950=CARTESIAN_POINT('Ctrl Pts',(194.319402961497,5.40423073479611,133.860444384439));
#212951=CARTESIAN_POINT('Ctrl Pts',(194.040955337684,5.49228854369214,127.909516169605));
#212952=CARTESIAN_POINT('Ctrl Pts',(193.762507713871,0.533201494146887,
124.618808581434));
#212953=CARTESIAN_POINT('Ctrl Pts',(193.484060090058,-4.91587168017823,
127.012321133451));
#212954=CARTESIAN_POINT('Ctrl Pts',(193.205612466245,-5.84749893410212,
132.890532719942));
#212955=CARTESIAN_POINT('Ctrl Pts',(192.927164842432,-1.40556033379022,
136.851654059523));
#212956=CARTESIAN_POINT('Ctrl Pts',(192.648717218619,4.32801954783523,135.255608152653));
#212957=CARTESIAN_POINT('Ctrl Pts',(192.370269594806,6.08436090050943,129.569083216569));
#212958=CARTESIAN_POINT('Ctrl Pts',(192.091821970994,2.24947182316989,125.017717865345));
#212959=CARTESIAN_POINT('Ctrl Pts',(191.81337434718,-3.65257196685492,125.783994510198));
#212960=CARTESIAN_POINT('Ctrl Pts',(191.534926723368,-6.19808055740059,
131.163742349203));
#212961=CARTESIAN_POINT('Ctrl Pts',(191.256479099555,-3.04785590876364,
136.213235933607));
#212962=CARTESIAN_POINT('Ctrl Pts',(190.978031475742,2.90319942398833,136.292237340818));
#212963=CARTESIAN_POINT('Ctrl Pts',(190.699583851929,6.18635631527163,131.328148137043));
#212964=CARTESIAN_POINT('Ctrl Pts',(190.421136228116,3.7845539731278,125.882723791311));
#212965=CARTESIAN_POINT('Ctrl Pts',(190.142688604304,-2.09506858458051,
124.960043253581));
#212966=CARTESIAN_POINT('Ctrl Pts',(189.86424098049,-6.04942546284962,129.408004862578));
#212967=CARTESIAN_POINT('Ctrl Pts',(189.585793356678,-4.44465587162338,
135.139149194637));
#212968=CARTESIAN_POINT('Ctrl Pts',(189.307345732864,1.24453533211424,136.886834590562));
#212969=CARTESIAN_POINT('Ctrl Pts',(189.028898109051,5.79005936456987,133.045023550676));
#212970=CARTESIAN_POINT('Ctrl Pts',(188.750450485239,5.01480170111087,127.144152737732));
#212971=CARTESIAN_POINT('Ctrl Pts',(188.472002861426,-0.368813738986236,
124.606834155258));
#212972=CARTESIAN_POINT('Ctrl Pts',(188.193555237613,-5.41350737050784,
127.764739625646));
#212973=CARTESIAN_POINT('Ctrl Pts',(187.9151076138,-5.48345219307025,133.715908293866));
#212974=CARTESIAN_POINT('Ctrl Pts',(187.636659989987,-0.51437233173317,
136.991506884579));
#212975=CARTESIAN_POINT('Ctrl Pts',(187.358212366174,4.92739057398128,134.581420314804));
#212976=CARTESIAN_POINT('Ctrl Pts',(187.079764742362,5.84112225861874,128.700400402891));
#212977=CARTESIAN_POINT('Ctrl Pts',(186.801317118548,1.38714794227173,124.752817144095));
#212978=CARTESIAN_POINT('Ctrl Pts',(186.522869494736,-4.34154756707868,
126.366306703083));
#212979=CARTESIAN_POINT('Ctrl Pts',(186.244421870923,-6.08057295867359,
132.058150998494));
#212980=CARTESIAN_POINT('Ctrl Pts',(185.96597424711,-2.23184885375068,136.597823184897));
#212981=CARTESIAN_POINT('Ctrl Pts',(185.687526623297,3.66783531589119,135.813586298303));
#212982=CARTESIAN_POINT('Ctrl Pts',(185.409078999484,6.19695801394562,130.42611572539));
#212983=CARTESIAN_POINT('Ctrl Pts',(185.130631375671,3.03137903541329,125.386233730096));
#212984=CARTESIAN_POINT('Ctrl Pts',(184.852183751858,-2.9198891855651,125.325345654173));
#212985=CARTESIAN_POINT('Ctrl Pts',(184.573736128045,-6.18792188952598,
130.299404664846));
#212986=CARTESIAN_POINT('Ctrl Pts',(184.295288504232,-3.76955667380246,
135.737493527599));
#212987=CARTESIAN_POINT('Ctrl Pts',(184.01684088042,2.11284697206427,136.642274242971));
#212988=CARTESIAN_POINT('Ctrl Pts',(183.738393256607,6.05364746891681,132.182297534532));
#212989=CARTESIAN_POINT('Ctrl Pts',(183.459945632794,4.43144167895468,126.456064115361));
#212990=CARTESIAN_POINT('Ctrl Pts',(183.181498008981,-1.2630425260055,124.725702755623));
#212991=CARTESIAN_POINT('Ctrl Pts',(182.903050385168,-5.79685235262429,
128.581331012064));
#212992=CARTESIAN_POINT('Ctrl Pts',(182.624602761355,-5.00363805916239,
134.479814874928));
#212993=CARTESIAN_POINT('Ctrl Pts',(182.346155137542,0.387675169361259,
137.000735831198));
#212994=CARTESIAN_POINT('Ctrl Pts',(182.06770751373,5.42273385622678,133.827490675898));
#212995=CARTESIAN_POINT('Ctrl Pts',(181.789259889916,5.47456504449634,127.876136685104));
#212996=CARTESIAN_POINT('Ctrl Pts',(181.510812266103,0.495538404244469,
124.615677436551));
#212997=CARTESIAN_POINT('Ctrl Pts',(181.232364642291,-4.93886382111119,
127.042315697369));
#212998=CARTESIAN_POINT('Ctrl Pts',(180.953917018477,-5.83469147177671,
132.926089453735));
#212999=CARTESIAN_POINT('Ctrl Pts',(180.675469394665,-1.36872270040423,
136.860098061879));
#213000=CARTESIAN_POINT('Ctrl Pts',(180.397021770852,4.35503536681857,135.229179797918));
#213001=CARTESIAN_POINT('Ctrl Pts',(180.118574147039,6.07672868724052,129.532068871648));
#213002=CARTESIAN_POINT('Ctrl Pts',(179.840126523226,2.21420520878857,125.004131904969));
#213003=CARTESIAN_POINT('Ctrl Pts',(179.561678899413,-3.68306468660213,
125.80632176824));
#213004=CARTESIAN_POINT('Ctrl Pts',(179.2832312756,-6.19577806271818,131.20146516627));
#213005=CARTESIAN_POINT('Ctrl Pts',(179.004783651788,-3.01487407978163,
136.231688883676));
#213006=CARTESIAN_POINT('Ctrl Pts',(178.726336027974,2.93655189768736,136.274463064253));
#213007=CARTESIAN_POINT('Ctrl Pts',(178.447888404162,6.18943013971724,131.290480325685));
#213008=CARTESIAN_POINT('Ctrl Pts',(178.169440780348,3.75452445381909,125.859777323623));
#213009=CARTESIAN_POINT('Ctrl Pts',(177.890993156536,-2.13060578642238,
124.972904812372));
#213010=CARTESIAN_POINT('Ctrl Pts',(177.612545532723,-6.05781339482078,
129.44485530364));
#213011=CARTESIAN_POINT('Ctrl Pts',(177.33409790891,-4.41818643401566,135.166124762878));
#213012=CARTESIAN_POINT('Ctrl Pts',(177.055650285097,1.28153801924328,136.879146056599));
#213013=CARTESIAN_POINT('Ctrl Pts',(176.777202661284,5.80359163943039,133.009736301615));
#213014=CARTESIAN_POINT('Ctrl Pts',(176.498755037472,4.99242806419446,127.113694031581));
#213015=CARTESIAN_POINT('Ctrl Pts',(176.220307413658,-0.406533008366379,
124.60919405498));
#213016=CARTESIAN_POINT('Ctrl Pts',(175.941859789846,-5.43191010648008,
127.797749498684));
#213017=CARTESIAN_POINT('Ctrl Pts',(175.663412166033,-5.46562718029972,
133.749233679521));
#213018=CARTESIAN_POINT('Ctrl Pts',(175.38496454222,-0.476699886155768,
136.994523381468));
#213019=CARTESIAN_POINT('Ctrl Pts',(175.106516918407,4.95029131528126,134.551355909651));
#213020=CARTESIAN_POINT('Ctrl Pts',(174.828069294595,5.82820663315002,128.664882815304));
#213021=CARTESIAN_POINT('Ctrl Pts',(174.549621670781,1.35028477887665,124.744485301934));
#213022=CARTESIAN_POINT('Ctrl Pts',(174.271174046969,-4.36848282210566,
126.392817162263));
#213023=CARTESIAN_POINT('Ctrl Pts',(173.992726423155,-6.07282812182305,
132.095141942134));
#213024=CARTESIAN_POINT('Ctrl Pts',(173.714278799343,-2.19654105173196,
136.611301742902));
#213025=CARTESIAN_POINT('Ctrl Pts',(173.435831175529,3.69825993790488,135.791166334329));
#213026=CARTESIAN_POINT('Ctrl Pts',(173.157383551717,6.19454071464915,130.388400091055));
#213027=CARTESIAN_POINT('Ctrl Pts',(172.878935927904,2.99834119476844,125.367881250842));
#213028=CARTESIAN_POINT('Ctrl Pts',(172.600488304091,-2.95318740599396,
125.343221361866));
#213029=CARTESIAN_POINT('Ctrl Pts',(172.322040680278,-6.1908810518732,130.337081657394));
#213030=CARTESIAN_POINT('Ctrl Pts',(172.043593056465,-3.7394574524341,135.760348489473));
#213031=CARTESIAN_POINT('Ctrl Pts',(171.765145432652,2.14834486313941,136.629304580736));
#213032=CARTESIAN_POINT('Ctrl Pts',(171.486697808839,6.06192320196904,132.145421734178));
#213033=CARTESIAN_POINT('Ctrl Pts',(171.208250185027,4.40489025960108,126.42916923593));
#213034=CARTESIAN_POINT('Ctrl Pts',(170.929802561213,-1.30002164048796,
124.733503877423));
#213035=CARTESIAN_POINT('Ctrl Pts',(170.651354937401,-5.81027716255637,
128.616659285268));
#213036=CARTESIAN_POINT('Ctrl Pts',(170.372907313588,-4.98117182005496,
134.510205342342));
#213037=CARTESIAN_POINT('Ctrl Pts',(170.094459689775,0.42538708130529,136.998261137926));
#213038=CARTESIAN_POINT('Ctrl Pts',(169.816012065962,5.44103603626017,133.794424944161));
#213039=CARTESIAN_POINT('Ctrl Pts',(169.537564442149,5.45663868327959,127.842865707018));
#213040=CARTESIAN_POINT('Ctrl Pts',(169.259116818336,0.457856951984399,
124.612775615598));
#213041=CARTESIAN_POINT('Ctrl Pts',(168.980669194523,-4.9616729506289,127.072449665244));
#213042=CARTESIAN_POINT('Ctrl Pts',(168.702221570711,-5.82166780281318,
132.961567566087));
#213043=CARTESIAN_POINT('Ctrl Pts',(168.423773946897,-1.33183434849535,
136.868317666657));
#213044=CARTESIAN_POINT('Ctrl Pts',(168.145326323085,4.38188980836473,135.202587479883));
#213045=CARTESIAN_POINT('Ctrl Pts',(167.866878699272,6.06887129855542,129.495101671966));
#213046=CARTESIAN_POINT('Ctrl Pts',(167.588431075459,2.17885654621902,124.9907608742));
#213047=CARTESIAN_POINT('Ctrl Pts',(167.309983451646,-3.71342092903282,
125.82883423045));
#213048=CARTESIAN_POINT('Ctrl Pts',(167.031535827833,-6.19324598120115,
131.239173268482));
#213049=CARTESIAN_POINT('Ctrl Pts',(166.75308820402,-2.98178053353198,136.249940722101));
#213050=CARTESIAN_POINT('Ctrl Pts',(166.474640580207,2.96979555637586,136.25648609103));
#213051=CARTESIAN_POINT('Ctrl Pts',(166.196192956395,6.19227461255283,131.252794500981));
#213052=CARTESIAN_POINT('Ctrl Pts',(165.917745332582,3.7243558092261,125.837014079288));
#213053=CARTESIAN_POINT('Ctrl Pts',(165.639297708769,-2.16606403788322,
124.985982457902));
#213054=CARTESIAN_POINT('Ctrl Pts',(165.360850084956,-6.06597685228888,
129.481756121673));
#213055=CARTESIAN_POINT('Ctrl Pts',(165.082402461143,-4.39155327888481,
135.192938704347));
#213056=CARTESIAN_POINT('Ctrl Pts',(164.80395483733,1.31849321850979,136.871232419228));
#213057=CARTESIAN_POINT('Ctrl Pts',(164.525507213517,5.81690886006848,132.974367331546));
#213058=CARTESIAN_POINT('Ctrl Pts',(164.247059589704,4.96986943102014,127.083372084437));
#213059=CARTESIAN_POINT('Ctrl Pts',(163.968611965891,-0.444237213516358,
124.611783518878));
#213060=CARTESIAN_POINT('Ctrl Pts',(163.690164342078,-5.45011156102575,
127.830870782803));
#213061=CARTESIAN_POINT('Ctrl Pts',(163.411716718265,-5.44759963670407,
133.782449941821));
#213062=CARTESIAN_POINT('Ctrl Pts',(163.133269094453,-0.439009776288703,
136.9973104996));
#213063=CARTESIAN_POINT('Ctrl Pts',(162.85482147064,4.97300862171615,134.52115265821));
#213064=CARTESIAN_POINT('Ctrl Pts',(162.576373846827,5.81507504134112,128.629444506854));
#213065=CARTESIAN_POINT('Ctrl Pts',(162.297926223014,1.31337158018249,124.736378010682));
#213066=CARTESIAN_POINT('Ctrl Pts',(162.019478599201,-4.39525620139515,
126.419491092807));
#213067=CARTESIAN_POINT('Ctrl Pts',(161.741030975388,-6.06485825409316,
132.132085055398));
#213068=CARTESIAN_POINT('Ctrl Pts',(161.462583351575,-2.16115185607673,
136.624565122567));
#213069=CARTESIAN_POINT('Ctrl Pts',(161.184135727762,3.72854751953661,135.768561582436));
#213070=CARTESIAN_POINT('Ctrl Pts',(160.905688103949,6.19189387436843,130.350699870288));
#213071=CARTESIAN_POINT('Ctrl Pts',(160.627240480137,2.96519224948793,125.349730222329));
#213072=CARTESIAN_POINT('Ctrl Pts',(160.348792856324,-2.9863761949775,125.361299434083));
#213073=CARTESIAN_POINT('Ctrl Pts',(160.070345232511,-6.19361080884636,
130.374775965136));
#213074=CARTESIAN_POINT('Ctrl Pts',(159.791897608698,-3.70921966409463,
135.783019805394));
#213075=CARTESIAN_POINT('Ctrl Pts',(159.513449984885,2.18376314650564,136.616119073061));
#213076=CARTESIAN_POINT('Ctrl Pts',(159.235002361072,6.06997430822783,132.108496240312));
#213077=CARTESIAN_POINT('Ctrl Pts',(158.956554737259,4.37817561541891,126.402436480826));
#213078=CARTESIAN_POINT('Ctrl Pts',(158.678107113446,-1.3369525821905,124.741529957054));
#213079=CARTESIAN_POINT('Ctrl Pts',(158.399659489633,-5.82348667053154,
128.652068624549));
#213080=CARTESIAN_POINT('Ctrl Pts',(158.121211865821,-4.95852100179383,
134.540458488317));
#213081=CARTESIAN_POINT('Ctrl Pts',(157.842764242008,0.463083230374652,
136.995556927392));
#213082=CARTESIAN_POINT('Ctrl Pts',(157.564316618195,5.45913659670229,133.761248414491));
#213083=CARTESIAN_POINT('Ctrl Pts',(157.285868994382,5.43851012430973,127.809704468215));
#213084=CARTESIAN_POINT('Ctrl Pts',(157.007421370569,0.420158533666468,
124.610103226106));
#213085=CARTESIAN_POINT('Ctrl Pts',(156.728973746756,-4.98429822353081,
127.102721920452));
#213086=CARTESIAN_POINT('Ctrl Pts',(156.450526122943,-5.80842840980828,
132.996965742341));
#213087=CARTESIAN_POINT('Ctrl Pts',(156.172078499131,-1.2948966449748,136.876312569277));
#213088=CARTESIAN_POINT('Ctrl Pts',(155.893630875317,4.40858187737264,135.175832183934));
#213089=CARTESIAN_POINT('Ctrl Pts',(155.615183251505,6.06078902561252,129.458182987356));
#213090=CARTESIAN_POINT('Ctrl Pts',(155.336735627692,2.14342714531882,124.977605268507));
#213091=CARTESIAN_POINT('Ctrl Pts',(155.058288003879,-3.74363956928552,
125.85153106262));
#213092=CARTESIAN_POINT('Ctrl Pts',(154.779840380066,-6.19048440667673,
131.276865258552));
#213093=CARTESIAN_POINT('Ctrl Pts',(154.501392756253,-2.94857649630798,
136.267990772552));
#213094=CARTESIAN_POINT('Ctrl Pts',(154.22294513244,3.00292916819795,136.238307087292));
#213095=CARTESIAN_POINT('Ctrl Pts',(153.944497508627,6.19488962837548,131.215092059396));
#213096=CARTESIAN_POINT('Ctrl Pts',(153.666049884815,3.69404915725887,125.814434901805));
#213097=CARTESIAN_POINT('Ctrl Pts',(153.387602261001,-2.20144202504465,
124.999275705575));
#213098=CARTESIAN_POINT('Ctrl Pts',(153.109154637189,-6.07391553275397,
129.518705949301));
#213099=CARTESIAN_POINT('Ctrl Pts',(152.830707013376,-4.36475739313218,
135.219590025439));
#213100=CARTESIAN_POINT('Ctrl Pts',(152.552259389563,1.3553995605252,136.863093971691));
#213101=CARTESIAN_POINT('Ctrl Pts',(152.27381176575,5.83001053300956,132.93891795108));
#213102=CARTESIAN_POINT('Ctrl Pts',(151.995364141937,4.94712663750637,127.053188019893));
#213103=CARTESIAN_POINT('Ctrl Pts',(151.716916518124,-0.481924957293099,
124.614602450997));
#213104=CARTESIAN_POINT('Ctrl Pts',(151.438468894311,-5.46811105968323,
127.864102250682));
#213105=CARTESIAN_POINT('Ctrl Pts',(151.160021270498,-5.4293702303005,133.815555849925));
#213106=CARTESIAN_POINT('Ctrl Pts',(150.881573646685,-0.40130339875292,
136.999868135696));
#213107=CARTESIAN_POINT('Ctrl Pts',(150.603126022873,4.99554165148768,134.490811679673));
#213108=CARTESIAN_POINT('Ctrl Pts',(150.324678399059,5.80172796978809,128.59408679072));
#213109=CARTESIAN_POINT('Ctrl Pts',(150.046230775247,1.27640971402146,124.728495570759));
#213110=CARTESIAN_POINT('Ctrl Pts',(149.767783151434,-4.42186671284978,
126.446327506304));
#213111=CARTESIAN_POINT('Ctrl Pts',(149.489335527621,-6.05666365081033,
132.168978969345));
#213112=CARTESIAN_POINT('Ctrl Pts',(149.210887903808,-2.12568257814469,
136.637612832414));
#213113=CARTESIAN_POINT('Ctrl Pts',(148.932440279995,3.75869693846883,135.74577288025));
#213114=CARTESIAN_POINT('Ctrl Pts',(148.653992656183,6.18901759118317,130.313016460088));
#213115=CARTESIAN_POINT('Ctrl Pts',(148.375545032369,2.93193342791814,125.331781317152));
#213116=CARTESIAN_POINT('Ctrl Pts',(148.097097408557,-3.01945432269288,
125.379579200934));
#213117=CARTESIAN_POINT('Ctrl Pts',(147.818649784743,-6.19611105929333,
130.412486191295));
#213118=CARTESIAN_POINT('Ctrl Pts',(147.540202160931,-3.67884442925635,
135.805506635269));
#213119=CARTESIAN_POINT('Ctrl Pts',(147.261754537118,2.21910050972548,136.602718208539));
#213120=CARTESIAN_POINT('Ctrl Pts',(146.983306913305,6.07780048935632,132.071522421221));
#213121=CARTESIAN_POINT('Ctrl Pts',(146.704859289492,4.35129873632927,126.375866840638));
#213122=CARTESIAN_POINT('Ctrl Pts',(146.426411665679,-1.37383398262348,
124.749780697104));
#213123=CARTESIAN_POINT('Ctrl Pts',(146.147964041867,-5.83648038706648,
128.687557717801));
#213124=CARTESIAN_POINT('Ctrl Pts',(145.869516418053,-4.93568644371351,
134.570573191811));
#213125=CARTESIAN_POINT('Ctrl Pts',(145.591068794241,0.500762219724632,
136.992623299802));
#213126=CARTESIAN_POINT('Ctrl Pts',(145.312621170428,5.47703486683029,133.727962316256));
#213127=CARTESIAN_POINT('Ctrl Pts',(145.034173546615,5.42018003934715,127.776654197497));
#213128=CARTESIAN_POINT('Ctrl Pts',(144.755725922802,0.382444546219556,
124.607660367099));
#213129=CARTESIAN_POINT('Ctrl Pts',(144.477278298989,-5.00673880142907,
127.133131341243));
#213130=CARTESIAN_POINT('Ctrl Pts',(144.198830675176,-5.79497378335261,
133.032282670807));
#213131=CARTESIAN_POINT('Ctrl Pts',(143.920383051363,-1.25791095858285,
136.884082473484));
#213132=CARTESIAN_POINT('Ctrl Pts',(143.64193542755,4.43511058475782,135.148914901497));
#213133=CARTESIAN_POINT('Ctrl Pts',(143.363487803737,6.05248216790344,129.421314185853));
#213134=CARTESIAN_POINT('Ctrl Pts',(143.085040179924,2.10791831893749,124.964665575378));
#213135=CARTESIAN_POINT('Ctrl Pts',(142.806592556112,-3.77371948759721,
125.87441142371));
#213136=CARTESIAN_POINT('Ctrl Pts',(142.528144932299,-6.18749344147606,
131.314539739788));
#213137=CARTESIAN_POINT('Ctrl Pts',(142.249697308486,-2.91526319849757,
136.285838366179));
#213138=CARTESIAN_POINT('Ctrl Pts',(141.971249684673,3.03595150537554,136.219926726669));
#213139=CARTESIAN_POINT('Ctrl Pts',(141.69280206086,6.19727509028471,131.177374398005));
#213140=CARTESIAN_POINT('Ctrl Pts',(141.414354437047,3.6636056209416,125.792040627854));
#213141=CARTESIAN_POINT('Ctrl Pts',(141.135906813234,-2.23673843696229,
125.012784062803));
#213142=CARTESIAN_POINT('Ctrl Pts',(140.857459189421,-6.0816291420453,129.555703417335));
#213143=CARTESIAN_POINT('Ctrl Pts',(140.579011565609,-4.33779976968917,
135.246077738584));
#213144=CARTESIAN_POINT('Ctrl Pts',(140.300563941795,1.39225567771152,136.854731015561));
#213145=CARTESIAN_POINT('Ctrl Pts',(140.022116317983,5.84289617276637,132.903389473806));
#213146=CARTESIAN_POINT('Ctrl Pts',(139.74366869417,4.92420052639575,127.023142956427));
#213147=CARTESIAN_POINT('Ctrl Pts',(139.465221070357,-0.519594843163371,
124.617650746882));
#213148=CARTESIAN_POINT('Ctrl Pts',(139.186773446544,-5.48590793547459,
127.897442670915));
#213149=CARTESIAN_POINT('Ctrl Pts',(138.908325822731,-5.41093963658633,
133.848550177083));
#213150=CARTESIAN_POINT('Ctrl Pts',(138.629878198918,-0.363582150772119,
137.002196194983));
#213151=CARTESIAN_POINT('Ctrl Pts',(138.351430575105,5.0178895696262,134.460334098336));
#213152=CARTESIAN_POINT('Ctrl Pts',(138.072982951292,5.78816591307159,128.558810977095));
#213153=CARTESIAN_POINT('Ctrl Pts',(137.79453532748,1.23940055002892,124.720838274248));
#213154=CARTESIAN_POINT('Ctrl Pts',(137.516087703667,-4.44831337040726,
126.473325408321));
#213155=CARTESIAN_POINT('Ctrl Pts',(137.237640079854,-6.0482446156285,132.205822316857));
#213156=CARTESIAN_POINT('Ctrl Pts',(136.959192456041,-2.09013453226308,
136.650444388955));
#213157=CARTESIAN_POINT('Ctrl Pts',(136.680744832228,3.78870707750376,135.722801072215));
#213158=CARTESIAN_POINT('Ctrl Pts',(136.402297208415,6.18591197167502,130.275351256826));
#213159=CARTESIAN_POINT('Ctrl Pts',(136.123849584602,2.89856596247695,125.314035200413));
#213160=CARTESIAN_POINT('Ctrl Pts',(135.845401960789,-3.05242056341787,
125.398059985055));
#213161=CARTESIAN_POINT('Ctrl Pts',(135.566954336976,-6.19838171056633,
130.450210938505));
#213162=CARTESIAN_POINT('Ctrl Pts',(135.288506713164,-3.64833287348497,
135.827808145838));
#213163=CARTESIAN_POINT('Ctrl Pts',(135.01005908935,2.25435564335981,136.589102483743));
#213164=CARTESIAN_POINT('Ctrl Pts',(134.731611465538,6.08540145535266,132.034501646982));
#213165=CARTESIAN_POINT('Ctrl Pts',(134.453163841725,4.32426061826468,126.349461299917));
#213166=CARTESIAN_POINT('Ctrl Pts',(134.174716217912,-1.41066447513297,
124.75825579184));
#213167=CARTESIAN_POINT('Ctrl Pts',(133.896268594099,-5.84925783067434,
128.723125249964));
#213168=CARTESIAN_POINT('Ctrl Pts',(133.617820970286,-4.91266899195694,
134.600548336913));
#213169=CARTESIAN_POINT('Ctrl Pts',(133.339373346473,0.538422653146471,
136.989460363863));
#213170=CARTESIAN_POINT('Ctrl Pts',(133.06092572266,5.49473018341705,133.694567882885));
#213171=CARTESIAN_POINT('Ctrl Pts',(132.782478098847,5.40164910761999,127.743716119554));
#213172=CARTESIAN_POINT('Ctrl Pts',(132.504030475035,0.344716387149417,
124.605447129098));
#213173=CARTESIAN_POINT('Ctrl Pts',(132.225582851222,-5.02899385277987,
127.163676800786));
#213174=CARTESIAN_POINT('Ctrl Pts',(131.947135227409,-5.78130442201224,
133.067517042801));
#213175=CARTESIAN_POINT('Ctrl Pts',(131.668687603596,-1.22087865983776,
136.891627091362));
#213176=CARTESIAN_POINT('Ctrl Pts',(131.390239979783,4.46147494748924,135.121836630005));
#213177=CARTESIAN_POINT('Ctrl Pts',(131.11179235597,6.04395103324181,129.384496633644));
#213178=CARTESIAN_POINT('Ctrl Pts',(130.833344732157,2.07233138286776,124.951942274296));
#213179=CARTESIAN_POINT('Ctrl Pts',(130.554897108344,-3.80365956934553,
125.897474465882));
#213180=CARTESIAN_POINT('Ctrl Pts',(130.276449484532,-6.18427319643048,
131.35219531615));
#213181=CARTESIAN_POINT('Ctrl Pts',(129.998001860718,-2.88184187453723,
136.303482841632));
#213182=CARTESIAN_POINT('Ctrl Pts',(129.719554236906,3.0688613442533,136.201345690253));
#213183=CARTESIAN_POINT('Ctrl Pts',(129.441106613093,6.1994309098865,131.139642914452));
#213184=CARTESIAN_POINT('Ctrl Pts',(129.16265898928,3.63302632837089,125.769832087263));
#213185=CARTESIAN_POINT('Ctrl Pts',(128.884211365467,-2.27195196571463,
125.026507029031));
#213186=CARTESIAN_POINT('Ctrl Pts',(128.605763741654,-6.08911739433215,
129.592747154821));
#213187=CARTESIAN_POINT('Ctrl Pts',(128.327316117841,-4.31068140748063,
135.272400862266));
#213188=CARTESIAN_POINT('Ctrl Pts',(128.048868494028,1.42906020435147,136.846143860731));
#213189=CARTESIAN_POINT('Ctrl Pts',(127.770420870216,5.85556530185681,132.867783216248));
#213190=CARTESIAN_POINT('Ctrl Pts',(127.491973246402,4.9010919472237,126.993238007373));
#213191=CARTESIAN_POINT('Ctrl Pts',(127.21352562259,-0.557245475255655,
124.620928293575));
#213192=CARTESIAN_POINT('Ctrl Pts',(126.935077998777,-5.50350152892981,
127.930890808061));
#213193=CARTESIAN_POINT('Ctrl Pts',(126.656630374964,-5.39230853851415,
133.881431700678));
#213194=CARTESIAN_POINT('Ctrl Pts',(126.378182751151,-0.325847430121078,
137.004294591193));
#213195=CARTESIAN_POINT('Ctrl Pts',(126.099735127338,5.04005154802147,134.429721043558));
#213196=CARTESIAN_POINT('Ctrl Pts',(125.821287503525,5.77438937373851,128.523618373138));
#213197=CARTESIAN_POINT('Ctrl Pts',(125.542839879712,1.20234545959337,124.713406404895));
#213198=CARTESIAN_POINT('Ctrl Pts',(125.264392255899,-4.47459519407686,
126.50048379844));
#213199=CARTESIAN_POINT('Ctrl Pts',(124.985944632086,-6.03960146051831,
132.24261373269));
#213200=CARTESIAN_POINT('Ctrl Pts',(124.707497008274,-2.05450903567761,
136.663059316712));
#213201=CARTESIAN_POINT('Ctrl Pts',(124.429049384461,3.81857682460466,135.69964700956));
#213202=CARTESIAN_POINT('Ctrl Pts',(124.150601760648,6.18257713092382,130.237705656202));
#213203=CARTESIAN_POINT('Ctrl Pts',(123.872154136835,2.86509108960817,125.296492529702));
#213204=CARTESIAN_POINT('Ctrl Pts',(123.593706513022,-3.08527369557641,
125.416741101634));
#213205=CARTESIAN_POINT('Ctrl Pts',(123.315258889209,-6.20042267852561,
130.487948808862));
#213206=CARTESIAN_POINT('Ctrl Pts',(123.036811265396,-3.61768612739718,
135.849923510712));
#213207=CARTESIAN_POINT('Ctrl Pts',(122.758363641583,2.28952724101679,136.575272403211));
#213208=CARTESIAN_POINT('Ctrl Pts',(122.47991601777,6.09277692456002,131.997435289415));
#213209=CARTESIAN_POINT('Ctrl Pts',(122.201468393958,4.29706226313277,126.323220837128));
#213210=CARTESIAN_POINT('Ctrl Pts',(121.923020770144,-1.44744269495155,
124.766954927214));
#213211=CARTESIAN_POINT('Ctrl Pts',(121.644573146332,-5.86181852788225,
128.758769903068));
#213212=CARTESIAN_POINT('Ctrl Pts',(121.366125522519,-4.88946949944416,
134.630382812884));
#213213=CARTESIAN_POINT('Ctrl Pts',(121.087677898706,0.576063135118759,
136.986068236777));
#213214=CARTESIAN_POINT('Ctrl Pts',(120.809230274893,5.51222189075617,133.661066351821));
#213215=CARTESIAN_POINT('Ctrl Pts',(120.53078265108,5.38291801579874,127.710891454918));
#213216=CARTESIAN_POINT('Ctrl Pts',(120.252335027267,0.306975454486648,
124.603463594118));
#213217=CARTESIAN_POINT('Ctrl Pts',(119.973887403454,-5.05106255291402,
127.194357167205));
#213218=CARTESIAN_POINT('Ctrl Pts',(119.695439779642,-5.76742083231046,
133.102667552701));
#213219=CARTESIAN_POINT('Ctrl Pts',(119.416992155829,-1.18380112098488,
136.898946143343));
#213220=CARTESIAN_POINT('Ctrl Pts',(119.138544532016,4.48767398862585,135.09459837285));
#213221=CARTESIAN_POINT('Ctrl Pts',(118.860096908203,6.03519593775195,129.347731695017));
#213222=CARTESIAN_POINT('Ctrl Pts',(118.58164928439,2.0366676557964,124.939435836727));
#213223=CARTESIAN_POINT('Ctrl Pts',(118.303201660577,-3.83345870508974,
125.920719334523));
#213224=CARTESIAN_POINT('Ctrl Pts',(118.024754036764,-6.18082379086727,
131.389830592295));
#213225=CARTESIAN_POINT('Ctrl Pts',(117.746306412951,-2.84831376286653,
136.320923545089));
#213226=CARTESIAN_POINT('Ctrl Pts',(117.467858789138,3.10165746534553,136.18256466657));
#213227=CARTESIAN_POINT('Ctrl Pts',(117.189411165326,6.20135700729606,131.101899006891));
#213228=CARTESIAN_POINT('Ctrl Pts',(116.910963541513,3.60231241267338,125.747810102979));
#213229=CARTESIAN_POINT('Ctrl Pts',(116.6325159177,-2.30708130645123,125.040444095748));
#213230=CARTESIAN_POINT('Ctrl Pts',(116.354068293887,-6.09638001213474,
129.62983578909));
#213231=CARTESIAN_POINT('Ctrl Pts',(116.075620670074,-4.28340331138726,
135.298558421074));
#213232=CARTESIAN_POINT('Ctrl Pts',(115.797173046261,1.46581177664024,136.837332825402));
#213233=CARTESIAN_POINT('Ctrl Pts',(115.518725422448,5.86801745082159,132.832100497806));
#213234=CARTESIAN_POINT('Ctrl Pts',(115.240277798635,4.87780175628715,126.963474280869));
#213235=CARTESIAN_POINT('Ctrl Pts',(114.961830174822,-0.594875458411799,
124.624434969628));
#213236=CARTESIAN_POINT('Ctrl Pts',(114.68338255101,-5.52089118811201,127.964445422689));
#213237=CARTESIAN_POINT('Ctrl Pts',(114.404934927196,-5.37347762646609,
133.914199202272));
#213238=CARTESIAN_POINT('Ctrl Pts',(114.126487303384,-0.288100635073559,
137.006163246571));
#213239=CARTESIAN_POINT('Ctrl Pts',(113.848039679571,5.06202676545313,134.398973649715));
#213240=CARTESIAN_POINT('Ctrl Pts',(113.569592055758,5.76039886228364,128.488510282924));
#213241=CARTESIAN_POINT('Ctrl Pts',(113.291144431945,1.16524581580469,124.706200238089));
#213242=CARTESIAN_POINT('Ctrl Pts',(113.012696808132,-4.50071120997606,
126.527801670297));
#213243=CARTESIAN_POINT('Ctrl Pts',(112.734249184319,-6.03073450575487,
132.279351853526));
#213244=CARTESIAN_POINT('Ctrl Pts',(112.455801560506,-2.01880740850426,
136.675457148234));
#213245=CARTESIAN_POINT('Ctrl Pts',(112.177353936694,3.84830507293705,135.676311550269));
#213246=CARTESIAN_POINT('Ctrl Pts',(111.898906312881,6.17901319250346,130.200081053184));
#213247=CARTESIAN_POINT('Ctrl Pts',(111.620458689068,2.8315100497353,125.279153955068));
#213248=CARTESIAN_POINT('Ctrl Pts',(111.342011065255,-3.11801250178361,
125.435621858436));
#213249=CARTESIAN_POINT('Ctrl Pts',(111.063563441442,-6.20223388754234,
130.525698403974));
#213250=CARTESIAN_POINT('Ctrl Pts',(110.785115817629,-3.58690532661952,
135.871851910398));
#213251=CARTESIAN_POINT('Ctrl Pts',(110.506668193816,2.32461399939974,136.56122847942));
#213252=CARTESIAN_POINT('Ctrl Pts',(110.228220570003,6.09992662367788,131.960324722029));
#213253=CARTESIAN_POINT('Ctrl Pts',(109.94977294619,4.26970467877848,126.297146424621));
#213254=CARTESIAN_POINT('Ctrl Pts',(109.671325322378,-1.48416727924886,
124.775877780875));
#213255=CARTESIAN_POINT('Ctrl Pts',(109.392877698565,-5.8741620132489,128.794490356288));
#213256=CARTESIAN_POINT('Ctrl Pts',(109.114430074752,-4.86608882584101,
134.660075514194));
#213257=CARTESIAN_POINT('Ctrl Pts',(108.835982450939,0.61368227085971,136.982447044243));
#213258=CARTESIAN_POINT('Ctrl Pts',(108.557534827126,5.52950934068608,133.627458964475));
#213259=CARTESIAN_POINT('Ctrl Pts',(108.279087203313,5.36398745797076,127.67818141992));
#213260=CARTESIAN_POINT('Ctrl Pts',(108.0006395795,0.269223146735527,124.601709835656));
#213261=CARTESIAN_POINT('Ctrl Pts',(107.722191955687,-5.07294408406776,
127.225171303631));
#213262=CARTESIAN_POINT('Ctrl Pts',(107.443744331874,-5.75332352870873,
133.137732897993));
#213263=CARTESIAN_POINT('Ctrl Pts',(107.165296708062,-1.14667971594628,
136.906039358215));
#213264=CARTESIAN_POINT('Ctrl Pts',(106.886849084249,4.51370673735246,135.067201139359));
#213265=CARTESIAN_POINT('Ctrl Pts',(106.608401460436,6.02621720585718,129.31102073231));
#213266=CARTESIAN_POINT('Ctrl Pts',(106.329953836623,2.00092845925606,124.927146726103));
#213267=CARTESIAN_POINT('Ctrl Pts',(106.05150621281,-3.86311579061174,125.944145168289));
#213268=CARTESIAN_POINT('Ctrl Pts',(105.773058588997,-6.17714535260555,
131.427444173636));
#213269=CARTESIAN_POINT('Ctrl Pts',(105.494610965184,-2.81468010588189,
136.338159830278));
#213270=CARTESIAN_POINT('Ctrl Pts',(105.216163341371,3.13433865337982,136.163584351558));
#213271=CARTESIAN_POINT('Ctrl Pts',(104.937715717558,6.20305331114115,131.064144073934));
#213272=CARTESIAN_POINT('Ctrl Pts',(104.659268093745,3.57146501196475,125.725975491034));
#213273=CARTESIAN_POINT('Ctrl Pts',(104.380820469933,-2.34212515744159,
125.054594746511));
#213274=CARTESIAN_POINT('Ctrl Pts',(104.10237284612,-6.10341672633411,129.666967945808));
#213275=CARTESIAN_POINT('Ctrl Pts',(103.823925222307,-4.25596649220884,
135.324549445729));
#213276=CARTESIAN_POINT('Ctrl Pts',(103.545477598494,1.50250903273456,136.828298236068));
#213277=CARTESIAN_POINT('Ctrl Pts',(103.267029974681,5.88025215824177,132.796342640716));
#213278=CARTESIAN_POINT('Ctrl Pts',(102.988582350868,4.85433081661274,126.933852879821));
#213279=CARTESIAN_POINT('Ctrl Pts',(102.710134727055,-0.63248339823904,
124.628170645098));
#213280=CARTESIAN_POINT('Ctrl Pts',(102.431687103242,-5.53807626864099,
127.998105271418));
#213281=CARTESIAN_POINT('Ctrl Pts',(102.153239479429,-5.35444759822839,
133.946851467654));
#213282=CARTESIAN_POINT('Ctrl Pts',(101.874791855617,-0.250343164351048,
137.00780209187));
#213283=CARTESIAN_POINT('Ctrl Pts',(101.596344231803,5.0838144076213,134.368093056165));
#213284=CARTESIAN_POINT('Ctrl Pts',(101.317896607991,5.74619489713063,128.453488007394));
#213285=CARTESIAN_POINT('Ctrl Pts',(101.039448984178,1.12810299340375,124.69922004086));
#213286=CARTESIAN_POINT('Ctrl Pts',(100.761001360365,-4.52666045036627,
126.55527801162));
#213287=CARTESIAN_POINT('Ctrl Pts',(100.482553736552,-6.0216440799065,132.316035318018));
#213288=CARTESIAN_POINT('Ctrl Pts',(100.204106112739,-1.98303097367997,
136.687637424115));
#213289=CARTESIAN_POINT('Ctrl Pts',(99.9256584889259,3.87789072090961,135.652795559044));
#213290=CARTESIAN_POINT('Ctrl Pts',(99.6472108651132,6.17522028847693,130.162478841968));
#213291=CARTESIAN_POINT('Ctrl Pts',(99.3687632413001,2.79782408721636,125.262020118999));
#213292=CARTESIAN_POINT('Ctrl Pts',(99.0903156174874,-3.15063576889091,
125.454701555827));
#213293=CARTESIAN_POINT('Ctrl Pts',(98.8118679936743,-6.20381527050148,
130.563458325018));
#213294=CARTESIAN_POINT('Ctrl Pts',(98.5334203698616,-3.55599161174595,
135.89359253233));
#213295=CARTESIAN_POINT('Ctrl Pts',(98.2549727460486,2.35961461835606,136.546971232774));
#213296=CARTESIAN_POINT('Ctrl Pts',(97.9765251222358,6.10685028777152,131.923171319966));
#213297=CARTESIAN_POINT('Ctrl Pts',(97.6980774984228,4.24218887894701,126.271239028595));
#213298=CARTESIAN_POINT('Ctrl Pts',(97.4196298746099,-1.52083686718185,
124.785024022185));
#213299=CARTESIAN_POINT('Ctrl Pts',(97.141182250797,-5.88628782938184,128.830285285991));
#213300=CARTESIAN_POINT('Ctrl Pts',(96.8627346269842,-4.842527837527,134.689625340572));
#213301=CARTESIAN_POINT('Ctrl Pts',(96.5842870031713,0.651278666378471,
136.978596920444));
#213302=CARTESIAN_POINT('Ctrl Pts',(96.3058393793584,5.54659189261388,133.593746966183));
#213303=CARTESIAN_POINT('Ctrl Pts',(96.0273917555454,5.34485813561491,127.645587226641));
#213304=CARTESIAN_POINT('Ctrl Pts',(95.7489441317327,0.231460862821695,
124.6001859187));
#213305=CARTESIAN_POINT('Ctrl Pts',(95.4704965079195,-5.09463763541278,
127.256118068232));
#213306=CARTESIAN_POINT('Ctrl Pts',(95.192048884107,-5.73901303358793,133.172711779316));
#213307=CARTESIAN_POINT('Ctrl Pts',(94.9136012602939,-1.10951582026908,
136.912906473138));
#213308=CARTESIAN_POINT('Ctrl Pts',(94.635153636481,4.53957222901603,135.039645944743));
#213309=CARTESIAN_POINT('Ctrl Pts',(94.3567060126683,6.01701517026768,129.274365105863));
#213310=CARTESIAN_POINT('Ctrl Pts',(94.0782583888551,1.96511511757592,124.915075397801));
#213311=CARTESIAN_POINT('Ctrl Pts',(93.7998107650425,-3.89262972695748,
125.967751099126));
#213312=CARTESIAN_POINT('Ctrl Pts',(93.5213631412293,-6.17323801795121,
131.465034666385));
#213313=CARTESIAN_POINT('Ctrl Pts',(93.2429155174167,-2.7809421498907,136.355191058501));
#213314=CARTESIAN_POINT('Ctrl Pts',(92.9644678936037,3.16690369734264,136.14440544854));
#213315=CARTESIAN_POINT('Ctrl Pts',(92.6860202697908,6.20451975856463,131.026379514606));
#213316=CARTESIAN_POINT('Ctrl Pts',(92.4075726459779,3.54048526930663,125.704329060518));
#213317=CARTESIAN_POINT('Ctrl Pts',(92.129125022165,-2.37708222012305,125.068958456964));
#213318=CARTESIAN_POINT('Ctrl Pts',(91.850677398352,-6.1102272761821,129.70414224903));
#213319=CARTESIAN_POINT('Ctrl Pts',(91.5722297745392,-4.22837196662692,
135.350372973126));
#213320=CARTESIAN_POINT('Ctrl Pts',(91.2937821507264,1.53915061280415,136.819040427511));
#213321=CARTESIAN_POINT('Ctrl Pts',(91.0153345269133,5.89226897075567,132.76051097));
#213322=CARTESIAN_POINT('Ctrl Pts',(90.7368869031008,4.8306799979248,126.90437490186));
#213323=CARTESIAN_POINT('Ctrl Pts',(90.4584392792875,-0.670067901161403,
124.632135181558));
#213324=CARTESIAN_POINT('Ctrl Pts',(90.1799916554748,-5.5550561337172,128.031869106972));
#213325=CARTESIAN_POINT('Ctrl Pts',(89.9015440316619,-5.3352191589658,133.979387286881));
#213326=CARTESIAN_POINT('Ctrl Pts',(89.6230964078489,-0.212576417070642,
137.009211066365));
#213327=CARTESIAN_POINT('Ctrl Pts',(89.3446487840362,5.10541366717708,134.337080407198));
#213328=CARTESIAN_POINT('Ctrl Pts',(89.0662011602232,5.73177800461257,128.418552844315));
#213329=CARTESIAN_POINT('Ctrl Pts',(88.7877535364103,1.09091836873142,124.69246607186));
#213330=CARTESIAN_POINT('Ctrl Pts',(88.5093059125973,-4.5524419536888,126.58291180426));
#213331=CARTESIAN_POINT('Ctrl Pts',(88.2308582887847,-6.0123305198223,132.352662766849));
#213332=CARTESIAN_POINT('Ctrl Pts',(87.9524106649715,-1.94718105691378,
136.69959969301));
#213333=CARTESIAN_POINT('Ctrl Pts',(87.6739630411587,3.90733267221543,135.629099907278));
#213334=CARTESIAN_POINT('Ctrl Pts',(87.395515417346,6.17119855939173,130.124900415918));
#213335=CARTESIAN_POINT('Ctrl Pts',(87.1170677935327,2.76403445029686,125.245091656395));
#213336=CARTESIAN_POINT('Ctrl Pts',(86.8386201697203,-3.18314228803115,
125.473979486801));
#213337=CARTESIAN_POINT('Ctrl Pts',(86.5601725459069,-6.20516676880425,
130.601227172784));
#213338=CARTESIAN_POINT('Ctrl Pts',(86.2817249220945,-3.52494612829556,
135.915144570902));
#213339=CARTESIAN_POINT('Ctrl Pts',(86.0032772982812,2.394527800925,136.532501191579));
#213340=CARTESIAN_POINT('Ctrl Pts',(85.7248296744686,6.11354766028192,131.885976459962));
#213341=CARTESIAN_POINT('Ctrl Pts',(85.4463820506556,4.21451588324655,126.245499609054));
#213342=CARTESIAN_POINT('Ctrl Pts',(85.1679344268427,-1.55745009994542,
124.794393312227));
#213343=CARTESIAN_POINT('Ctrl Pts',(84.8894868030298,-5.89819552695468,
128.86615336578));
#213344=CARTESIAN_POINT('Ctrl Pts',(84.611039179217,-4.81878740756302,134.719031197036));
#213345=CARTESIAN_POINT('Ctrl Pts',(84.332591555404,0.68885092852684,136.974518008049));
#213346=CARTESIAN_POINT('Ctrl Pts',(84.0541439315912,5.56346891353935,133.559931606153));
#213347=CARTESIAN_POINT('Ctrl Pts',(83.7756963077782,5.32553075757526,127.613110082872));
#213348=CARTESIAN_POINT('Ctrl Pts',(83.4972486839655,0.193690002040587,
124.598891899719));
#213349=CARTESIAN_POINT('Ctrl Pts',(83.2188010601524,-5.11614240308669,
127.287196314267));
#213350=CARTESIAN_POINT('Ctrl Pts',(82.9403534363397,-5.72448987722869,
133.207602900518));
#213351=CARTESIAN_POINT('Ctrl Pts',(82.6619058125266,-1.07231081107503,
136.919547233648));
#213352=CARTESIAN_POINT('Ctrl Pts',(82.3834581887138,4.56526950516122,135.011933810073));
#213353=CARTESIAN_POINT('Ctrl Pts',(82.1050105649009,6.00759017196827,129.237766173961));
#213354=CARTESIAN_POINT('Ctrl Pts',(81.826562941088,1.92922895783247,124.903222299129));
#213355=CARTESIAN_POINT('Ctrl Pts',(81.5481153172751,-3.92199942047723,
125.991536252305));
#213356=CARTESIAN_POINT('Ctrl Pts',(81.2696676934623,-6.16910193169181,
131.502600677615));
#213357=CARTESIAN_POINT('Ctrl Pts',(80.9912200696492,-2.74710114506546,
136.372016598662));
#213358=CARTESIAN_POINT('Ctrl Pts',(80.7127724458365,3.19935139052435,136.125028668197));
#213359=CARTESIAN_POINT('Ctrl Pts',(80.4343248220235,6.20575629522666,130.988606728286));
#213360=CARTESIAN_POINT('Ctrl Pts',(80.1558771982107,3.50937433266497,125.682871613546));
#213361=CARTESIAN_POINT('Ctrl Pts',(79.8774295743978,-2.41195119914859,
125.083534694853));
#213362=CARTESIAN_POINT('Ctrl Pts',(79.5989819505849,-6.11681140931136,
129.741357321249));
#213363=CARTESIAN_POINT('Ctrl Pts',(79.320534326772,-4.20062075716678,135.376028046362));
#213364=CARTESIAN_POINT('Ctrl Pts',(79.0420867029591,1.57573515908161,136.809559742781));
#213365=CARTESIAN_POINT('Ctrl Pts',(78.7636390791462,5.90406744307602,132.724606813414));
#213366=CARTESIAN_POINT('Ctrl Pts',(78.4851914553333,4.80685017661309,126.875041439303));
#213367=CARTESIAN_POINT('Ctrl Pts',(78.2067438315204,-0.707627574471386,
124.636328432103));
#213368=CARTESIAN_POINT('Ctrl Pts',(77.9282962077074,-5.57183015414549,
128.065735678218));
#213369=CARTESIAN_POINT('Ctrl Pts',(77.6498485838947,-5.31579302119528,
134.011805454327));
#213370=CARTESIAN_POINT('Ctrl Pts',(77.3714009600817,-0.174801792692954,
137.010390117845));
#213371=CARTESIAN_POINT('Ctrl Pts',(77.0929533362689,5.12682374375196,134.305936852001));
#213372=CARTESIAN_POINT('Ctrl Pts',(76.814505712456,5.7171487189526,128.38370608822));
#213373=CARTESIAN_POINT('Ctrl Pts',(76.536058088643,1.05369331967776,124.68593858136));
#213374=CARTESIAN_POINT('Ctrl Pts',(76.2576104648302,-4.57805476460059,
126.610702024239));
#213375=CARTESIAN_POINT('Ctrl Pts',(75.9791628410172,-6.00279417061961,
132.389232842773));
#213376=CARTESIAN_POINT('Ctrl Pts',(75.7007152172044,-1.91125898663751,
136.711343511654));
#213377=CARTESIAN_POINT('Ctrl Pts',(75.4222675933915,3.93662983587222,135.605225473025));
#213378=CARTESIAN_POINT('Ctrl Pts',(75.1438199695785,6.16694815427437,130.087347167514));
#213379=CARTESIAN_POINT('Ctrl Pts',(74.8653723457658,2.73014239106432,125.228369194547));
#213380=CARTESIAN_POINT('Ctrl Pts',(74.5869247219528,-3.21553085466319,
125.493454937009));
#213381=CARTESIAN_POINT('Ctrl Pts',(74.3084770981399,-6.20628833237051,
130.639003547736));
#213382=CARTESIAN_POINT('Ctrl Pts',(74.0300294743271,-3.49377002667009,
135.936507227495));
#213383=CARTESIAN_POINT('Ctrl Pts',(73.7515818505141,2.42935225338577,136.517818892029));
#213384=CARTESIAN_POINT('Ctrl Pts',(73.4731342267013,6.1200184930355,131.848741520285));
#213385=CARTESIAN_POINT('Ctrl Pts',(73.1946866028884,4.18668671711015,126.219929119786));
#213386=CARTESIAN_POINT('Ctrl Pts',(72.9162389790755,-1.59400562082267,
124.803985303816));
#213387=CARTESIAN_POINT('Ctrl Pts',(72.6377913552626,-5.90988466472314,
128.902093266552));
#213388=CARTESIAN_POINT('Ctrl Pts',(72.3593437314497,-4.79486841565966,
134.748291993943));
#213389=CARTESIAN_POINT('Ctrl Pts',(72.0808961076369,0.726397665050741,
136.970210458201));
#213390=CARTESIAN_POINT('Ctrl Pts',(71.8024484838239,5.58013977807825,133.526014137426));
#213391=CARTESIAN_POINT('Ctrl Pts',(71.524000860011,5.30600604003494,127.580751192065));
#213392=CARTESIAN_POINT('Ctrl Pts',(71.2455532361981,0.155911964005252,
124.597827826664));
#213393=CARTESIAN_POINT('Ctrl Pts',(70.9671056123853,-5.13745759022245,
127.318404890117));
#213394=CARTESIAN_POINT('Ctrl Pts',(70.6886579885723,-5.70975459779179,
133.242404968692));
#213395=CARTESIAN_POINT('Ctrl Pts',(70.4102103647595,-1.03506606700937,
136.925961393668));
#213396=CARTESIAN_POINT('Ctrl Pts',(70.1317627409465,4.59079761356593,134.98406576223));
#213397=CARTESIAN_POINT('Ctrl Pts',(69.8533151171337,5.99794256020584,129.201225292793));
#213398=CARTESIAN_POINT('Ctrl Pts',(69.5748674933208,1.89327130980037,124.891587869307));
#213399=CARTESIAN_POINT('Ctrl Pts',(69.2964198695077,-3.95122378286636,
126.015499746463));
#213400=CARTESIAN_POINT('Ctrl Pts',(69.0179722456952,-6.16473724709165,
131.540140815303));
#213401=CARTESIAN_POINT('Ctrl Pts',(68.7395246218819,-2.71315834539685,
136.388635827283));
#213402=CARTESIAN_POINT('Ctrl Pts',(68.4610769980694,3.23168053056381,136.105454728543));
#213403=CARTESIAN_POINT('Ctrl Pts',(68.1826293742561,6.20676287530703,130.950827114659));
#213404=CARTESIAN_POINT('Ctrl Pts',(67.9041817504435,3.47813335486666,125.661603945233));
#213405=CARTESIAN_POINT('Ctrl Pts',(67.6257341266304,-2.44673080243567,
125.09832292005));
#213406=CARTESIAN_POINT('Ctrl Pts',(67.3472865028177,-6.12316888174425,
129.778611783445));
#213407=CARTESIAN_POINT('Ctrl Pts',(67.0688388790048,-4.17271389215982,
135.401513714782));
#213408=CARTESIAN_POINT('Ctrl Pts',(66.7903912551918,1.61226131591331,136.799856533191));
#213409=CARTESIAN_POINT('Ctrl Pts',(66.511943631379,5.91564713800617,132.688631501398));
#213410=CARTESIAN_POINT('Ctrl Pts',(66.233496007566,4.78284223570014,126.845853579115));
#213411=CARTESIAN_POINT('Ctrl Pts',(65.9550483837533,-0.745161026381345,
124.640750241348));
#213412=CARTESIAN_POINT('Ctrl Pts',(65.6766007599402,-5.58839770835831,
128.099703730218));
#213413=CARTESIAN_POINT('Ctrl Pts',(65.3981531361275,-5.2961699047596,134.044104768727));
#213414=CARTESIAN_POINT('Ctrl Pts',(65.1197055123145,-0.137020690970298,
137.011339202618));
#213415=CARTESIAN_POINT('Ctrl Pts',(64.8412578885016,5.14804384398771,134.274663544608));
#213416=CARTESIAN_POINT('Ctrl Pts',(64.5628102646887,5.70230758224426,128.348949030369));
#213417=CARTESIAN_POINT('Ctrl Pts',(64.2843626408759,1.01642922563077,124.679637811238));
#213418=CARTESIAN_POINT('Ctrl Pts',(64.0059150170629,-4.60349793400934,
126.638647641779));
#213419=CARTESIAN_POINT('Ctrl Pts',(63.72746739325,-5.9930353856715,132.425744190676));
#213420=CARTESIAN_POINT('Ctrl Pts',(63.4490197694371,-1.87526609395646,
136.722868444874));
#213421=CARTESIAN_POINT('Ctrl Pts',(63.1705721456243,3.96578112626272,135.581173140958));
#213422=CARTESIAN_POINT('Ctrl Pts',(62.8921245218114,6.16246923062527,130.049820488308));
#213423=CARTESIAN_POINT('Ctrl Pts',(62.6136768979985,2.69614916540168,125.211853353112));
#213424=CARTESIAN_POINT('Ctrl Pts',(62.3352292741856,-3.24780026861702,
125.513127184779));
#213425=CARTESIAN_POINT('Ctrl Pts',(62.0567816503727,-6.20717991964031,
130.676786050054));
#213426=CARTESIAN_POINT('Ctrl Pts',(61.7783340265599,-3.46246446211126,
135.957679710507));
#213427=CARTESIAN_POINT('Ctrl Pts',(61.4998864027468,2.46408668530527,136.502924878181));
#213428=CARTESIAN_POINT('Ctrl Pts',(61.2214387789342,6.12626254625314,131.81146788069));
#213429=CARTESIAN_POINT('Ctrl Pts',(60.942991155121,4.15870241175792,126.194528508313));
#213430=CARTESIAN_POINT('Ctrl Pts',(60.6645435313083,-1.63050207523548,
124.813799641521));
#213431=CARTESIAN_POINT('Ctrl Pts',(60.3860959074953,-5.92135480954196,
128.938103656541));
#213432=CARTESIAN_POINT('Ctrl Pts',(60.1076482836825,-4.77077174814381,
134.777406647022));
#213433=CARTESIAN_POINT('Ctrl Pts',(59.8292006598696,0.763917484641806,
136.965674430521));
#213434=CARTESIAN_POINT('Ctrl Pts',(59.5507530360567,5.59660386848551,133.491995816827));
#213435=CARTESIAN_POINT('Ctrl Pts',(59.2723054122438,5.28628470648961,127.548511753291));
#213436=CARTESIAN_POINT('Ctrl Pts',(58.9938577884309,0.11812814859451,124.596993738963));
#213437=CARTESIAN_POINT('Ctrl Pts',(58.715410164618,-5.15858240697801,127.34974263934));
#213438=CARTESIAN_POINT('Ctrl Pts',(58.4369625408051,-5.69480774129836,
133.277116694236));
#213439=CARTESIAN_POINT('Ctrl Pts',(58.1585149169922,-0.997782968190397,
136.932148715521));
#213440=CARTESIAN_POINT('Ctrl Pts',(57.8800672931793,4.61615560827684,134.956042833877));
#213441=CARTESIAN_POINT('Ctrl Pts',(57.6016196693665,5.98807269247603,129.164743816393));
#213442=CARTESIAN_POINT('Ctrl Pts',(57.3231720455535,1.85724350590365,124.880172539454));
#213443=CARTESIAN_POINT('Ctrl Pts',(57.0447244217407,-3.98030173120474,
126.039640693622));
#213444=CARTESIAN_POINT('Ctrl Pts',(56.7662767979277,-6.16014412588574,
131.577653688385));
#213445=CARTESIAN_POINT('Ctrl Pts',(56.4878291741149,-2.67911500864857,
136.405048128532));
#213446=CARTESIAN_POINT('Ctrl Pts',(56.209381550302,3.26388991949243,136.085684354897));
#213447=CARTESIAN_POINT('Ctrl Pts',(55.9309339264891,6.20753946150667,130.913042073662));
#213448=CARTESIAN_POINT('Ctrl Pts',(55.6524863026762,3.44676349355797,125.640526843659));
#213449=CARTESIAN_POINT('Ctrl Pts',(55.3740386788633,-2.48141974121268,
125.113322584571));
#213450=CARTESIAN_POINT('Ctrl Pts',(55.0955910550504,-6.12929945790263,
129.815904255142));
#213451=CARTESIAN_POINT('Ctrl Pts',(54.8171434312375,-4.14465240570495,
135.426829034002));
#213452=CARTESIAN_POINT('Ctrl Pts',(54.5386958074246,1.64872772980914,136.789931158292));
#213453=CARTESIAN_POINT('Ctrl Pts',(54.2602481836117,5.92700762645589,132.652586367033));
#213454=CARTESIAN_POINT('Ctrl Pts',(53.9818005597989,4.75865706480954,126.81681240286));
#213455=CARTESIAN_POINT('Ctrl Pts',(53.703352935986,-0.78266686607524,124.645400445441));
#213456=CARTESIAN_POINT('Ctrl Pts',(53.4249053121731,-5.604758182439,128.133772004274));
#213457=CARTESIAN_POINT('Ctrl Pts',(53.1464576883601,-5.27635053680027,
134.076284033214));
#213458=CARTESIAN_POINT('Ctrl Pts',(52.8680100645473,-0.0992345118958833,
137.012058285519));
#213459=CARTESIAN_POINT('Ctrl Pts',(52.5895624407343,5.1690731815654,134.243261643865));
#213460=CARTESIAN_POINT('Ctrl Pts',(52.3111148169216,5.68725514443172,128.314282958697));
#213461=CARTESIAN_POINT('Ctrl Pts',(52.0326671931086,0.979127467424884,
124.673563994973));
#213462=CARTESIAN_POINT('Ctrl Pts',(51.7542195692957,-4.62877051910935,
126.666747621346));
#213463=CARTESIAN_POINT('Ctrl Pts',(51.4757719454828,-5.98305452659317,
132.462195457613));
#213464=CARTESIAN_POINT('Ctrl Pts',(51.1973243216699,-1.83920371260068,
136.734174065611));
#213465=CARTESIAN_POINT('Ctrl Pts',(50.9188766978571,3.99478546317524,135.556943802347));
#213466=CARTESIAN_POINT('Ctrl Pts',(50.6404290740441,6.15776195441257,130.012321768865));
#213467=CARTESIAN_POINT('Ctrl Pts',(50.3619814502312,2.66205603294,125.195544744091));
#213468=CARTESIAN_POINT('Ctrl Pts',(50.0835338264184,-3.27994933413751,
125.532995501151));
#213469=CARTESIAN_POINT('Ctrl Pts',(49.8050862026055,-6.20784149757545,
130.714573279694));
#213470=CARTESIAN_POINT('Ctrl Pts',(49.5266385787925,-3.43103059465853,
135.978661235386));
#213471=CARTESIAN_POINT('Ctrl Pts',(49.2481909549797,2.4987298095866,136.487819701939));
#213472=CARTESIAN_POINT('Ctrl Pts',(48.9697433311668,6.13227958855924,131.774156922365));
#213473=CARTESIAN_POINT('Ctrl Pts',(48.6912957073539,4.13056400415832,126.169298715863));
#213474=CARTESIAN_POINT('Ctrl Pts',(48.412848083541,-1.66693811079436,124.823835961664));
#213475=CARTESIAN_POINT('Ctrl Pts',(48.1344004597282,-5.93260553638082,
128.974183201367));
#213476=CARTESIAN_POINT('Ctrl Pts',(47.8559528359152,-4.7464982979263,134.806374077418));
#213477=CARTESIAN_POINT('Ctrl Pts',(47.5775052121024,0.801408996989757,
136.960910093092));
#213478=CARTESIAN_POINT('Ctrl Pts',(47.2990575882894,5.61286057467834,133.457877904919));
#213479=CARTESIAN_POINT('Ctrl Pts',(47.0206099644766,5.26636748772036,127.516392961194));
#213480=CARTESIAN_POINT('Ctrl Pts',(46.7421623406636,0.0803399559020909,
124.596389667526));
#213481=CARTESIAN_POINT('Ctrl Pts',(46.4637147168508,-5.17951607056515,
127.381208400702));
#213482=CARTESIAN_POINT('Ctrl Pts',(46.1852670930379,-5.67964986161014,
133.311736790894));
#213483=CARTESIAN_POINT('Ctrl Pts',(45.9068194692249,-0.960462896156299,
136.938108969933));
#213484=CARTESIAN_POINT('Ctrl Pts',(45.6283718454121,4.64134254964412,134.927866063412));
#213485=CARTESIAN_POINT('Ctrl Pts',(45.3499242215992,5.97798093451044,129.128323096598));
#213486=CARTESIAN_POINT('Ctrl Pts',(45.0714765977863,1.82114688116607,124.868976732569));
#213487=CARTESIAN_POINT('Ctrl Pts',(44.7930289739735,-4.00923218799886,
126.063958199228));
#213488=CARTESIAN_POINT('Ctrl Pts',(44.5145813501605,-6.15532273827383,
131.615137906808));
#213489=CARTESIAN_POINT('Ctrl Pts',(44.2361337263477,-2.644972396308,136.421252894246));
#213490=CARTESIAN_POINT('Ctrl Pts',(43.9576861025347,3.29597836378001,136.065718279858));
#213491=CARTESIAN_POINT('Ctrl Pts',(43.6792384787219,6.20808602504863,130.875253005433));
#213492=CARTESIAN_POINT('Ctrl Pts',(43.4007908549089,3.41526591116036,125.619641089845));
#213493=CARTESIAN_POINT('Ctrl Pts',(43.1223432310961,-2.5160167300689,125.128533132602));
#213494=CARTESIAN_POINT('Ctrl Pts',(42.8438956072832,-6.13520291061547,
129.853233354452));
#213495=CARTESIAN_POINT('Ctrl Pts',(42.5654479834703,-4.11643733763101,
135.451973065955));
#213496=CARTESIAN_POINT('Ctrl Pts',(42.2870003596574,1.68513304949262,136.779783985877));
#213497=CARTESIAN_POINT('Ctrl Pts',(42.0085527358444,5.93814848745852,132.616472745983));
#213498=CARTESIAN_POINT('Ctrl Pts',(41.7301051120316,4.73429556013123,126.787918986671));
#213499=CARTESIAN_POINT('Ctrl Pts',(41.4516574882187,-0.820143703760798,
124.65027887207));
#213500=CARTESIAN_POINT('Ctrl Pts',(41.1732098644058,-5.62091097014408,
128.167939237972));
#213501=CARTESIAN_POINT('Ctrl Pts',(40.8947622405929,-5.25633565173145,
134.108342055376));
#213502=CARTESIAN_POINT('Ctrl Pts',(40.61631461678,-0.0614446556499193,
137.012547339898));
#213503=CARTESIAN_POINT('Ctrl Pts',(40.3378669929672,5.18991097723558,134.211732313379));
#213504=CARTESIAN_POINT('Ctrl Pts',(40.0594193691542,5.67199196328813,128.279709157768));
#213505=CARTESIAN_POINT('Ctrl Pts',(39.7809717453414,0.941789427290636,
124.66771735763));
#213506=CARTESIAN_POINT('Ctrl Pts',(39.5025241215285,-4.65387158341555,
126.695000921683));
#213507=CARTESIAN_POINT('Ctrl Pts',(39.2240764977156,-5.97285196322902,
132.49858529287));
#213508=CARTESIAN_POINT('Ctrl Pts',(38.9456288739027,-1.80307317887526,
136.745259954929));
#213509=CARTESIAN_POINT('Ctrl Pts',(38.6671812500898,4.02364177184326,135.532538355018));
#213510=CARTESIAN_POINT('Ctrl Pts',(38.3887336262769,6.15282650006613,129.974852398711));
#213511=CARTESIAN_POINT('Ctrl Pts',(38.110286002464,2.62786425701304,125.179443971804));
#213512=CARTESIAN_POINT('Ctrl Pts',(37.8318383786511,-3.31197685992897,
125.553059149895));
#213513=CARTESIAN_POINT('Ctrl Pts',(37.5533907548383,-6.20827304166094,
130.752363836438));
#213514=CARTESIAN_POINT('Ctrl Pts',(37.2749431310254,-3.3994695891056,135.999451024653));
#213515=CARTESIAN_POINT('Ctrl Pts',(36.9964955072125,2.53328034251594,136.47250392303));
#213516=CARTESIAN_POINT('Ctrl Pts',(36.7180478833995,6.13806939699002,131.73681002788));
#213517=CARTESIAN_POINT('Ctrl Pts',(36.4396002595867,4.10227253699055,126.144240677337));
#213518=CARTESIAN_POINT('Ctrl Pts',(36.1611526357737,-1.70331237734853,
124.834093892349));
#213519=CARTESIAN_POINT('Ctrl Pts',(35.8827050119609,-5.94363642833981,
129.01033056409));
#213520=CARTESIAN_POINT('Ctrl Pts',(35.604257388148,-4.72204896446884,134.835193211735));
#213521=CARTESIAN_POINT('Ctrl Pts',(35.3258097643351,0.838870812832614,
136.955917622458));
#213522=CARTESIAN_POINT('Ctrl Pts',(35.0473621405222,5.62890929425843,133.423661665951));
#213523=CARTESIAN_POINT('Ctrl Pts',(34.7689145167094,5.24625512176713,127.484396005948));
#213524=CARTESIAN_POINT('Ctrl Pts',(34.4904668928964,0.0425487861828518,
124.596015634733));
#213525=CARTESIAN_POINT('Ctrl Pts',(34.2120192690835,-5.20025780527969,
127.412801008228));
#213526=CARTESIAN_POINT('Ctrl Pts',(33.9335716452707,-5.66428152040741,
133.346263975806));
#213527=CARTESIAN_POINT('Ctrl Pts',(33.6551240214578,-0.923107233816384,
136.943841936043));
#213528=CARTESIAN_POINT('Ctrl Pts',(33.3766763976448,4.66635750435639,134.899536494936));
#213529=CARTESIAN_POINT('Ctrl Pts',(33.098228773832,5.96766766026296,129.091964482989));
#213530=CARTESIAN_POINT('Ctrl Pts',(32.8197811500191,1.78498277316083,124.858000863516));
#213531=CARTESIAN_POINT('Ctrl Pts',(32.5413335262063,-4.03801408121996,
126.08845136219));
#213532=CARTESIAN_POINT('Ctrl Pts',(32.2628859023933,-6.15027326291425,
131.65259208158));
#213533=CARTESIAN_POINT('Ctrl Pts',(31.9844382785804,-2.6107317735426,136.437249523951));
#213534=CARTESIAN_POINT('Ctrl Pts',(31.7059906547675,3.32794467437699,136.045557243275));
#213535=CARTESIAN_POINT('Ctrl Pts',(31.4275430309546,6.20840254567991,130.837461310262));
#213536=CARTESIAN_POINT('Ctrl Pts',(31.1490954071417,3.3836417748287,125.598947457719));
#213537=CARTESIAN_POINT('Ctrl Pts',(30.8706477833288,-2.55052048699994,
125.143954000505));
#213538=CARTESIAN_POINT('Ctrl Pts',(30.5922001595159,-6.14087902112821,
129.890597698133));
#213539=CARTESIAN_POINT('Ctrl Pts',(30.3137525357031,-4.08806973345779,
135.476944878919));
#213540=CARTESIAN_POINT('Ctrl Pts',(30.0353049118902,1.72147592595096,136.769415391952));
#213541=CARTESIAN_POINT('Ctrl Pts',(29.7568572880773,5.94906930818524,132.58029197645));
#213542=CARTESIAN_POINT('Ctrl Pts',(29.4784096642643,4.70975862438989,126.759174401203));
#213543=CARTESIAN_POINT('Ctrl Pts',(29.1999620404515,-0.857590150719802,
124.65538534046));
#213544=CARTESIAN_POINT('Ctrl Pts',(28.9215144166386,-5.63685547292606,
128.202204165235));
#213545=CARTESIAN_POINT('Ctrl Pts',(28.6430667928257,-5.23612599121204,
134.140277647291));
#213546=CARTESIAN_POINT('Ctrl Pts',(28.3646191690128,-0.0236525225496446,
137.012806347637));
#213547=CARTESIAN_POINT('Ctrl Pts',(28.0861715451999,5.2105564588459,134.180076721482));
#213548=CARTESIAN_POINT('Ctrl Pts',(27.807723921387,5.65651860439647,128.245228908728));
#213549=CARTESIAN_POINT('Ctrl Pts',(27.5292762975741,0.904416488802812,
124.662098115861));
#213550=CARTESIAN_POINT('Ctrl Pts',(27.2508286737613,-4.67880019679877,
126.723406495856));
#213551=CARTESIAN_POINT('Ctrl Pts',(26.9723810499484,-5.96242807363892,
132.53491234801));
#213552=CARTESIAN_POINT('Ctrl Pts',(26.6939334261354,-1.76687583160983,
136.756125702037));
#213553=CARTESIAN_POINT('Ctrl Pts',(26.4154858023226,4.05234898298581,135.507957703324));
#213554=CARTESIAN_POINT('Ctrl Pts',(26.1370381785097,6.14766305047102,129.937413766291));
#213555=CARTESIAN_POINT('Ctrl Pts',(25.8585905546968,2.59357510460964,125.163551632871));
#213556=CARTESIAN_POINT('Ctrl Pts',(25.5801429308839,-3.34388165920016,
125.573317387547));
#213557=CARTESIAN_POINT('Ctrl Pts',(25.301695307071,-6.2084745359058,130.790156319941));
#213558=CARTESIAN_POINT('Ctrl Pts',(25.0232476832582,-3.36778261495664,
136.020048307934));
#213559=CARTESIAN_POINT('Ctrl Pts',(24.7448000594452,2.56773700381057,136.456978108987));
#213560=CARTESIAN_POINT('Ctrl Pts',(24.4663524356323,6.14363175700203,131.69942858114));
#213561=CARTESIAN_POINT('Ctrl Pts',(24.1879048118195,4.07382905860539,126.11935532127));
#213562=CARTESIAN_POINT('Ctrl Pts',(23.9094571880065,-1.73962352703587,
124.844573053462));
#213563=CARTESIAN_POINT('Ctrl Pts',(23.6310095641937,-5.95444707666522,
129.046544405257));
#213564=CARTESIAN_POINT('Ctrl Pts',(23.3525619403807,-4.69742465375045,
134.863862982068));
#213565=CARTESIAN_POINT('Ctrl Pts',(23.0741143165679,0.876301544009003,
136.950697203617));
#213566=CARTESIAN_POINT('Ctrl Pts',(22.795666692755,5.64474943253441,133.389348367819));
#213567=CARTESIAN_POINT('Ctrl Pts',(22.5172190689421,5.22594835390121,127.452522073212));
#213568=CARTESIAN_POINT('Ctrl Pts',(22.2387714451292,0.0047560398029127,
124.595871654449));
#213569=CARTESIAN_POINT('Ctrl Pts',(21.9603238213163,-5.22080684252888,
127.444519291243));
#213570=CARTESIAN_POINT('Ctrl Pts',(21.6818761975034,-5.64870328716988,
133.380696969555));
#213571=CARTESIAN_POINT('Ctrl Pts',(21.4034285736905,-0.885717365398449,
136.949347401415));
#213572=CARTESIAN_POINT('Ctrl Pts',(21.1249809498776,4.69119954547528,134.871055178212));
#213573=CARTESIAN_POINT('Ctrl Pts',(20.8465333260648,5.95713325189572,129.055669322849));
#213574=CARTESIAN_POINT('Ctrl Pts',(20.5680857022518,1.74875252196249,124.847245339011));
#213575=CARTESIAN_POINT('Ctrl Pts',(20.289638078439,-4.06664634434428,126.113119274905));
#213576=CARTESIAN_POINT('Ctrl Pts',(20.011190454626,-6.14499588691713,131.690014824823));
#213577=CARTESIAN_POINT('Ctrl Pts',(19.7327428308132,-2.57639440915122,
136.453037424885));
#213578=CARTESIAN_POINT('Ctrl Pts',(19.4542952070003,3.35978766676044,136.025201992224));
#213579=CARTESIAN_POINT('Ctrl Pts',(19.1758475831874,6.20848901167171,130.799668388532));
#213580=CARTESIAN_POINT('Ctrl Pts',(18.8973999593745,3.3518922564065,125.578446714094));
#213581=CARTESIAN_POINT('Ctrl Pts',(18.6189523355616,-2.58492973345636,
125.159584616859));
#213582=CARTESIAN_POINT('Ctrl Pts',(18.3405047117487,-6.14632757911053,
129.927995901635));
#213583=CARTESIAN_POINT('Ctrl Pts',(18.0620570879358,-4.05955064435711,
135.501743547556));
#213584=CARTESIAN_POINT('Ctrl Pts',(17.7836094641229,1.75775501248606,136.758825760728));
#213585=CARTESIAN_POINT('Ctrl Pts',(17.5051618403101,5.95976968396092,132.544045399129));
#213586=CARTESIAN_POINT('Ctrl Pts',(17.2267142164972,4.68504716681072,126.730579711598));
#213587=CARTESIAN_POINT('Ctrl Pts',(16.9482665926842,-0.8950048193604,124.660719661391));
#213588=CARTESIAN_POINT('Ctrl Pts',(16.6698189688713,-5.65259109995534,
128.236565516362));
#213589=CARTESIAN_POINT('Ctrl Pts',(16.3913713450585,-5.21572230411858,
134.172089625574));
#213590=CARTESIAN_POINT('Ctrl Pts',(16.1129237212456,0.0141404870033325,
137.012835299135));
#213591=CARTESIAN_POINT('Ctrl Pts',(15.8344760974327,5.23100886137047,134.148296041183));
#213592=CARTESIAN_POINT('Ctrl Pts',(15.5560284736198,5.64083564112771,128.210843489254));
#213593=CARTESIAN_POINT('Ctrl Pts',(15.2775808498069,0.8670100368296,124.656706477888));
#213594=CARTESIAN_POINT('Ctrl Pts',(14.999133225994,-4.70355543551987,126.751963291284));
#213595=CARTESIAN_POINT('Ctrl Pts',(14.7206856021811,-5.95178324408404,
132.571175276918));
#213596=CARTESIAN_POINT('Ctrl Pts',(14.4422379783683,-1.73061301211068,
136.766770904302));
#213597=CARTESIAN_POINT('Ctrl Pts',(14.1637903545553,4.08090603284655,135.48320275811));
#213598=CARTESIAN_POINT('Ctrl Pts',(13.8853427307424,6.14227179696077,129.900007258904));
#213599=CARTESIAN_POINT('Ctrl Pts',(13.6068951069296,2.55918984632695,125.147868316191));
#213600=CARTESIAN_POINT('Ctrl Pts',(13.3284474831167,-3.37566254970675,
125.593769463429));
#213601=CARTESIAN_POINT('Ctrl Pts',(13.0499998593037,-6.20844597284355,
130.827949329789));
#213602=CARTESIAN_POINT('Ctrl Pts',(12.7715522354909,-3.33597084638438,
136.04045232199));
#213603=CARTESIAN_POINT('Ctrl Pts',(12.493104611678,2.60209851666622,136.441242835124));
#213604=CARTESIAN_POINT('Ctrl Pts',(12.2146569878651,6.14896646247997,131.662013967328));
#213605=CARTESIAN_POINT('Ctrl Pts',(11.9362093640522,4.04523462298623,126.094643569795));
#213606=CARTESIAN_POINT('Ctrl Pts',(11.6577617402393,-1.77587021433397,
124.855273056695));
#213607=CARTESIAN_POINT('Ctrl Pts',(11.3793141164265,-5.96503708076441,
129.08282338295));
#213608=CARTESIAN_POINT('Ctrl Pts',(11.1008664926135,-4.67262627823404,
134.892382326048));
#213609=CARTESIAN_POINT('Ctrl Pts',(10.8224188688007,0.913699803509421,
136.945249030013));
#213610=CARTESIAN_POINT('Ctrl Pts',(10.5439712449878,5.6603804025445,133.354939282016));
#213611=CARTESIAN_POINT('Ctrl Pts',(10.2655236211749,5.20544793659703,127.420772344084));
#213612=CARTESIAN_POINT('Ctrl Pts',(9.98707599736195,-0.0330368828140487,
124.595957732005));
#213613=CARTESIAN_POINT('Ctrl Pts',(9.70862837354909,-5.24116242086055,
127.476362074414));
#213614=CARTESIAN_POINT('Ctrl Pts',(9.43018074973619,-5.63291573915475,
133.415034496211));
#213615=CARTESIAN_POINT('Ctrl Pts',(9.15173312592329,-0.848294676398009,
136.954625162043));
#213616=CARTESIAN_POINT('Ctrl Pts',(8.87328550211039,4.71586775246963,134.842423168626));
#213617=CARTESIAN_POINT('Ctrl Pts',(8.59483787829755,5.94637809976527,129.019438961107));
#213618=CARTESIAN_POINT('Ctrl Pts',(8.3163902544846,1.71245747009635,124.836710557603));
#213619=CARTESIAN_POINT('Ctrl Pts',(8.03794263067172,-4.09512791639282,
126.137961023291));
#213620=CARTESIAN_POINT('Ctrl Pts',(7.75949500685887,-6.1394908058375,131.727404749824));
#213621=CARTESIAN_POINT('Ctrl Pts',(7.48104738304595,-2.54196157551782,
136.468616012024));
#213622=CARTESIAN_POINT('Ctrl Pts',(7.20259975923305,3.39150616097622,136.004653280976));
#213623=CARTESIAN_POINT('Ctrl Pts',(6.92415213542018,6.20834541982004,130.761875640674));
#213624=CARTESIAN_POINT('Ctrl Pts',(6.64570451160728,3.32001853238404,125.558139618628));
#213625=CARTESIAN_POINT('Ctrl Pts',(6.36725688779438,-2.61924319439064,
125.175424402463));
#213626=CARTESIAN_POINT('Ctrl Pts',(6.08880926398148,-6.15154838266407,
129.965426579154));
#213627=CARTESIAN_POINT('Ctrl Pts',(5.81036164016863,-4.03088112711464,
135.52636815294));
#213628=CARTESIAN_POINT('Ctrl Pts',(5.53191401635571,1.79396896476278,136.748015484609));
#213629=CARTESIAN_POINT('Ctrl Pts',(5.2534663925428,5.97024921827925,132.507734357147));
#213630=CARTESIAN_POINT('Ctrl Pts',(4.97501876872993,4.66016210308585,126.702135977443));
#213631=CARTESIAN_POINT('Ctrl Pts',(4.69657114491704,-0.932386323268277,
124.666281637197));
#213632=CARTESIAN_POINT('Ctrl Pts',(4.41812352110413,-5.66811726814286,
128.27102201808));
#213633=CARTESIAN_POINT('Ctrl Pts',(4.13967589729124,-5.19512534651691,
134.203776811419));
#213634=CARTESIAN_POINT('Ctrl Pts',(3.86122827347838,0.051932972575587,
137.012634193321));
#213635=CARTESIAN_POINT('Ctrl Pts',(3.58278064966546,5.25126742693796,134.116391450127));
#213636=CARTESIAN_POINT('Ctrl Pts',(3.30433302585255,5.62494365461986,128.176554173511));
#213637=CARTESIAN_POINT('Ctrl Pts',(3.02588540203969,0.829571457480427,
124.651542643499));
#213638=CARTESIAN_POINT('Ctrl Pts',(2.74743777822681,-4.72813638226476,
126.780670249786));
#213639=CARTESIAN_POINT('Ctrl Pts',(2.46899015441389,-5.9409178690121,132.607372735859));
#213640=CARTESIAN_POINT('Ctrl Pts',(2.19054253060099,-1.69428606410994,
136.77719516726));
#213641=CARTESIAN_POINT('Ctrl Pts',(1.91209490678813,4.10931186323347,135.458274436681));
#213642=CARTESIAN_POINT('Ctrl Pts',(1.63364728297522,6.13665293931019,129.862634262664));
#213643=CARTESIAN_POINT('Ctrl Pts',(1.35519965916232,2.52470975632363,125.132394602912));
#213644=CARTESIAN_POINT('Ctrl Pts',(1.07675203534945,-3.40731835379603,
125.614414619682));
#213645=CARTESIAN_POINT('Ctrl Pts',(0.798304411536565,-6.20818735353264,
130.86574146555));
#213646=CARTESIAN_POINT('Ctrl Pts',(0.519856787723634,-3.30403546218559,
136.060662310741));
#213647=CARTESIAN_POINT('Ctrl Pts',(0.241409163910791,2.63636360780418,
136.425298684517));
#213648=CARTESIAN_POINT('Ctrl Pts',(-0.0370384599021062,6.15407331574431,
131.624567572855));
#213649=CARTESIAN_POINT('Ctrl Pts',(-0.315486083715014,4.01649028971072,
126.070106338619));
#213650=CARTESIAN_POINT('Ctrl Pts',(-0.593933707527915,-1.81205109610819,
124.866193505555));
#213651=CARTESIAN_POINT('Ctrl Pts',(-0.872381331340776,-5.97540604822092,
129.119166152838));
#213652=CARTESIAN_POINT('Ctrl Pts',(-1.15082895515369,-4.6476547568326,
134.920750186879));
#213653=CARTESIAN_POINT('Ctrl Pts',(-1.42927657896659,0.951064205527318,
136.939573303531));
#213654=CARTESIAN_POINT('Ctrl Pts',(-1.70772420277945,5.67580162507719,
133.320435683583));
#213655=CARTESIAN_POINT('Ctrl Pts',(-1.98617182659235,5.18475462950527,
127.389147995065));
#213656=CARTESIAN_POINT('Ctrl Pts',(-2.26461945040527,-0.0708285812371651,
124.596273864213));
#213657=CARTESIAN_POINT('Ctrl Pts',(-2.54306707421816,-5.26132378599129,
127.508328177794));
#213658=CARTESIAN_POINT('Ctrl Pts',(-2.82151469803103,-5.61691946137538,
133.449275283389));
#213659=CARTESIAN_POINT('Ctrl Pts',(-3.09996232184393,-0.810840553526189,
136.959675022356));
#213660=CARTESIAN_POINT('Ctrl Pts',(-3.37840994565684,4.74036121125036,
134.813641527147));
#213661=CARTESIAN_POINT('Ctrl Pts',(-3.6568575694697,5.93540260240737,128.983274740293));
#213662=CARTESIAN_POINT('Ctrl Pts',(-3.9353051932826,1.6760989624889,124.826396909662));
#213663=CARTESIAN_POINT('Ctrl Pts',(-4.21375281709551,-4.12345774197041,
126.162975686831));
#213664=CARTESIAN_POINT('Ctrl Pts',(-4.49220044090841,-6.13375822366836,
131.764760471086));
#213665=CARTESIAN_POINT('Ctrl Pts',(-4.77064806472125,-2.50743454856317,
136.483984708096));
#213666=CARTESIAN_POINT('Ctrl Pts',(-5.04909568853418,3.4230989816841,135.983911870971));
#213667=CARTESIAN_POINT('Ctrl Pts',(-5.32754331234708,6.20797177544568,
130.724084467112));
#213668=CARTESIAN_POINT('Ctrl Pts',(-5.60599093615995,3.28802178385396,
125.538026923812));
#213669=CARTESIAN_POINT('Ctrl Pts',(-5.88443855997284,-2.65345959830539,
125.191472770368));
#213670=CARTESIAN_POINT('Ctrl Pts',(-6.16288618378574,-6.15654123833006,
130.002888343683));
#213671=CARTESIAN_POINT('Ctrl Pts',(-6.44133380759864,-4.00206224408943,
135.550817782599));
#213672=CARTESIAN_POINT('Ctrl Pts',(-6.71978143141151,1.83011644085978,
136.736984964173));
#213673=CARTESIAN_POINT('Ctrl Pts',(-6.9982290552244,5.98050752281724,132.471360196026));
#213674=CARTESIAN_POINT('Ctrl Pts',(-7.27667667903734,4.63510435534053,
126.673844252731));
#213675=CARTESIAN_POINT('Ctrl Pts',(-7.55512430285017,-0.969733277257762,
124.672071061776));
#213676=CARTESIAN_POINT('Ctrl Pts',(-7.83357192666308,-5.68343340216059,
128.305572393592));
#213677=CARTESIAN_POINT('Ctrl Pts',(-8.112019550476,-5.17433588163501,134.235338030648));
#213678=CARTESIAN_POINT('Ctrl Pts',(-8.39046717428886,0.0897235337524442,
137.012203037646));
#213679=CARTESIAN_POINT('Ctrl Pts',(-8.66891479810176,5.27133140485959,
134.084364130551));
#213680=CARTESIAN_POINT('Ctrl Pts',(-8.94736242191464,5.60884323375645,
128.142362232103));
#213681=CARTESIAN_POINT('Ctrl Pts',(-9.22581004572757,0.792102138056052,
124.646606804043));
#213682=CARTESIAN_POINT('Ctrl Pts',(-9.50425766954039,-4.75254212617725,
126.809526307613));
#213683=CARTESIAN_POINT('Ctrl Pts',(-9.78270529335335,-5.92983235104376,
132.643503383524));
#213684=CARTESIAN_POINT('Ctrl Pts',(-10.0611529171662,-1.65789633371603,
136.787398104638));
#213685=CARTESIAN_POINT('Ctrl Pts',(-10.3396005409791,4.13756542155812,
135.433173662763));
#213686=CARTESIAN_POINT('Ctrl Pts',(-10.618048164792,6.13080668572826,129.82529616244));
#213687=CARTESIAN_POINT('Ctrl Pts',(-10.8964957886049,2.49013611227157,
125.11713106642));
#213688=CARTESIAN_POINT('Ctrl Pts',(-11.1749434124178,-3.4388478984508,
125.635252091294));
#213689=CARTESIAN_POINT('Ctrl Pts',(-11.4533910362307,-6.20769868755626,
130.90353132682));
#213690=CARTESIAN_POINT('Ctrl Pts',(-11.7318386600436,-3.2719776457377,
136.080677525301));
#213691=CARTESIAN_POINT('Ctrl Pts',(-12.0102862838565,2.67053100751937,
136.409146247984));
#213692=CARTESIAN_POINT('Ctrl Pts',(-12.2887339076694,6.15895212755882,
131.587090785312));
#213693=CARTESIAN_POINT('Ctrl Pts',(-12.5671815314823,3.98759712391021,
126.045744536976));
#213694=CARTESIAN_POINT('Ctrl Pts',(-12.8456291552951,-1.84816483166266,
124.877333995382));
#213695=CARTESIAN_POINT('Ctrl Pts',(-13.1240767791081,-5.98555359480885,
129.155571368227));
#213696=CARTESIAN_POINT('Ctrl Pts',(-13.4025244029209,-4.62251101487491,
134.948965513381));
#213697=CARTESIAN_POINT('Ctrl Pts',(-13.6809720267338,0.988393365511613,
136.933670234486));
#213698=CARTESIAN_POINT('Ctrl Pts',(-13.9594196505467,5.69101252869335,
133.285838851062));
#213699=CARTESIAN_POINT('Ctrl Pts',(-14.2378672743596,5.16386919942402,
127.357650198006));
#213700=CARTESIAN_POINT('Ctrl Pts',(-14.5163148981725,-0.108617655081171,
124.59682003936));
#213701=CARTESIAN_POINT('Ctrl Pts',(-14.7947625219854,-5.28129019083405,
127.540416416869));
#213702=CARTESIAN_POINT('Ctrl Pts',(-15.0732101457983,-5.60071504657988,
133.483418062279));
#213703=CARTESIAN_POINT('Ctrl Pts',(-15.3516577696111,-0.77335638465969,
136.96449679523));
#213704=CARTESIAN_POINT('Ctrl Pts',(-15.6301053934241,4.76467901420313,
134.784711320289));
#213705=CARTESIAN_POINT('Ctrl Pts',(-15.908553017237,5.92420716652329,128.947178000488));
#213706=CARTESIAN_POINT('Ctrl Pts',(-16.1870006410499,1.63967834641818,
124.816304777366));
#213707=CARTESIAN_POINT('Ctrl Pts',(-16.4654482648627,-4.15163477130477,
126.188162338596));
#213708=CARTESIAN_POINT('Ctrl Pts',(-16.7438958886757,-6.12779835283271,
131.802080604377));
#213709=CARTESIAN_POINT('Ctrl Pts',(-17.0223435124885,-2.4728146076992,
136.499142943608));
#213710=CARTESIAN_POINT('Ctrl Pts',(-17.3007911363014,3.45456495820035,
135.96297853079));
#213711=CARTESIAN_POINT('Ctrl Pts',(-17.5792387601143,6.20736809239421,
130.686296268213));
#213712=CARTESIAN_POINT('Ctrl Pts',(-17.8576863839272,3.25590319646751,
125.518109374927));
#213713=CARTESIAN_POINT('Ctrl Pts',(-18.13613400774,-2.6875776772989,125.207729125896));
#213714=CARTESIAN_POINT('Ctrl Pts',(-18.414581631553,-6.16130596109642,
130.040379807061));
#213715=CARTESIAN_POINT('Ctrl Pts',(-18.6930292553659,-3.97309506317598,
135.575091530542));
#213716=CARTESIAN_POINT('Ctrl Pts',(-18.9714768791788,1.86619610131902,
136.72573460816));
#213717=CARTESIAN_POINT('Ctrl Pts',(-19.2499245029916,5.99054421744964,
132.434924263623));
#213718=CARTESIAN_POINT('Ctrl Pts',(-19.5283721268046,4.6098748520987,126.645705585822));
#213719=CARTESIAN_POINT('Ctrl Pts',(-19.8068197506174,-1.00704429742433,
124.678087720601));
#213720=CARTESIAN_POINT('Ctrl Pts',(-20.0852673744304,-5.6985389344635,
128.340215362621));
#213721=CARTESIAN_POINT('Ctrl Pts',(-20.3637149982432,-5.15335467983417,
134.266772113748));
#213722=CARTESIAN_POINT('Ctrl Pts',(-20.6421626220562,0.127510770190762,
137.011541848088));
#213723=CARTESIAN_POINT('Ctrl Pts',(-20.920610245869,5.29120005165768,134.05221526924));
#213724=CARTESIAN_POINT('Ctrl Pts',(-21.1990578696819,5.59253497514422,
128.108268932023));
#213725=CARTESIAN_POINT('Ctrl Pts',(-21.4775054934948,0.754603466995427,
124.64189914242));
#213726=CARTESIAN_POINT('Ctrl Pts',(-21.7559531173077,-4.77677176289349,
126.838530395495));
#213727=CARTESIAN_POINT('Ctrl Pts',(-22.0344007411205,-5.91852710095694,
132.679565881077));
#213728=CARTESIAN_POINT('Ctrl Pts',(-22.3128483649335,-1.62144516936395,
136.797379338361));
#213729=CARTESIAN_POINT('Ctrl Pts',(-22.5912959887463,4.16566566087426,
135.407901366475));
#213730=CARTESIAN_POINT('Ctrl Pts',(-22.8697436125593,6.12473325285015,
129.787994341809));
#213731=CARTESIAN_POINT('Ctrl Pts',(-23.1481912363721,2.45547019531011,
125.102078272311));
#213732=CARTESIAN_POINT('Ctrl Pts',(-23.426638860185,-3.47025001533206,
125.656281106122));
#213733=CARTESIAN_POINT('Ctrl Pts',(-23.7050864839979,-6.20697999302203,
130.941317513284));
#213734=CARTESIAN_POINT('Ctrl Pts',(-23.9835341078108,-3.23979858495512,
136.100497223997));
#213735=CARTESIAN_POINT('Ctrl Pts',(-24.2619817316237,2.70459944972584,
136.392786124057));
#213736=CARTESIAN_POINT('Ctrl Pts',(-24.5404293554366,6.16360271713728,
131.549584993415));
#213737=CARTESIAN_POINT('Ctrl Pts',(-24.8188769792495,3.95855619623184,
126.021559067602));
#213738=CARTESIAN_POINT('Ctrl Pts',(-25.0973246030624,-1.88421008278963,
124.88869411336));
#213739=CARTESIAN_POINT('Ctrl Pts',(-25.3757722268753,-5.99547934450715,
129.192037680109));
#213740=CARTESIAN_POINT('Ctrl Pts',(-25.6542198506882,-4.59719598407162,
134.977027260026));
#213741=CARTESIAN_POINT('Ctrl Pts',(-25.932667474501,1.02568590021626,136.92754004162));
#213742=CARTESIAN_POINT('Ctrl Pts',(-26.211115098314,5.7060125497474,133.251150066453));
#213743=CARTESIAN_POINT('Ctrl Pts',(-26.4895627221268,5.14279242027056,
127.326280120068));
#213744=CARTESIAN_POINT('Ctrl Pts',(-26.7680103459397,-0.146402704058008,
124.597596237205));
#213745=CARTESIAN_POINT('Ctrl Pts',(-27.0464579697526,-5.30106089552683,
127.572625602596));
#213746=CARTESIAN_POINT('Ctrl Pts',(-27.3249055935655,-5.58430309522854,
133.517461567711));
#213747=CARTESIAN_POINT('Ctrl Pts',(-27.6033532173784,-0.735843558787732,
136.969090301993));
#213748=CARTESIAN_POINT('Ctrl Pts',(-27.8818008411913,4.78882026022281,
134.755633620073));
#213749=CARTESIAN_POINT('Ctrl Pts',(-28.1602484650042,5.91279220696403,
128.911150079267));
#213750=CARTESIAN_POINT('Ctrl Pts',(-28.4386960888171,1.60319697146318,
124.806434534681));
#213751=CARTESIAN_POINT('Ctrl Pts',(-28.7171437126299,-4.17965796028613,
126.213520045287));
#213752=CARTESIAN_POINT('Ctrl Pts',(-28.9955913364429,-6.12161141417542,
131.839363766787));
#213753=CARTESIAN_POINT('Ctrl Pts',(-29.2740389602557,-2.43810303578058,
136.514090156867));
#213754=CARTESIAN_POINT('Ctrl Pts',(-29.5524865840687,3.48590292454168,
135.941854036124));
#213755=CARTESIAN_POINT('Ctrl Pts',(-29.8309342078815,6.20653439303521,
130.648512444231));
#213756=CARTESIAN_POINT('Ctrl Pts',(-30.1093818316944,3.22366396039099,
125.498387710026));
#213757=CARTESIAN_POINT('Ctrl Pts',(-30.3878294555073,-2.72159616711309,
125.224192866663));
#213758=CARTESIAN_POINT('Ctrl Pts',(-30.6662770793202,-6.16584237440457,
130.077899580028));
#213759=CARTESIAN_POINT('Ctrl Pts',(-30.9447247031331,-3.94398065776386,
135.599188497297));
#213760=CARTESIAN_POINT('Ctrl Pts',(-31.2231723269461,1.90220660919519,
136.714264833456));
#213761=CARTESIAN_POINT('Ctrl Pts',(-31.5016199507588,6.00035893026297,
132.398427910084));
#213762=CARTESIAN_POINT('Ctrl Pts',(-31.7800675745718,4.58447452824918,
126.617721019404));
#213763=CARTESIAN_POINT('Ctrl Pts',(-32.0585151983846,-1.04431800119413,
124.68433139072));
#213764=CARTESIAN_POINT('Ctrl Pts',(-32.3369628221976,-5.71343330531054,
128.374949641459));
#213765=CARTESIAN_POINT('Ctrl Pts',(-32.6154104460104,-5.1321825185805,
134.298077895915));
#213766=CARTESIAN_POINT('Ctrl Pts',(-32.8938580698234,0.165293281670594,
137.010650649146));
#213767=CARTESIAN_POINT('Ctrl Pts',(-33.1723056936362,5.31087263109202,
134.019946057479));
#213768=CARTESIAN_POINT('Ctrl Pts',(-33.4507533174492,5.57601948309184,
128.074275536613));
#213769=CARTESIAN_POINT('Ctrl Pts',(-33.729200941262,0.717076833825826,
124.637419833072));
#213770=CARTESIAN_POINT('Ctrl Pts',(-34.0076485650749,-4.80082439457541,
126.867681438675));
#213771=CARTESIAN_POINT('Ctrl Pts',(-34.2860961888878,-5.90700253767186,
132.715558892209));
#213772=CARTESIAN_POINT('Ctrl Pts',(-34.5645438127007,-1.58493392176466,
136.807138498572));
#213773=CARTESIAN_POINT('Ctrl Pts',(-34.8429914365135,4.19361153991761,
135.382458484293));
#213774=CARTESIAN_POINT('Ctrl Pts',(-35.1214390603265,6.11843286572883,
129.750730183006));
#213775=CARTESIAN_POINT('Ctrl Pts',(-35.3998866841394,2.42071328999757,
125.087236778371));
#213776=CARTESIAN_POINT('Ctrl Pts',(-35.6783343079523,-3.50152354082281,
125.677500884929));
#213777=CARTESIAN_POINT('Ctrl Pts',(-35.9567819317651,-6.20603129656164,
130.979098624759));
#213778=CARTESIAN_POINT('Ctrl Pts',(-36.2352295555781,-3.2074994722443,
136.120120672404));
#213779=CARTESIAN_POINT('Ctrl Pts',(-36.5136771793909,2.73856767200523,
136.376218918968));
#213780=CARTESIAN_POINT('Ctrl Pts',(-36.7921248032039,6.1680249121504,131.512051586954));
#213781=CARTESIAN_POINT('Ctrl Pts',(-37.0705724270167,3.92936858279784,
125.997550826698));
#213782=CARTESIAN_POINT('Ctrl Pts',(-37.3490200508296,-1.92018551381882,
124.900273438536));
#213783=CARTESIAN_POINT('Ctrl Pts',(-37.6274676746425,-6.00518292951342,
129.228563737208));
#213784=CARTESIAN_POINT('Ctrl Pts',(-37.9059152984554,-4.57171060248077,
135.004934386972));
#213785=CARTESIAN_POINT('Ctrl Pts',(-38.1843629222683,1.0629404277527,136.921182952087));
#213786=CARTESIAN_POINT('Ctrl Pts',(-38.4628105460811,5.72080113240803,
133.216370615161));
#213787=CARTESIAN_POINT('Ctrl Pts',(-38.7412581698941,5.12152507305273,
127.295038923683));
#213788=CARTESIAN_POINT('Ctrl Pts',(-39.0197057937069,-0.184182328028525,
124.598602428988));
#213789=CARTESIAN_POINT('Ctrl Pts',(-39.2981534175199,-5.32063516745863,
127.604954541453));
#213790=CARTESIAN_POINT('Ctrl Pts',(-39.5766010413327,-5.56768421547239,
133.55140453819));
#213791=CARTESIAN_POINT('Ctrl Pts',(-39.8550486651457,-0.698303465962086,
136.973455372429));
#213792=CARTESIAN_POINT('Ctrl Pts',(-40.1334962889585,4.81278405474664,
134.726409503982));
#213793=CARTESIAN_POINT('Ctrl Pts',(-40.4119439127715,5.90115814671511,
128.875192311658));
#213794=CARTESIAN_POINT('Ctrl Pts',(-40.6903915365843,1.56665618945481,
124.796786547352));
#213795=CARTESIAN_POINT('Ctrl Pts',(-40.9688391603973,-4.20752627050468,
126.239047867263));
#213796=CARTESIAN_POINT('Ctrl Pts',(-41.2472867842101,-6.11519763695597,
131.876608576776));
#213797=CARTESIAN_POINT('Ctrl Pts',(-41.5257344080229,-2.40330111905734,
136.528825793999));
#213798=CARTESIAN_POINT('Ctrl Pts',(-41.8041820318359,3.51711171946819,
135.920539169751));
#213799=CARTESIAN_POINT('Ctrl Pts',(-42.0826296556488,6.20547070826194,
130.610734395262));
#213800=CARTESIAN_POINT('Ctrl Pts',(-42.3610772794617,3.19130527026066,
125.478862659902));
#213801=CARTESIAN_POINT('Ctrl Pts',(-42.6395249032745,-2.75551380718057,
125.240863382598));
#213802=CARTESIAN_POINT('Ctrl Pts',(-42.9179725270875,-6.17015031015604,
130.115446272278));
#213803=CARTESIAN_POINT('Ctrl Pts',(-43.1964201509003,-3.91472010669807,
135.623107789941));
#213804=CARTESIAN_POINT('Ctrl Pts',(-43.4748677747133,1.93814663010615,
136.702576065077));
#213805=CARTESIAN_POINT('Ctrl Pts',(-43.7533153985261,6.00995129756958,
132.361872487794));
#213806=CARTESIAN_POINT('Ctrl Pts',(-44.031763022339,4.55890432500984,126.589891590455));
#213807=CARTESIAN_POINT('Ctrl Pts',(-44.3102106461518,-1.08155300737633,
124.690801840773));
#213808=CARTESIAN_POINT('Ctrl Pts',(-44.5886582699649,-5.72811596278534,
128.409773943013));
#213809=CARTESIAN_POINT('Ctrl Pts',(-44.8671058937777,-5.11082018241628,
134.329254217104));
#213810=CARTESIAN_POINT('Ctrl Pts',(-45.1455535175906,0.2030696681468,137.009529473845));
#213811=CARTESIAN_POINT('Ctrl Pts',(-45.4240011414034,5.33034841418793,
133.987557691017));
#213812=CARTESIAN_POINT('Ctrl Pts',(-45.7024487652165,5.55929736958694,
128.040383305508));
#213813=CARTESIAN_POINT('Ctrl Pts',(-45.9808963890292,0.679523629110432,
124.633169041983));
#213814=CARTESIAN_POINT('Ctrl Pts',(-46.2593440128422,-4.82469912994364,
126.896978356949));
#213815=CARTESIAN_POINT('Ctrl Pts',(-46.537791636655,-5.89525908823553,
132.751481083186));
#213816=CARTESIAN_POINT('Ctrl Pts',(-46.816239260468,-1.54836394385628,
136.816675223641));
#213817=CARTESIAN_POINT('Ctrl Pts',(-47.0946868842807,4.22140202314317,
135.35684595901));
#213818=CARTESIAN_POINT('Ctrl Pts',(-47.3731345080937,6.11190575782758,
129.713505066864));
#213819=CARTESIAN_POINT('Ctrl Pts',(-47.6515821319066,2.38586668426401,
125.072607134557));
#213820=CARTESIAN_POINT('Ctrl Pts',(-47.9300297557195,-3.53266731607082,
125.69891064141));
#213821=CARTESIAN_POINT('Ctrl Pts',(-48.2084773795324,-6.20485263332943,
131.016873261253));
#213822=CARTESIAN_POINT('Ctrl Pts',(-48.4869250033452,-3.17508150446096,
136.139547143367));
#213823=CARTESIAN_POINT('Ctrl Pts',(-48.7653726271582,2.77243441565242,
136.359445246621));
#213824=CARTESIAN_POINT('Ctrl Pts',(-49.043820250971,6.1722185487321,131.474491956744));
#213825=CARTESIAN_POINT('Ctrl Pts',(-49.322267874784,3.900035365166,125.973720703898));
#213826=CARTESIAN_POINT('Ctrl Pts',(-49.6007154985968,-1.95608979166789,
124.912071541833));
#213827=CARTESIAN_POINT('Ctrl Pts',(-49.8791631224098,-6.0146639902579,
129.265148186042));
#213828=CARTESIAN_POINT('Ctrl Pts',(-50.1576107462225,-4.54605581447205,
135.032685860113));
#213829=CARTESIAN_POINT('Ctrl Pts',(-50.4360583700356,1.10015556764067,
136.914599201455));
#213830=CARTESIAN_POINT('Ctrl Pts',(-50.7145059938484,5.73537772867887,
133.181501785951));
#213831=CARTESIAN_POINT('Ctrl Pts',(-50.9929536176612,5.10006794583985,
127.263927766504));
#213832=CARTESIAN_POINT('Ctrl Pts',(-51.2714012414742,-0.221955127055423,
124.599838577421));
#213833=CARTESIAN_POINT('Ctrl Pts',(-51.5498488652871,-5.34001228129766,
127.637402035479));
#213834=CARTESIAN_POINT('Ctrl Pts',(-51.8282964891,-5.5508590231301,133.585245715947));
#213835=CARTESIAN_POINT('Ctrl Pts',(-52.1067441129128,-0.660737497244709,
136.977591844792));
#213836=CARTESIAN_POINT('Ctrl Pts',(-52.3851917367258,4.8365695097872,134.697040054928));
#213837=CARTESIAN_POINT('Ctrl Pts',(-52.6636393605386,5.889305416881,128.83930603009));
#213838=CARTESIAN_POINT('Ctrl Pts',(-52.9420869843516,1.53005735442545,
124.78736117289));
#213839=CARTESIAN_POINT('Ctrl Pts',(-53.2205346081644,-4.23523866929,126.264744858582));
#213840=CARTESIAN_POINT('Ctrl Pts',(-53.4989822319774,-6.1085572588392,
131.913813654221));
#213841=CARTESIAN_POINT('Ctrl Pts',(-53.7774298557902,-2.36841014712749,
136.543349308967));
#213842=CARTESIAN_POINT('Ctrl Pts',(-54.0558774796031,3.54819018652628,
135.8990347215));
#213843=CARTESIAN_POINT('Ctrl Pts',(-54.334325103416,6.20417707748961,130.572963521183));
#213844=CARTESIAN_POINT('Ctrl Pts',(-54.6127727272289,3.15882832513996,
125.459534948064));
#213845=CARTESIAN_POINT('Ctrl Pts',(-54.8912203510417,-2.7893293406706,
125.257740055968));
#213846=CARTESIAN_POINT('Ctrl Pts',(-55.1696679748547,-6.17422960871856,
130.153018492501));
#213847=CARTESIAN_POINT('Ctrl Pts',(-55.4481155986676,-3.88531449423931,
135.646848522136));
#213848=CARTESIAN_POINT('Ctrl Pts',(-55.7265632224805,1.97401483228084,
136.690668736158));
#213849=CARTESIAN_POINT('Ctrl Pts',(-56.0050108462934,6.01932096392068,
132.32525935133));
#213850=CARTESIAN_POINT('Ctrl Pts',(-56.2834584701062,4.53316518989421,
126.562218330207));
#213851=CARTESIAN_POINT('Ctrl Pts',(-56.5619060939192,-1.11874793621411,
124.697498830995));
#213852=CARTESIAN_POINT('Ctrl Pts',(-56.840353717732,-5.74258636281662,
128.444686976857));
#213853=CARTESIAN_POINT('Ctrl Pts',(-57.118801341545,-5.08926846293066,
134.360299922064));
#213854=CARTESIAN_POINT('Ctrl Pts',(-57.3972489653578,0.240838529802063,
137.00817836373));
#213855=CARTESIAN_POINT('Ctrl Pts',(-57.6756965891708,5.34962667926312,
133.955051370017));
#213856=CARTESIAN_POINT('Ctrl Pts',(-57.9541442129836,5.54236925427356,
128.0065934946));
#213857=CARTESIAN_POINT('Ctrl Pts',(-58.2325918367966,0.641945244397073,
124.629146926667));
#213858=CARTESIAN_POINT('Ctrl Pts',(-58.5110394606094,-4.84839508431156,
126.92642006471));
#213859=CARTESIAN_POINT('Ctrl Pts',(-58.7894870844223,-5.88329718780563,
132.787331122898));
#213860=CARTESIAN_POINT('Ctrl Pts',(-59.0679347082352,-1.5117365907523,
136.825989160181));
#213861=CARTESIAN_POINT('Ctrl Pts',(-59.3463823320481,4.24903608076433,
135.331064739709));
#213862=CARTESIAN_POINT('Ctrl Pts',(-59.624829955861,6.10515217101086,129.676320372777));
#213863=CARTESIAN_POINT('Ctrl Pts',(-59.9032775796738,2.3509316693629,125.058189882977));
#213864=CARTESIAN_POINT('Ctrl Pts',(-60.1817252034868,-3.56368018703254,
125.720509582217));
#213865=CARTESIAN_POINT('Ctrl Pts',(-60.4601728272995,-6.20344404700091,
131.054640023013));
#213866=CARTESIAN_POINT('Ctrl Pts',(-60.7386204511126,-3.14254588286485,
136.158775917031));
#213867=CARTESIAN_POINT('Ctrl Pts',(-61.0170680749254,2.80619842572279,
136.342465728569));
#213868=CARTESIAN_POINT('Ctrl Pts',(-61.2955156987383,6.17618347148551,
131.436907494571));
#213869=CARTESIAN_POINT('Ctrl Pts',(-61.5739633225512,3.87055763028967,
125.950069582238));
#213870=CARTESIAN_POINT('Ctrl Pts',(-61.8524109463641,-1.9919215858902,
124.924087986069));
#213871=CARTESIAN_POINT('Ctrl Pts',(-62.130858570177,-6.02392217541635,
129.301789670958));
#213872=CARTESIAN_POINT('Ctrl Pts',(-62.4093061939898,-4.5202325706933,
135.060280651108));
#213873=CARTESIAN_POINT('Ctrl Pts',(-62.6877538178028,1.13732994085927,
136.907789033684));
#213874=CARTESIAN_POINT('Ctrl Pts',(-62.9662014416156,5.74974179841868,
133.146544870902));
#213875=CARTESIAN_POINT('Ctrl Pts',(-63.2446490654287,5.0784218337339,127.232947801366));
#213876=CARTESIAN_POINT('Ctrl Pts',(-63.5230966892413,-0.25971970145348,
124.601304636701));
#213877=CARTESIAN_POINT('Ctrl Pts',(-63.8015443130544,-5.3591915190178,
127.669966882319));
#213878=CARTESIAN_POINT('Ctrl Pts',(-64.0799919368672,-5.53382814166538,
133.618983846983));
#213879=CARTESIAN_POINT('Ctrl Pts',(-64.3584395606801,-0.623147044656387,
136.9814995658));
#213880=CARTESIAN_POINT('Ctrl Pts',(-64.636887184493,4.86017574396616,134.667526361205));
#213881=CARTESIAN_POINT('Ctrl Pts',(-64.9153348083059,5.8772344566688,128.803492564343));
#213882=CARTESIAN_POINT('Ctrl Pts',(-65.1937824321189,1.4934018225579,124.778158760555));
#213883=CARTESIAN_POINT('Ctrl Pts',(-65.4722300559316,-4.26279412974889,
126.290610067033));
#213884=CARTESIAN_POINT('Ctrl Pts',(-65.7506776797446,-6.10169052588679,
131.950977620477));
#213885=CARTESIAN_POINT('Ctrl Pts',(-66.0291253035574,-2.33343141288849,
136.5576601636));
#213886=CARTESIAN_POINT('Ctrl Pts',(-66.3075729273703,3.57913717409239,
135.877341488227));
#213887=CARTESIAN_POINT('Ctrl Pts',(-66.5860205511832,6.20265354865397,
130.535201221608));
#213888=CARTESIAN_POINT('Ctrl Pts',(-66.8644681749961,3.126234328474,125.440405290707));
#213889=CARTESIAN_POINT('Ctrl Pts',(-67.142915798809,-2.82304151453613,
125.274822261403));
#213890=CARTESIAN_POINT('Ctrl Pts',(-67.421363422622,-6.17808011893247,
130.190614848446));
#213891=CARTESIAN_POINT('Ctrl Pts',(-67.6998110464348,-3.85576491002292,
135.670409814162));
#213892=CARTESIAN_POINT('Ctrl Pts',(-67.9782586702478,2.00980988661012,
136.678543287925));
#213893=CARTESIAN_POINT('Ctrl Pts',(-68.2567062940606,6.02846758211988,
132.288589857404));
#213894=CARTESIAN_POINT('Ctrl Pts',(-68.5351539178734,4.50725807667536,
126.534702264101));
#213895=CARTESIAN_POINT('Ctrl Pts',(-68.8136015416864,-1.15590140943545,
124.704422113226));
#213896=CARTESIAN_POINT('Ctrl Pts',(-69.0920491654993,-5.75684396919829,
128.479687449276));
#213897=CARTESIAN_POINT('Ctrl Pts',(-69.3704967893121,-5.0675281587308,
134.391213860386));
#213898=CARTESIAN_POINT('Ctrl Pts',(-69.648944413125,0.278598467097045,
137.006597368867));
#213899=CARTESIAN_POINT('Ctrl Pts',(-69.9273920369379,5.36870671195437,
133.922428299012));
#213900=CARTESIAN_POINT('Ctrl Pts',(-70.2058396607509,5.52523576442926,
127.972907355982));
#213901=CARTESIAN_POINT('Ctrl Pts',(-70.4842872845636,0.604343072166899,
124.625353636165));
#213902=CARTESIAN_POINT('Ctrl Pts',(-70.7627349083767,-4.87191137961658,
126.956005470983));
#213903=CARTESIAN_POINT('Ctrl Pts',(-71.0411825321895,-5.87111727963483,
132.823107682909));
#213904=CARTESIAN_POINT('Ctrl Pts',(-71.3196301560023,-1.47505321969301,
136.835079963061));
#213905=CARTESIAN_POINT('Ctrl Pts',(-71.5980777798154,4.27651268879093,
135.305115781721));
#213906=CARTESIAN_POINT('Ctrl Pts',(-71.8765254036282,6.09817235553532,
129.639177478635));
#213907=CARTESIAN_POINT('Ctrl Pts',(-72.1549730274411,2.31590953982396,
125.043985557866));
#213908=CARTESIAN_POINT('Ctrl Pts',(-72.433420651254,-3.5945610045145,125.742296906994));
#213909=CARTESIAN_POINT('Ctrl Pts',(-72.7118682750669,-6.20180558977201,
131.092397510578));
#213910=CARTESIAN_POINT('Ctrl Pts',(-72.9903158988798,-3.109893813075,136.177806280867));
#213911=CARTESIAN_POINT('Ctrl Pts',(-73.2687635226926,2.8398584510789,136.325280993997));
#213912=CARTESIAN_POINT('Ctrl Pts',(-73.5472111465057,6.17991953348924,
131.399299593141));
#213913=CARTESIAN_POINT('Ctrl Pts',(-73.8256587703184,3.84093647047644,
125.926598338115));
#213914=CARTESIAN_POINT('Ctrl Pts',(-74.1041063941314,-2.02767956872624,
124.93632232597));
#213915=CARTESIAN_POINT('Ctrl Pts',(-74.3825540179442,-6.0329571419232,
129.338486834193));
#213916=CARTESIAN_POINT('Ctrl Pts',(-74.6610016417573,-4.49424182803428,
135.08771773742));
#213917=CARTESIAN_POINT('Ctrl Pts',(-74.9394492655699,1.17446216989917,
136.900752701129));
#213918=CARTESIAN_POINT('Ctrl Pts',(-75.217896889383,5.76389280936176,133.111501165354));
#213919=CARTESIAN_POINT('Ctrl Pts',(-75.4963445131958,5.05658753883907,
127.202100176243));
#213920=CARTESIAN_POINT('Ctrl Pts',(-75.7747921370087,-0.297474651842549,
124.603000552501));
#213921=CARTESIAN_POINT('Ctrl Pts',(-76.0532397608216,-5.37817216992523,
127.702647875272));
#213922=CARTESIAN_POINT('Ctrl Pts',(-76.3316873846344,-5.51659220216403,
133.65261768112));
#213923=CARTESIAN_POINT('Ctrl Pts',(-76.6101350084474,-0.585533501125347,
136.985178390654));
#213924=CARTESIAN_POINT('Ctrl Pts',(-76.8885826322602,4.8836018825454,134.637869516455));
#213925=CARTESIAN_POINT('Ctrl Pts',(-77.1670302560731,5.86494571337264,
128.767753241497));
#213926=CARTESIAN_POINT('Ctrl Pts',(-77.4454778798861,1.4566909521364,124.769179651345));
#213927=CARTESIAN_POINT('Ctrl Pts',(-77.7239255036988,-4.29019163080361,
126.316642534169));
#213928=CARTESIAN_POINT('Ctrl Pts',(-78.0023731275119,-6.09459769254796,
131.988099098418));
#213929=CARTESIAN_POINT('Ctrl Pts',(-78.2808207513247,-2.29836621249045,
136.571757827603));
#213930=CARTESIAN_POINT('Ctrl Pts',(-78.5592683751376,3.60995153541429,
135.855460273781));
#213931=CARTESIAN_POINT('Ctrl Pts',(-78.8377159989505,6.20090017820995,
130.497448895834));
#213932=CARTESIAN_POINT('Ctrl Pts',(-79.1161636227633,3.09352448804556,
125.421474396687));
#213933=CARTESIAN_POINT('Ctrl Pts',(-79.3946112465763,-2.85664907955992,
125.292109365916));
#213934=CARTESIAN_POINT('Ctrl Pts',(-79.6730588703891,-6.18170169811556,
130.228233946967));
#213935=CARTESIAN_POINT('Ctrl Pts',(-79.9515064942021,-3.8260724490201,
135.693790792945));
#213936=CARTESIAN_POINT('Ctrl Pts',(-80.2299541180149,2.04553046669522,
136.666200169693));
#213937=CARTESIAN_POINT('Ctrl Pts',(-80.5084017418279,6.03739081323573,
132.251865364817));
#213938=CARTESIAN_POINT('Ctrl Pts',(-80.7868493656406,4.48118394535095,
126.507344411756));
#213939=CARTESIAN_POINT('Ctrl Pts',(-81.0652969894537,-1.19301205030527,
124.711571430921));
#213940=CARTESIAN_POINT('Ctrl Pts',(-81.3437446132665,-5.77088825360962,
128.514774063314));
#213941=CARTESIAN_POINT('Ctrl Pts',(-81.6221922370794,-5.04560007541116,
134.421994886542));
#213942=CARTESIAN_POINT('Ctrl Pts',(-81.9006398608923,0.316348080823153,
137.00478654784));
#213943=CARTESIAN_POINT('Ctrl Pts',(-82.179087484705,5.38758780524389,133.889689686862));
#213944=CARTESIAN_POINT('Ctrl Pts',(-82.4575351085182,5.50789753494193,
127.939326137905));
#213945=CARTESIAN_POINT('Ctrl Pts',(-82.7359827323308,0.566718505781886,
124.621789311041));
#213946=CARTESIAN_POINT('Ctrl Pts',(-83.0144303561439,-4.89524714445407,
126.985733479472));
#213947=CARTESIAN_POINT('Ctrl Pts',(-83.2928779799568,-5.858719815054,132.858809437506));
#213948=CARTESIAN_POINT('Ctrl Pts',(-83.5713256037696,-1.43831518999427,
136.843947295418));
#213949=CARTESIAN_POINT('Ctrl Pts',(-83.8497732275826,4.30383082906709,
135.279000046597));
#213950=CARTESIAN_POINT('Ctrl Pts',(-84.1282208513953,6.09096657004034,
129.602077760783));
#213951=CARTESIAN_POINT('Ctrl Pts',(-84.4066684752085,2.28080159340614,
125.029994685571));
#213952=CARTESIAN_POINT('Ctrl Pts',(-84.685116099021,-3.6253086242162,125.764271808403));
#213953=CARTESIAN_POINT('Ctrl Pts',(-84.9635637228342,-6.19993732235617,
131.130144324829));
#213954=CARTESIAN_POINT('Ctrl Pts',(-85.242011346647,-3.07712650502686,
136.196637529698));
#213955=CARTESIAN_POINT('Ctrl Pts',(-85.5204589704598,2.87341324443482,
136.307891679689));
#213956=CARTESIAN_POINT('Ctrl Pts',(-85.7989065942728,6.18342659630218,
131.361669646028));
#213957=CARTESIAN_POINT('Ctrl Pts',(-86.0773542180856,3.81117298335027,
125.903307841269));
#213958=CARTESIAN_POINT('Ctrl Pts',(-86.3558018418987,-2.06336241514917,
124.948774108188));
#213959=CARTESIAN_POINT('Ctrl Pts',(-86.6342494657113,-6.04176855498474,
129.375238315919));
#213960=CARTESIAN_POINT('Ctrl Pts',(-86.9126970895244,-4.46808454959173,
135.114996102359));
#213961=CARTESIAN_POINT('Ctrl Pts',(-87.1911447133372,1.2115508788106,136.893490464523));
#213962=CARTESIAN_POINT('Ctrl Pts',(-87.4695923371502,5.77783023713722,
133.076371967865));
#213963=CARTESIAN_POINT('Ctrl Pts',(-87.7480399609628,5.03456587023344,
127.171386034204));
#213964=CARTESIAN_POINT('Ctrl Pts',(-88.026487584776,-0.33521857919891,
124.60492626198));
#213965=CARTESIAN_POINT('Ctrl Pts',(-88.3049352085887,-5.39695353068522,
127.735443803332));
#213966=CARTESIAN_POINT('Ctrl Pts',(-88.5833828324018,-5.49915184330967,
133.686145972045));
#213967=CARTESIAN_POINT('Ctrl Pts',(-88.8618304562145,-0.547898260434929,
136.988628183031));
#213968=CARTESIAN_POINT('Ctrl Pts',(-89.1402780800275,4.90684705746115,
134.608070619623));
#213969=CARTESIAN_POINT('Ctrl Pts',(-89.4187257038403,5.85243964235601,
128.732089385887));
#213970=CARTESIAN_POINT('Ctrl Pts',(-89.6971733276532,1.41992610349655,
124.760424177987));
#213971=CARTESIAN_POINT('Ctrl Pts',(-89.9756209514662,-4.31743015722937,
126.342841295349));
#213972=CARTESIAN_POINT('Ctrl Pts',(-90.254068575279,-6.08727902165076,
132.025176712493));
#213973=CARTESIAN_POINT('Ctrl Pts',(-90.5325161990919,-2.26321584528708,
136.585641778581));
#213974=CARTESIAN_POINT('Ctrl Pts',(-90.8109638229048,3.64063212865448,
135.833391888981));
#213975=CARTESIAN_POINT('Ctrl Pts',(-91.0894114467178,6.19891703112955,
130.459707942787));
#213976=CARTESIAN_POINT('Ctrl Pts',(-91.3678590705306,3.06070001592934,
125.402742967496));
#213977=CARTESIAN_POINT('Ctrl Pts',(-91.6463066943433,-2.89015079040179,
125.309600728926));
#213978=CARTESIAN_POINT('Ctrl Pts',(-91.9247543181566,-6.18509421206894,
130.265874394073));
#213979=CARTESIAN_POINT('Ctrl Pts',(-92.2032019419691,-3.79623821149537,
135.716990592095));
#213980=CARTESIAN_POINT('Ctrl Pts',(-92.4816495657822,2.08117524889636,
136.653639838841));
#213981=CARTESIAN_POINT('Ctrl Pts',(-92.7600971895951,6.04609032661485,
132.21508723441));
#213982=CARTESIAN_POINT('Ctrl Pts',(-93.0385448134079,4.45494376210749,
126.480145786926));
#213983=CARTESIAN_POINT('Ctrl Pts',(-93.3169924372209,-1.23007848367479,
124.718946519161));
#213984=CARTESIAN_POINT('Ctrl Pts',(-93.5954400610337,-5.78471869563455,
128.549945518824));
#213985=CARTESIAN_POINT('Ctrl Pts',(-93.8738876848466,-5.02348502552524,
134.45264185993));
#213986=CARTESIAN_POINT('Ctrl Pts',(-94.1523353086595,0.354085972155003,
137.002745967751));
#213987=CARTESIAN_POINT('Ctrl Pts',(-94.4307829324724,5.40626925948619,
133.85683674671));
#213988=CARTESIAN_POINT('Ctrl Pts',(-94.7092305562852,5.49035520828578,
127.905851084735));
#213989=CARTESIAN_POINT('Ctrl Pts',(-94.9876781800983,0.529072939433998,
124.618454083368));
#213990=CARTESIAN_POINT('Ctrl Pts',(-95.2661258039109,-4.91840151410816,
127.015602988595));
#213991=CARTESIAN_POINT('Ctrl Pts',(-95.5445734277241,-5.84610525345601,
132.894435063746));
#213992=CARTESIAN_POINT('Ctrl Pts',(-95.8230210515366,-1.40152386299717,
136.85259082867));
#213993=CARTESIAN_POINT('Ctrl Pts',(-96.10146867535,4.33098948930923,135.252718502061));
#213994=CARTESIAN_POINT('Ctrl Pts',(-96.3799162991623,6.08353508153927,
129.565022593965));
#213995=CARTESIAN_POINT('Ctrl Pts',(-96.6583639229758,2.245609131046,125.01621778453));
#213996=CARTESIAN_POINT('Ctrl Pts',(-96.9368115467883,-3.65592190677386,
125.786433472156));
#213997=CARTESIAN_POINT('Ctrl Pts',(-97.2152591706015,-6.19783931398261,
131.167879067045));
#213998=CARTESIAN_POINT('Ctrl Pts',(-97.493706794414,-3.04424517292474,
136.215268965725));
#213999=CARTESIAN_POINT('Ctrl Pts',(-97.7721544182274,2.90686156240656,
136.290298430015));
#214000=CARTESIAN_POINT('Ctrl Pts',(-98.0506020420397,6.18670452996842,
131.324019047625));
#214001=CARTESIAN_POINT('Ctrl Pts',(-98.3290496658531,3.78126827180747,
125.880198954735));
#214002=CARTESIAN_POINT('Ctrl Pts',(-98.6074972896656,-2.09896880291958,
124.961442871316));
#214003=CARTESIAN_POINT('Ctrl Pts',(-98.8859449134787,-6.05035608809047,
129.412042754299));
#214004=CARTESIAN_POINT('Ctrl Pts',(-99.1643925372916,-4.44176170463296,
135.142114735114));
#214005=CARTESIAN_POINT('Ctrl Pts',(-99.4428401611044,1.24859469325925,
136.886002592972));
#214006=CARTESIAN_POINT('Ctrl Pts',(-99.7212877849174,5.79155356528836,
133.041158580159));
#214007=CARTESIAN_POINT('Ctrl Pts',(-99.9997354087301,5.01235764393804,
127.140806513377));
#214008=CARTESIAN_POINT('Ctrl Pts',(-100.278183032543,-0.37295008490757,
124.607081693777));
#214009=CARTESIAN_POINT('Ctrl Pts',(-100.556630656356,-5.41553490534739,
127.768353451233));
#214010=CARTESIAN_POINT('Ctrl Pts',(-100.835078280169,-5.48150771136145,
133.719567477352));
#214011=CARTESIAN_POINT('Ctrl Pts',(-101.113525903981,-0.510242717172956,
136.9918488151));
#214012=CARTESIAN_POINT('Ctrl Pts',(-101.391973527794,4.92991040735466,
134.578130774917));
#214013=CARTESIAN_POINT('Ctrl Pts',(-101.670421151607,5.83971670703623,
128.696502319049));
#214014=CARTESIAN_POINT('Ctrl Pts',(-101.94886877542,1.38310863897239,124.751892664915));
#214015=CARTESIAN_POINT('Ctrl Pts',(-102.227316399233,-4.34450869969331,
126.36920537977));
#214016=CARTESIAN_POINT('Ctrl Pts',(-102.505764023046,-6.07973478439049,
132.062209088779));
#214017=CARTESIAN_POINT('Ctrl Pts',(-102.784211646859,-2.22798161378826,
136.599311502058));
#214018=CARTESIAN_POINT('Ctrl Pts',(-103.062659270672,3.6711778169323,135.811137151577));
#214019=CARTESIAN_POINT('Ctrl Pts',(-103.341106894485,6.19670418089893,
130.42197976097));
#214020=CARTESIAN_POINT('Ctrl Pts',(-103.619554518298,3.02776212844844,
125.384211697232));
#214021=CARTESIAN_POINT('Ctrl Pts',(-103.89800214211,-2.92354540564323,
125.327295702285));
#214022=CARTESIAN_POINT('Ctrl Pts',(-104.176449765923,-6.18825753508174,
130.303534794984));
#214023=CARTESIAN_POINT('Ctrl Pts',(-104.454897389736,-3.76626330296762,
135.740008351935));
#214024=CARTESIAN_POINT('Ctrl Pts',(-104.733345013549,2.1167429123828,136.640862760796));
#214025=CARTESIAN_POINT('Ctrl Pts',(-105.011792637362,6.05456579989334,
132.17825682901));
#214026=CARTESIAN_POINT('Ctrl Pts',(-105.290240261175,4.42853849928509,
126.453107397468));
#214027=CARTESIAN_POINT('Ctrl Pts',(-105.568687884988,-1.26709933603374,
124.726547104658));
#214028=CARTESIAN_POINT('Ctrl Pts',(-105.847135508801,-5.79833478278087,
128.585200512514));
#214029=CARTESIAN_POINT('Ctrl Pts',(-106.125583132613,-5.00118382855433,
134.483153644914));
#214030=CARTESIAN_POINT('Ctrl Pts',(-106.404030756427,0.391810742700936,
137.000475704212));
#214031=CARTESIAN_POINT('Ctrl Pts',(-106.682478380239,5.42475038243292,
133.823870695931));
#214032=CARTESIAN_POINT('Ctrl Pts',(-106.960926004052,5.47260943449832,
127.872483436902));
#214033=CARTESIAN_POINT('Ctrl Pts',(-107.239373627865,0.491407768093767,
124.615348076738));
#214034=CARTESIAN_POINT('Ctrl Pts',(-107.517821251678,-4.94137363058539,
127.045612891524));
#214035=CARTESIAN_POINT('Ctrl Pts',(-107.796268875491,-5.83327406227795,
132.929983241508));
#214036=CARTESIAN_POINT('Ctrl Pts',(-108.074716499304,-1.36468060201792,
136.861010242526));
#214037=CARTESIAN_POINT('Ctrl Pts',(-108.353164123117,4.3579876631431,135.22627212199));
#214038=CARTESIAN_POINT('Ctrl Pts',(-108.631611746929,6.07587816540856,
129.528013351273));
#214039=CARTESIAN_POINT('Ctrl Pts',(-108.910059370743,2.21033345681367,
125.00265536525));
#214040=CARTESIAN_POINT('Ctrl Pts',(-109.188506994555,-3.68639971780079,
125.808781077045));
#214041=CARTESIAN_POINT('Ctrl Pts',(-109.466954618368,-6.19551164239422,
131.205600338952));
#214042=CARTESIAN_POINT('Ctrl Pts',(-109.745402242181,-3.01125103519769,
136.233699898554));
#214043=CARTESIAN_POINT('Ctrl Pts',(-110.023849865994,2.94020216555433,
136.272501896897));
#214044=CARTESIAN_POINT('Ctrl Pts',(-110.302297489807,6.18975321302316,
131.286349193086));
#214045=CARTESIAN_POINT('Ctrl Pts',(-110.58074511362,3.75122344397827,125.857272534824));
#214046=CARTESIAN_POINT('Ctrl Pts',(-110.859192737433,-2.13449741262907,
124.974328145912));
#214047=CARTESIAN_POINT('Ctrl Pts',(-111.137640361246,-6.05871942302636,
129.44889878553));
#214048=CARTESIAN_POINT('Ctrl Pts',(-111.416087985058,-4.41527426856075,
135.169072630797));
#214049=CARTESIAN_POINT('Ctrl Pts',(-111.694535608871,1.28559224057236,
136.878289363941));
#214050=CARTESIAN_POINT('Ctrl Pts',(-111.972983232684,5.8050622852923,133.005862307081));
#214051=CARTESIAN_POINT('Ctrl Pts',(-112.251430856497,4.9899636828869,127.110362746893));
#214052=CARTESIAN_POINT('Ctrl Pts',(-112.52987848031,-0.410667770813077,
124.609466768025));
#214053=CARTESIAN_POINT('Ctrl Pts',(-112.808326104123,-5.43391560537209,
127.801375599495));
#214054=CARTESIAN_POINT('Ctrl Pts',(-113.086773727936,-5.46366046012913,
133.752880958598));
#214055=CARTESIAN_POINT('Ctrl Pts',(-113.365221351749,-0.472568266679477,
136.994840167519));
#214056=CARTESIAN_POINT('Ctrl Pts',(-113.643668975562,4.95279107760506,
134.548051091771));
#214057=CARTESIAN_POINT('Ctrl Pts',(-113.922116599375,5.8267773788663,128.660993359675));
#214058=CARTESIAN_POINT('Ctrl Pts',(-114.200564223187,1.34623992284899,
124.74358542827));
#214059=CARTESIAN_POINT('Ctrl Pts',(-114.479011847001,-4.37142625478972,
126.395733810498));
#214060=CARTESIAN_POINT('Ctrl Pts',(-114.757459470813,-6.07196526032194,
132.099194855029));
#214061=CARTESIAN_POINT('Ctrl Pts',(-115.035907094626,-2.19266482361144,
136.612766491501));
#214062=CARTESIAN_POINT('Ctrl Pts',(-115.314354718439,3.70158746836604,
135.788696886227));
#214063=CARTESIAN_POINT('Ctrl Pts',(-115.592802342252,6.19426170951602,
130.384265748418));
#214064=CARTESIAN_POINT('Ctrl Pts',(-115.871249966065,2.99471204612843,
125.36588127258));
#214065=CARTESIAN_POINT('Ctrl Pts',(-116.149697589878,-2.95683168783455,
125.345193630298));
#214066=CARTESIAN_POINT('Ctrl Pts',(-116.428145213691,-6.19119154993583,
130.34121375418));
#214067=CARTESIAN_POINT('Ctrl Pts',(-116.706592837503,-3.73614883416816,
135.762843219532));
#214068=CARTESIAN_POINT('Ctrl Pts',(-116.985040461316,2.1522321391827,136.627869409019));
#214069=CARTESIAN_POINT('Ctrl Pts',(-117.263488085129,6.06281691900968,
132.14137551338));
#214070=CARTESIAN_POINT('Ctrl Pts',(-117.541935708942,4.40196913533955,
126.426230245297));
#214071=CARTESIAN_POINT('Ctrl Pts',(-117.820383332755,-1.30407323556081,
124.73437290577));
#214072=CARTESIAN_POINT('Ctrl Pts',(-118.098830956568,-5.81173601049948,
128.620537737998));
#214073=CARTESIAN_POINT('Ctrl Pts',(-118.377278580381,-4.97869731087745,
134.51352911087));
#214074=CARTESIAN_POINT('Ctrl Pts',(-118.655726204194,0.429520994555717,
136.997975841351));
#214075=CARTESIAN_POINT('Ctrl Pts',(-118.934173828006,5.44303048925927,
133.790792756097));
#214076=CARTESIAN_POINT('Ctrl Pts',(-119.21262145182,5.45466087115571,127.839224430854));
#214077=CARTESIAN_POINT('Ctrl Pts',(-119.491069075632,0.453724387457947,
124.612471406243));
#214078=CARTESIAN_POINT('Ctrl Pts',(-119.769516699445,-4.96416264264509,
127.075762076232));
#214079=CARTESIAN_POINT('Ctrl Pts',(-120.047964323258,-5.82022671698453,
132.965452653541));
#214080=CARTESIAN_POINT('Ctrl Pts',(-120.326411947071,-1.32778677229758,
136.869205225004));
#214081=CARTESIAN_POINT('Ctrl Pts',(-120.604859570884,4.38482435014149,
135.199661886361));
#214082=CARTESIAN_POINT('Ctrl Pts',(-120.883307194697,6.06799610537801,
129.491051404098));
#214083=CARTESIAN_POINT('Ctrl Pts',(-121.16175481851,2.17497587786225,124.989307930291));
#214084=CARTESIAN_POINT('Ctrl Pts',(-121.440202442323,-3.71674092793051,
125.831313794972));
#214085=CARTESIAN_POINT('Ctrl Pts',(-121.718650066136,-6.19295439384353,
131.243306742772));
#214086=CARTESIAN_POINT('Ctrl Pts',(-121.997097689948,-2.97814531445616,
136.251929645219));
#214087=CARTESIAN_POINT('Ctrl Pts',(-122.275545313761,2.97343381842962,
136.254502739794));
#214088=CARTESIAN_POINT('Ctrl Pts',(-122.553992937574,6.19257253249627,
131.248661478285));
#214089=CARTESIAN_POINT('Ctrl Pts',(-122.832440561387,3.72103961318487,
125.83452943108));
#214090=CARTESIAN_POINT('Ctrl Pts',(-123.1108881852,-2.16994692775201,124.987429454503));
#214091=CARTESIAN_POINT('Ctrl Pts',(-123.389335809013,-6.06685824988591,
129.485805043896));
#214092=CARTESIAN_POINT('Ctrl Pts',(-123.667783432826,-4.38862322287681,
135.19586879047));
#214093=CARTESIAN_POINT('Ctrl Pts',(-123.946231056639,1.32254214979223,
136.870351063246));
#214094=CARTESIAN_POINT('Ctrl Pts',(-124.224678680451,5.81835589657845,
132.97048445655));
#214095=CARTESIAN_POINT('Ctrl Pts',(-124.503126304264,4.96738481689638,
127.080055862859));
#214096=CARTESIAN_POINT('Ctrl Pts',(-124.781573928077,-0.448370239273912,
124.612081396343));
#214097=CARTESIAN_POINT('Ctrl Pts',(-125.06002155189,-5.4520949496557,127.834509024472));
#214098=CARTESIAN_POINT('Ctrl Pts',(-125.338469175703,-5.44561075094924,
133.786085181339));
#214099=CARTESIAN_POINT('Ctrl Pts',(-125.616916799516,-0.434876304995071,
136.997602129441));
#214100=CARTESIAN_POINT('Ctrl Pts',(-125.895364423329,4.97548822036069,
134.517832684797));
#214101=CARTESIAN_POINT('Ctrl Pts',(-126.173812047142,5.8136221373178,128.625563823564));
#214102=CARTESIAN_POINT('Ctrl Pts',(-126.452259670955,1.30932132131015,
124.735502775877));
#214103=CARTESIAN_POINT('Ctrl Pts',(-126.730707294768,-4.39818182507867,
126.422425604514));
#214104=CARTESIAN_POINT('Ctrl Pts',(-127.00915491858,-6.0639707373477,132.136132640718));
#214105=CARTESIAN_POINT('Ctrl Pts',(-127.287602542393,-2.15726678343353,
136.626006248326));
#214106=CARTESIAN_POINT('Ctrl Pts',(-127.566050166206,3.73185995611441,
135.766071924465));
#214107=CARTESIAN_POINT('Ctrl Pts',(-127.844497790019,6.19158970748781,
130.346567302635));
#214108=CARTESIAN_POINT('Ctrl Pts',(-128.122945413832,2.96155099365221,
125.34775237278));
#214109=CARTESIAN_POINT('Ctrl Pts',(-128.401393037645,-2.99000840354028,
125.363293849751));
#214110=CARTESIAN_POINT('Ctrl Pts',(-128.679840661458,-6.19389614791022,
130.378909875453));
#214111=CARTESIAN_POINT('Ctrl Pts',(-128.958288285271,-3.70589592099968,
135.785494348734));
#214112=CARTESIAN_POINT('Ctrl Pts',(-129.236735909083,2.18764161422919,
136.614660264981));
#214113=CARTESIAN_POINT('Ctrl Pts',(-129.515183532897,6.07084337821547,
132.104444654172));
#214114=CARTESIAN_POINT('Ctrl Pts',(-129.793631156709,4.37523665480886,
126.399515326358));
#214115=CARTESIAN_POINT('Ctrl Pts',(-130.072078780522,-1.34099881217456,
124.742423632508));
#214116=CARTESIAN_POINT('Ctrl Pts',(-130.350526404335,-5.82492188220296,
128.655955885842));
#214117=CARTESIAN_POINT('Ctrl Pts',(-130.628974028148,-4.95602630574081,
134.543767132223));
#214118=CARTESIAN_POINT('Ctrl Pts',(-130.907421651961,0.467215330352083,
136.995246471799));
#214119=CARTESIAN_POINT('Ctrl Pts',(-131.185869275774,5.46110890258918,
133.757604152921));
#214120=CARTESIAN_POINT('Ctrl Pts',(-131.464316899587,5.43651018334856,
127.80607529902));
#214121=CARTESIAN_POINT('Ctrl Pts',(-131.742764523399,0.416024193898128,
124.60982417848));
#214122=CARTESIAN_POINT('Ctrl Pts',(-132.021212147213,-4.98676770583297,
127.106049425532));
#214123=CARTESIAN_POINT('Ctrl Pts',(-132.299659771025,-5.80696370104951,
133.000841985516));
#214124=CARTESIAN_POINT('Ctrl Pts',(-132.578107394838,-1.2908437409496,
136.877175472434));
#214125=CARTESIAN_POINT('Ctrl Pts',(-132.856555018651,4.41149855586104,
135.172888781227));
#214126=CARTESIAN_POINT('Ctrl Pts',(-133.135002642464,6.05988919352027,
129.454138122079));
#214127=CARTESIAN_POINT('Ctrl Pts',(-133.413450266277,2.13953770437982,
124.976175974248));
#214128=CARTESIAN_POINT('Ctrl Pts',(-133.69189789009,-3.74694441285829,
125.854030790976));
#214129=CARTESIAN_POINT('Ctrl Pts',(-133.970345513903,-6.19016766309031,
131.280996881284));
#214130=CARTESIAN_POINT('Ctrl Pts',(-134.248793137716,-2.94492923744478,
136.269957530209));
#214131=CARTESIAN_POINT('Ctrl Pts',(-134.527240761528,3.00655528962129,
136.236301625668));
#214132=CARTESIAN_POINT('Ctrl Pts',(-134.805688385342,6.19516238391663,
131.210957299752));
#214133=CARTESIAN_POINT('Ctrl Pts',(-135.084136009154,3.69071789790064,
125.811970486258));
#214134=CARTESIAN_POINT('Ctrl Pts',(-135.362583632967,-2.2053160346932,
125.000746311619));
#214135=CARTESIAN_POINT('Ctrl Pts',(-135.64103125678,-6.07477226708194,
129.522760161825));
#214136=CARTESIAN_POINT('Ctrl Pts',(-135.919478880593,-4.36180955514542,
135.222502221193));
#214137=CARTESIAN_POINT('Ctrl Pts',(-136.197926504406,1.35944305172635,
136.862187985044));
#214138=CARTESIAN_POINT('Ctrl Pts',(-136.476374128219,5.83143390654715,
132.935026339502));
#214139=CARTESIAN_POINT('Ctrl Pts',(-136.754821752032,4.9446218826347,127.049886984307));
#214140=CARTESIAN_POINT('Ctrl Pts',(-137.033269375845,-0.486056093210629,
124.614925481843));
#214141=CARTESIAN_POINT('Ctrl Pts',(-137.311716999657,-5.47007226455594,
127.867752498391));
#214142=CARTESIAN_POINT('Ctrl Pts',(-137.59016462347,-5.42735925266033,
133.819178915179));
#214143=CARTESIAN_POINT('Ctrl Pts',(-137.868612247283,-0.397168228809268,
137.000134598521));
#214144=CARTESIAN_POINT('Ctrl Pts',(-138.147059871096,4.99800099457058,
134.487476673751));
#214145=CARTESIAN_POINT('Ctrl Pts',(-138.425507494909,5.80025146986304,
128.590215023569));
#214146=CARTESIAN_POINT('Ctrl Pts',(-138.703955118722,1.27235420238826,
124.727645007244));
#214147=CARTESIAN_POINT('Ctrl Pts',(-138.982402742535,-4.42477441912264,
126.449279772744));
#214148=CARTESIAN_POINT('Ctrl Pts',(-139.260850366348,-6.05575151170779,
132.173021077107));
#214149=CARTESIAN_POINT('Ctrl Pts',(-139.539297990161,-2.12178880494131,
136.639030281933));
#214150=CARTESIAN_POINT('Ctrl Pts',(-139.817745613973,3.76199415842019,
135.743263104665));
#214151=CARTESIAN_POINT('Ctrl Pts',(-140.096193237787,6.18868827382574,
130.308885820552));
#214152=CARTESIAN_POINT('Ctrl Pts',(-140.374640861599,2.92828019981485,
125.329825669606));
#214153=CARTESIAN_POINT('Ctrl Pts',(-140.653088485412,-3.02307432338508,
125.381595689934));
#214154=CARTESIAN_POINT('Ctrl Pts',(-140.931536109225,-6.19637122878504,
130.416621761961));
#214155=CARTESIAN_POINT('Ctrl Pts',(-141.209983733038,-3.675505684495,135.807960900193));
#214156=CARTESIAN_POINT('Ctrl Pts',(-141.488431356851,2.22297002541115,
136.601235818153));
#214157=CARTESIAN_POINT('Ctrl Pts',(-141.766878980664,6.07864488008735,
132.06746561987));
#214158=CARTESIAN_POINT('Ctrl Pts',(-142.045326604476,4.34834204827492,
126.372963630579));
#214159=CARTESIAN_POINT('Ctrl Pts',(-142.32377422829,-1.3778746975837,124.750698986551));
#214160=CARTESIAN_POINT('Ctrl Pts',(-142.602221852102,-5.83789190928377,
128.691453643612));
#214161=CARTESIAN_POINT('Ctrl Pts',(-142.880669475915,-4.93317165322728,
134.573866588494));
#214162=CARTESIAN_POINT('Ctrl Pts',(-143.159117099728,0.504892353312588,
136.992287696695));
#214163=CARTESIAN_POINT('Ctrl Pts',(-143.437564723541,5.47898495252035,
133.72430611622));
#214164=CARTESIAN_POINT('Ctrl Pts',(-143.716012347354,5.4181580436573,127.77303726975));
#214165=CARTESIAN_POINT('Ctrl Pts',(-143.994459971167,0.378308584408798,
124.607406491544));
#214166=CARTESIAN_POINT('Ctrl Pts',(-144.27290759498,-5.00918798250961,
127.136473817112));
#214167=CARTESIAN_POINT('Ctrl Pts',(-144.551355218793,-5.79348550593904,
133.036149926065));
#214168=CARTESIAN_POINT('Ctrl Pts',(-144.829802842605,-1.2538528769121,
136.884920689477));
#214169=CARTESIAN_POINT('Ctrl Pts',(-145.108250466418,4.43800929187927,
135.145953798675));
#214170=CARTESIAN_POINT('Ctrl Pts',(-145.386698090231,6.05155773023994,
129.417274873051));
#214171=CARTESIAN_POINT('Ctrl Pts',(-145.665145714044,2.10402024954095,
124.963259983731));
#214172=CARTESIAN_POINT('Ctrl Pts',(-145.943593337857,-3.77700905338292,
125.876931223274));
#214173=CARTESIAN_POINT('Ctrl Pts',(-146.22204096167,-6.18715155339789,
131.318669357863));
#214174=CARTESIAN_POINT('Ctrl Pts',(-146.500488585483,-2.9116040349975,
136.287782885497));
#214175=CARTESIAN_POINT('Ctrl Pts',(-146.778936209295,3.03956535180104,
136.217899228972));
#214176=CARTESIAN_POINT('Ctrl Pts',(-147.057383833109,6.19752267131684,
131.173238054629));
#214177=CARTESIAN_POINT('Ctrl Pts',(-147.335831456921,3.66025942170698,
125.789596536289));
#214178=CARTESIAN_POINT('Ctrl Pts',(-147.614279080735,-2.24060342283806,
125.014278223797));
#214179=CARTESIAN_POINT('Ctrl Pts',(-147.892726704547,-6.08246118135759,
129.559762769929));
#214180=CARTESIAN_POINT('Ctrl Pts',(-148.17117432836,-4.33483425895693,
135.248971936054));
#214181=CARTESIAN_POINT('Ctrl Pts',(-148.449621952173,1.39629357899829,
136.853800431821));
#214182=CARTESIAN_POINT('Ctrl Pts',(-148.728069575986,5.84429583058792,
132.899489269852));
#214183=CARTESIAN_POINT('Ctrl Pts',(-149.006517199799,4.9216757235908,127.019857229157));
#214184=CARTESIAN_POINT('Ctrl Pts',(-149.284964823612,-0.52372393616008,
124.617998919139));
#214185=CARTESIAN_POINT('Ctrl Pts',(-149.563412447425,-5.48784688391679,
127.901104789406));
#214186=CARTESIAN_POINT('Ctrl Pts',(-149.841860071237,-5.40890664157841,
133.852160933818));
#214187=CARTESIAN_POINT('Ctrl Pts',(-150.12030769505,-0.359445435409253,
137.002437480918));
#214188=CARTESIAN_POINT('Ctrl Pts',(-150.398755318863,5.02032856601553,
134.456984183485));
#214189=CARTESIAN_POINT('Ctrl Pts',(-150.677202942676,5.78666587195703,
128.554948269553));
#214190=CARTESIAN_POINT('Ctrl Pts',(-150.955650566489,1.23533993591347,
124.720012413542));
#214191=CARTESIAN_POINT('Ctrl Pts',(-151.234098190302,-4.45120305152329,
126.476295320094));
#214192=CARTESIAN_POINT('Ctrl Pts',(-151.512545814115,-6.0473078879686,
132.209858797279));
#214193=CARTESIAN_POINT('Ctrl Pts',(-151.790993437928,-2.08623220278462,
136.651838109709));
#214194=CARTESIAN_POINT('Ctrl Pts',(-152.069441061741,3.79198895864895,
135.720271272016));
#214195=CARTESIAN_POINT('Ctrl Pts',(-152.347888685554,6.18555751604382,
130.27122269847));
#214196=CARTESIAN_POINT('Ctrl Pts',(-152.626336309366,2.89490089747778,
125.312101827337));
#214197=CARTESIAN_POINT('Ctrl Pts',(-152.904783933179,-3.05602822209906,
125.400098472666));
#214198=CARTESIAN_POINT('Ctrl Pts',(-153.183231556992,-6.19861670084527,
130.454348016274));
#214199=CARTESIAN_POINT('Ctrl Pts',(-153.461679180805,-3.64497925077551,
135.830242041403));
#214200=CARTESIAN_POINT('Ctrl Pts',(-153.740126804618,2.25821606362131,
136.587596565983));
#214201=CARTESIAN_POINT('Ctrl Pts',(-154.018574428431,6.08622113553776,
132.030439780749));
#214202=CARTESIAN_POINT('Ctrl Pts',(-154.297022052244,4.32128631232727,
126.346576141847));
#214203=CARTESIAN_POINT('Ctrl Pts',(-154.575469676057,-1.41469952533967,
124.759198661251));
#214204=CARTESIAN_POINT('Ctrl Pts',(-154.85391729987,-5.85064561113321,
128.727029695929));
#214205=CARTESIAN_POINT('Ctrl Pts',(-155.132364923682,-4.9101342002235,
134.603826364333));
#214206=CARTESIAN_POINT('Ctrl Pts',(-155.410812547495,0.542550667301237,
136.989099625678));
#214207=CARTESIAN_POINT('Ctrl Pts',(-155.689260171308,5.49665797664923,
133.690899879866));
#214208=CARTESIAN_POINT('Ctrl Pts',(-155.967707795121,5.39960513212718,
127.740111567281));
#214209=CARTESIAN_POINT('Ctrl Pts',(-156.246155418934,0.340578956555753,
124.605218435021));
#214210=CARTESIAN_POINT('Ctrl Pts',(-156.524603042747,-5.03142264188343,
127.167034123586));
#214211=CARTESIAN_POINT('Ctrl Pts',(-156.80305066656,-5.77979263109261,
133.071375166841));
#214212=CARTESIAN_POINT('Ctrl Pts',(-157.081498290373,-1.21681555089514,
136.89244058913));
#214213=CARTESIAN_POINT('Ctrl Pts',(-157.359945914186,4.46435557583064,
135.118857936792));
#214214=CARTESIAN_POINT('Ctrl Pts',(-157.638393537999,6.04300202426259,
129.380463022997));
#214215=CARTESIAN_POINT('Ctrl Pts',(-157.916841161811,2.06842482945845,
124.950560437346));
#214216=CARTESIAN_POINT('Ctrl Pts',(-158.195288785624,-3.80693373544809,
125.900014243279));
#214217=CARTESIAN_POINT('Ctrl Pts',(-158.473736409437,-6.18390617652933,
131.356322776543));
#214218=CARTESIAN_POINT('Ctrl Pts',(-158.75218403325,-2.87817094199197,
136.305405050556));
#214219=CARTESIAN_POINT('Ctrl Pts',(-159.030631657063,3.07246278176887,
136.199296231612));
#214220=CARTESIAN_POINT('Ctrl Pts',(-159.309079280876,6.19965330723533,
131.135505140616));
#214221=CARTESIAN_POINT('Ctrl Pts',(-159.587526904689,3.62966531325439,
125.767408410247));
#214222=CARTESIAN_POINT('Ctrl Pts',(-159.865974528502,-2.27580778459908,
125.028024689608));
#214223=CARTESIAN_POINT('Ctrl Pts',(-160.144422152314,-6.08992470779737,
129.596811497064));
#214224=CARTESIAN_POINT('Ctrl Pts',(-160.422869776128,-4.3076983338908,
135.275276954208));
#214225=CARTESIAN_POINT('Ctrl Pts',(-160.70131739994,1.43309236609815,136.845188714382));
#214226=CARTESIAN_POINT('Ctrl Pts',(-160.979765023753,5.85694119209746,
132.863874564441));
#214227=CARTESIAN_POINT('Ctrl Pts',(-161.258212647566,4.89854719004298,
126.989967710171));
#214228=CARTESIAN_POINT('Ctrl Pts',(-161.536660271379,-0.561372372326459,
124.621301594343));
#214229=CARTESIAN_POINT('Ctrl Pts',(-161.815107895192,-5.50541814909322,
127.934564661631));
#214230=CARTESIAN_POINT('Ctrl Pts',(-162.093555519005,-5.39025360147175,
133.885030015096));
#214231=CARTESIAN_POINT('Ctrl Pts',(-162.372003142818,-0.32170932262588,
137.004510691297));
#214232=CARTESIAN_POINT('Ctrl Pts',(-162.650450766631,5.04247010733932,
134.426356343909));
#214233=CARTESIAN_POINT('Ctrl Pts',(-162.928898390443,5.77286584701905,
128.519764868338));
#214234=CARTESIAN_POINT('Ctrl Pts',(-163.207346014257,1.19827989346308,
124.712605277602));
#214235=CARTESIAN_POINT('Ctrl Pts',(-163.485793638069,-4.47746674295796,
126.503471245498));
#214236=CARTESIAN_POINT('Ctrl Pts',(-163.764241261882,-6.03864017901171,
132.246644436198));
#214237=CARTESIAN_POINT('Ctrl Pts',(-164.042688885695,-2.05059829452646,
136.664429257056));
#214238=CARTESIAN_POINT('Ctrl Pts',(-164.321136509508,3.82184324533235,
135.697097278492));
#214239=CARTESIAN_POINT('Ctrl Pts',(-164.599584133321,6.18219755015336,
130.23357933201));
#214240=CARTESIAN_POINT('Ctrl Pts',(-164.878031757134,2.86141432352365,
125.294581502737));
#214241=CARTESIAN_POINT('Ctrl Pts',(-165.156479380946,-3.08886887856293,
125.418801512319));
#214242=CARTESIAN_POINT('Ctrl Pts',(-165.43492700476,-6.20063248088431,
130.492087240433));
#214243=CARTESIAN_POINT('Ctrl Pts',(-165.713374628572,-3.61431775100944,
135.85233694673));
#214244=CARTESIAN_POINT('Ctrl Pts',(-165.991822252385,2.2933784228048,136.573743013877));
#214245=CARTESIAN_POINT('Ctrl Pts',(-166.270269876198,6.09357186382579,
131.993368508814));
#214246=CARTESIAN_POINT('Ctrl Pts',(-166.548717500011,4.2940704495262,126.320353837957));
#214247=CARTESIAN_POINT('Ctrl Pts',(-166.827165123824,-1.45147193088449,
124.767922341652));
#214248=CARTESIAN_POINT('Ctrl Pts',(-167.105612747637,-5.86318251515793,
128.762682724506));
#214249=CARTESIAN_POINT('Ctrl Pts',(-167.38406037145,-4.88691480039125,
134.633645349573));
#214250=CARTESIAN_POINT('Ctrl Pts',(-167.662507995262,0.580188876875391,
136.985682376883));
#214251=CARTESIAN_POINT('Ctrl Pts',(-167.940955619076,5.51412732009539,
133.657386681736));
#214252=CARTESIAN_POINT('Ctrl Pts',(-168.219403242888,5.38085213624319,
127.707299411689));
#214253=CARTESIAN_POINT('Ctrl Pts',(-168.497850866701,0.302836708424229,
124.60326008999));
#214254=CARTESIAN_POINT('Ctrl Pts',(-168.776298490514,-5.05347086004094,
127.197729212531));
#214255=CARTESIAN_POINT('Ctrl Pts',(-169.054746114327,-5.7658855839047,
133.106516402559));
#214256=CARTESIAN_POINT('Ctrl Pts',(-169.33319373814,-1.17973313533045,
136.899734892741));
#214257=CARTESIAN_POINT('Ctrl Pts',(-169.611641361953,4.49053643144484,
135.091602199623));
#214258=CARTESIAN_POINT('Ctrl Pts',(-169.890088985766,6.03422239262278,
129.34370393599));
#214259=CARTESIAN_POINT('Ctrl Pts',(-170.168536609579,2.03275276313275,
124.938077805679));
#214260=CARTESIAN_POINT('Ctrl Pts',(-170.446984233392,-3.83671735018369,
125.923278995643));
#214261=CARTESIAN_POINT('Ctrl Pts',(-170.725431857205,-6.18043165274327,
131.393955742061));
#214262=CARTESIAN_POINT('Ctrl Pts',(-171.003879481017,-2.84463119730373,
136.32282337239));
#214263=CARTESIAN_POINT('Ctrl Pts',(-171.282327104831,3.10524636049842,
136.180493322929));
#214264=CARTESIAN_POINT('Ctrl Pts',(-171.560774728643,6.20155421272058,
131.097759955922));
#214265=CARTESIAN_POINT('Ctrl Pts',(-171.839222352457,3.59893670621881,
125.745406930321));
#214266=CARTESIAN_POINT('Ctrl Pts',(-172.117669976268,-2.31092781546573,
125.04198519967));
#214267=CARTESIAN_POINT('Ctrl Pts',(-172.396117600082,-6.09716256983718,
129.633904970377));
#214268=CARTESIAN_POINT('Ctrl Pts',(-172.674565223895,-4.2804027854792,
135.301416300912));
#214269=CARTESIAN_POINT('Ctrl Pts',(-172.953012847708,1.469838049433,136.836353151837));
#214270=CARTESIAN_POINT('Ctrl Pts',(-173.23146047152,5.86936952249723,132.828183542982));
#214271=CARTESIAN_POINT('Ctrl Pts',(-173.509908095334,4.8752371390276,126.960219534917));
#214272=CARTESIAN_POINT('Ctrl Pts',(-173.788355719146,-0.599000006633149,
124.624833385073));
#214273=CARTESIAN_POINT('Ctrl Pts',(-174.06680334296,-5.5227854089755,127.968130875202));
#214274=CARTESIAN_POINT('Ctrl Pts',(-174.345250966772,-5.37140082353563,
133.917784941036));
#214275=CARTESIAN_POINT('Ctrl Pts',(-174.623698590585,-0.283961288785237,
137.006354152836));
#214276=CARTESIAN_POINT('Ctrl Pts',(-174.902146214398,5.06442479807889,
134.39559428995));
#214277=CARTESIAN_POINT('Ctrl Pts',(-175.18059383821,5.75885190641417,128.484666123661));
#214278=CARTESIAN_POINT('Ctrl Pts',(-175.459041462024,1.16117544831056,
124.705423873895));
#214279=CARTESIAN_POINT('Ctrl Pts',(-175.737489085836,-4.50356452021585,
126.530806541938));
#214280=CARTESIAN_POINT('Ctrl Pts',(-176.01593670965,-6.02974870602229,
132.28337663076));
#214281=CARTESIAN_POINT('Ctrl Pts',(-176.294384333462,-2.01488840059438,
136.676803257405));
#214282=CARTESIAN_POINT('Ctrl Pts',(-176.572831957276,3.85155591220881,
135.67374198281));
#214283=CARTESIAN_POINT('Ctrl Pts',(-176.851279581088,6.17860850065921,
130.195957116059));
#214284=CARTESIAN_POINT('Ctrl Pts',(-177.129727204901,2.82782171880919,
125.277265345029));
#214285=CARTESIAN_POINT('Ctrl Pts',(-177.408174828714,-3.12159507585506,
125.437704115845));
#214286=CARTESIAN_POINT('Ctrl Pts',(-177.686622452527,-6.20241849420629,
130.529838035997));
#214287=CARTESIAN_POINT('Ctrl Pts',(-177.965070076339,-3.58352232136993,
135.874244797437));
#214288=CARTESIAN_POINT('Ctrl Pts',(-178.243517700153,2.32845580000743,
136.559675675186));
#214289=CARTESIAN_POINT('Ctrl Pts',(-178.521965323965,6.10069679256748,
131.956253177754));
#214290=CARTESIAN_POINT('Ctrl Pts',(-178.800412947778,4.26669546836545,
126.294297690589));
#214291=CARTESIAN_POINT('Ctrl Pts',(-179.078860571591,-1.48819055160311,
124.776869704492));
#214292=CARTESIAN_POINT('Ctrl Pts',(-179.357308195404,-5.8755021567984,
128.798411408209));
#214293=CARTESIAN_POINT('Ctrl Pts',(-179.635755819217,-4.86351431413387,
134.663322439258));
#214294=CARTESIAN_POINT('Ctrl Pts',(-179.91420344303,0.617805587336893,
136.982036076937));
#214295=CARTESIAN_POINT('Ctrl Pts',(-180.192651066843,5.53139233552561,
133.623767763677));
#214296=CARTESIAN_POINT('Ctrl Pts',(-180.471098690656,5.36189975090491,
127.674602018838));
#214297=CARTESIAN_POINT('Ctrl Pts',(-180.749546314469,0.265083238567079,
124.601531529021));
#214298=CARTESIAN_POINT('Ctrl Pts',(-181.027993938281,-5.07533181997731,
127.22855794653));
#214299=CARTESIAN_POINT('Ctrl Pts',(-181.306441562095,-5.75176487970607,
133.141572331048));
#214300=CARTESIAN_POINT('Ctrl Pts',(-181.584889185907,-1.14260700432061,
136.906803330016));
#214301=CARTESIAN_POINT('Ctrl Pts',(-181.86333680972,4.5165508885802,135.064187597142));
#214302=CARTESIAN_POINT('Ctrl Pts',(-182.141784433533,6.02521916065313,
129.306998974155));
#214303=CARTESIAN_POINT('Ctrl Pts',(-182.420232057346,1.99700537240587,
124.925812551278));
#214304=CARTESIAN_POINT('Ctrl Pts',(-182.698679681159,-3.86635879394691,
125.946724618282));
#214305=CARTESIAN_POINT('Ctrl Pts',(-182.977127304972,-6.17672811078948,
131.431566859916));
#214306=CARTESIAN_POINT('Ctrl Pts',(-183.255574928785,-2.81098604376035,
136.340037205557));
#214307=CARTESIAN_POINT('Ctrl Pts',(-183.534022552597,3.13791487318212,
136.161491199671));
#214308=CARTESIAN_POINT('Ctrl Pts',(-183.81247017641,6.20322531733387,131.060003899207));
#214309=CARTESIAN_POINT('Ctrl Pts',(-184.090917800223,3.56807473926006,
125.723592911784));
#214310=CARTESIAN_POINT('Ctrl Pts',(-184.369365424036,-2.34596221405232,
125.056159236672));
#214311=CARTESIAN_POINT('Ctrl Pts',(-184.647813047849,-6.10417449927606,
129.671041815353));
#214312=CARTESIAN_POINT('Ctrl Pts',(-184.926260671662,-4.25294862516783,
135.327389007565));
#214313=CARTESIAN_POINT('Ctrl Pts',(-185.204708295475,1.50652926737877,
136.827294071589));
#214314=CARTESIAN_POINT('Ctrl Pts',(-185.483155919288,5.88158036125089,
132.792417528021));
#214315=CARTESIAN_POINT('Ctrl Pts',(-185.761603543101,4.85174643430717,
126.930613805724));
#214316=CARTESIAN_POINT('Ctrl Pts',(-186.040051166913,-0.6366054447743,
124.628594160457));
#214317=CARTESIAN_POINT('Ctrl Pts',(-186.318498790727,-5.53994802001346,
128.001802186308));
#214318=CARTESIAN_POINT('Ctrl Pts',(-186.596946414539,-5.35234900636664,
133.950424497894));
#214319=CARTESIAN_POINT('Ctrl Pts',(-186.875394038353,-0.246202732654624,
137.007967797222));
#214320=CARTESIAN_POINT('Ctrl Pts',(-187.153841662165,5.08619182469514,
134.364699161505));
#214321=CARTESIAN_POINT('Ctrl Pts',(-187.432289285978,5.744624569434,128.449653336115));
#214322=CARTESIAN_POINT('Ctrl Pts',(-187.71073690979,1.12402797537536,124.698468468532));
#214323=CARTESIAN_POINT('Ctrl Pts',(-187.989184533604,-4.52949541623416,
126.558300196495));
#214324=CARTESIAN_POINT('Ctrl Pts',(-188.267632157416,-6.0206337984771,
132.32005401984));
#214325=CARTESIAN_POINT('Ctrl Pts',(-188.54607978123,-1.97910384423165,
136.688959652232));
#214326=CARTESIAN_POINT('Ctrl Pts',(-188.824527405043,3.88112585826452,
135.650206250412));
#214327=CARTESIAN_POINT('Ctrl Pts',(-189.102975028855,6.17479050055486,
130.158357444724));
#214328=CARTESIAN_POINT('Ctrl Pts',(-189.381422652668,2.79412432812102,
125.260153995869));
#214329=CARTESIAN_POINT('Ctrl Pts',(-189.659870276481,-3.15420560129371,
125.456805582802));
#214330=CARTESIAN_POINT('Ctrl Pts',(-189.938317900294,-6.20397467462999,
130.567599004095));
#214331=CARTESIAN_POINT('Ctrl Pts',(-190.216765524107,-3.55259410299321,
135.89596478172));
#214332=CARTESIAN_POINT('Ctrl Pts',(-190.49521314792,2.36344689542356,136.545395071179));
#214333=CARTESIAN_POINT('Ctrl Pts',(-190.773660771733,6.10759565774615,
131.919095162891));
#214334=CARTESIAN_POINT('Ctrl Pts',(-191.052108395545,4.23916238323504,
126.26840866526));
#214335=CARTESIAN_POINT('Ctrl Pts',(-191.330556019359,-1.52485402687357,
124.786040418225));
#214336=CARTESIAN_POINT('Ctrl Pts',(-191.609003643171,-5.88760407954571,
128.834214423098));
#214337=CARTESIAN_POINT('Ctrl Pts',(-191.887451266984,-4.83993360856504,
134.692856533694));
#214338=CARTESIAN_POINT('Ctrl Pts',(-192.165898890797,0.655399404785621,
136.978160860955));
#214339=CARTESIAN_POINT('Ctrl Pts',(-192.44434651461,5.54845238317892,133.59004437145));
#214340=CARTESIAN_POINT('Ctrl Pts',(-192.722794138423,5.34274867839911,
127.642020600343));
#214341=CARTESIAN_POINT('Ctrl Pts',(-193.001241762236,0.227319945953055,
124.600032816164));
#214342=CARTESIAN_POINT('Ctrl Pts',(-193.279689386049,-5.09700471162664,
127.259519183211));
#214343=CARTESIAN_POINT('Ctrl Pts',(-193.558137009861,-5.73743104174462,
133.176541653297));
#214344=CARTESIAN_POINT('Ctrl Pts',(-193.836584633675,-1.105438533588,136.913645639033));
#214345=CARTESIAN_POINT('Ctrl Pts',(-194.115032257487,4.5423979832614,135.036615145204));
#214346=CARTESIAN_POINT('Ctrl Pts',(-194.3934798813,6.01599266197172,129.270349497605));
#214347=CARTESIAN_POINT('Ctrl Pts',(-194.671927505113,1.96118398191049,
124.913765128639));
#214348=CARTESIAN_POINT('Ctrl Pts',(-194.950375128926,-3.89585696836267,
125.970350242409));
#214349=CARTESIAN_POINT('Ctrl Pts',(-195.228822752739,-6.17279568790409,
131.469154736412));
#214350=CARTESIAN_POINT('Ctrl Pts',(-195.507270376552,-2.77723672809589,
136.357045912194));
#214351=CARTESIAN_POINT('Ctrl Pts',(-195.785718000365,3.17046710927626,
136.142290565968));
#214352=CARTESIAN_POINT('Ctrl Pts',(-196.064165624178,6.20466655915177,
131.022238369536));
#214353=CARTESIAN_POINT('Ctrl Pts',(-196.342613247991,3.5370805559797,125.701967162963));
#214354=CARTESIAN_POINT('Ctrl Pts',(-196.621060871803,-2.38090968214636,
125.070546275391));
#214355=CARTESIAN_POINT('Ctrl Pts',(-196.899508495616,-6.11096023628406,
129.708220655875));
#214356=CARTESIAN_POINT('Ctrl Pts',(-197.177956119429,-4.22533687028115,
135.353194111738));
#214357=CARTESIAN_POINT('Ctrl Pts',(-197.456403743242,1.54316466032852,
136.818011809327));
#214358=CARTESIAN_POINT('Ctrl Pts',(-197.734851367055,5.89357325588093,
132.75657784488));
#214359=CARTESIAN_POINT('Ctrl Pts',(-198.013298990868,4.82807594633875,
126.901151619645));
#214360=CARTESIAN_POINT('Ctrl Pts',(-198.291746614681,-0.674187293266194,
124.632583781138));
#214361=CARTESIAN_POINT('Ctrl Pts',(-198.570194238494,-5.55690534624021,
128.035577347248));
#214362=CARTESIAN_POINT('Ctrl Pts',(-198.848641862306,-5.33309885593691,
133.982947476197));
#214363=CARTESIAN_POINT('Ctrl Pts',(-199.12708948612,-0.2084350533912,137.009351564664));
#214364=CARTESIAN_POINT('Ctrl Pts',(-199.405537109932,5.10777038060287,
134.333672103408));
#214365=CARTESIAN_POINT('Ctrl Pts',(-199.683984733745,5.7301843632779,128.414727803113));
#214366=CARTESIAN_POINT('Ctrl Pts',(-199.962432357558,1.08683885116959,
124.691739319248));
#214367=CARTESIAN_POINT('Ctrl Pts',(-200.240879981371,-4.5552584701342,
126.585951190383));
#214368=CARTESIAN_POINT('Ctrl Pts',(-200.519327605184,-6.01129579413245,
132.356675244344));
#214369=CARTESIAN_POINT('Ctrl Pts',(-200.797775228997,-1.94324595144814,
136.700897991079));
#214370=CARTESIAN_POINT('Ctrl Pts',(-201.076222852809,3.91055198777426,
135.626490953421));
#214371=CARTESIAN_POINT('Ctrl Pts',(-201.354670476623,6.17074369131775,
130.120781711275));
#214372=CARTESIAN_POINT('Ctrl Pts',(-201.633118100435,2.76032340012831,
125.243248089324));
#214373=CARTESIAN_POINT('Ctrl Pts',(-201.911565724248,-3.18669924648382,
125.476105205376));
#214374=CARTESIAN_POINT('Ctrl Pts',(-202.190013348061,-6.20530096449064,
130.605368745483));
#214375=CARTESIAN_POINT('Ctrl Pts',(-202.468460971874,-3.52153424193529,
135.91749609474));
#214376=CARTESIAN_POINT('Ctrl Pts',(-202.746908595687,2.39835041244635,
136.530901731028));
#214377=CARTESIAN_POINT('Ctrl Pts',(-203.0253562195,6.11426820372151,131.881895841131));
#214378=CARTESIAN_POINT('Ctrl Pts',(-203.303803843313,4.21147221438356,
126.242687721299));
#214379=CARTESIAN_POINT('Ctrl Pts',(-203.582251467125,-1.56146099811728,
124.795434143027));
#214380=CARTESIAN_POINT('Ctrl Pts',(-203.860699090939,-5.89948783495869,
128.870090442477));
#214381=CARTESIAN_POINT('Ctrl Pts',(-204.139146714752,-4.81617355747646,
134.722246538484));
#214382=CARTESIAN_POINT('Ctrl Pts',(-204.417594338564,0.69296893616836,
136.974056872534));
#214383=CARTESIAN_POINT('Ctrl Pts',(-204.696041962377,5.56530683088876,
133.556217754686));
#214384=CARTESIAN_POINT('Ctrl Pts',(-204.97448958619,5.32339962837619,127.60955636352));
#214385=CARTESIAN_POINT('Ctrl Pts',(-205.252937210003,0.18954822991528,
124.598764006957));
#214386=CARTESIAN_POINT('Ctrl Pts',(-205.531384833816,-5.11848873189165,
127.290611775294));
#214387=CARTESIAN_POINT('Ctrl Pts',(-205.809832457629,-5.72288460116635,
133.211423073505));
#214388=CARTESIAN_POINT('Ctrl Pts',(-206.088280081441,-1.06822910042401,
136.920261566246));
#214389=CARTESIAN_POINT('Ctrl Pts',(-206.366727705255,4.56807675771487,
135.00888586552));
#214390=CARTESIAN_POINT('Ctrl Pts',(-206.645175329067,6.00654323846982,
129.233756864401));
#214391=CARTESIAN_POINT('Ctrl Pts',(-206.92362295288,1.92528991902147,124.901935984182));
#214392=CARTESIAN_POINT('Ctrl Pts',(-207.202070576693,-3.92521078036628,
125.994154992568));
#214393=CARTESIAN_POINT('Ctrl Pts',(-207.480518200506,-6.16863452980439,
131.506717978718));
#214394=CARTESIAN_POINT('Ctrl Pts',(-207.758965824319,-2.74338450090264,
136.373848862034));
#214395=CARTESIAN_POINT('Ctrl Pts',(-208.037413448132,3.20290186254569,
136.12289213331));
#214396=CARTESIAN_POINT('Ctrl Pts',(-208.315861071945,6.20587788476857,
130.984464766326));
#214397=CARTESIAN_POINT('Ctrl Pts',(-208.594308695758,3.50595530487857,
125.680530485208));
#214398=CARTESIAN_POINT('Ctrl Pts',(-208.872756319571,-2.41576892475653,
125.085145782709));
#214399=CARTESIAN_POINT('Ctrl Pts',(-209.151203943383,-6.11751952941318,
129.745440114266));
#214400=CARTESIAN_POINT('Ctrl Pts',(-209.429651567197,-4.19756854398286,
135.378830657213));
#214401=CARTESIAN_POINT('Ctrl Pts',(-209.708099191009,1.57974287074426,
136.808506709009));
#214402=CARTESIAN_POINT('Ctrl Pts',(-209.986546814822,5.90534776198698,
132.720665821612));
#214403=CARTESIAN_POINT('Ctrl Pts',(-210.264994438635,4.80422655224024,
126.87183406841));
#214404=CARTESIAN_POINT('Ctrl Pts',(-210.543442062448,-0.711744159500396,
124.63680209928));
#214405=CARTESIAN_POINT('Ctrl Pts',(-210.821889686261,-5.57365675929581,
128.06945510647));
#214406=CARTESIAN_POINT('Ctrl Pts',(-211.100337310074,-5.31365108556781,
134.015352670796));
#214407=CARTESIAN_POINT('Ctrl Pts',(-211.378784933887,-0.170659650490228,
137.010505403884));
#214408=CARTESIAN_POINT('Ctrl Pts',(-211.657232557699,5.12915966620077,
134.302514265376));
#214409=CARTESIAN_POINT('Ctrl Pts',(-211.935680181513,5.71553182303293,
128.379890818834));
#214410=CARTESIAN_POINT('Ctrl Pts',(-212.214127805325,1.04960945375051,
124.685236675394));
#214411=CARTESIAN_POINT('Ctrl Pts',(-212.492575429138,-4.58085272725645,
126.613758498985));
#214412=CARTESIAN_POINT('Ctrl Pts',(-212.771023052951,-6.00173503901134,
132.393238947258));
#214413=CARTESIAN_POINT('Ctrl Pts',(-213.049470676764,-1.90731605097184,
136.712617831564));
#214414=CARTESIAN_POINT('Ctrl Pts',(-213.327918300577,3.93983321034183,
135.602596970618));
#214415=CARTESIAN_POINT('Ctrl Pts',(-213.60636592439,6.16646822290386,130.083231308093));
#214416=CARTESIAN_POINT('Ctrl Pts',(-213.884813548203,2.72642018733693,
125.226548251849));
#214417=CARTESIAN_POINT('Ctrl Pts',(-214.163261172015,-3.21907480736146,
125.495602268416));
#214418=CARTESIAN_POINT('Ctrl Pts',(-214.441708795829,-6.20639731464204,
130.643145860587));
#214419=CARTESIAN_POINT('Ctrl Pts',(-214.720156419641,-3.49034388913101,
135.938837938644));
#214420=CARTESIAN_POINT('Ctrl Pts',(-214.998604043455,2.43316505771265,
136.516196191791));
#214421=CARTESIAN_POINT('Ctrl Pts',(-215.277051667267,6.12071418324004,
131.844656590906));
#214422=CARTESIAN_POINT('Ctrl Pts',(-215.55549929108,4.18362598788043,126.217135811804));
#214423=CARTESIAN_POINT('Ctrl Pts',(-215.833946914893,-1.59801010884951,
124.805050530808));
#214424=CARTESIAN_POINT('Ctrl Pts',(-216.112394538706,-5.91115298268039,
128.90603813695));
#214425=CARTESIAN_POINT('Ctrl Pts',(-216.390842162519,-4.79223504130557,
134.75149136457));
#214426=CARTESIAN_POINT('Ctrl Pts',(-216.669289786332,0.730512789332353,
136.969724263749));
#214427=CARTESIAN_POINT('Ctrl Pts',(-216.947737410145,5.5819550541073,133.522289166845));
#214428=CARTESIAN_POINT('Ctrl Pts',(-217.226185033957,5.3038533178224,127.577210511344));
#214429=CARTESIAN_POINT('Ctrl Pts',(-217.50463265777,0.151769490097695,
124.597725148413));
#214430=CARTESIAN_POINT('Ctrl Pts',(-217.783080281583,-5.13978308467467,
127.321834570635));
#214431=CARTESIAN_POINT('Ctrl Pts',(-218.061527905396,-5.70812609699421,
133.24621529913));
#214432=CARTESIAN_POINT('Ctrl Pts',(-218.339975529209,-1.03098008363786,
136.9266508665));
#214433=CARTESIAN_POINT('Ctrl Pts',(-218.618423153022,4.59358626040416,
134.981000785606));
#214434=CARTESIAN_POINT('Ctrl Pts',(-218.896870776835,5.99687124029931,
129.197222430498));
#214435=CARTESIAN_POINT('Ctrl Pts',(-219.175318400648,1.88932451380644,
124.890325556239));
#214436=CARTESIAN_POINT('Ctrl Pts',(-219.45376602446,-3.95441914224089,
126.018137986666));
#214437=CARTESIAN_POINT('Ctrl Pts',(-219.732213648274,-6.16424479068368,
131.544255194914));
#214438=CARTESIAN_POINT('Ctrl Pts',(-220.010661272086,-2.70943061658779,
136.390445432439));
#214439=CARTESIAN_POINT('Ctrl Pts',(-220.289108895899,3.23521793110825,
136.103296620509));
#214440=CARTESIAN_POINT('Ctrl Pts',(-220.567556519712,6.20685924929812,
130.94668448929));
#214441=CARTESIAN_POINT('Ctrl Pts',(-220.846004143525,3.47470013931478,
125.659283672863));
#214442=CARTESIAN_POINT('Ctrl Pts',(-221.124451767337,-2.45053865016082,
125.099957217636));
#214443=CARTESIAN_POINT('Ctrl Pts',(-221.402899391151,-6.12385213560643,
129.782698811345));
#214444=CARTESIAN_POINT('Ctrl Pts',(-221.681347014963,-4.16964467523852,
135.404297694017));
#214445=CARTESIAN_POINT('Ctrl Pts',(-221.959794638777,1.61626254320698,
136.79877912285));
#214446=CARTESIAN_POINT('Ctrl Pts',(-222.238242262589,5.91690344326002,
132.684682788949));
#214447=CARTESIAN_POINT('Ctrl Pts',(-222.516689886402,4.7801991357601,126.842662238393));
#214448=CARTESIAN_POINT('Ctrl Pts',(-222.795137510215,-0.749274651793031,
124.64124895857));
#214449=CARTESIAN_POINT('Ctrl Pts',(-223.073585134028,-5.59020163845046,
128.103434208622));
#214450=CARTESIAN_POINT('Ctrl Pts',(-223.352032757841,-5.29400641590365,
134.047638880903));
#214451=CARTESIAN_POINT('Ctrl Pts',(-223.630480381654,-0.132877923733138,
137.011429272127));
#214452=CARTESIAN_POINT('Ctrl Pts',(-223.908928005467,5.15035888890098,
134.271226801972));
#214453=CARTESIAN_POINT('Ctrl Pts',(-224.187375629279,5.70066749165438,
128.345143674176));
#214454=CARTESIAN_POINT('Ctrl Pts',(-224.465823253093,1.01234116266713,
124.678960777928));
#214455=CARTESIAN_POINT('Ctrl Pts',(-224.744270876905,-4.60627723919628,
126.641721091889));
#214456=CARTESIAN_POINT('Ctrl Pts',(-225.022718500718,-5.99195188739136,
132.4297437737));
#214457=CARTESIAN_POINT('Ctrl Pts',(-225.301166124531,-1.87131547419729,
136.724118739406));
#214458=CARTESIAN_POINT('Ctrl Pts',(-225.579613748344,3.96896844094108,
135.578525187401));
#214459=CARTESIAN_POINT('Ctrl Pts',(-225.858061372157,6.16196425374224,
130.045707626623));
#214460=CARTESIAN_POINT('Ctrl Pts',(-226.13650899597,2.69241594604283,125.210055102262));
#214461=CARTESIAN_POINT('Ctrl Pts',(-226.414956619783,-3.25133108423828,
125.515296049447));
#214462=CARTESIAN_POINT('Ctrl Pts',(-226.693404243596,-6.20726368445854,
130.680928949564));
#214463=CARTESIAN_POINT('Ctrl Pts',(-226.971851867408,-3.45902420035033,
135.959989522602));
#214464=CARTESIAN_POINT('Ctrl Pts',(-227.250299491222,2.46788954115291,
136.501278998386));
#214465=CARTESIAN_POINT('Ctrl Pts',(-227.528747115034,6.12693335744362,
131.80737879213));
#214466=CARTESIAN_POINT('Ctrl Pts',(-227.807194738847,4.15562473557794,
126.191753883612));
#214467=CARTESIAN_POINT('Ctrl Pts',(-228.08564236266,-1.63450000472891,
124.81488922523));
#214468=CARTESIAN_POINT('Ctrl Pts',(-228.364089986473,-5.9225990904546,
128.942056174461));
#214469=CARTESIAN_POINT('Ctrl Pts',(-228.642537610286,-4.76811894710285,
134.780589928275));
#214470=CARTESIAN_POINT('Ctrl Pts',(-228.920985234099,0.768029573076269,
136.965163195147));
#214471=CARTESIAN_POINT('Ctrl Pts',(-229.199432857912,5.59839643592858,
133.48825986516));
#214472=CARTESIAN_POINT('Ctrl Pts',(-229.477880481725,5.28411047103341,
127.544984242401));
#214473=CARTESIAN_POINT('Ctrl Pts',(-229.756328105537,0.11398512640586,
124.59691627903));
#214474=CARTESIAN_POINT('Ctrl Pts',(-230.03477572935,-5.16088698090536,
127.353186412258));
#214475=CARTESIAN_POINT('Ctrl Pts',(-230.313223353163,-5.69315607611037,
133.280917040931));
#214476=CARTESIAN_POINT('Ctrl Pts',(-230.591670976976,-0.993692863505588,
136.932813303039));
#214477=CARTESIAN_POINT('Ctrl Pts',(-230.870118600789,4.6189255460653,134.952960938754));
#214478=CARTESIAN_POINT('Ctrl Pts',(-231.148566224602,5.98697702585963,
129.160747549691));
#214479=CARTESIAN_POINT('Ctrl Pts',(-231.427013848415,1.85328909897679,
124.878934275042));
#214480=CARTESIAN_POINT('Ctrl Pts',(-231.705461472227,-3.98348097165998,
126.042298336002));
#214481=CARTESIAN_POINT('Ctrl Pts',(-231.983909096041,-6.15962663320533,
131.581764994044));
#214482=CARTESIAN_POINT('Ctrl Pts',(-232.262356719853,-2.6753763333251,
136.406835008417));
#214483=CARTESIAN_POINT('Ctrl Pts',(-232.540804343666,3.26741411748112,
136.083504753687));
#214484=CARTESIAN_POINT('Ctrl Pts',(-232.819251967479,6.20761061637562,
130.90889893839));
#214485=CARTESIAN_POINT('Ctrl Pts',(-233.097699591292,3.44331621745904,
125.638227513236));
#214486=CARTESIAN_POINT('Ctrl Pts',(-233.376147215105,-2.48521756995422,
125.114980031328));
#214487=CARTESIAN_POINT('Ctrl Pts',(-233.654594838918,-6.12995782020675,
129.819995366479));
#214488=CARTESIAN_POINT('Ctrl Pts',(-233.933042462731,-4.14156629877734,
135.429594278462));
#214489=CARTESIAN_POINT('Ctrl Pts',(-234.211490086544,1.65272232446679,
136.788829411307));
#214490=CARTESIAN_POINT('Ctrl Pts',(-234.489937710357,5.92823987150001,
132.648630080257));
#214491=CARTESIAN_POINT('Ctrl Pts',(-234.768385334169,4.75599458724306,
126.813637210565));
#214492=CARTESIAN_POINT('Ctrl Pts',(-235.046832957982,-0.786777379437916,
124.64592419423));
#214493=CARTESIAN_POINT('Ctrl Pts',(-235.325280581795,-5.6065393706272,
128.137513394595));
#214494=CARTESIAN_POINT('Ctrl Pts',(-235.603728205608,-5.27416557488518,
134.079804910139));
#214495=CARTESIAN_POINT('Ctrl Pts',(-235.882175829421,-0.0950912731361558,
137.012123135159));
#214496=CARTESIAN_POINT('Ctrl Pts',(-236.160623453234,5.17136726315852,
134.239810872567));
#214497=CARTESIAN_POINT('Ctrl Pts',(-236.439071077047,5.68559191994549,
128.310487656705));
#214498=CARTESIAN_POINT('Ctrl Pts',(-236.71751870086,0.975035358909668,
124.672911859406));
#214499=CARTESIAN_POINT('Ctrl Pts',(-236.995966324673,-4.63153106383903,
126.669837932931));
#214500=CARTESIAN_POINT('Ctrl Pts',(-237.274413948486,-5.98194670179065,
132.466188370973));
#214501=CARTESIAN_POINT('Ctrl Pts',(-237.552861572298,-1.83524555513966,
136.735400288432));
#214502=CARTESIAN_POINT('Ctrl Pts',(-237.831309196112,3.99795659995517,
135.554276495761));
#214503=CARTESIAN_POINT('Ctrl Pts',(-238.109756819924,6.15723195072914,
130.008212057319));
#214504=CARTESIAN_POINT('Ctrl Pts',(-238.388204443737,2.65831193628575,
125.193769251723));
#214505=CARTESIAN_POINT('Ctrl Pts',(-238.66665206755,-3.28346688184612,
125.535185818711));
#214506=CARTESIAN_POINT('Ctrl Pts',(-238.945099691363,-6.20790004183648,
130.718716612347));
#214507=CARTESIAN_POINT('Ctrl Pts',(-239.223547315176,-3.42757633615586,
135.980950062836));
#214508=CARTESIAN_POINT('Ctrl Pts',(-239.501994938989,2.50252257603867,
136.486150703575));
#214509=CARTESIAN_POINT('Ctrl Pts',(-239.780442562802,6.13292549587844,
131.770063826148));
#214510=CARTESIAN_POINT('Ctrl Pts',(-240.058890186614,4.12746949507249,
126.166542877259));
#214511=CARTESIAN_POINT('Ctrl Pts',(-240.337337810428,-1.67092933361012,
124.824949861719));
#214512=CARTESIAN_POINT('Ctrl Pts',(-240.61578543424,-5.93382573414137,
128.978143220346));
#214513=CARTESIAN_POINT('Ctrl Pts',(-240.894233058053,-4.74382616849909,
134.80954115134));
#214514=CARTESIAN_POINT('Ctrl Pts',(-241.172680681866,0.805517897201924,
136.960373835741));
#214515=CARTESIAN_POINT('Ctrl Pts',(-241.451128305679,5.6146303671111,133.454131110603));
#214516=CARTESIAN_POINT('Ctrl Pts',(-241.729575929492,5.26417181958768,
127.512878750849));
#214517=CARTESIAN_POINT('Ctrl Pts',(-242.008023553305,0.0761965389532375,
124.596337428779));
#214518=CARTESIAN_POINT('Ctrl Pts',(-242.286471177117,-5.18179963857104,
127.384666138411));
#214519=CARTESIAN_POINT('Ctrl Pts',(-242.564918800931,-5.67797509323448,
133.315527013022));
#214520=CARTESIAN_POINT('Ctrl Pts',(-242.843366424743,-0.956368821719198,
136.938748647509));
#214521=CARTESIAN_POINT('Ctrl Pts',(-243.121814048556,4.64409367574132,
134.924767363992));
#214522=CARTESIAN_POINT('Ctrl Pts',(-243.400261672369,5.9768609617849,129.124333573571));
#214523=CARTESIAN_POINT('Ctrl Pts',(-243.678709296182,1.81718500983798,
124.867762562695));
#214524=CARTESIAN_POINT('Ctrl Pts',(-243.957156919995,-4.01239519172672,
126.066635145309));
#214525=CARTESIAN_POINT('Ctrl Pts',(-244.235604543808,-6.15478022849689,
131.619245986169));
#214526=CARTESIAN_POINT('Ctrl Pts',(-244.514052167621,-2.64122291300849,
136.423016982646));
#214527=CARTESIAN_POINT('Ctrl Pts',(-244.792499791433,3.29948922862226,
136.063517266237));
#214528=CARTESIAN_POINT('Ctrl Pts',(-245.070947415247,6.20813195815889,
130.871109513785));
#214529=CARTESIAN_POINT('Ctrl Pts',(-245.349395039059,3.41180470225455,
125.617362786572));
#214530=CARTESIAN_POINT('Ctrl Pts',(-245.627842662872,-2.51980439909662,
125.13021366711));
#214531=CARTESIAN_POINT('Ctrl Pts',(-245.906290286685,-6.13583635696575,
129.857328397629));
#214532=CARTESIAN_POINT('Ctrl Pts',(-246.184737910498,-4.1133344550539,
135.454719473173));
#214533=CARTESIAN_POINT('Ctrl Pts',(-246.463185534311,1.68912086349306,
136.778657943074));
#214534=CARTESIAN_POINT('Ctrl Pts',(-246.741633158124,5.93935662663147,
132.612509031482));
#214535=CARTESIAN_POINT('Ctrl Pts',(-247.020080781937,4.73161380359756,
126.784760060463));
#214536=CARTESIAN_POINT('Ctrl Pts',(-247.29852840575,-0.824250952757648,
124.650827633015));
#214537=CARTESIAN_POINT('Ctrl Pts',(-247.576976029562,-5.62266935042617,
128.171691401572));
#214538=CARTESIAN_POINT('Ctrl Pts',(-247.855423653376,-5.25412929772145,
134.111849566585));
#214539=CARTESIAN_POINT('Ctrl Pts',(-248.133871277188,-0.0573010988966442,
137.012586967267));
#214540=CARTESIAN_POINT('Ctrl Pts',(-248.412318901001,5.19218401050035,
134.208267641291));
#214541=CARTESIAN_POINT('Ctrl Pts',(-248.690766524814,5.67030566653712,
128.275924050614));
#214542=CARTESIAN_POINT('Ctrl Pts',(-248.969214148627,0.937693424858449,
124.667090143972));
#214543=CARTESIAN_POINT('Ctrl Pts',(-249.24766177244,-4.65661326539506,
126.698107980232));
#214544=CARTESIAN_POINT('Ctrl Pts',(-249.526109396252,-5.97171985295489,
132.502571388608));
#214545=CARTESIAN_POINT('Ctrl Pts',(-249.804557020066,-1.79910763038337,
136.746462060605));
#214546=CARTESIAN_POINT('Ctrl Pts',(-250.083004643878,4.02679661321771,
135.52985179424));
#214547=CARTESIAN_POINT('Ctrl Pts',(-250.361452267692,6.15227148922063,
129.970745989595));
#214548=CARTESIAN_POINT('Ctrl Pts',(-250.639899891504,2.62410942180459,
125.177691303707));
#214549=CARTESIAN_POINT('Ctrl Pts',(-250.918347515317,-3.31548100938434,
125.555270839195));
#214550=CARTESIAN_POINT('Ctrl Pts',(-251.19679513913,-6.20830636318893,
130.756507448682));
#214551=CARTESIAN_POINT('Ctrl Pts',(-251.475242762943,-3.39600146187203,
136.001718782677));
#214552=CARTESIAN_POINT('Ctrl Pts',(-251.753690386756,2.53706287905323,
136.47081186788));
#214553=CARTESIAN_POINT('Ctrl Pts',(-252.032138010569,6.13869037645988,
131.732713075798));
#214554=CARTESIAN_POINT('Ctrl Pts',(-252.310585634382,4.09916130974965,
126.141503726722));
#214555=CARTESIAN_POINT('Ctrl Pts',(-252.589033258195,-1.70729674574642,
124.835232067896));
#214556=CARTESIAN_POINT('Ctrl Pts',(-252.867480882007,-5.94483249743877,
129.014297936587));
#214557=CARTESIAN_POINT('Ctrl Pts',(-253.14592850582,-4.71935760622846,
134.838343962485));
#214558=CARTESIAN_POINT('Ctrl Pts',(-253.424376129633,0.842976373616159,
136.955356360136));
#214559=CARTESIAN_POINT('Ctrl Pts',(-253.702823753446,5.63065624411703,
133.419904173236));
#214560=CARTESIAN_POINT('Ctrl Pts',(-253.981271377259,5.24403810606461,
127.480895216153));
#214561=CARTESIAN_POINT('Ctrl Pts',(-254.259719001072,0.0384051209378723,
124.595988638398));
#214562=CARTESIAN_POINT('Ctrl Pts',(-254.538166624885,-5.20252026939218,
127.416272546179));
#214563=CARTESIAN_POINT('Ctrl Pts',(-254.816614248698,-5.66258373611722,
133.350044001689));
#214564=CARTESIAN_POINT('Ctrl Pts',(-255.095061872511,-0.919009293725241,
136.944456550123));
#214565=CARTESIAN_POINT('Ctrl Pts',(-255.373509496324,4.6690896269236,134.896421351226));
#214566=CARTESIAN_POINT('Ctrl Pts',(-255.651957120136,5.96652359266914,
129.087981388513));
#214567=CARTESIAN_POINT('Ctrl Pts',(-255.93040474395,1.78101326373629,124.856811707331));
#214568=CARTESIAN_POINT('Ctrl Pts',(-256.208852367762,-4.04116012583712,
126.091145862189));
#214569=CARTESIAN_POINT('Ctrl Pts',(-256.487299991575,-6.14970689884083,
131.656699899059));
#214570=CARTESIAN_POINT('Ctrl Pts',(-256.765747615388,-2.60696946356087,
136.438984870644));
#214571=CARTESIAN_POINT('Ctrl Pts',(-257.044195239201,3.33143800190474,
136.043346010603));
#214572=CARTESIAN_POINT('Ctrl Pts',(-257.322642863014,6.2084309480058,130.833296634437));
#214573=CARTESIAN_POINT('Ctrl Pts',(-257.601090486826,3.38015223603414,
125.596729883064));
#214574=CARTESIAN_POINT('Ctrl Pts',(-257.87953811064,-2.5542704291637,125.145582755354));
#214575=CARTESIAN_POINT('Ctrl Pts',(-258.157985734452,-6.14153931545366,
129.894837769574));
#214576=CARTESIAN_POINT('Ctrl Pts',(-258.436433358265,-4.08485240479644,
135.479405634932));
#214577=CARTESIAN_POINT('Ctrl Pts',(-258.714880982078,1.72527217059264,
136.768768758555));
#214578=CARTESIAN_POINT('Ctrl Pts',(-258.993328605892,5.95060195420752,
132.575369498931));
#214579=CARTESIAN_POINT('Ctrl Pts',(-259.271776229703,4.70639920604184,
126.75783223591));
#214580=CARTESIAN_POINT('Ctrl Pts',(-259.550223853517,-0.860449444711704,
124.652528659269));
#214581=CARTESIAN_POINT('Ctrl Pts',(-259.82867147733,-5.64095031490746,
128.212697490595));
#214582=CARTESIAN_POINT('Ctrl Pts',(-260.060711163841,-5.29799179572588,
133.142936715762));
#214583=CARTESIAN_POINT('Ctrl Pts',(-260.246372125917,-2.62679689981868,
135.594171577488));
#214584=CARTESIAN_POINT('Ctrl Pts',(-260.339217213388,-0.889986900407246,
136.05080276614));
#214585=CARTESIAN_POINT('Ctrl Pts',(-260.385654363559,-0.0148419801173944,
136.053268468065));
#214586=CARTESIAN_POINT('Ctrl Pts',(209.997106195361,2.85369542052185,134.803838223542));
#214587=CARTESIAN_POINT('Ctrl Pts',(209.950688331758,3.52024512455777,134.328247120061));
#214588=CARTESIAN_POINT('Ctrl Pts',(209.857862530854,4.598911638141,133.039517383424));
#214589=CARTESIAN_POINT('Ctrl Pts',(209.672220855345,5.31158968331849,129.722011776094));
#214590=CARTESIAN_POINT('Ctrl Pts',(209.440181168834,2.90445768035623,125.771581499823));
#214591=CARTESIAN_POINT('Ctrl Pts',(209.161733545021,-2.67328939945229,
125.640965885288));
#214592=CARTESIAN_POINT('Ctrl Pts',(208.883285921209,-5.78445646322271,
130.262241799363));
#214593=CARTESIAN_POINT('Ctrl Pts',(208.604838297395,-3.58517659481558,
135.378114005881));
#214594=CARTESIAN_POINT('Ctrl Pts',(208.326390673583,1.91144119617671,136.292814641374));
#214595=CARTESIAN_POINT('Ctrl Pts',(208.04794304977,5.65009034124608,132.162897902674));
#214596=CARTESIAN_POINT('Ctrl Pts',(207.769495425957,4.19734896093999,126.785079177362));
#214597=CARTESIAN_POINT('Ctrl Pts',(207.491047802144,-1.1129569716493,125.100504449821));
#214598=CARTESIAN_POINT('Ctrl Pts',(207.212600178331,-5.4002948496084,128.657642803108));
#214599=CARTESIAN_POINT('Ctrl Pts',(206.934152554519,-4.72513942780656,
134.187431620732));
#214600=CARTESIAN_POINT('Ctrl Pts',(206.655704930705,0.292248586550605,
136.608384944684));
#214601=CARTESIAN_POINT('Ctrl Pts',(206.377257306892,5.04104249491135,133.695701483205));
#214602=CARTESIAN_POINT('Ctrl Pts',(206.09880968308,5.15738153042831,128.12602865207));
#214603=CARTESIAN_POINT('Ctrl Pts',(205.820362059267,0.534329935251406,
125.017605890956));
#214604=CARTESIAN_POINT('Ctrl Pts',(205.541914435454,-4.57974002364783,
127.226931288585));
#214605=CARTESIAN_POINT('Ctrl Pts',(205.263466811641,-5.48525514562618,
132.723737743954));
#214606=CARTESIAN_POINT('Ctrl Pts',(204.985019187828,-1.35008742798131,
136.456731302353));
#214607=CARTESIAN_POINT('Ctrl Pts',(204.706571564015,4.02574397595362,134.995471850294));
#214608=CARTESIAN_POINT('Ctrl Pts',(204.428123940202,5.70211370766606,129.682786179275));
#214609=CARTESIAN_POINT('Ctrl Pts',(204.149676316389,2.13851930815143,125.40077248911));
#214610=CARTESIAN_POINT('Ctrl Pts',(203.871228692576,-3.39026975841633,
126.084392381055));
#214611=CARTESIAN_POINT('Ctrl Pts',(203.592781068764,-5.8035665963141,131.105432460946));
#214612=CARTESIAN_POINT('Ctrl Pts',(203.314333444951,-2.88366922283368,
135.849802245147));
#214613=CARTESIAN_POINT('Ctrl Pts',(203.035885821138,2.68617927581077,135.957657646429));
#214614=CARTESIAN_POINT('Ctrl Pts',(202.757438197325,5.78756025537181,131.329884836407));
#214615=CARTESIAN_POINT('Ctrl Pts',(202.478990573512,3.57045609392238,126.219180939555));
#214616=CARTESIAN_POINT('Ctrl Pts',(202.200542949699,-1.92772278905516,
125.322033169903));
#214617=CARTESIAN_POINT('Ctrl Pts',(201.922095325886,-5.6544186046078,129.462876497226));
#214618=CARTESIAN_POINT('Ctrl Pts',(201.643647702073,-4.18497995558374,
134.836478196445));
#214619=CARTESIAN_POINT('Ctrl Pts',(201.36520007826,1.13025082464198,136.504760820331));
#214620=CARTESIAN_POINT('Ctrl Pts',(201.086752454448,5.4068363130258,132.934654138033));
#214621=CARTESIAN_POINT('Ctrl Pts',(200.808304830635,4.71480336828096,127.406911780982));
#214622=CARTESIAN_POINT('Ctrl Pts',(200.529857206822,-0.309903540913717,
125.001258930184));
#214623=CARTESIAN_POINT('Ctrl Pts',(200.251409583008,-5.04982423566531,
127.928373032793));
#214624=CARTESIAN_POINT('Ctrl Pts',(199.972961959197,-5.14920315545485,
133.498379226012));
#214625=CARTESIAN_POINT('Ctrl Pts',(199.694514335383,-0.516715927947778,
136.59271392819));
#214626=CARTESIAN_POINT('Ctrl Pts',(199.416066711571,4.59060799437092,134.367834714685));
#214627=CARTESIAN_POINT('Ctrl Pts',(199.137619087757,5.47938743352869,128.868296891315));
#214628=CARTESIAN_POINT('Ctrl Pts',(198.859171463945,1.33287750423228,125.147907050397));
#214629=CARTESIAN_POINT('Ctrl Pts',(198.580723840131,-4.03848173676817,
126.625521704588));
#214630=CARTESIAN_POINT('Ctrl Pts',(198.302276216319,-5.69867355247927,
131.943285172176));
#214631=CARTESIAN_POINT('Ctrl Pts',(198.023828592506,-2.12206276914206,
136.214432613634));
#214632=CARTESIAN_POINT('Ctrl Pts',(197.745380968693,3.4046200305072,135.513988187415));
#214633=CARTESIAN_POINT('Ctrl Pts',(197.46693334488,5.80262334705539,130.485626102603));
#214634=CARTESIAN_POINT('Ctrl Pts',(197.188485721067,2.86829928156946,125.750165465994));
#214635=CARTESIAN_POINT('Ctrl Pts',(196.910038097254,-2.70185169946893,
125.65926326252));
#214636=CARTESIAN_POINT('Ctrl Pts',(196.631590473441,-5.78913296148881,
130.296454176353));
#214637=CARTESIAN_POINT('Ctrl Pts',(196.353142849628,-3.5564838467683,135.400386297052));
#214638=CARTESIAN_POINT('Ctrl Pts',(196.074695225815,1.94440017923737,136.280795346639));
#214639=CARTESIAN_POINT('Ctrl Pts',(195.796247602003,5.6584754297534,132.128628418917));
#214640=CARTESIAN_POINT('Ctrl Pts',(195.51779997819,4.17268819221861,126.759524075833));
#214641=CARTESIAN_POINT('Ctrl Pts',(195.239352354377,-1.14759564681435,
125.107426913349));
#214642=CARTESIAN_POINT('Ctrl Pts',(194.960904730564,-5.41329514958902,
128.690533514357));
#214643=CARTESIAN_POINT('Ctrl Pts',(194.682457106751,-4.70444086406131,
134.216143957018));
#214644=CARTESIAN_POINT('Ctrl Pts',(194.404009482938,0.327564750825761,
136.606492185605));
#214645=CARTESIAN_POINT('Ctrl Pts',(194.125561859125,5.0585543621317,133.664964953048));
#214646=CARTESIAN_POINT('Ctrl Pts',(193.847114235312,5.14097963875765,128.094682084473));
#214647=CARTESIAN_POINT('Ctrl Pts',(193.568666611499,0.499095778182989,
125.014461412655));
#214648=CARTESIAN_POINT('Ctrl Pts',(193.290218987687,-4.60143272035756,
127.254875257849));
#214649=CARTESIAN_POINT('Ctrl Pts',(193.011771363874,-5.4734693413749,132.757092746623));
#214650=CARTESIAN_POINT('Ctrl Pts',(192.733323740061,-1.31565503151135,
136.464844805061));
#214651=CARTESIAN_POINT('Ctrl Pts',(192.454876116248,4.05118197898966,134.970888425217));
#214652=CARTESIAN_POINT('Ctrl Pts',(192.176428492435,5.69518066204141,129.648096536341));
#214653=CARTESIAN_POINT('Ctrl Pts',(191.897980868622,2.1055865417199,125.38785485147));
#214654=CARTESIAN_POINT('Ctrl Pts',(191.619533244809,-3.4189387468211,126.105117354624));
#214655=CARTESIAN_POINT('Ctrl Pts',(191.341085620997,-5.80162635147675,
131.140754845624));
#214656=CARTESIAN_POINT('Ctrl Pts',(191.062637997183,-2.85290276432908,
135.867262474811));
#214657=CARTESIAN_POINT('Ctrl Pts',(190.784190373371,2.71749909118881,135.941210633695));
#214658=CARTESIAN_POINT('Ctrl Pts',(190.505742749557,5.79065203911519,131.29464457683));
#214659=CARTESIAN_POINT('Ctrl Pts',(190.227295125745,3.54247865217362,126.197531513104));
#214660=CARTESIAN_POINT('Ctrl Pts',(189.948847501932,-1.96105955641241,
125.333869340265));
#214661=CARTESIAN_POINT('Ctrl Pts',(189.670399878119,-5.66247983574075,
129.497321402909));
#214662=CARTESIAN_POINT('Ctrl Pts',(189.391952254306,-4.160357773542,134.861878651407));
#214663=CARTESIAN_POINT('Ctrl Pts',(189.113504630493,1.16492983776554,136.497775047581));
#214664=CARTESIAN_POINT('Ctrl Pts',(188.83505700668,5.41970383815296,132.901701721328));
#214665=CARTESIAN_POINT('Ctrl Pts',(188.556609382867,4.69403477852959,127.378274381527));
#214666=CARTESIAN_POINT('Ctrl Pts',(188.278161759054,-0.345222926215044,
125.003252919028));
#214667=CARTESIAN_POINT('Ctrl Pts',(187.999714135242,-5.0672376268456,127.959166031618));
#214668=CARTESIAN_POINT('Ctrl Pts',(187.721266511429,-5.13270849672517,
133.529673973213));
#214669=CARTESIAN_POINT('Ctrl Pts',(187.442818887616,-0.48147100486422,
136.595752079925));
#214670=CARTESIAN_POINT('Ctrl Pts',(187.164371263803,4.61221481930072,134.339824357932));
#214671=CARTESIAN_POINT('Ctrl Pts',(186.88592363999,5.4675005437485,128.834978175547));
#214672=CARTESIAN_POINT('Ctrl Pts',(186.607476016177,1.29842037074208,125.139898247696));
#214673=CARTESIAN_POINT('Ctrl Pts',(186.329028392364,-4.06384469161484,
126.650182513385));
#214674=CARTESIAN_POINT('Ctrl Pts',(186.050580768551,-5.69163501222784,
131.977953513933));
#214675=CARTESIAN_POINT('Ctrl Pts',(185.772133144738,-2.08909080843167,
136.227249975919));
#214676=CARTESIAN_POINT('Ctrl Pts',(185.493685520926,3.4332257905535,135.493176040453));
#214677=CARTESIAN_POINT('Ctrl Pts',(185.215237897112,5.80057561042411,130.450309792719));
#214678=CARTESIAN_POINT('Ctrl Pts',(184.9367902733,2.83747981818726,125.732798956676));
#214679=CARTESIAN_POINT('Ctrl Pts',(184.658342649487,-2.73312130836828,
125.675805527429));
#214680=CARTESIAN_POINT('Ctrl Pts',(184.379895025674,-5.79211747293216,
130.331703682172));
#214681=CARTESIAN_POINT('Ctrl Pts',(184.101447401861,-3.52844064054064,
135.421950469967));
#214682=CARTESIAN_POINT('Ctrl Pts',(183.822999778048,1.97770076659953,136.26885776521));
#214683=CARTESIAN_POINT('Ctrl Pts',(183.544552154236,5.66643178528845,132.094159137294));
#214684=CARTESIAN_POINT('Ctrl Pts',(183.266104530422,4.14798881387936,126.734198679909));
#214685=CARTESIAN_POINT('Ctrl Pts',(182.98765690661,-1.18225323696583,125.114518204765));
#214686=CARTESIAN_POINT('Ctrl Pts',(182.709209282797,-5.42606231932092,
128.72352494273));
#214687=CARTESIAN_POINT('Ctrl Pts',(182.430761658984,-4.68358520810093,
134.244718011395));
#214688=CARTESIAN_POINT('Ctrl Pts',(182.152314035171,0.362877903506298,
136.604390705933));
#214689=CARTESIAN_POINT('Ctrl Pts',(181.873866411358,5.07587394936235,133.634119096483));
#214690=CARTESIAN_POINT('Ctrl Pts',(181.595418787545,5.12438980598236,128.063437686296));
#214691=CARTESIAN_POINT('Ctrl Pts',(181.316971163732,0.463841771263853,
125.011530548415));
#214692=CARTESIAN_POINT('Ctrl Pts',(181.038523539919,-4.62295419131585,
127.282951248603));
#214693=CARTESIAN_POINT('Ctrl Pts',(180.760075916106,-5.46148109594396,
132.790375128456));
#214694=CARTESIAN_POINT('Ctrl Pts',(180.481628292294,-1.2811736815839,136.472748695004));
#214695=CARTESIAN_POINT('Ctrl Pts',(180.203180668481,4.07646975733793,134.946150534538));
#214696=CARTESIAN_POINT('Ctrl Pts',(179.924733044668,5.68803663588505,129.61344977806));
#214697=CARTESIAN_POINT('Ctrl Pts',(179.646285420855,2.07257572209157,125.37513790386));
#214698=CARTESIAN_POINT('Ctrl Pts',(179.367837797042,-3.44748102935117,
126.12601647128));
#214699=CARTESIAN_POINT('Ctrl Pts',(179.089390173229,-5.79947113363144,
131.176064759319));
#214700=CARTESIAN_POINT('Ctrl Pts',(178.810942549416,-2.82203058602,135.884535099843));
#214701=CARTESIAN_POINT('Ctrl Pts',(178.532494925603,2.74871820628535,135.924573271475));
#214702=CARTESIAN_POINT('Ctrl Pts',(178.254047301791,5.79352924936408,131.259386150458));
#214703=CARTESIAN_POINT('Ctrl Pts',(177.975599677977,3.51436994191561,126.176052793945));
#214704=CARTESIAN_POINT('Ctrl Pts',(177.697152054165,-1.99432365563702,
125.345908221933));
#214705=CARTESIAN_POINT('Ctrl Pts',(177.418704430351,-5.6703312417861,129.531814741282));
#214706=CARTESIAN_POINT('Ctrl Pts',(177.140256806539,-4.135581427815,134.887128753614));
#214707=CARTESIAN_POINT('Ctrl Pts',(176.861809182726,1.19956568393359,136.490578303229));
#214708=CARTESIAN_POINT('Ctrl Pts',(176.583361558913,5.43237053418876,132.868671586896));
#214709=CARTESIAN_POINT('Ctrl Pts',(176.3049139351,4.67309224957875,127.349763936946));
#214710=CARTESIAN_POINT('Ctrl Pts',(176.026466311287,-0.380529519146142,
125.005461870054));
#214711=CARTESIAN_POINT('Ctrl Pts',(175.748018687475,-5.08446324967622,
127.990064460173));
#214712=CARTESIAN_POINT('Ctrl Pts',(175.469571063661,-5.11602364359241,
133.560867732924));
#214713=CARTESIAN_POINT('Ctrl Pts',(175.191123439849,-0.446208240696769,
136.59857562952));
#214714=CARTESIAN_POINT('Ctrl Pts',(174.912675816035,4.63365073691483,134.311682993269));
#214715=CARTESIAN_POINT('Ctrl Pts',(174.634228192223,5.45541105372469,128.801732435971));
#214716=CARTESIAN_POINT('Ctrl Pts',(174.35578056841,1.26391512380778,125.132099343732));
#214717=CARTESIAN_POINT('Ctrl Pts',(174.077332944597,-4.089057059202,126.674997256779));
#214718=CARTESIAN_POINT('Ctrl Pts',(173.798885320784,-5.68438556634791,
132.012578367773));
#214719=CARTESIAN_POINT('Ctrl Pts',(173.520437696972,-2.0560414356932,136.239866391045));
#214720=CARTESIAN_POINT('Ctrl Pts',(173.241990073158,3.46170433115548,135.472190147709));
#214721=CARTESIAN_POINT('Ctrl Pts',(172.963542449346,5.79831293133042,130.41500660232));
#214722=CARTESIAN_POINT('Ctrl Pts',(172.685094825533,2.80655521094699,125.715620375941));
#214723=CARTESIAN_POINT('Ctrl Pts',(172.40664720172,-2.76428964045241,125.692537832834));
#214724=CARTESIAN_POINT('Ctrl Pts',(172.128199577907,-5.79488735533246,
130.366970702468));
#214725=CARTESIAN_POINT('Ctrl Pts',(171.849751954094,-3.50026668664755,
135.443343536393));
#214726=CARTESIAN_POINT('Ctrl Pts',(171.571304330281,2.01092806953244,136.256717694829));
#214727=CARTESIAN_POINT('Ctrl Pts',(171.292856706468,5.6741781691098,132.059642061713));
#214728=CARTESIAN_POINT('Ctrl Pts',(171.014409082656,4.12313573028927,126.709024105332));
#214729=CARTESIAN_POINT('Ctrl Pts',(170.735961458842,-1.21686701828875,
125.121820335384));
#214730=CARTESIAN_POINT('Ctrl Pts',(170.45751383503,-5.43862842431808,128.756593477234));
#214731=CARTESIAN_POINT('Ctrl Pts',(170.179066211217,-4.66255600016836,
134.273164582064));
#214732=CARTESIAN_POINT('Ctrl Pts',(169.900618587404,0.398177609612544,
136.602074304013));
#214733=CARTESIAN_POINT('Ctrl Pts',(169.62217096359,5.09300544821711,133.603168382178));
#214734=CARTESIAN_POINT('Ctrl Pts',(169.343723339778,5.10761008705837,128.032294854024));
#214735=CARTESIAN_POINT('Ctrl Pts',(169.065275715965,0.428570576517446,
125.008814339624));
#214736=CARTESIAN_POINT('Ctrl Pts',(168.786828092152,-4.64430435700642,
127.311157726477));
#214737=CARTESIAN_POINT('Ctrl Pts',(168.508380468339,-5.4492904733226,132.823583917792));
#214738=CARTESIAN_POINT('Ctrl Pts',(168.229932844526,-1.24664485729461,
136.480442540741));
#214739=CARTESIAN_POINT('Ctrl Pts',(167.951485220714,4.10160648060013,134.92125916831));
#214740=CARTESIAN_POINT('Ctrl Pts',(167.673037596901,5.6806818374394,129.578847149419));
#214741=CARTESIAN_POINT('Ctrl Pts',(167.394589973088,2.03948810240773,125.362622138095));
#214742=CARTESIAN_POINT('Ctrl Pts',(167.116142349275,-3.47589556420378,
126.147088945699));
#214743=CARTESIAN_POINT('Ctrl Pts',(166.837694725462,-5.79710101425052,
131.21136089938));
#214744=CARTESIAN_POINT('Ctrl Pts',(166.559247101649,-2.79105383632985,
135.901619477142));
#214745=CARTESIAN_POINT('Ctrl Pts',(166.280799477836,2.77983546661788,135.907746177893));
#214746=CARTESIAN_POINT('Ctrl Pts',(166.002351854023,5.79619177825601,131.224110862948));
#214747=CARTESIAN_POINT('Ctrl Pts',(165.72390423021,3.48613100538707,126.154745578436));
#214748=CARTESIAN_POINT('Ctrl Pts',(165.445456606397,-2.02751385446508,
125.358149368562));
#214749=CARTESIAN_POINT('Ctrl Pts',(165.167008982585,-5.67797253162207,
129.566355234311));
#214750=CARTESIAN_POINT('Ctrl Pts',(164.888561358772,-4.11065183659732,
134.912227567346));
#214751=CARTESIAN_POINT('Ctrl Pts',(164.610113734959,1.23415707975413,136.483170853989));
#214752=CARTESIAN_POINT('Ctrl Pts',(164.331666111146,5.44483593173667,132.835564958663));
#214753=CARTESIAN_POINT('Ctrl Pts',(164.053218487333,4.65197655747607,127.321381503715));
#214754=CARTESIAN_POINT('Ctrl Pts',(163.77477086352,-0.415822011415935,
125.007885701408));
#214755=CARTESIAN_POINT('Ctrl Pts',(163.496323239708,-5.10150046585131,
128.021067173507));
#214756=CARTESIAN_POINT('Ctrl Pts',(163.217875615894,-5.09914921432216,
133.591959349252));
#214757=CARTESIAN_POINT('Ctrl Pts',(162.939427992082,-0.41092894211879,
136.601184472346));
#214758=CARTESIAN_POINT('Ctrl Pts',(162.660980368268,4.65491495289691,134.283411663486));
#214759=CARTESIAN_POINT('Ctrl Pts',(162.382532744456,5.443119411438,128.768560904517));
#214760=CARTESIAN_POINT('Ctrl Pts',(162.104085120643,1.22936304203373,125.124510627495));
#214761=CARTESIAN_POINT('Ctrl Pts',(161.82563749683,-4.11411790527609,126.69996501525));
#214762=CARTESIAN_POINT('Ctrl Pts',(161.547189873017,-5.67692548347038,
132.04715845066));
#214763=CARTESIAN_POINT('Ctrl Pts',(161.268742249204,-2.02291587558315,
136.252281391507));
#214764=CARTESIAN_POINT('Ctrl Pts',(160.990294625391,3.49005459703047,135.451031286826));
#214765=CARTESIAN_POINT('Ctrl Pts',(160.711847001578,5.79583539361873,130.379717839577));
#214766=CARTESIAN_POINT('Ctrl Pts',(160.433399377766,2.77552660577121,125.698630360346));
#214767=CARTESIAN_POINT('Ctrl Pts',(160.154951753952,-2.79535554076737,
125.70945955871));
#214768=CARTESIAN_POINT('Ctrl Pts',(159.87650413014,-5.79744250605075,130.402253930408));
#214769=CARTESIAN_POINT('Ctrl Pts',(159.598056506327,-3.47196302908515,
135.4645647036));
#214770=CARTESIAN_POINT('Ctrl Pts',(159.319608882514,2.04408085678626,136.244375585352));
#214771=CARTESIAN_POINT('Ctrl Pts',(159.041161258701,5.68171429417248,132.025078471215));
#214772=CARTESIAN_POINT('Ctrl Pts',(158.762713634888,4.09812986238831,126.684001284956));
#214773=CARTESIAN_POINT('Ctrl Pts',(158.484266011075,-1.25143570815684,
125.129333034622));
#214774=CARTESIAN_POINT('Ctrl Pts',(158.205818387262,-5.450992998939,128.789737892503));
#214775=CARTESIAN_POINT('Ctrl Pts',(157.927370763449,-4.64135401950845,
134.301482614925));
#214776=CARTESIAN_POINT('Ctrl Pts',(157.648923139637,0.43346256110109,136.59954306568));
#214777=CARTESIAN_POINT('Ctrl Pts',(157.370475515823,5.10994822388206,133.572113957021));
#214778=CARTESIAN_POINT('Ctrl Pts',(157.092027892011,5.09064110376424,128.001254741669));
#214779=CARTESIAN_POINT('Ctrl Pts',(156.813580268198,0.39328350093061,125.006312886931));
#214780=CARTESIAN_POINT('Ctrl Pts',(156.535132644385,-4.66548242629113,
127.339493646268));
#214781=CARTESIAN_POINT('Ctrl Pts',(156.256685020572,-5.43689792523874,
132.856717884066));
#214782=CARTESIAN_POINT('Ctrl Pts',(155.978237396759,-1.21206983812162,
136.487926057176));
#214783=CARTESIAN_POINT('Ctrl Pts',(155.699789772946,4.12659121732586,134.896215248893));
#214784=CARTESIAN_POINT('Ctrl Pts',(155.421342149133,5.67311653923917,129.544289932631));
#214785=CARTESIAN_POINT('Ctrl Pts',(155.142894525321,2.0063249087422,125.350308017949));
#214786=CARTESIAN_POINT('Ctrl Pts',(154.864446901507,-3.50418129846815,
126.168333997033));
#214787=CARTESIAN_POINT('Ctrl Pts',(154.585999277695,-5.79451608115961,
131.246641957895));
#214788=CARTESIAN_POINT('Ctrl Pts',(154.307551653882,-2.75997366311328,
135.918514973638));
#214789=CARTESIAN_POINT('Ctrl Pts',(154.029104030069,2.81084971912495,135.890729976482));
#214790=CARTESIAN_POINT('Ctrl Pts',(153.750656406256,5.79863952713012,131.188820021437));
#214791=CARTESIAN_POINT('Ctrl Pts',(153.472208782443,3.457762888992,126.133610656121));
#214792=CARTESIAN_POINT('Ctrl Pts',(153.19376115863,-2.0606289230217,125.370592326552));
#214793=CARTESIAN_POINT('Ctrl Pts',(152.915313534817,-5.68540342209783,
129.600941602086));
#214794=CARTESIAN_POINT('Ctrl Pts',(152.636865911004,-4.08556992366409,
134.937174162558));
#214795=CARTESIAN_POINT('Ctrl Pts',(152.358418287191,1.26870274343019,136.475552974349));
#214796=CARTESIAN_POINT('Ctrl Pts',(152.079970663379,5.45709956888678,132.802383063404));
#214797=CARTESIAN_POINT('Ctrl Pts',(151.801523039566,4.63068848467127,127.293128133558));
#214798=CARTESIAN_POINT('Ctrl Pts',(151.523075415753,-0.451099095248245,
125.010524323271));
#214799=CARTESIAN_POINT('Ctrl Pts',(151.24462779194,-5.11834864405056,128.052173022803));
#214800=CARTESIAN_POINT('Ctrl Pts',(150.966180168127,-5.08208583420252,
133.622947670083));
#214801=CARTESIAN_POINT('Ctrl Pts',(150.687732544314,-0.375634416417742,
136.603578511732));
#214802=CARTESIAN_POINT('Ctrl Pts',(150.409284920501,4.67600667929353,134.255011416186));
#214803=CARTESIAN_POINT('Ctrl Pts',(150.130837296688,5.43062607235983,128.735464810371));
#214804=CARTESIAN_POINT('Ctrl Pts',(149.852389672876,1.19476540576009,125.117132380189));
#214805=CARTESIAN_POINT('Ctrl Pts',(149.573942049063,-4.13902630119825,
126.725084863609));
#214806=CARTESIAN_POINT('Ctrl Pts',(149.29549442525,-5.66925504003138,132.081692481218));
#214807=CARTESIAN_POINT('Ctrl Pts',(149.017046801437,-1.98971535558138,
136.264494517259));
#214808=CARTESIAN_POINT('Ctrl Pts',(148.738599177624,3.5182755376489,135.429700241853));
#214809=CARTESIAN_POINT('Ctrl Pts',(148.460151553811,5.79314308909515,130.344444812129));
#214810=CARTESIAN_POINT('Ctrl Pts',(148.181703929998,2.74439515243632,125.681829539465));
#214811=CARTESIAN_POINT('Ctrl Pts',(147.903256306185,-2.82631785815477,
125.726570078021));
#214812=CARTESIAN_POINT('Ctrl Pts',(147.624808682372,-5.79978283040501,
130.437552058559));
#214813=CARTESIAN_POINT('Ctrl Pts',(147.346361058559,-3.4435307166558,135.48561318523));
#214814=CARTESIAN_POINT('Ctrl Pts',(147.067913434747,2.07715789987228,136.23183189412));
#214815=CARTESIAN_POINT('Ctrl Pts',(146.789465810933,5.68903988122249,131.990469646568));
#214816=CARTESIAN_POINT('Ctrl Pts',(146.511018187121,4.07297213677825,126.65913114601));
#214817=CARTESIAN_POINT('Ctrl Pts',(146.232570563308,-1.2859580256146,125.137056024094));
#214818=CARTESIAN_POINT('Ctrl Pts',(145.954122939495,-5.46315558500969,
128.822956960357));
#214819=CARTESIAN_POINT('Ctrl Pts',(145.675675315682,-4.61998005176852,
134.329671060644));
#214820=CARTESIAN_POINT('Ctrl Pts',(145.397227691869,0.468731450475054,
136.596797084732));
#214821=CARTESIAN_POINT('Ctrl Pts',(145.118780068056,5.12670164853643,133.540956971746));
#214822=CARTESIAN_POINT('Ctrl Pts',(144.840332444244,5.07348348489189,127.970318499433));
#214823=CARTESIAN_POINT('Ctrl Pts',(144.56188482043,0.357981852079004,125.004026283029));
#214824=CARTESIAN_POINT('Ctrl Pts',(144.283437196618,-4.6864876144088,127.367957957979));
#214825=CARTESIAN_POINT('Ctrl Pts',(144.004989572805,-5.42430391090288,
132.889775799486));
#214826=CARTESIAN_POINT('Ctrl Pts',(143.726541948992,-1.17744990525502,
136.495198967004));
#214827=CARTESIAN_POINT('Ctrl Pts',(143.448094325179,4.15142304169647,134.871019704297));
#214828=CARTESIAN_POINT('Ctrl Pts',(143.169646701366,5.66534102161933,129.509779408224));
#214829=CARTESIAN_POINT('Ctrl Pts',(142.891199077553,1.9730873699693,125.338195999729));
#214830=CARTESIAN_POINT('Ctrl Pts',(142.61275145374,-3.53233718400576,126.189750838038));
#214831=CARTESIAN_POINT('Ctrl Pts',(142.334303829928,-5.79171643014443,
131.281906627513));
#214832=CARTESIAN_POINT('Ctrl Pts',(142.055856206114,-2.72879121805762,
135.935220963265));
#214833=CARTESIAN_POINT('Ctrl Pts',(141.777408582302,2.84175981456215,135.873525297782));
#214834=CARTESIAN_POINT('Ctrl Pts',(141.498960958489,5.80087240528401,131.153514933643));
#214835=CARTESIAN_POINT('Ctrl Pts',(141.220513334676,3.42926664392146,126.112648810165));
#214836=CARTESIAN_POINT('Ctrl Pts',(140.942065710863,-2.09366763421581,
125.383236634823));
#214837=CARTESIAN_POINT('Ctrl Pts',(140.66361808705,-5.69262363785895,129.635572562993));
#214838=CARTESIAN_POINT('Ctrl Pts',(140.385170463237,-4.06033661843482,
134.961967614844));
#214839=CARTESIAN_POINT('Ctrl Pts',(140.106722839424,1.30320139485961,136.467724946589));
#214840=CARTESIAN_POINT('Ctrl Pts',(139.828275215611,5.46916099120554,132.769127130691));
#214841=CARTESIAN_POINT('Ctrl Pts',(139.549827591798,4.60922882000175,127.26500487341));
#214842=CARTESIAN_POINT('Ctrl Pts',(139.271379967986,-0.486359463437733,
125.013377637868));
#214843=CARTESIAN_POINT('Ctrl Pts',(138.992932344173,-5.13500715995863,
128.083380855422));
#214844=CARTESIAN_POINT('Ctrl Pts',(138.71448472036,-5.06483413552331,133.653831547135));
#214845=CARTESIAN_POINT('Ctrl Pts',(138.436037096547,-0.340325971445257,
136.605757658967));
#214846=CARTESIAN_POINT('Ctrl Pts',(138.157589472734,4.69692513454305,134.226483303753));
#214847=CARTESIAN_POINT('Ctrl Pts',(137.879141848921,5.41793149943546,128.70244537992));
#214848=CARTESIAN_POINT('Ctrl Pts',(137.600694225109,1.16012349701482,125.109964875215));
#214849=CARTESIAN_POINT('Ctrl Pts',(137.322246601295,-4.16378132397874,
126.750355871033));
#214850=CARTESIAN_POINT('Ctrl Pts',(137.043798977483,-5.66137452026194,
132.116179179772));
#214851=CARTESIAN_POINT('Ctrl Pts',(136.765351353669,-1.95644110594549,
136.276505315742));
#214852=CARTESIAN_POINT('Ctrl Pts',(136.486903729857,3.54636610727348,135.408197803219));
#214853=CARTESIAN_POINT('Ctrl Pts',(136.208456106044,5.79023611752392,130.309188827029));
#214854=CARTESIAN_POINT('Ctrl Pts',(135.930008482231,2.71316200452982,125.665218535856));
#214855=CARTESIAN_POINT('Ctrl Pts',(135.651560858418,-2.85717544529452,
125.743868756725));
#214856=CARTESIAN_POINT('Ctrl Pts',(135.373113234605,-5.80190824167357,
130.472863778936));
#214857=CARTESIAN_POINT('Ctrl Pts',(135.094665610792,-3.41497080292952,
135.506488201326));
#214858=CARTESIAN_POINT('Ctrl Pts',(134.816217986979,2.11015797310843,136.219087085943));
#214859=CARTESIAN_POINT('Ctrl Pts',(134.537770363167,5.69615465880763,131.955816870215));
#214860=CARTESIAN_POINT('Ctrl Pts',(134.259322739353,4.04766348568775,126.634414610068));
#214861=CARTESIAN_POINT('Ctrl Pts',(133.980875115541,-1.32043269142476,
125.144989017623));
#214862=CARTESIAN_POINT('Ctrl Pts',(133.702427491728,-5.47511573184112,
128.856249449853));
#214863=CARTESIAN_POINT('Ctrl Pts',(133.423979867915,-4.59843488896879,
134.357728874689));
#214864=CARTESIAN_POINT('Ctrl Pts',(133.145532244102,0.503982970832797,
136.59383646292));
#214865=CARTESIAN_POINT('Ctrl Pts',(132.867084620289,5.14326510137581,133.509698580887));
#214866=CARTESIAN_POINT('Ctrl Pts',(132.588636996476,5.05613786622328,127.93948727367));
#214867=CARTESIAN_POINT('Ctrl Pts',(132.310189372663,0.322666938078297,
125.001954612649));
#214868=CARTESIAN_POINT('Ctrl Pts',(132.03174174885,-4.70731914300451,127.396549606854));
#214869=CARTESIAN_POINT('Ctrl Pts',(131.753294125038,-5.41150889699075,
132.92275643908));
#214870=CARTESIAN_POINT('Ctrl Pts',(131.474846501225,-1.14278634154918,
136.502261000723));
#214871=CARTESIAN_POINT('Ctrl Pts',(131.196398877412,4.17610103355955,134.845673468154));
#214872=CARTESIAN_POINT('Ctrl Pts',(130.917951253599,5.65735557270449,129.475316855001));
#214873=CARTESIAN_POINT('Ctrl Pts',(130.639503629786,1.93977671771839,125.326286532249));
#214874=CARTESIAN_POINT('Ctrl Pts',(130.361056005973,-3.56036217749005,
126.211338675105));
#214875=CARTESIAN_POINT('Ctrl Pts',(130.08260838216,-5.788702164947,131.317153601487));
#214876=CARTESIAN_POINT('Ctrl Pts',(129.804160758347,-2.69750765663984,
135.951736826975));
#214877=CARTESIAN_POINT('Ctrl Pts',(129.525713134534,2.87256460754407,135.856132779323));
#214878=CARTESIAN_POINT('Ctrl Pts',(129.247265510721,5.80289032997773,131.118196907806));
#214879=CARTESIAN_POINT('Ctrl Pts',(128.968817886909,3.40064332611445,126.091860817314));
#214880=CARTESIAN_POINT('Ctrl Pts',(128.690370263096,-2.12662876378584,
125.396081824838));
#214881=CARTESIAN_POINT('Ctrl Pts',(128.411922639283,-5.69963291135762,
129.670246833772));
#214882=CARTESIAN_POINT('Ctrl Pts',(128.13347501547,-4.03495285593914,134.986607005474));
#214883=CARTESIAN_POINT('Ctrl Pts',(127.855027391657,1.33765175568188,136.459687060782));
#214884=CARTESIAN_POINT('Ctrl Pts',(127.576579767844,5.48101975175251,132.73579839283));
#214885=CARTESIAN_POINT('Ctrl Pts',(127.298132144031,4.5875983586632,127.237012765392));
#214886=CARTESIAN_POINT('Ctrl Pts',(127.019684520218,-0.521601809398458,
125.016445539469));
#214887=CARTESIAN_POINT('Ctrl Pts',(126.741236896406,-5.15147539628782,
128.114689514947));
#214888=CARTESIAN_POINT('Ctrl Pts',(126.462789272592,-5.0473947575527,133.684609835992));
#214889=CARTESIAN_POINT('Ctrl Pts',(126.18434164878,-0.305004915568794,
136.607721833301));
#214890=CARTESIAN_POINT('Ctrl Pts',(125.905894024967,4.71766954350447,134.197828383304));
#214891=CARTESIAN_POINT('Ctrl Pts',(125.627446401154,5.40503616306688,128.669503836711));
#214892=CARTESIAN_POINT('Ctrl Pts',(125.348998777341,1.12543859946687,125.10300837817));
#214893=CARTESIAN_POINT('Ctrl Pts',(125.070551153528,-4.18838205631096,
126.775777101093));
#214894=CARTESIAN_POINT('Ctrl Pts',(124.792103529715,-5.65328421617778,
132.150617268407));
#214895=CARTESIAN_POINT('Ctrl Pts',(124.513655905902,-1.9230943596648,136.288313341892));
#214896=CARTESIAN_POINT('Ctrl Pts',(124.23520828209,3.57432526499779,135.386524767704));
#214897=CARTESIAN_POINT('Ctrl Pts',(123.956760658277,5.78711458662396,130.273951190703));
#214898=CARTESIAN_POINT('Ctrl Pts',(123.678313034464,2.68182831940755,125.648797965047));
#214899=CARTESIAN_POINT('Ctrl Pts',(123.399865410651,-2.88792715874745,
125.761354953818));
#214900=CARTESIAN_POINT('Ctrl Pts',(123.121417786838,-5.8038186610986,130.50818778305));
#214901=CARTESIAN_POINT('Ctrl Pts',(122.842970163025,-3.38628434620416,
135.527188978355));
#214902=CARTESIAN_POINT('Ctrl Pts',(122.564522539212,2.1430798536649,136.206141633086));
#214903=CARTESIAN_POINT('Ctrl Pts',(122.286074915399,5.703058363287,131.921121426228));
#214904=CARTESIAN_POINT('Ctrl Pts',(122.007627291586,4.02220484693838,126.609852593007));
#214905=CARTESIAN_POINT('Ctrl Pts',(121.729179667773,-1.35485842811595,
125.153131721247));
#214906=CARTESIAN_POINT('Ctrl Pts',(121.450732043961,-5.48687299624567,
128.889614127324));
#214907=CARTESIAN_POINT('Ctrl Pts',(121.172284420148,-4.57671932947311,
134.385655017367));
#214908=CARTESIAN_POINT('Ctrl Pts',(120.893836796335,0.539215815916097,
136.59066130995));
#214909=CARTESIAN_POINT('Ctrl Pts',(120.615389172522,5.15963796863542,133.478339942736));
#214910=CARTESIAN_POINT('Ctrl Pts',(120.336941548709,5.0386048905067,127.908762206842));
#214911=CARTESIAN_POINT('Ctrl Pts',(120.058493924896,0.287340067535411,
125.000097952557));
#214912=CARTESIAN_POINT('Ctrl Pts',(119.780046301083,-4.72797624015824,
127.42526753342));
#214913=CARTESIAN_POINT('Ctrl Pts',(119.50159867727,-5.39851335762638,132.955658580739));
#214914=CARTESIAN_POINT('Ctrl Pts',(119.223151053457,-1.10808043147514,
136.509111896649));
#214915=CARTESIAN_POINT('Ctrl Pts',(118.944703429644,4.20062427846316,134.820177479675));
#214916=CARTESIAN_POINT('Ctrl Pts',(118.666255805832,5.64916048839838,129.440903549983));
#214917=CARTESIAN_POINT('Ctrl Pts',(118.387808182019,1.90639418632776,125.314580056818));
#214918=CARTESIAN_POINT('Ctrl Pts',(118.109360558206,-3.58825524044456,
126.23309670829));
#214919=CARTESIAN_POINT('Ctrl Pts',(117.830912934393,-5.785473397262,131.352381573729));
#214920=CARTESIAN_POINT('Ctrl Pts',(117.55246531058,-2.66612413808396,135.968061952766));
#214921=CARTESIAN_POINT('Ctrl Pts',(117.274017686767,2.9032629565882,135.838553065588));
#214922=CARTESIAN_POINT('Ctrl Pts',(116.995570062954,5.80469322643624,131.082867252651));
#214923=CARTESIAN_POINT('Ctrl Pts',(116.717122439142,3.37189399621826,126.071247447876));
#214924=CARTESIAN_POINT('Ctrl Pts',(116.438674815328,-2.15951109034483,
125.409127420613));
#214925=CARTESIAN_POINT('Ctrl Pts',(116.160227191516,-5.70643098286277,
129.704963129555));
#214926=CARTESIAN_POINT('Ctrl Pts',(115.881779567703,-4.00941957678149,
135.011091421425));
#214927=CARTESIAN_POINT('Ctrl Pts',(115.60333194389,1.37205254932662,136.451439614773));
#214928=CARTESIAN_POINT('Ctrl Pts',(115.324884320077,5.49267541109693,132.702398084833));
#214929=CARTESIAN_POINT('Ctrl Pts',(115.046436696264,4.56579790218037,127.20915284676));
#214930=CARTESIAN_POINT('Ctrl Pts',(114.767989072451,-0.556824827212187,
125.019727914392));
#214931=CARTESIAN_POINT('Ctrl Pts',(114.489541448638,-5.1677527428018,128.146097841224));
#214932=CARTESIAN_POINT('Ctrl Pts',(114.211093824825,-5.02976834651319,
133.715281396157));
#214933=CARTESIAN_POINT('Ctrl Pts',(113.932646201012,-0.269672557622912,
136.60947096195));
#214934=CARTESIAN_POINT('Ctrl Pts',(113.6541985772,4.73823913748602,134.169047716661));
#214935=CARTESIAN_POINT('Ctrl Pts',(113.375750953387,5.39194054109557,128.636641401405));
#214936=CARTESIAN_POINT('Ctrl Pts',(113.097303329574,1.09071199837779,125.09626314683));
#214937=CARTESIAN_POINT('Ctrl Pts',(112.818855705761,-4.21282758660586,
126.801347611796));
#214938=CARTESIAN_POINT('Ctrl Pts',(112.540408081948,-5.64498442756793,
132.185005471008));
#214939=CARTESIAN_POINT('Ctrl Pts',(112.261960458135,-1.8896763524154,136.299918158156));
#214940=CARTESIAN_POINT('Ctrl Pts',(111.983512834322,3.60215197478495,135.364681938413));
#214941=CARTESIAN_POINT('Ctrl Pts',(111.705065210509,5.78377861206482,130.238733208892));
#214942=CARTESIAN_POINT('Ctrl Pts',(111.426617586696,2.65039525815055,125.632568435507));
#214943=CARTESIAN_POINT('Ctrl Pts',(111.148169962883,-2.91857185899754,
125.77902802134));
#214944=CARTESIAN_POINT('Ctrl Pts',(110.869722339071,-5.80551401788879,
130.543522761958));
#214945=CARTESIAN_POINT('Ctrl Pts',(110.591274715258,-3.35747240946702,
135.547714749242));
#214946=CARTESIAN_POINT('Ctrl Pts',(110.312827091445,2.17592232160915,136.192996015246));
#214947=CARTESIAN_POINT('Ctrl Pts',(110.034379467632,5.70975073884148,131.886384600257));
#214948=CARTESIAN_POINT('Ctrl Pts',(109.755931843819,3.99659716390926,126.585446004984));
#214949=CARTESIAN_POINT('Ctrl Pts',(109.477484220006,-1.38923396002991,
125.161483833236));
#214950=CARTESIAN_POINT('Ctrl Pts',(109.199036596193,-5.49842694255352,
128.923049756431));
#214951=CARTESIAN_POINT('Ctrl Pts',(108.92058897238,-4.55483417795961,134.413448453863));
#214952=CARTESIAN_POINT('Ctrl Pts',(108.642141348568,0.57442868015902,136.58727174348));
#214953=CARTESIAN_POINT('Ctrl Pts',(108.363693724754,5.17581964361271,133.446882219296));
#214954=CARTESIAN_POINT('Ctrl Pts',(108.085246100942,5.02088520743284,127.878144437479));
#214955=CARTESIAN_POINT('Ctrl Pts',(107.806798477129,0.252002549500665,
124.998456371553));
#214956=CARTESIAN_POINT('Ctrl Pts',(107.528350853316,-4.74845814041369,
127.454110673523));
#214957=CARTESIAN_POINT('Ctrl Pts',(107.249903229503,-5.38531777436419,
132.988481005259));
#214958=CARTESIAN_POINT('Ctrl Pts',(106.97145560569,-1.07333346107335,136.515751400918));
#214959=CARTESIAN_POINT('Ctrl Pts',(106.693007981877,4.22499186768932,134.794532683627));
#214960=CARTESIAN_POINT('Ctrl Pts',(106.414560358064,5.64075607237289,129.406540768369));
#214961=CARTESIAN_POINT('Ctrl Pts',(106.136112734251,1.87294101279944,125.303077007226));
#214962=CARTESIAN_POINT('Ctrl Pts',(105.857665110439,-3.61601533928142,
126.25502413134));
#214963=CARTESIAN_POINT('Ctrl Pts',(105.579217486626,-5.78203024673271,
131.387589238853));
#214964=CARTESIAN_POINT('Ctrl Pts',(105.300769862813,-2.63464182531766,
135.984195735705));
#214965=CARTESIAN_POINT('Ctrl Pts',(105.022322239,2.93385372415587,135.820786808));
#214966=CARTESIAN_POINT('Ctrl Pts',(104.743874615187,5.80628102785255,131.047527277329));
#214967=CARTESIAN_POINT('Ctrl Pts',(104.465426991374,3.34301971955009,126.050809465687));
#214968=CARTESIAN_POINT('Ctrl Pts',(104.186979367561,-2.19231339542621,
125.422372938737));
#214969=CARTESIAN_POINT('Ctrl Pts',(103.908531743748,-5.71301760046937,
129.739720163916));
#214970=CARTESIAN_POINT('Ctrl Pts',(103.630084119935,-3.98373772710686,
135.03541995542));
#214971=CARTESIAN_POINT('Ctrl Pts',(103.351636496123,1.40640250105958,136.442982914176));
#214972=CARTESIAN_POINT('Ctrl Pts',(103.07318887231,5.50412753733405,132.66892744436));
#214973=CARTESIAN_POINT('Ctrl Pts',(102.794741248497,4.54382825837723,127.181426149873));
#214974=CARTESIAN_POINT('Ctrl Pts',(102.516293624684,-0.592027211677165,
125.023224641008));
#214975=CARTESIAN_POINT('Ctrl Pts',(102.237846000871,-5.18383859633749,
128.177604670405));
#214976=CARTESIAN_POINT('Ctrl Pts',(101.959398377058,-5.01195555555783,
133.745845091081));
#214977=CARTESIAN_POINT('Ctrl Pts',(101.680950753245,-0.234330206861215,
136.611004980102));
#214978=CARTESIAN_POINT('Ctrl Pts',(101.402503129432,4.75863315427373,134.140142370299));
#214979=CARTESIAN_POINT('Ctrl Pts',(101.124055505619,5.37864511878468,128.603859291732));
#214980=CARTESIAN_POINT('Ctrl Pts',(100.845607881807,1.05594498055446,125.089729431141));
#214981=CARTESIAN_POINT('Ctrl Pts',(100.567160257994,-4.23711700902531,
126.827066455619));
#214982=CARTESIAN_POINT('Ctrl Pts',(100.288712634181,-5.63647546198416,
132.219342513305));
#214983=CARTESIAN_POINT('Ctrl Pts',(100.010265010368,-1.85618832251382,
136.311319334515));
#214984=CARTESIAN_POINT('Ctrl Pts',(99.731817386555,3.62984520550588,135.342670124737));
#214985=CARTESIAN_POINT('Ctrl Pts',(99.4533697627421,5.78022831746224,130.203536186614));
#214986=CARTESIAN_POINT('Ctrl Pts',(99.1749221389292,2.61886398552269,125.616530548629));
#214987=CARTESIAN_POINT('Ctrl Pts',(98.8964745151164,-2.9491084104941,125.796887304409));
#214988=CARTESIAN_POINT('Ctrl Pts',(98.6180268913035,-5.80699424922206,
130.578867406308));
#214989=CARTESIAN_POINT('Ctrl Pts',(98.3395792674906,-3.32853606035512,
135.568064753397));
#214990=CARTESIAN_POINT('Ctrl Pts',(98.0611316436778,2.20868415995158,136.179650719541));
#214991=CARTESIAN_POINT('Ctrl Pts',(97.7826840198649,5.71623153748262,131.851607679491));
#214992=CARTESIAN_POINT('Ctrl Pts',(97.5042363960519,3.97084138550236,126.561195750394));
#214993=CARTESIAN_POINT('Ctrl Pts',(97.2257887722391,-1.42355801336861,
125.170045044101));
#214994=CARTESIAN_POINT('Ctrl Pts',(96.9473411484261,-5.50977714262889,
128.956555098203));
#214995=CARTESIAN_POINT('Ctrl Pts',(96.6688935246133,-4.53278024539068,
134.441108154283));
#214996=CARTESIAN_POINT('Ctrl Pts',(96.3904459008004,0.609620258735999,
136.583667889112));
#214997=CARTESIAN_POINT('Ctrl Pts',(96.1119982769875,5.19180952668969,133.415326576248));
#214998=CARTESIAN_POINT('Ctrl Pts',(95.8335506531746,5.00297947361121,127.847635100131));
#214999=CARTESIAN_POINT('Ctrl Pts',(95.5551030293618,0.216655693418756,
124.997029930466));
#215000=CARTESIAN_POINT('Ctrl Pts',(95.2766554055487,-4.7687640848064,127.483077958369));
#215001=CARTESIAN_POINT('Ctrl Pts',(94.9982077817361,-5.37192263617151,
133.021222496396));
#215002=CARTESIAN_POINT('Ctrl Pts',(94.7197601579228,-1.03854671790542,
136.522179267501));
#215003=CARTESIAN_POINT('Ctrl Pts',(94.4413125341102,4.24920289828813,134.768740030285));
#215004=CARTESIAN_POINT('Ctrl Pts',(94.1628649102971,5.63214263605674,129.372229783482));
#215005=CARTESIAN_POINT('Ctrl Pts',(93.8844172864844,1.83941843675322,125.29177780972));
#215006=CARTESIAN_POINT('Ctrl Pts',(93.6059696626714,-3.6436414453401,126.277120131727));
#215007=CARTESIAN_POINT('Ctrl Pts',(93.3275220388585,-5.77837284094635,
131.422775292226));
#215008=CARTESIAN_POINT('Ctrl Pts',(93.0490744150458,-2.60306188492951,
136.000137577949));
#215009=CARTESIAN_POINT('Ctrl Pts',(92.7706267912327,2.96433577669487,135.802834664895));
#215010=CARTESIAN_POINT('Ctrl Pts',(92.49217916742,5.80765367539012,131.012178291378));
#215011=CARTESIAN_POINT('Ctrl Pts',(92.213731543607,3.31402156605677,126.030547628085));
#215012=CARTESIAN_POINT('Ctrl Pts',(91.9352839197941,-2.22503446352861,
125.435817888395));
#215013=CARTESIAN_POINT('Ctrl Pts',(91.6568362959812,-5.71939252010779,
129.77451664892));
#215014=CARTESIAN_POINT('Ctrl Pts',(91.3783886721684,-3.95790825856573,
135.059591705955));
#215015=CARTESIAN_POINT('Ctrl Pts',(91.0999410483554,1.44070033803066,136.434317272356));
#215016=CARTESIAN_POINT('Ctrl Pts',(90.8214934245425,5.51537570610103,132.635387711677));
#215017=CARTESIAN_POINT('Ctrl Pts',(90.5430458007297,4.52169024134706,127.153833702157));
#215018=CARTESIAN_POINT('Ctrl Pts',(90.2645981769166,-0.627207658356129,
125.026935589742));
#215019=CARTESIAN_POINT('Ctrl Pts',(89.9861505531037,-5.19973236082766,
128.209208834995));
#215020=CARTESIAN_POINT('Ctrl Pts',(89.707702929291,-4.99395704474619,133.776299788217));
#215021=CARTESIAN_POINT('Ctrl Pts',(89.4292553054779,-0.198979172907652,
136.61232383091));
#215022=CARTESIAN_POINT('Ctrl Pts',(89.1508076816652,4.77885083815996,134.111113415317));
#215023=CARTESIAN_POINT('Ctrl Pts',(88.8723600578521,5.36515038880097,128.571158722445));
#215024=CARTESIAN_POINT('Ctrl Pts',(88.5939124340396,1.02113883430145,125.08340747321));
#215025=CARTESIAN_POINT('Ctrl Pts',(88.3154648102263,-4.26124942351577,
126.85293267954));
#215026=CARTESIAN_POINT('Ctrl Pts',(88.0370171864138,-5.62775763472933,
132.253627122929));
#215027=CARTESIAN_POINT('Ctrl Pts',(87.7585695626006,-1.82263151087143,
136.322516448493));
#215028=CARTESIAN_POINT('Ctrl Pts',(87.480121938788,3.65740393097785,135.320490142334));
#215029=CARTESIAN_POINT('Ctrl Pts',(87.2016743149749,5.77646383437373,130.168361428106));
#215030=CARTESIAN_POINT('Ctrl Pts',(86.9232266911622,2.58723566992664,125.600684898703));
#215031=CARTESIAN_POINT('Ctrl Pts',(86.6447790673492,-2.97953568169397,
125.814932141244));
#215032=CARTESIAN_POINT('Ctrl Pts',(86.3663314435363,-5.80825930024783,
130.614220406392));
#215033=CARTESIAN_POINT('Ctrl Pts',(86.0878838197235,-3.29947637111547,
135.588238236744));
#215034=CARTESIAN_POINT('Ctrl Pts',(85.8094361959104,2.24136415469026,136.166106240484));
#215035=CARTESIAN_POINT('Ctrl Pts',(85.5309885720977,5.72250051906197,131.816791952599));
#215036=CARTESIAN_POINT('Ctrl Pts',(85.2525409482847,3.94493846610766,126.537102727838));
#215037=CARTESIAN_POINT('Ctrl Pts',(84.9740933244718,-1.45782931624159,
125.178815036599));
#215038=CARTESIAN_POINT('Ctrl Pts',(84.6956457006588,-5.52092317588609,
128.990128911089));
#215039=CARTESIAN_POINT('Ctrl Pts',(84.417198076846,-4.51055834898274,134.468633093685));
#215040=CARTESIAN_POINT('Ctrl Pts',(84.138750453033,0.644789247610192,136.579849880389));
#215041=CARTESIAN_POINT('Ctrl Pts',(83.8603028292202,5.20760702535536,133.383674182895));
#215042=CARTESIAN_POINT('Ctrl Pts',(83.5818552054073,4.98488835254533,127.817235325336));
#215043=CARTESIAN_POINT('Ctrl Pts',(83.3034075815944,0.181300809080568,
124.995818682153));
#215044=CARTESIAN_POINT('Ctrl Pts',(83.0249599577814,-4.78889332089225,
127.512168314565));
#215045=CARTESIAN_POINT('Ctrl Pts',(82.7465123339688,-5.35832843941005,
133.053881840899));
#215046=CARTESIAN_POINT('Ctrl Pts',(82.4680647101557,-1.00372149100682,
136.528395258211));
#215047=CARTESIAN_POINT('Ctrl Pts',(82.1896170863428,4.27325647311088,134.742800475408));
#215048=CARTESIAN_POINT('Ctrl Pts',(81.91116946253,5.62332049862395,129.337971866731));
#215049=CARTESIAN_POINT('Ctrl Pts',(81.632721838717,1.80582770038043,125.280682882997));
#215050=CARTESIAN_POINT('Ctrl Pts',(81.3542742149043,-3.67113253492515,
126.299383890674));
#215051=CARTESIAN_POINT('Ctrl Pts',(81.0758265910913,-5.77450131542928,
131.457938430015));
#215052=CARTESIAN_POINT('Ctrl Pts',(80.7973789672785,-2.57138548712596,
136.015886888767));
#215053=CARTESIAN_POINT('Ctrl Pts',(80.5189313434656,2.99470798468153,135.784697301496));
#215054=CARTESIAN_POINT('Ctrl Pts',(80.2404837196526,5.80881111818491,130.976821604667));
#215055=CARTESIAN_POINT('Ctrl Pts',(79.9620360958398,3.2849006102757,126.010462685879));
#215056=CARTESIAN_POINT('Ctrl Pts',(79.6835884720269,-2.25767308216064,
125.449461771377));
#215057=CARTESIAN_POINT('Ctrl Pts',(79.4051408482139,-5.72555550555307,
129.809351295171));
#215058=CARTESIAN_POINT('Ctrl Pts',(79.1266932244012,-3.93193212827854,
135.083605777338));
#215059=CARTESIAN_POINT('Ctrl Pts',(78.8482456005881,1.47494478932078,136.425443010422));
#215060=CARTESIAN_POINT('Ctrl Pts',(78.5697979767754,5.526419500593,132.601780129612));
#215061=CARTESIAN_POINT('Ctrl Pts',(78.2913503529625,4.49938467142216,127.126376526057));
#215062=CARTESIAN_POINT('Ctrl Pts',(78.0129027291494,-0.662364863624755,
125.030860623086));
#215063=CARTESIAN_POINT('Ctrl Pts',(77.7344551053368,-5.21543344732299,
128.240909163888));
#215064=CARTESIAN_POINT('Ctrl Pts',(77.4560074815235,-4.97577348101974,
133.806644359053));
#215065=CARTESIAN_POINT('Ctrl Pts',(77.1775598577108,-0.163620765707691,
136.613427465507));
#215066=CARTESIAN_POINT('Ctrl Pts',(76.8991122338979,4.79889143997102,134.081961927395));
#215067=CARTESIAN_POINT('Ctrl Pts',(76.620664610085,5.35145685119646,128.538540905275));
#215068=CARTESIAN_POINT('Ctrl Pts',(76.3422169862721,0.986294849373407,
125.077297507303));
#215069=CARTESIAN_POINT('Ctrl Pts',(76.0637693624593,-4.28522393584178,
126.878945325076));
#215070=CARTESIAN_POINT('Ctrl Pts',(75.7853217386464,-5.61883126884571,
132.287858029448));
#215071=CARTESIAN_POINT('Ctrl Pts',(75.5068741148335,-1.78900716094817,
136.333509085178));
#215072=CARTESIAN_POINT('Ctrl Pts',(75.2284264910206,3.68482713000219,135.298142813091));
#215073=CARTESIAN_POINT('Ctrl Pts',(74.9499788672077,5.77248530229349,130.133210236781));
#215074=CARTESIAN_POINT('Ctrl Pts',(74.6715312433948,2.55551148336137,125.585032072894));
#215075=CARTESIAN_POINT('Ctrl Pts',(74.3930836195819,-3.0098525451033,125.833161863185));
#215076=CARTESIAN_POINT('Ctrl Pts',(74.1146359957691,-5.80930912408932,
130.649580452192));
#215077=CARTESIAN_POINT('Ctrl Pts',(73.8361883719562,-3.27029441856551,
135.608234451746));
#215078=CARTESIAN_POINT('Ctrl Pts',(73.5577407481433,2.273961094856,136.152363079971));
#215079=CARTESIAN_POINT('Ctrl Pts',(73.2792931243304,5.72855745128013,131.781938709691));
#215080=CARTESIAN_POINT('Ctrl Pts',(73.0008455005175,3.91888936556733,126.513167830092));
#215081=CARTESIAN_POINT('Ctrl Pts',(72.7223978767045,-1.49204659871303,
125.187793485758));
#215082=CARTESIAN_POINT('Ctrl Pts',(72.4439502528918,-5.53186462930466,
129.023769950998));
#215083=CARTESIAN_POINT('Ctrl Pts',(72.1655026290786,-4.48816931217651,
134.496022252122));
#215084=CARTESIAN_POINT('Ctrl Pts',(71.8870550052659,0.679934343581693,
136.575817858786));
#215085=CARTESIAN_POINT('Ctrl Pts',(71.6086073814528,5.22321155422762,133.351926212129));
#215086=CARTESIAN_POINT('Ctrl Pts',(71.3301597576401,4.96661251460835,127.786946239566));
#215087=CARTESIAN_POINT('Ctrl Pts',(71.0517121338272,0.145939206574258,
124.994822671498));
#215088=CARTESIAN_POINT('Ctrl Pts',(70.7732645100143,-4.80884510277506,
127.541380664158));
#215089=CARTESIAN_POINT('Ctrl Pts',(70.4948168862015,-5.34453568781766,
133.086457828568));
#215090=CARTESIAN_POINT('Ctrl Pts',(70.2163692623885,-0.968859070839113,
136.534399142713));
#215091=CARTESIAN_POINT('Ctrl Pts',(69.9379216385757,4.29715170084345,134.716714980192));
#215092=CARTESIAN_POINT('Ctrl Pts',(69.6594740147628,5.61428998698222,129.303768287553));
#215093=CARTESIAN_POINT('Ctrl Pts',(69.3810263909498,1.77217004839796,125.269792638185));
#215094=CARTESIAN_POINT('Ctrl Pts',(69.102578767137,-3.69848758934425,126.321814583191));
#215095=CARTESIAN_POINT('Ctrl Pts',(68.8241311433241,-5.77041581364239,
131.493077349239));
#215096=CARTESIAN_POINT('Ctrl Pts',(68.5456835195112,-2.53961380568736,
136.031443084562));
#215097=CARTESIAN_POINT('Ctrl Pts',(68.2672358956983,3.02496922266262,135.76637538989));
#215098=CARTESIAN_POINT('Ctrl Pts',(67.9887882718854,5.80975331334755,130.94145852735));
#215099=CARTESIAN_POINT('Ctrl Pts',(67.7103406480725,3.25565793129432,125.990555383323));
#215100=CARTESIAN_POINT('Ctrl Pts',(67.4318930242597,-2.29022804188655,
125.463304082106));
#215101=CARTESIAN_POINT('Ctrl Pts',(67.1534454004468,-5.73150632843341,
129.844222811859));
#215102=CARTESIAN_POINT('Ctrl Pts',(66.8749977766338,-3.90581029880048,
135.107461279717));
#215103=CARTESIAN_POINT('Ctrl Pts',(66.5965501528209,1.50913458598933,136.416360457212));
#215104=CARTESIAN_POINT('Ctrl Pts',(66.3181025290079,5.53725851157817,132.568105943505));
#215105=CARTESIAN_POINT('Ctrl Pts',(66.0396549051952,4.47691237514338,127.09905563901));
#215106=CARTESIAN_POINT('Ctrl Pts',(65.7612072813823,-0.69749752471975,
125.034999595595));
#215107=CARTESIAN_POINT('Ctrl Pts',(65.4827596575694,-5.23094127401388,
128.272704482416));
#215108=CARTESIAN_POINT('Ctrl Pts',(65.2043120337565,-4.95740553817722,
133.836877679162));
#215109=CARTESIAN_POINT('Ctrl Pts',(64.9258644099437,-0.128256295479839,
136.614315842995));
#215110=CARTESIAN_POINT('Ctrl Pts',(64.6474167861306,4.81875421709505,134.05268898675));
#215111=CARTESIAN_POINT('Ctrl Pts',(64.3689691623179,5.33756501339024,128.506007048888));
#215112=CARTESIAN_POINT('Ctrl Pts',(64.0905215385049,0.951414316927145,
125.071399759827));
#215113=CARTESIAN_POINT('Ctrl Pts',(63.8120739146922,-4.30903965761881,
126.905103428319));
#215114=CARTESIAN_POINT('Ctrl Pts',(63.5336262908791,-5.60969669510319,
132.322033964426));
#215115=CARTESIAN_POINT('Ctrl Pts',(63.2551786670663,-1.75531651870651,
136.344296837232));
#215116=CARTESIAN_POINT('Ctrl Pts',(62.9767310432534,3.71211378640213,135.275628965096));
#215117=CARTESIAN_POINT('Ctrl Pts',(62.6982834194405,5.76829286864752,130.098083915181));
#215118=CARTESIAN_POINT('Ctrl Pts',(62.4198357956276,2.52369260137852,125.569572651222));
#215119=CARTESIAN_POINT('Ctrl Pts',(62.1413881718147,-3.04005787731984,
125.851575794724));
#215120=CARTESIAN_POINT('Ctrl Pts',(61.8629405480017,-5.81014368184488,
130.684946233427));
#215121=CARTESIAN_POINT('Ctrl Pts',(61.5844929241889,-3.24099128405306,
135.628052657436));
#215122=CARTESIAN_POINT('Ctrl Pts',(61.3060453003759,2.306473772557,136.138421747261));
#215123=CARTESIAN_POINT('Ctrl Pts',(61.0275976765631,5.73440210969521,131.747049242268));
#215124=CARTESIAN_POINT('Ctrl Pts',(60.7491500527502,3.89269504914048,126.489391944074));
#215125=CARTESIAN_POINT('Ctrl Pts',(60.4707024289374,-1.5262085928491,125.196980058879));
#215126=CARTESIAN_POINT('Ctrl Pts',(60.1922548051244,-5.54260109744501,
129.057476971348));
#215127=CARTESIAN_POINT('Ctrl Pts',(59.9138071813117,-4.46561396460588,
134.52327461468));
#215128=CARTESIAN_POINT('Ctrl Pts',(59.6353595574987,0.715054244335847,
136.571571973714));
#215129=CARTESIAN_POINT('Ctrl Pts',(59.3569119336859,5.23862253507484,133.320083840384));
#215130=CARTESIAN_POINT('Ctrl Pts',(59.0784643098728,4.94815263701827,127.756768965196));
#215131=CARTESIAN_POINT('Ctrl Pts',(58.80001668606,0.110572196236736,124.994041935407));
#215132=CARTESIAN_POINT('Ctrl Pts',(58.5215690622471,-4.82861869113419,
127.570713924673));
#215133=CARTESIAN_POINT('Ctrl Pts',(58.2431214384343,-5.3305448924898,133.118949252284));
#215134=CARTESIAN_POINT('Ctrl Pts',(57.9646738146213,-0.933960749242644,
136.54019069853));
#215135=CARTESIAN_POINT('Ctrl Pts',(57.6862261908085,4.32088769603949,134.690484511247));
#215136=CARTESIAN_POINT('Ctrl Pts',(57.4077785669955,5.6050514357603,129.269620313377));
#215137=CARTESIAN_POINT('Ctrl Pts',(57.1293309431827,1.73844672800264,125.259107478825));
#215138=CARTESIAN_POINT('Ctrl Pts',(56.8508833193697,-3.72570559494523,
126.3444113781));
#215139=CARTESIAN_POINT('Ctrl Pts',(56.5724356955568,-5.76611648697549,
131.528190747811));
#215140=CARTESIAN_POINT('Ctrl Pts',(56.293988071744,-2.50774801792579,136.046805588895));
#215141=CARTESIAN_POINT('Ctrl Pts',(56.0155404479311,3.05511836929639,135.747869609001));
#215142=CARTESIAN_POINT('Ctrl Pts',(55.7370928241181,5.81048022596477,130.906090369819));
#215143=CARTESIAN_POINT('Ctrl Pts',(55.4586452003054,3.22629461271119,125.97082645809));
#215144=CARTESIAN_POINT('Ctrl Pts',(55.1801975764924,-2.32269813636975,
125.477344307648));
#215145=CARTESIAN_POINT('Ctrl Pts',(54.9017499526795,-5.73724476823917,
129.879129906805));
#215146=CARTESIAN_POINT('Ctrl Pts',(54.6233023288666,-3.87954373808533,
135.131157329118));
#215147=CARTESIAN_POINT('Ctrl Pts',(54.3448547050537,1.54326846112093,136.407069949284));
#215148=CARTESIAN_POINT('Ctrl Pts',(54.0664070812409,5.54789233741261,132.534366401168));
#215149=CARTESIAN_POINT('Ctrl Pts',(53.7879594574279,4.45427418523046,127.071872053402));
#215150=CARTESIAN_POINT('Ctrl Pts',(53.5095118336151,-0.732604339787292,
125.039352353899));
#215151=CARTESIAN_POINT('Ctrl Pts',(53.2310642098022,-5.24625526625226,
128.304593612394));
#215152=CARTESIAN_POINT('Ctrl Pts',(52.9526165859893,-4.93885389684926,
133.866998628235));
#215153=CARTESIAN_POINT('Ctrl Pts',(52.6741689621764,-0.0928870726681018,
136.614988930455));
#215154=CARTESIAN_POINT('Ctrl Pts',(52.3957213383635,4.83843843350925,134.023295678104));
#215155=CARTESIAN_POINT('Ctrl Pts',(52.1172737145507,5.32347539014984,128.473558358838));
#215156=CARTESIAN_POINT('Ctrl Pts',(51.8388260907377,0.91649852947334,125.065714449322));
#215157=CARTESIAN_POINT('Ctrl Pts',(51.5603784669247,-4.33269570634681,
126.931406019971));
#215158=CARTESIAN_POINT('Ctrl Pts',(51.2819308431118,-5.6003542519866,132.356153661459));
#215159=CARTESIAN_POINT('Ctrl Pts',(51.0034832192991,-1.72156083256576,
136.354879304913));
#215160=CARTESIAN_POINT('Ctrl Pts',(50.7250355954861,3.73926288906064,135.252949432607));
#215161=CARTESIAN_POINT('Ctrl Pts',(50.4465879716733,5.76388668878802,130.062983764924));
#215162=CARTESIAN_POINT('Ctrl Pts',(50.1681403478604,2.49178020303801,125.554307206545));
#215163=CARTESIAN_POINT('Ctrl Pts',(49.8896927240475,-3.07015055907373,
125.870173253527));
#215164=CARTESIAN_POINT('Ctrl Pts',(49.6112451002346,-5.81076294258959,
130.720316439607));
#215165=CARTESIAN_POINT('Ctrl Pts',(49.3327974764216,-3.21156805341676,
135.647692119444));
#215166=CARTESIAN_POINT('Ctrl Pts',(49.0543498526089,2.33890098302428,136.124282758954));
#215167=CARTESIAN_POINT('Ctrl Pts',(48.7759022287959,5.74003427773134,131.712124843171));
#215168=CARTESIAN_POINT('Ctrl Pts',(48.497454604983,3.86635648746696,126.465775950806));
#215169=CARTESIAN_POINT('Ctrl Pts',(48.2190069811701,-1.56031403276457,
125.206374415548));
#215170=CARTESIAN_POINT('Ctrl Pts',(47.9405593573573,-5.55313218246346,
129.091248723115));
#215171=CARTESIAN_POINT('Ctrl Pts',(47.6621117335443,-4.44289314206747,
134.550389171513));
#215172=CARTESIAN_POINT('Ctrl Pts',(47.3836641097315,0.750147648492217,
136.567112382502));
#215173=CARTESIAN_POINT('Ctrl Pts',(47.1052164859186,5.25383939683757,133.288148247589));
#215174=CARTESIAN_POINT('Ctrl Pts',(46.8267688621057,4.92950940381243,127.726704620456));
#215175=CARTESIAN_POINT('Ctrl Pts',(46.5483212382927,0.0752010886061242,
124.993476502813));
#215176=CARTESIAN_POINT('Ctrl Pts',(46.2698736144798,-4.84821335325179,
127.600167009156));
#215177=CARTESIAN_POINT('Ctrl Pts',(45.991425990667,-5.31635657186091,133.151354908068));
#215178=CARTESIAN_POINT('Ctrl Pts',(45.7129783668541,-0.899027819386881,
136.545769711054));
#215179=CARTESIAN_POINT('Ctrl Pts',(45.4345307430412,4.344463579153,134.664110040551));
#215180=CARTESIAN_POINT('Ctrl Pts',(45.1560831192283,5.5956051872961,129.235529209567));
#215181=CARTESIAN_POINT('Ctrl Pts',(44.8776354954154,1.70465898882477,125.248627800858));
#215182=CARTESIAN_POINT('Ctrl Pts',(44.5991878716026,-3.7527855431554,126.367173438067));
#215183=CARTESIAN_POINT('Ctrl Pts',(44.3207402477896,-5.76160349474165,
131.563277324591));
#215184=CARTESIAN_POINT('Ctrl Pts',(44.0422926239769,-2.47578930463884,
136.0619738325));
#215185=CARTESIAN_POINT('Ctrl Pts',(43.7638450001637,3.08515430739569,135.72918064457));
#215186=CARTESIAN_POINT('Ctrl Pts',(43.485397376351,5.8109918291003,130.870718442656));
#215187=CARTESIAN_POINT('Ctrl Pts',(43.206949752538,3.19681174259461,125.951276641244));
#215188=CARTESIAN_POINT('Ctrl Pts',(42.9285021287252,-2.3550821624196,125.491581927739));
#215189=CARTESIAN_POINT('Ctrl Pts',(42.6500545049123,-5.74277061233009,
129.914071286517));
#215190=CARTESIAN_POINT('Ctrl Pts',(42.3716068810994,-3.85313341945026,
135.154693047476));
#215191=CARTESIAN_POINT('Ctrl Pts',(42.0931592572865,1.57734514987214,136.397571830902));
#215192=CARTESIAN_POINT('Ctrl Pts',(41.8147116334736,5.5583205840564,132.50056275283));
#215193=CARTESIAN_POINT('Ctrl Pts',(41.5362640096606,4.43147094054935,127.04482677653));
#215194=CARTESIAN_POINT('Ctrl Pts',(41.2578163858478,-0.767684007931795,
125.043918736703));
#215195=CARTESIAN_POINT('Ctrl Pts',(40.9793687620349,-5.26137485657243,
128.336575372158));
#215196=CARTESIAN_POINT('Ctrl Pts',(40.700921138222,-4.9201192444739,133.897006090131));
#215197=CARTESIAN_POINT('Ctrl Pts',(40.4224735144091,-0.0575144078915333,
136.615446702946));
#215198=CARTESIAN_POINT('Ctrl Pts',(40.1440258905964,4.85794335980812,133.993783090635));
#215199=CARTESIAN_POINT('Ctrl Pts',(39.8655782667833,5.30918850357096,128.441196037522));
#215200=CARTESIAN_POINT('Ctrl Pts',(39.5871306429705,0.8815487808295,125.060241786462));
#215201=CARTESIAN_POINT('Ctrl Pts',(39.3086830191576,-4.35619120544207,
126.957852125381));
#215202=CARTESIAN_POINT('Ctrl Pts',(39.0302353953447,-5.59080428568363,
132.39021585623));
#215203=CARTESIAN_POINT('Ctrl Pts',(38.7517877715318,-1.6877413533555,136.365256096082));
#215204=CARTESIAN_POINT('Ctrl Pts',(38.4733401477189,3.76627343195761,135.230105056025));
#215205=CARTESIAN_POINT('Ctrl Pts',(38.194892523906,5.7592669259876,130.027911086658));
#215206=CARTESIAN_POINT('Ctrl Pts',(37.9164449000932,2.45977547086574,125.539236304527));
#215207=CARTESIAN_POINT('Ctrl Pts',(37.6379972762802,-3.10012947526937,
125.888953550457));
#215208=CARTESIAN_POINT('Ctrl Pts',(37.3595496524674,-5.81116688337655,
130.755689760074));
#215209=CARTESIAN_POINT('Ctrl Pts',(37.0811020286545,-3.18202581694541,
135.667152110023));
#215210=CARTESIAN_POINT('Ctrl Pts',(36.8026544048415,2.3712415246555,136.109946638975));
#215211=CARTESIAN_POINT('Ctrl Pts',(36.5242067810287,5.74545374668639,131.677166806538));
#215212=CARTESIAN_POINT('Ctrl Pts',(36.2457591572158,3.83987465653194,126.442320725389));
#215213=CARTESIAN_POINT('Ctrl Pts',(35.9673115334029,-1.59436165466975,
125.215976207654));
#215214=CARTESIAN_POINT('Ctrl Pts',(35.6888639095901,-5.56345749412674,
129.125083954872));
#215215=CARTESIAN_POINT('Ctrl Pts',(35.4104162857771,-4.42000768648982,
134.57736491788));
#215216=CARTESIAN_POINT('Ctrl Pts',(35.1319686619643,0.785213255651605,
136.562439250406));
#215217=CARTESIAN_POINT('Ctrl Pts',(34.8535210381513,5.26886157564935,133.25612061713));
#215218=CARTESIAN_POINT('Ctrl Pts',(34.5750734143385,4.91068350582282,127.69675431939));
#215219=CARTESIAN_POINT('Ctrl Pts',(34.2966257905255,0.0398271943713243,
124.993126394665));
#215220=CARTESIAN_POINT('Ctrl Pts',(34.0181781667127,-4.86762836304081,
127.629738826211));
#215221=CARTESIAN_POINT('Ctrl Pts',(33.7397305428998,-5.30197125168398,
133.183673595116));
#215222=CARTESIAN_POINT('Ctrl Pts',(33.4612829190869,-0.864061575724654,
136.551135973552));
#215223=CARTESIAN_POINT('Ctrl Pts',(33.182835295274,4.36787847657091,134.637592545421));
#215224=CARTESIAN_POINT('Ctrl Pts',(32.9043876714611,5.58595159162396,129.201496239381));
#215225=CARTESIAN_POINT('Ctrl Pts',(32.6259400476482,1.67080808288091,125.238353992614));
#215226=CARTESIAN_POINT('Ctrl Pts',(32.3474924238352,-3.77972643051725,
126.390099919638));
#215227=CARTESIAN_POINT('Ctrl Pts',(32.0690448000224,-5.75687700417149,
131.598335779433));
#215228=CARTESIAN_POINT('Ctrl Pts',(31.7905971762095,-2.44373885006871,
136.076947253315));
#215229=CARTESIAN_POINT('Ctrl Pts',(31.5121495523967,3.11507592396733,135.71030918912));
#215230=CARTESIAN_POINT('Ctrl Pts',(31.2337019285837,5.81128810379662,130.835344056578));
#215231=CARTESIAN_POINT('Ctrl Pts',(30.9552543047708,3.16721041344351,125.931906657209));
#215232=CARTESIAN_POINT('Ctrl Pts',(30.676806680958,-2.38737892003384,125.506016414799));
#215233=CARTESIAN_POINT('Ctrl Pts',(30.398359057145,-5.74808365594406,129.949045656226));
#215234=CARTESIAN_POINT('Ctrl Pts',(30.1199114333322,-3.82658032153943,
135.178067562667));
#215235=CARTESIAN_POINT('Ctrl Pts',(29.8414638095193,1.61136338951851,136.387866454021));
#215236=CARTESIAN_POINT('Ctrl Pts',(29.5630161857064,5.56854286508694,132.466696251098));
#215237=CARTESIAN_POINT('Ctrl Pts',(29.2845685618935,4.40850348608286,127.017920810568));
#215238=CARTESIAN_POINT('Ctrl Pts',(29.0061209380806,-0.802735229263066,
125.048698574801));
#215239=CARTESIAN_POINT('Ctrl Pts',(28.7276733142678,-5.27629948471241,
128.368648576612));
#215240=CARTESIAN_POINT('Ctrl Pts',(28.4492256904548,-4.90120227527057,
133.926898952911));
#215241=CARTESIAN_POINT('Ctrl Pts',(28.170778066642,-0.0221396118974229,
136.615689143506));
#215242=CARTESIAN_POINT('Ctrl Pts',(27.892330442829,4.87726827322928,133.964152317942));
#215243=CARTESIAN_POINT('Ctrl Pts',(27.6138828190162,5.29470488305963,128.408921284139));
#215244=CARTESIAN_POINT('Ctrl Pts',(27.3354351952032,0.846566366071392,
125.054981974037));
#215245=CARTESIAN_POINT('Ctrl Pts',(27.0569875713904,-4.37952528427021,
126.984440764576));
#215246=CARTESIAN_POINT('Ctrl Pts',(26.7785399475775,-5.58104715007188,
132.424219286554));
#215247=CARTESIAN_POINT('Ctrl Pts',(26.5000923237646,-1.65385933426847,
136.375426826225));
#215248=CARTESIAN_POINT('Ctrl Pts',(26.2216446999517,3.79314441420758,135.207096681855));
#215249=CARTESIAN_POINT('Ctrl Pts',(25.9431970761388,5.75443375143326,129.992867180015));
#215250=CARTESIAN_POINT('Ctrl Pts',(25.6647494523259,2.42767959080881,125.524360503627));
#215251=CARTESIAN_POINT('Ctrl Pts',(25.3863018285131,-3.12999351502748,
125.907915989602));
#215252=CARTESIAN_POINT('Ctrl Pts',(25.1078542047001,-5.81135548923757,
130.791064884058));
#215253=CARTESIAN_POINT('Ctrl Pts',(24.8294065808873,-3.152365669337,135.686431908074));
#215254=CARTESIAN_POINT('Ctrl Pts',(24.5509589570743,2.40349419906,136.095413918554));
#215255=CARTESIAN_POINT('Ctrl Pts',(24.2725113332615,5.75066031573997,131.64217642775));
#215256=CARTESIAN_POINT('Ctrl Pts',(23.9940637094486,3.81325053762949,126.419027136963));
#215257=CARTESIAN_POINT('Ctrl Pts',(23.7156160856357,-1.62835019691723,
125.2257850794));
#215258=CARTESIAN_POINT('Ctrl Pts',(23.4371684618228,-5.57357664982666,
129.158981412844));
#215259=CARTESIAN_POINT('Ctrl Pts',(23.1587208380098,-4.39695844590187,
134.604200854185));
#215260=CARTESIAN_POINT('Ctrl Pts',(22.880273214197,0.820249766445046,136.557552750588));
#215261=CARTESIAN_POINT('Ctrl Pts',(22.6018255903841,5.28368851485763,133.224002135804));
#215262=CARTESIAN_POINT('Ctrl Pts',(22.3233779665712,4.89167564065013,127.666919171818));
#215263=CARTESIAN_POINT('Ctrl Pts',(22.0449303427584,0.00445182432539013,
124.992991623939));
#215264=CARTESIAN_POINT('Ctrl Pts',(21.7664827189454,-4.88686300107076,
127.659428280044));
#215265=CARTESIAN_POINT('Ctrl Pts',(21.4880350951325,-5.28738946501251,
133.215904115845));
#215266=CARTESIAN_POINT('Ctrl Pts',(21.2095874713197,-0.829063313942982,
136.556289287176));
#215267=CARTESIAN_POINT('Ctrl Pts',(20.9311398475068,4.39113152064558,134.610933008472));
#215268=CARTESIAN_POINT('Ctrl Pts',(20.6526922236938,5.57609100646137,129.167522663925));
#215269=CARTESIAN_POINT('Ctrl Pts',(20.374244599881,1.6368952645291,125.228286434793));
#215270=CARTESIAN_POINT('Ctrl Pts',(20.0957969760681,-3.80652725872624,
126.413189973261));
#215271=CARTESIAN_POINT('Ctrl Pts',(19.8173493522552,-5.75193719040684,
131.633364813234));
#215272=CARTESIAN_POINT('Ctrl Pts',(19.5389017284423,-2.41159784185683,
136.091725296493));
#215273=CARTESIAN_POINT('Ctrl Pts',(19.2604541046294,3.14488211025528,135.691255941942));
#215274=CARTESIAN_POINT('Ctrl Pts',(18.9820064808165,5.81136903907515,130.799968522399));
#215275=CARTESIAN_POINT('Ctrl Pts',(18.7035588570036,3.13749172214556,125.912717223747));
#215276=CARTESIAN_POINT('Ctrl Pts',(18.4251112331907,-2.41958721244422,
125.52064723395));
#215277=CARTESIAN_POINT('Ctrl Pts',(18.1466636093778,-5.75318370220431,
129.984051719947));
#215278=CARTESIAN_POINT('Ctrl Pts',(17.868215985565,-3.79988542828747,135.201280008538));
#215279=CARTESIAN_POINT('Ctrl Pts',(17.589768361752,1.64532191950215,136.377954178279));
#215280=CARTESIAN_POINT('Ctrl Pts',(17.3113207379392,5.57855880171371,132.432768150908));
#215281=CARTESIAN_POINT('Ctrl Pts',(17.0328731141263,4.38537267289848,126.991155152525));
#215282=CARTESIAN_POINT('Ctrl Pts',(16.7544254903134,-0.83775670494522,
125.053691691071));
#215283=CARTESIAN_POINT('Ctrl Pts',(16.4759778665005,-5.29102859763445,
128.400812037271));
#215284=CARTESIAN_POINT('Ctrl Pts',(16.1975302426876,-4.88210369021464,
133.956676108886));
#215285=CARTESIAN_POINT('Ctrl Pts',(15.9190826188747,0.013236004487936,
136.61571624315));
#215286=CARTESIAN_POINT('Ctrl Pts',(15.6406349950618,4.89641245768097,133.934404458007));
#215287=CARTESIAN_POINT('Ctrl Pts',(15.3621873712489,5.2800250653117,128.376735294641));
#215288=CARTESIAN_POINT('Ctrl Pts',(15.0837397474361,0.811552581485459,
125.049935206953));
#215289=CARTESIAN_POINT('Ctrl Pts',(14.8052921236231,-4.40269707817821,
127.011170952307));
#215290=CARTESIAN_POINT('Ctrl Pts',(14.5268444998103,-5.57108320670569,
132.458162692417));
#215291=CARTESIAN_POINT('Ctrl Pts',(14.2483968759974,-1.6199160308156,136.385391118461));
#215292=CARTESIAN_POINT('Ctrl Pts',(13.9699492521845,3.81987484009636,135.18392516268));
#215293=CARTESIAN_POINT('Ctrl Pts',(13.6915016283715,5.74938734422005,129.95785334356));
#215294=CARTESIAN_POINT('Ctrl Pts',(13.4130540045587,2.39549375219187,125.509680355073));
#215295=CARTESIAN_POINT('Ctrl Pts',(13.1346063807458,-3.15974157172482,
125.927059868305));
#215296=CARTESIAN_POINT('Ctrl Pts',(12.8561587569329,-5.81132875318382,
130.82644050072));
#215297=CARTESIAN_POINT('Ctrl Pts',(12.57771113312,-3.12258870965941,135.705530799178));
#215298=CARTESIAN_POINT('Ctrl Pts',(12.2992635093071,2.43565781110307,136.080685136208));
#215299=CARTESIAN_POINT('Ctrl Pts',(12.0208158854942,5.75565379196074,131.607155003388));
#215300=CARTESIAN_POINT('Ctrl Pts',(11.7423682616813,3.78648511732596,126.395896048684));
#215301=CARTESIAN_POINT('Ctrl Pts',(11.4639206378685,-1.66227840004959,
125.235800667314));
#215302=CARTESIAN_POINT('Ctrl Pts',(11.1854730140555,-5.58348927459409,
129.192939840948));
#215303=CARTESIAN_POINT('Ctrl Pts',(10.9070253902426,-4.37374627440173,
134.630895986013));
#215304=CARTESIAN_POINT('Ctrl Pts',(10.6285777664298,0.855255882581734,
136.552453064119));
#215305=CARTESIAN_POINT('Ctrl Pts',(10.3501301426169,5.29831966504511,133.19179399377));
#215306=CARTESIAN_POINT('Ctrl Pts',(10.071682518804,4.87248651263752,127.637200283293));
#215307=CARTESIAN_POINT('Ctrl Pts',(9.79323489499104,-0.0309237106847325,
124.993072195629));
#215308=CARTESIAN_POINT('Ctrl Pts',(9.51478727117816,-4.90591655459505,
127.689234270502));
#215309=CARTESIAN_POINT('Ctrl Pts',(9.23633964736526,-5.27261175218,133.248045275945));
#215310=CARTESIAN_POINT('Ctrl Pts',(8.95789202355236,-0.794034330915497,
136.561229460968));
#215311=CARTESIAN_POINT('Ctrl Pts',(8.67944439973947,4.41422184972672,134.584132417584));
#215312=CARTESIAN_POINT('Ctrl Pts',(8.40099677592661,5.56602379719609,129.1336097421));
#215313=CARTESIAN_POINT('Ctrl Pts',(8.12254915211368,1.60292179042129,125.218425500451));
#215314=CARTESIAN_POINT('Ctrl Pts',(7.84410152830078,-3.83318703466779,
126.436442743329));
#215315=CARTESIAN_POINT('Ctrl Pts',(7.56565390448795,-5.74678423649425,
131.668363127979));
#215316=CARTESIAN_POINT('Ctrl Pts',(7.28720628067502,-2.37936747100029,
136.106307414428));
#215317=CARTESIAN_POINT('Ctrl Pts',(7.00875865686212,3.17457176177998,135.672021609062));
#215318=CARTESIAN_POINT('Ctrl Pts',(6.73031103304925,5.81123463193681,130.764593150968));
#215319=CARTESIAN_POINT('Ctrl Pts',(6.45186340923634,3.10765676993803,125.89370905193));
#215320=CARTESIAN_POINT('Ctrl Pts',(6.17341578542346,-2.45170584616043,
125.535473843045));
#215321=CARTESIAN_POINT('Ctrl Pts',(5.89496816161054,-5.75807056212669,
130.019088180515));
#215322=CARTESIAN_POINT('Ctrl Pts',(5.61652053779771,-3.77304972888379,
135.224329524944));
#215323=CARTESIAN_POINT('Ctrl Pts',(5.33807291398477,1.67921948147701,136.367835370977));
#215324=CARTESIAN_POINT('Ctrl Pts',(5.05962529017187,5.58836802279258,132.398779709476));
#215325=CARTESIAN_POINT('Ctrl Pts',(4.781177666359,4.36207935811697,126.964530794212));
#215326=CARTESIAN_POINT('Ctrl Pts',(4.50273004254611,-0.872747137244579,
125.058897900495));
#215327=CARTESIAN_POINT('Ctrl Pts',(4.2242824187332,-5.30556164954619,128.433064562307));
#215328=CARTESIAN_POINT('Ctrl Pts',(3.94583479492031,-4.86282419701095,
133.986336454649));
#215329=CARTESIAN_POINT('Ctrl Pts',(3.66738717110745,0.0486111304084952,
136.615528000873));
#215330=CARTESIAN_POINT('Ctrl Pts',(3.38893954729453,4.91537520376836,133.904540613147));
#215331=CARTESIAN_POINT('Ctrl Pts',(3.11049192348162,5.26514959429328,128.344639261694));
#215332=CARTESIAN_POINT('Ctrl Pts',(2.83204429966877,0.776508724519974,
125.045101672218));
#215333=CARTESIAN_POINT('Ctrl Pts',(2.55359667585587,-4.42570572852705,
127.038041698076));
#215334=CARTESIAN_POINT('Ctrl Pts',(2.27514905204296,-5.56091282480238,
132.492044816037));
#215335=CARTESIAN_POINT('Ctrl Pts',(1.99670142823006,-1.58591270077849,
136.395148603559));
#215336=CARTESIAN_POINT('Ctrl Pts',(1.7182538044172,3.84646371911817,135.160591357131));
#215337=CARTESIAN_POINT('Ctrl Pts',(1.43980618060429,5.7441278913444,129.922870874744));
#215338=CARTESIAN_POINT('Ctrl Pts',(1.16135855679139,2.36321914767325,125.495196402842));
#215339=CARTESIAN_POINT('Ctrl Pts',(0.882910932978526,-3.18937254303613,
125.946384477181));
#215340=CARTESIAN_POINT('Ctrl Pts',(0.604463309165634,-5.81108667620601,
130.861815299204));
#215341=CARTESIAN_POINT('Ctrl Pts',(0.326015685352703,-3.09269604130886,
135.724448075619));
#215342=CARTESIAN_POINT('Ctrl Pts',(0.0475680615398608,2.46773116894999,
136.065760837718));
#215343=CARTESIAN_POINT('Ctrl Pts',(-0.230879562273037,5.76043399031358,
131.572103831187));
#215344=CARTESIAN_POINT('Ctrl Pts',(-0.509327186085944,3.75957938742415,
126.37292831768));
#215345=CARTESIAN_POINT('Ctrl Pts',(-0.787774809898847,-1.69614500684454,
125.246022600264));
#215346=CARTESIAN_POINT('Ctrl Pts',(-1.06622243371171,-5.59319500111311,
129.226957980841));
#215347=CARTESIAN_POINT('Ctrl Pts',(-1.34467005752462,-4.35037203212501,
134.657449324165));
#215348=CARTESIAN_POINT('Ctrl Pts',(-1.62311768133752,0.890230306896913,
136.547140379971));
#215349=CARTESIAN_POINT('Ctrl Pts',(-1.90156530515039,5.31275448404895,
133.159497384516));
#215350=CARTESIAN_POINT('Ctrl Pts',(-2.18001292896328,4.85311683284533,
127.607598755059));
#215351=CARTESIAN_POINT('Ctrl Pts',(-2.4584605527762,-0.0662980998053887,
124.993368106748));
#215352=CARTESIAN_POINT('Ctrl Pts',(-2.73690817658909,-4.92478831757726,
127.719155693111));
#215353=CARTESIAN_POINT('Ctrl Pts',(-3.01535580040196,-5.25763866077998,
133.280095884409));
#215354=CARTESIAN_POINT('Ctrl Pts',(-3.29380342421486,-0.758975924653704,
136.565956311869));
#215355=CARTESIAN_POINT('Ctrl Pts',(-3.57225104802777,4.43714860819409,
134.557191765862));
#215356=CARTESIAN_POINT('Ctrl Pts',(-3.85069867184063,5.55575033687191,
129.099758730564));
#215357=CARTESIAN_POINT('Ctrl Pts',(-4.12914629565353,1.56888891945708,
125.208771554989));
#215358=CARTESIAN_POINT('Ctrl Pts',(-4.40759391946644,-3.85970477045413,
126.459857368199));
#215359=CARTESIAN_POINT('Ctrl Pts',(-4.68604154327934,-5.74141833337845,
131.703329426794));
#215360=CARTESIAN_POINT('Ctrl Pts',(-4.96448916709218,-2.34704893180687,
136.120693066776));
#215361=CARTESIAN_POINT('Ctrl Pts',(-5.24293679090511,3.20414377838073,
135.652606903212));
#215362=CARTESIAN_POINT('Ctrl Pts',(-5.52138441471801,5.81088488736209,
130.729219253137));
#215363=CARTESIAN_POINT('Ctrl Pts',(-5.79983203853088,3.07770666236606,
125.874882846113));
#215364=CARTESIAN_POINT('Ctrl Pts',(-6.07827966234377,-2.48373363101511,
125.550495692676));
#215365=CARTESIAN_POINT('Ctrl Pts',(-6.35672728615668,-5.7627440546269,
130.054153739642));
#215366=CARTESIAN_POINT('Ctrl Pts',(-6.63517490996957,-3.74607421773465,
135.247215257776));
#215367=CARTESIAN_POINT('Ctrl Pts',(-6.91362253378244,1.71305481935644,
136.357510407073));
#215368=CARTESIAN_POINT('Ctrl Pts',(-7.19207015759534,5.59797016483923,
132.36473218626));
#215369=CARTESIAN_POINT('Ctrl Pts',(-7.47051778140826,4.33862440488076,
126.938048722207));
#215370=CARTESIAN_POINT('Ctrl Pts',(-7.74896540522111,-0.907705229577551,
125.064317010151));
#215371=CARTESIAN_POINT('Ctrl Pts',(-8.027413029034,-5.31989810191992,128.46540495659));
#215372=CARTESIAN_POINT('Ctrl Pts',(-8.30586065284694,-4.84336451006833,
134.015878891129));
#215373=CARTESIAN_POINT('Ctrl Pts',(-8.58430827665978,0.0839844550257475,
136.615124423653));
#215374=CARTESIAN_POINT('Ctrl Pts',(-8.86275590047269,4.93415580881975,
133.874561889976));
#215375=CARTESIAN_POINT('Ctrl Pts',(-9.14120352428557,5.25007902122049,
128.312634374625));
#215376=CARTESIAN_POINT('Ctrl Pts',(-9.4196511480985,0.741436093738357,
125.040481548942));
#215377=CARTESIAN_POINT('Ctrl Pts',(-9.69809877191133,-4.44855038272257,
127.065052006178));
#215378=CARTESIAN_POINT('Ctrl Pts',(-9.97654639572428,-5.5505363812293,
132.525864401898));
#215379=CARTESIAN_POINT('Ctrl Pts',(-10.2549940195371,-1.55185060416301,
136.404698919952));
#215380=CARTESIAN_POINT('Ctrl Pts',(-10.53344164335,3.87291006601234,135.137096129849));
#215381=CARTESIAN_POINT('Ctrl Pts',(-10.8118892671629,5.7386555876974,129.887921069854));
#215382=CARTESIAN_POINT('Ctrl Pts',(-11.0903368909758,2.33085697319978,
125.480909183646));
#215383=CARTESIAN_POINT('Ctrl Pts',(-11.3687845147887,-3.21888533097506,
125.965889100148));
#215384=CARTESIAN_POINT('Ctrl Pts',(-11.6472321386015,-5.81062926727439,
130.897187968684));
#215385=CARTESIAN_POINT('Ctrl Pts',(-11.9256797624145,-3.06268877196916,
135.743183036409));
#215386=CARTESIAN_POINT('Ctrl Pts',(-12.2041273862274,2.49971308411117,
136.050641576106));
#215387=CARTESIAN_POINT('Ctrl Pts',(-12.4825750100403,5.76500073366654,
131.537024209977));
#215388=CARTESIAN_POINT('Ctrl Pts',(-12.7610226338531,3.73253434492532,
126.350124795028));
#215389=CARTESIAN_POINT('Ctrl Pts',(-13.039470257666,-1.7299487623625,125.256450499474));
#215390=CARTESIAN_POINT('Ctrl Pts',(-13.3179178814789,-5.60269346973446,
129.261034571969));
#215391=CARTESIAN_POINT('Ctrl Pts',(-13.5963655052918,-4.32683658521273,
134.683859884699));
#215392=CARTESIAN_POINT('Ctrl Pts',(-13.8748131291047,0.925171743400955,
136.541614895008));
#215393=CARTESIAN_POINT('Ctrl Pts',(-14.1532607529176,5.3269924369816,133.127113504801));
#215394=CARTESIAN_POINT('Ctrl Pts',(-14.4317083767304,4.83356731902416,
127.578115684011));
#215395=CARTESIAN_POINT('Ctrl Pts',(-14.7101560005434,-0.101670032225581,
124.99387934633));
#215396=CARTESIAN_POINT('Ctrl Pts',(-14.9886036243562,-4.94347759071707,
127.749191439124));
#215397=CARTESIAN_POINT('Ctrl Pts',(-15.2670512481692,-5.24247074564602,
133.312054753593));
#215398=CARTESIAN_POINT('Ctrl Pts',(-15.545498871982,-0.723889394260118,
136.570469664722));
#215399=CARTESIAN_POINT('Ctrl Pts',(-15.823946495795,4.45991094648802,134.530112051601));
#215400=CARTESIAN_POINT('Ctrl Pts',(-16.1023941196078,5.54527100617588,
129.065970883678));
#215401=CARTESIAN_POINT('Ctrl Pts',(-16.3808417434207,1.53479791273714,
125.199324956138));
#215402=CARTESIAN_POINT('Ctrl Pts',(-16.6592893672336,-3.88607948346057,
126.483432980235));
#215403=CARTESIAN_POINT('Ctrl Pts',(-16.9377369910465,-5.73583967989507,
131.738262413989));
#215404=CARTESIAN_POINT('Ctrl Pts',(-17.2161846148594,-2.31464342185212,
136.134881720468));
#215405=CARTESIAN_POINT('Ctrl Pts',(-17.4946322386723,3.23359706425542,
135.633012543814));
#215406=CARTESIAN_POINT('Ctrl Pts',(-17.7730798624852,5.81031981831091,
130.693848139697));
#215407=CARTESIAN_POINT('Ctrl Pts',(-18.0515274862981,3.04764250924188,
125.856239303907));
#215408=CARTESIAN_POINT('Ctrl Pts',(-18.3299751101109,-2.51566938020671,
125.565712226204));
#215409=CARTESIAN_POINT('Ctrl Pts',(-18.6084227339239,-5.76720400652691,
130.089247097961));
#215410=CARTESIAN_POINT('Ctrl Pts',(-18.8868703577367,-3.71895989442774,
135.269936358996));
#215411=CARTESIAN_POINT('Ctrl Pts',(-19.1653179815497,1.74682667935956,
136.346979669161));
#215412=CARTESIAN_POINT('Ctrl Pts',(-19.4437656053625,5.60736487204277,
132.330626842902));
#215413=CARTESIAN_POINT('Ctrl Pts',(-19.7222132291754,4.31500868232164,
126.91170991781));
#215414=CARTESIAN_POINT('Ctrl Pts',(-20.0006608529883,-0.942629686559699,
125.069948819234));
#215415=CARTESIAN_POINT('Ctrl Pts',(-20.2791084768012,-5.33403742351306,
128.497832021735));
#215416=CARTESIAN_POINT('Ctrl Pts',(-20.5575561006141,-4.82372535047263,
134.045302323618));
#215417=CARTESIAN_POINT('Ctrl Pts',(-20.836003724427,0.119354667568119,
136.614505526443));
#215418=CARTESIAN_POINT('Ctrl Pts',(-21.1144513482399,4.95275357691331,
133.844469399368));
#215419=CARTESIAN_POINT('Ctrl Pts',(-21.3928989720528,5.23481390453873,
128.280721819388));
#215420=CARTESIAN_POINT('Ctrl Pts',(-21.6713465958657,0.706335988769417,
125.036075008324));
#215421=CARTESIAN_POINT('Ctrl Pts',(-21.9497942196786,-4.47123019424771,
127.092200875735));
#215422=CARTESIAN_POINT('Ctrl Pts',(-22.2282418434914,-5.53995426048939,
132.559620196804));
#215423=CARTESIAN_POINT('Ctrl Pts',(-22.5066894673044,-1.5177310031529,
136.41404171375));
#215424=CARTESIAN_POINT('Ctrl Pts',(-22.7851370911172,3.89921290079955,
135.11344035146));
#215425=CARTESIAN_POINT('Ctrl Pts',(-23.0635847149301,5.73297063605735,
129.853005223969));
#215426=CARTESIAN_POINT('Ctrl Pts',(-23.342032338743,2.298408427964,125.466819226899));
#215427=CARTESIAN_POINT('Ctrl Pts',(-23.6204799625559,-3.24827884193431,
125.985573014458));
#215428=CARTESIAN_POINT('Ctrl Pts',(-23.8989275863688,-5.80995654333829,
130.932557198412));
#215429=CARTESIAN_POINT('Ctrl Pts',(-24.1773752101816,-3.03256801357094,
135.761734987319));
#215430=CARTESIAN_POINT('Ctrl Pts',(-24.4558228339946,2.53160237148462,
136.035327911625));
#215431=CARTESIAN_POINT('Ctrl Pts',(-24.7342704578075,5.76935385279724,
131.501917439649));
#215432=CARTESIAN_POINT('Ctrl Pts',(-25.0127180816204,3.70535099199371,
126.327486325724));
#215433=CARTESIAN_POINT('Ctrl Pts',(-25.2911657054332,-1.76368841399288,
125.267083978533));
#215434=CARTESIAN_POINT('Ctrl Pts',(-25.5696133292462,-5.61198432848891,
129.295168351611));
#215435=CARTESIAN_POINT('Ctrl Pts',(-25.8480609530591,-4.30314080577957,
134.71012668896));
#215436=CARTESIAN_POINT('Ctrl Pts',(-26.1265085768719,0.960078897325804,
136.535876813977));
#215437=CARTESIAN_POINT('Ctrl Pts',(-26.4049562006848,5.3410329962505,133.094643554625));
#215438=CARTESIAN_POINT('Ctrl Pts',(-26.6834038244978,4.81383869558843,
127.548752162656));
#215439=CARTESIAN_POINT('Ctrl Pts',(-26.9618514483106,-0.137038197225328,
124.994605895435));
#215440=CARTESIAN_POINT('Ctrl Pts',(-27.2402990721235,-4.96198368147699,
127.779340395554));
#215441=CARTESIAN_POINT('Ctrl Pts',(-27.5187466959364,-5.22710856883054,
133.343920699249));
#215442=CARTESIAN_POINT('Ctrl Pts',(-27.7971943197493,-0.688776039878604,
136.574769352283));
#215443=CARTESIAN_POINT('Ctrl Pts',(-28.0756419435621,4.48250802114168,
134.502894278251));
#215444=CARTESIAN_POINT('Ctrl Pts',(-28.3540895673751,5.53458619342344,
129.032247453463));
#215445=CARTESIAN_POINT('Ctrl Pts',(-28.632537191188,1.50065003351598,125.190086053944));
#215446=CARTESIAN_POINT('Ctrl Pts',(-28.9109848150008,-3.91231019636288,
126.507168705834));
#215447=CARTESIAN_POINT('Ctrl Pts',(-29.1894324388138,-5.73004848276283,
131.773160795109));
#215448=CARTESIAN_POINT('Ctrl Pts',(-29.4678800626266,-2.28215214193419,
136.148872849742));
#215449=CARTESIAN_POINT('Ctrl Pts',(-29.7463276864396,3.26293052800175,
135.613239256942));
#215450=CARTESIAN_POINT('Ctrl Pts',(-30.0247753102524,5.80953944572202,
130.658481121338));
#215451=CARTESIAN_POINT('Ctrl Pts',(-30.3032229340653,3.01746542460398,
125.837779116156));
#215452=CARTESIAN_POINT('Ctrl Pts',(-30.5816705578782,-2.54751191034413,
125.581122879776));
#215453=CARTESIAN_POINT('Ctrl Pts',(-30.8601181816911,-5.77145025256159,
130.124366955075));
#215454=CARTESIAN_POINT('Ctrl Pts',(-31.138565805504,-3.69170776369427,
135.292491986665));
#215455=CARTESIAN_POINT('Ctrl Pts',(-31.4170134293169,1.78053381005746,
136.336243547461));
#215456=CARTESIAN_POINT('Ctrl Pts',(-31.6954610531298,5.6165517962788,132.296464943187));
#215457=CARTESIAN_POINT('Ctrl Pts',(-31.9739086769427,4.29123306552915,
126.885515357016));
#215458=CARTESIAN_POINT('Ctrl Pts',(-32.2523563007555,-0.977519214052166,
125.075793119056));
#215459=CARTESIAN_POINT('Ctrl Pts',(-32.5308039245685,-5.34797909038788,
128.530344556146));
#215460=CARTESIAN_POINT('Ctrl Pts',(-32.8092515483813,-4.80390744596015,
134.07460566182));
#215461=CARTESIAN_POINT('Ctrl Pts',(-33.0876991721943,0.154720457379397,
136.613671332177));
#215462=CARTESIAN_POINT('Ctrl Pts',(-33.3661467960071,4.9711678189017,133.814264256411));
#215463=CARTESIAN_POINT('Ctrl Pts',(-33.64459441982,5.21935480990263,128.248902778514));
#215464=CARTESIAN_POINT('Ctrl Pts',(-33.9230420436329,0.671209710260644,
125.031882213649));
#215465=CARTESIAN_POINT('Ctrl Pts',(-34.2014896674458,-4.49374432269368,
127.119487300736));
#215466=CARTESIAN_POINT('Ctrl Pts',(-34.4799372912587,-5.52916685470707,
132.59331094992));
#215467=CARTESIAN_POINT('Ctrl Pts',(-34.7583849150716,-1.48355516206214,
136.423176638752));
#215468=CARTESIAN_POINT('Ctrl Pts',(-35.0368325388844,3.92537124881898,
135.089624898536));
#215469=CARTESIAN_POINT('Ctrl Pts',(-35.3152801626974,5.72707324708195,
129.818124630907));
#215470=CARTESIAN_POINT('Ctrl Pts',(-35.5937277865103,2.26587471435868,
125.45292705471));
#215471=CARTESIAN_POINT('Ctrl Pts',(-35.8721754103231,-3.27755198672651,
126.005435490714));
#215472=CARTESIAN_POINT('Ctrl Pts',(-36.1506230341361,-5.80906852932597,
130.967921677768));
#215473=CARTESIAN_POINT('Ctrl Pts',(-36.4290706579489,-3.00233488224952,
135.780103240898));
#215474=CARTESIAN_POINT('Ctrl Pts',(-36.7075182817618,2.56339784940132,
136.019820411726));
#215475=CARTESIAN_POINT('Ctrl Pts',(-36.9859659055747,5.77349318639923,
131.466784821096));
#215476=CARTESIAN_POINT('Ctrl Pts',(-37.2644135293876,3.67803033591843,
126.305013748643));
#215477=CARTESIAN_POINT('Ctrl Pts',(-37.5428611532005,-1.79736271150026,
125.277922643415));
#215478=CARTESIAN_POINT('Ctrl Pts',(-37.8213087770133,-5.62106723310019,
129.329358054928));
#215479=CARTESIAN_POINT('Ctrl Pts',(-38.0997564008263,-4.27928557188161,
134.736248763623));
#215480=CARTESIAN_POINT('Ctrl Pts',(-38.3782040246392,0.994950475174061,
136.529926349506));
#215481=CARTESIAN_POINT('Ctrl Pts',(-38.656651648452,5.35487564157755,133.062088737171));
#215482=CARTESIAN_POINT('Ctrl Pts',(-38.9350992722649,4.79393169358958,
127.51950927907));
#215483=CARTESIAN_POINT('Ctrl Pts',(-39.2135468960779,-0.172401284224016,
124.995547727136));
#215484=CARTESIAN_POINT('Ctrl Pts',(-39.4919945198907,-4.98030590410683,
127.809601445221));
#215485=CARTESIAN_POINT('Ctrl Pts',(-39.7704421437036,-5.21155269958477,
133.375692540572));
#215486=CARTESIAN_POINT('Ctrl Pts',(-40.0488897675166,-0.65363716264763,
136.578855215227));
#215487=CARTESIAN_POINT('Ctrl Pts',(-40.3273373913294,4.50493899481217,
134.475539454375));
#215488=CARTESIAN_POINT('Ctrl Pts',(-40.6057850151423,5.52369629454426,
128.998589689552));
#215489=CARTESIAN_POINT('Ctrl Pts',(-40.8842326389552,1.46644654715595,
125.181055190758));
#215490=CARTESIAN_POINT('Ctrl Pts',(-41.1626802627681,-3.93839593717207,
126.531063665459));
#215491=CARTESIAN_POINT('Ctrl Pts',(-41.441127886581,-5.72404495657686,
131.808023276983));
#215492=CARTESIAN_POINT('Ctrl Pts',(-41.7195755103939,-2.24957629602936,
136.162665936149));
#215493=CARTESIAN_POINT('Ctrl Pts',(-41.9980231342068,3.29214308265742,
135.593287775304));
#215494=CARTESIAN_POINT('Ctrl Pts',(-42.2764707580197,5.80854379851262,
130.623119508596));
#215495=CARTESIAN_POINT('Ctrl Pts',(-42.5549183818325,2.98717652667487,
125.81950296691));
#215496=CARTESIAN_POINT('Ctrl Pts',(-42.8333660056454,-2.57926004149102,
125.596727082342));
#215497=CARTESIAN_POINT('Ctrl Pts',(-43.1118136294584,-5.7754826353847,
130.159512009603));
#215498=CARTESIAN_POINT('Ctrl Pts',(-43.3902612532712,-3.66431883537201,
135.314881304976));
#215499=CARTESIAN_POINT('Ctrl Pts',(-43.6687088770841,1.81417496242045,
136.325302439805));
#215500=CARTESIAN_POINT('Ctrl Pts',(-43.947156500897,5.62553059712261,132.262247752997));
#215501=CARTESIAN_POINT('Ctrl Pts',(-44.2256041247099,4.26729843551711,
126.859466010475));
#215502=CARTESIAN_POINT('Ctrl Pts',(-44.5040517485228,-1.01237251921066,
125.081849693053));
#215503=CARTESIAN_POINT('Ctrl Pts',(-44.7824993723357,-5.3617225859308,
128.562941355057));
#215504=CARTESIAN_POINT('Ctrl Pts',(-45.0609469961486,-4.78391153089065,
134.103787819889));
#215505=CARTESIAN_POINT('Ctrl Pts',(-45.3393946199614,0.190080513966956,
136.612621871764));
#215506=CARTESIAN_POINT('Ctrl Pts',(-45.6178422437743,4.98939785243841,
133.783947580368));
#215507=CARTESIAN_POINT('Ctrl Pts',(-45.8962898675873,5.20370231015464,
128.217178431071));
#215508=CARTESIAN_POINT('Ctrl Pts',(-46.1747374914001,0.636058559829223,
125.027903320286));
#215509=CARTESIAN_POINT('Ctrl Pts',(-46.453185115213,-4.51609193379101,
127.146910270074));
#215510=CARTESIAN_POINT('Ctrl Pts',(-46.7316327390259,-5.51817456361365,
132.626935412823));
#215511=CARTESIAN_POINT('Ctrl Pts',(-47.0100803628388,-1.4493243472895,
136.43210335646));
#215512=CARTESIAN_POINT('Ctrl Pts',(-47.2885279866517,3.95138414076325,
135.06565065357));
#215513=CARTESIAN_POINT('Ctrl Pts',(-47.5669756104645,5.72096363930122,
129.783280583183));
#215514=CARTESIAN_POINT('Ctrl Pts',(-47.8454232342775,2.23325703793269,
125.439233181862));
#215515=CARTESIAN_POINT('Ctrl Pts',(-48.1238708580903,-3.30670368062431,
126.025475792906));
#215516=CARTESIAN_POINT('Ctrl Pts',(-48.4023184819033,-5.80796525814313,
131.00328009631));
#215517=CARTESIAN_POINT('Ctrl Pts',(-48.6807661057162,-2.97199049830493,
135.798287116504));
#215518=CARTESIAN_POINT('Ctrl Pts',(-48.9592137295291,2.59509833966803,
136.004119651047));
#215519=CARTESIAN_POINT('Ctrl Pts',(-49.2376613533419,5.77741858108801,
131.431627656171));
#215520=CARTESIAN_POINT('Ctrl Pts',(-49.5161089771548,3.65057338907646,
126.282707896514));
#215521=CARTESIAN_POINT('Ctrl Pts',(-49.7945566009678,-1.8309704070716,
125.288966092489));
#215522=CARTESIAN_POINT('Ctrl Pts',(-50.0730042247805,-5.62994184699806,
129.363602415007));
#215523=CARTESIAN_POINT('Ctrl Pts',(-50.3514518485936,-4.25527176748286,
134.762225140725));
#215524=CARTESIAN_POINT('Ctrl Pts',(-50.6298994724063,1.02978518476655,
136.52376372209));
#215525=CARTESIAN_POINT('Ctrl Pts',(-50.9083470962193,5.36851986001845,
133.029450258773));
#215526=CARTESIAN_POINT('Ctrl Pts',(-51.1867947200322,4.77384705068883,
127.490388116857));
#215527=CARTESIAN_POINT('Ctrl Pts',(-51.465242343845,-0.207757982829986,
124.996704806535));
#215528=CARTESIAN_POINT('Ctrl Pts',(-51.743689967658,-4.99844357966987,
127.839973466791));
#215529=CARTESIAN_POINT('Ctrl Pts',(-52.0221375914708,-5.19580371433717,
133.407369100245));
#215530=CARTESIAN_POINT('Ctrl Pts',(-52.3005852152837,-0.618474064651215,
136.58272710215));
#215531=CARTESIAN_POINT('Ctrl Pts',(-52.5790328390967,4.52720303631132,
134.448048593619));
#215532=CARTESIAN_POINT('Ctrl Pts',(-52.8574804629095,5.51260171306762,
128.964998839148));
#215533=CARTESIAN_POINT('Ctrl Pts',(-53.1359280867224,1.43218872108006,
125.172232701224));
#215534=CARTESIAN_POINT('Ctrl Pts',(-53.4143757105353,-3.96433573927151,
126.555116973674));
#215535=CARTESIAN_POINT('Ctrl Pts',(-53.6928233343482,-5.71782932379997,
131.842848567767));
#215536=CARTESIAN_POINT('Ctrl Pts',(-53.9712709581611,-2.21691709124776,
136.176260468582));
#215537=CARTESIAN_POINT('Ctrl Pts',(-54.249718581974,3.32123364574025,135.573158838211));
#215538=CARTESIAN_POINT('Ctrl Pts',(-54.5281662057869,5.80733291357678,
130.58776461181));
#215539=CARTESIAN_POINT('Ctrl Pts',(-54.8066138295998,2.95677693782102,
125.801411533396));
#215540=CARTESIAN_POINT('Ctrl Pts',(-55.0850614534126,-2.61091259720856,
125.612524255684));
#215541=CARTESIAN_POINT('Ctrl Pts',(-55.3635090772256,-5.77930100557468,
130.194680959234));
#215542=CARTESIAN_POINT('Ctrl Pts',(-55.6419567010384,-3.63679412436797,
135.337103484283));
#215543=CARTESIAN_POINT('Ctrl Pts',(-55.9204043248514,1.8477488898629,136.314156751619));
#215544=CARTESIAN_POINT('Ctrl Pts',(-56.1988519486642,5.63430094186134,
132.227976540264));
#215545=CARTESIAN_POINT('Ctrl Pts',(-56.4772995724772,4.24320567919224,
126.833562843453));
#215546=CARTESIAN_POINT('Ctrl Pts',(-56.7557471962901,-1.04718831053316,
125.088118316796));
#215547=CARTESIAN_POINT('Ctrl Pts',(-57.0341948201028,-5.3752674008715,
128.595621210585));
#215548=CARTESIAN_POINT('Ctrl Pts',(-57.3126424439159,-4.76373834622006,
134.13284771647));
#215549=CARTESIAN_POINT('Ctrl Pts',(-57.5910900677287,0.225433527051438,
136.611357184097));
#215550=CARTESIAN_POINT('Ctrl Pts',(-57.8695376915416,5.00744300200284,
133.753520494635));
#215551=CARTESIAN_POINT('Ctrl Pts',(-58.1479853153544,5.18785698530388,
128.185549952615));
#215552=CARTESIAN_POINT('Ctrl Pts',(-58.4264329391674,0.600883840013963,
125.024138475672));
#215553=CARTESIAN_POINT('Ctrl Pts',(-58.7048805629802,-4.53827219944114,
127.174468767579));
#215554=CARTESIAN_POINT('Ctrl Pts',(-58.9833281867932,-5.5069777945324,
132.660492339548));
#215555=CARTESIAN_POINT('Ctrl Pts',(-59.261775810606,-1.41503982726995,
136.440821536091));
#215556=CARTESIAN_POINT('Ctrl Pts',(-59.540223434419,3.97725061271504,135.041518504932));
#215557=CARTESIAN_POINT('Ctrl Pts',(-59.8186710582318,5.71464203910897,
129.748474371954));
#215558=CARTESIAN_POINT('Ctrl Pts',(-60.0971186820448,2.20055660734573,
125.425738115783));
#215559=CARTESIAN_POINT('Ctrl Pts',(-60.3755663058576,-3.3357328434014,
126.045693178431));
#215560=CARTESIAN_POINT('Ctrl Pts',(-60.6540139296705,-5.80664677067165,
131.038631143817));
#215561=CARTESIAN_POINT('Ctrl Pts',(-60.9324615534834,-2.94153598615947,
135.816285940328));
#215562=CARTESIAN_POINT('Ctrl Pts',(-61.2109091772963,2.62670266761142,
135.988226211385));
#215563=CARTESIAN_POINT('Ctrl Pts',(-61.4893568011092,5.78112989140647,
131.396447247635));
#215564=CARTESIAN_POINT('Ctrl Pts',(-61.767804424922,3.62298116889529,126.260569595891));
#215565=CARTESIAN_POINT('Ctrl Pts',(-62.046252048735,-1.86451025536104,
125.300213916535));
#215566=CARTESIAN_POINT('Ctrl Pts',(-62.3246996725479,-5.63860784133039,
129.39790016291));
#215567=CARTESIAN_POINT('Ctrl Pts',(-62.6031472963608,-4.23110028242386,
134.788054857702));
#215568=CARTESIAN_POINT('Ctrl Pts',(-62.8815949201736,1.0645817352901,136.517389160091));
#215569=CARTESIAN_POINT('Ctrl Pts',(-63.1600425439866,5.38196514598156,
132.99672932886));
#215570=CARTESIAN_POINT('Ctrl Pts',(-63.4384901677994,4.75358551113023,
127.461389755115));
#215571=CARTESIAN_POINT('Ctrl Pts',(-63.7169377916123,-0.243106982887504,
124.998077090756));
#215572=CARTESIAN_POINT('Ctrl Pts',(-63.9953854154252,-5.0163960360679,
127.870455334816));
#215573=CARTESIAN_POINT('Ctrl Pts',(-64.2738330392381,-5.17986219667218,
133.438949204482));
#215574=CARTESIAN_POINT('Ctrl Pts',(-64.552280663051,-0.583288048870894,
136.586384869579));
#215575=CARTESIAN_POINT('Ctrl Pts',(-64.8307282868638,4.54929932063727,
134.420422714664));
#215576=CARTESIAN_POINT('Ctrl Pts',(-65.1091759106768,5.50130286010717,
128.93147614697));
#215577=CARTESIAN_POINT('Ctrl Pts',(-65.3876235344896,1.39787782472419,
125.16361891226));
#215578=CARTESIAN_POINT('Ctrl Pts',(-65.6660711583025,-3.99012864145221,
126.579327739175));
#215579=CARTESIAN_POINT('Ctrl Pts',(-65.9445187821156,-5.71140181475477,
131.877635376998));
#215580=CARTESIAN_POINT('Ctrl Pts',(-66.2229664059283,-2.18417573778792,
136.189655943291));
#215581=CARTESIAN_POINT('Ctrl Pts',(-66.5014140297413,3.35020113928917,
135.552853191544));
#215582=CARTESIAN_POINT('Ctrl Pts',(-66.7798616535541,5.80590683578406,
130.552417741069));
#215583=CARTESIAN_POINT('Ctrl Pts',(-67.0583092773671,2.92626778451039,
125.783505486001));
#215584=CARTESIAN_POINT('Ctrl Pts',(-67.3367569011799,-2.64246840459962,
125.628513814431));
#215585=CARTESIAN_POINT('Ctrl Pts',(-67.6152045249929,-5.78290522164069,
130.229872500769));
#215586=CARTESIAN_POINT('Ctrl Pts',(-67.8936521488056,-3.60913465062,135.359157701137));
#215587=CARTESIAN_POINT('Ctrl Pts',(-68.1720997726187,1.88125434829088,
136.302806895912));
#215588=CARTESIAN_POINT('Ctrl Pts',(-68.4505473964314,5.64286250550667,
132.193652574919));
#215589=CARTESIAN_POINT('Ctrl Pts',(-68.7289950202444,4.21895568932047,
126.807806815805));
#215590=CARTESIAN_POINT('Ctrl Pts',(-69.0074426440573,-1.08196529790749,
125.094598758));
#215591=CARTESIAN_POINT('Ctrl Pts',(-69.2858902678701,-5.38861303330182,
128.628382911763));
#215592=CARTESIAN_POINT('Ctrl Pts',(-69.564337891683,-4.74338863947339,
134.161784274737));
#215593=CARTESIAN_POINT('Ctrl Pts',(-69.8427855154959,0.260778186613682,
136.609877316035));
#215594=CARTESIAN_POINT('Ctrl Pts',(-70.1212331393089,5.02530259892534,
133.722984126697));
#215595=CARTESIAN_POINT('Ctrl Pts',(-70.3996807631217,5.17181942250469,
128.154018515153));
#215596=CARTESIAN_POINT('Ctrl Pts',(-70.6781283869345,0.5656868542273,125.020587819316));
#215597=CARTESIAN_POINT('Ctrl Pts',(-70.9565760107477,-4.56028429774593,
127.202161772061));
#215598=CARTESIAN_POINT('Ctrl Pts',(-71.2350236345604,-5.49557696236377,
132.693980486629));
#215599=CARTESIAN_POINT('Ctrl Pts',(-71.5134712583732,-1.38070287242923,
136.449330854589));
#215600=CARTESIAN_POINT('Ctrl Pts',(-71.7919188821862,4.00296970618273,
135.017229346852));
#215601=CARTESIAN_POINT('Ctrl Pts',(-72.0703665059991,5.70810868075446,
129.71370728698));
#215602=CARTESIAN_POINT('Ctrl Pts',(-72.348814129812,2.16777463432419,125.412442356538));
#215603=CARTESIAN_POINT('Ctrl Pts',(-72.6272617536249,-3.36463839937136,
126.06608689813));
#215604=CARTESIAN_POINT('Ctrl Pts',(-72.9057093774378,-5.80511311576878,
131.073973510343));
#215605=CARTESIAN_POINT('Ctrl Pts',(-73.1841570012506,-2.91097247431594,
135.834099045416));
#215606=CARTESIAN_POINT('Ctrl Pts',(-73.4626046250635,2.65820966212185,
135.972140681676));
#215607=CARTESIAN_POINT('Ctrl Pts',(-73.7410522488765,5.78462697983096,
131.361244899111));
#215608=CARTESIAN_POINT('Ctrl Pts',(-74.0194998726893,3.59525469781404,
126.238599667113));
#215609=CARTESIAN_POINT('Ctrl Pts',(-74.2979474965022,-1.89798101353784,
125.31166569876));
#215610=CARTESIAN_POINT('Ctrl Pts',(-74.5763951203151,-5.64706489497548,
129.432250027724));
#215611=CARTESIAN_POINT('Ctrl Pts',(-74.854842744128,-4.20677201238788,
134.813736957424));
#215612=CARTESIAN_POINT('Ctrl Pts',(-75.1332903679409,1.09933883734644,
136.510802899716));
#215613=CARTESIAN_POINT('Ctrl Pts',(-75.4117379917539,5.39521100124704,
132.963927159917));
#215614=CARTESIAN_POINT('Ctrl Pts',(-75.6901856155667,4.73314782571214,
127.432515268386));
#215615=CARTESIAN_POINT('Ctrl Pts',(-75.9686332393795,-0.278446974526432,
124.99966452895));
#215616=CARTESIAN_POINT('Ctrl Pts',(-76.2470808631926,-5.03416260806588,
127.901045919781));
#215617=CARTESIAN_POINT('Ctrl Pts',(-76.5255284870053,-5.16372873730878,
133.470431683069));
#215618=CARTESIAN_POINT('Ctrl Pts',(-76.8039761108183,-0.548080419137594,
136.589828381972));
#215619=CARTESIAN_POINT('Ctrl Pts',(-77.0824237346311,4.57122702900371,
134.392662841198));
#215620=CARTESIAN_POINT('Ctrl Pts',(-77.360871358444,5.48980015434633,128.898022855216));
#215621=CARTESIAN_POINT('Ctrl Pts',(-77.639318982257,1.36351512949127,125.155214143056));
#215622=CARTESIAN_POINT('Ctrl Pts',(-77.9177666060698,-4.0157736879487,
126.603695064822));
#215623=CARTESIAN_POINT('Ctrl Pts',(-78.1962142298826,-5.70476266761487,
131.91238241564));
#215624=CARTESIAN_POINT('Ctrl Pts',(-78.4746618536957,-2.15135344889296,
136.202851863901));
#215625=CARTESIAN_POINT('Ctrl Pts',(-78.7531094775085,3.37904448990285,
135.532371587738));
#215626=CARTESIAN_POINT('Ctrl Pts',(-79.0315571013213,5.8042656179783,130.517080206165));
#215627=CARTESIAN_POINT('Ctrl Pts',(-79.3100047251342,2.8956501972711,125.765785488239));
#215628=CARTESIAN_POINT('Ctrl Pts',(-79.5884523489472,-2.67392629435197,
125.644695166086));
#215629=CARTESIAN_POINT('Ctrl Pts',(-79.8668999727601,-5.78629515002701,
130.265085330171));
#215630=CARTESIAN_POINT('Ctrl Pts',(-80.1453475965729,-3.58134143906054,
135.38104313831));
#215631=CARTESIAN_POINT('Ctrl Pts',(-80.4237952203859,1.91469009614739,
136.291253293255));
#215632=CARTESIAN_POINT('Ctrl Pts',(-80.7022428441988,5.65121497080658,
132.15927712885));
#215633=CARTESIAN_POINT('Ctrl Pts',(-80.9806904680116,4.19454936449412,
126.782198881926));
#215634=CARTESIAN_POINT('Ctrl Pts',(-81.2591380918246,-1.11670219266007,
125.10129077653));
#215635=CARTESIAN_POINT('Ctrl Pts',(-81.5375857156372,-5.40175898869456,
128.661225244595));
#215636=CARTESIAN_POINT('Ctrl Pts',(-81.8160333394505,-4.72286316471603,
134.190596422436));
#215637=CARTESIAN_POINT('Ctrl Pts',(-82.0944809632629,0.296113182944105,
136.608182322418));
#215638=CARTESIAN_POINT('Ctrl Pts',(-82.3729285870762,5.04297598141181,
133.692339608092));
#215639=CARTESIAN_POINT('Ctrl Pts',(-82.6513762108889,5.15559021603496,
128.122585287091));
#215640=CARTESIAN_POINT('Ctrl Pts',(-82.9298238347018,0.530468906706182,
125.017251482786));
#215641=CARTESIAN_POINT('Ctrl Pts',(-83.2082714585147,-4.58212741303929,
127.229988257347));
#215642=CARTESIAN_POINT('Ctrl Pts',(-83.4867190823277,-5.48397248956967,
132.72739861315));
#215643=CARTESIAN_POINT('Ctrl Pts',(-83.7651667061405,-1.34631475513585,
136.45763099664));
#215644=CARTESIAN_POINT('Ctrl Pts',(-84.0436143299535,4.02854046813582,
134.992784079373));
#215645=CARTESIAN_POINT('Ctrl Pts',(-84.3220619537663,5.70136380633342,
129.678980616565));
#215646=CARTESIAN_POINT('Ctrl Pts',(-84.6005095775792,2.13491233361711,
125.399346396808));
#215647=CARTESIAN_POINT('Ctrl Pts',(-84.8789572013921,-3.39341927742779,
126.086656196302));
#215648=CARTESIAN_POINT('Ctrl Pts',(-85.1574048252049,-5.80336435026449,
131.109305886265));
#215649=CARTESIAN_POINT('Ctrl Pts',(-85.4358524490179,-2.88030109531746,
135.851725771696));
#215650=CARTESIAN_POINT('Ctrl Pts',(-85.7143000728307,2.68961815569484,
135.955863657977));
#215651=CARTESIAN_POINT('Ctrl Pts',(-85.9927476966438,5.78790971677558,
131.326021915035));
#215652=CARTESIAN_POINT('Ctrl Pts',(-86.2711953204564,3.56739500324825,
126.216798924288));
#215653=CARTESIAN_POINT('Ctrl Pts',(-86.5496429442695,-1.93138144132926,
125.323321014816));
#215654=CARTESIAN_POINT('Ctrl Pts',(-86.8280905680822,-5.65531269455438,
129.466650736599));
#215655=CARTESIAN_POINT('Ctrl Pts',(-87.1065381918953,-4.18228785886808,
134.83927048823));
#215656=CARTESIAN_POINT('Ctrl Pts',(-87.3849858157081,1.13405520299706,
136.504005185026));
#215657=CARTESIAN_POINT('Ctrl Pts',(-87.663433439521,5.40825693498488,132.931044967442));
#215658=CARTESIAN_POINT('Ctrl Pts',(-87.9418810633338,4.71253475176078,
127.403765726628));
#215659=CARTESIAN_POINT('Ctrl Pts',(-88.2203286871468,-0.313776648210234,
125.00146706229));
#215660=CARTESIAN_POINT('Ctrl Pts',(-88.4987763109598,-5.05174263731727,
127.931744088139));
#215661=CARTESIAN_POINT('Ctrl Pts',(-88.7772239347726,-5.14740393407785,
133.501815369412));
#215662=CARTESIAN_POINT('Ctrl Pts',(-89.0556715585855,-0.512852480082647,
136.593057511728));
#215663=CARTESIAN_POINT('Ctrl Pts',(-89.3341191823985,4.59298534887173,
134.364770001874));
#215664=CARTESIAN_POINT('Ctrl Pts',(-89.6125668062112,5.47809402202166,
128.864640203508));
#215665=CARTESIAN_POINT('Ctrl Pts',(-89.8910144300243,1.32910190870433,
125.147018705051));
#215666=CARTESIAN_POINT('Ctrl Pts',(-90.169462053837,-4.04126992847403,
126.628218047677));
#215667=CARTESIAN_POINT('Ctrl Pts',(-90.44790967765,-5.69791212839678,131.947088396125));
#215668=CARTESIAN_POINT('Ctrl Pts',(-90.7263573014627,-2.1184514408047,
136.215847741432));
#215669=CARTESIAN_POINT('Ctrl Pts',(-91.0048049252757,3.40776262878029,
135.511714785749));
#215670=CARTESIAN_POINT('Ctrl Pts',(-91.2832525490887,5.80240932097568,
130.48175331654));
#215671=CARTESIAN_POINT('Ctrl Pts',(-91.5617001729014,2.86492531064864,
125.748252196732));
#215672=CARTESIAN_POINT('Ctrl Pts',(-91.8401477967144,-2.70528510078237,
125.661067711041));
#215673=CARTESIAN_POINT('Ctrl Pts',(-92.1185954205271,-5.78947066511866,
130.30031814262));
#215674=CARTESIAN_POINT('Ctrl Pts',(-92.3970430443404,-3.55341551957677,
135.402758984829));
#215675=CARTESIAN_POINT('Ctrl Pts',(-92.6754906681528,1.94805489445803,
136.279496371773));
#215676=CARTESIAN_POINT('Ctrl Pts',(-92.9539382919661,5.6593580282576,132.124851475851));
#215677=CARTESIAN_POINT('Ctrl Pts',(-93.2323859157787,4.16998760909852,
126.75673999073));
#215678=CARTESIAN_POINT('Ctrl Pts',(-93.5108335395918,-1.15139770760221,
125.10819412441));
#215679=CARTESIAN_POINT('Ctrl Pts',(-93.7892811634045,-5.41470477992152,
128.694146992097));
#215680=CARTESIAN_POINT('Ctrl Pts',(-94.0677287872175,-4.70216268252734,
134.219283091922));
#215681=CARTESIAN_POINT('Ctrl Pts',(-94.3461764110305,0.331437206691851,
136.606272266052));
#215682=CARTESIAN_POINT('Ctrl Pts',(-94.6246240348431,5.0604624945689,133.661588074364));
#215683=CARTESIAN_POINT('Ctrl Pts',(-94.9030716586564,5.13916996727372,
128.0912514332));
#215684=CARTESIAN_POINT('Ctrl Pts',(-95.1815192824688,0.495231302464415,
125.014129589715));
#215685=CARTESIAN_POINT('Ctrl Pts',(-95.459966906282,-4.60380073591605,
127.257947192314));
#215686=CARTESIAN_POINT('Ctrl Pts',(-95.7384145300948,-5.47216480615837,
132.760745480792));
#215687=CARTESIAN_POINT('Ctrl Pts',(-96.0168621539077,-1.31187674965409,
136.465721654678));
#215688=CARTESIAN_POINT('Ctrl Pts',(-96.2953097777207,4.05396195104042,
134.96818360832));
#215689=CARTESIAN_POINT('Ctrl Pts',(-96.5737574015334,5.69440766577999,
129.64429564752));
#215690=CARTESIAN_POINT('Ctrl Pts',(-96.8522050253465,2.10197092294792,
125.386450721867));
#215691=CARTESIAN_POINT('Ctrl Pts',(-97.1306526491593,-3.42207441108517,
126.107400310748));
#215692=CARTESIAN_POINT('Ctrl Pts',(-97.4091002729722,-5.80140053895979,
131.144626962327));
#215693=CARTESIAN_POINT('Ctrl Pts',(-97.6875478967851,-2.8495229857029,
135.869165466005));
#215694=CARTESIAN_POINT('Ctrl Pts',(-97.965995520598,2.72092698447821,135.93939574344));
#215695=CARTESIAN_POINT('Ctrl Pts',(-98.2444431444108,5.79097798059694,
131.290779600608));
#215696=CARTESIAN_POINT('Ctrl Pts',(-98.5228907682237,3.53940311754856,
126.195168175249));
#215697=CARTESIAN_POINT('Ctrl Pts',(-98.8013383920368,-1.96471030107164,
125.33517943281));
#215698=CARTESIAN_POINT('Ctrl Pts',(-99.0797860158496,-5.6633509344415,
129.501101014807));
#215699=CARTESIAN_POINT('Ctrl Pts',(-99.3582336396624,-4.15764872913354,
134.864654503967));
#215700=CARTESIAN_POINT('Ctrl Pts',(-99.6366812634755,1.16872954581563,
136.496996267908));
#215701=CARTESIAN_POINT('Ctrl Pts',(-99.9151288872883,5.42110246377302,
132.898083969897));
#215702=CARTESIAN_POINT('Ctrl Pts',(-100.193576511101,4.69174705310118,
127.375142195163));
#215703=CARTESIAN_POINT('Ctrl Pts',(-100.472024134914,-0.34909469478497,
125.003484623986));
#215704=CARTESIAN_POINT('Ctrl Pts',(-100.750471758727,-5.06913547238742,
127.96254870236));
#215705=CARTESIAN_POINT('Ctrl Pts',(-101.02891938254,-5.13088839190121,
133.533099100579));
#215706=CARTESIAN_POINT('Ctrl Pts',(-101.307367006353,-0.47760553709043,
136.596072139193));
#215707=CARTESIAN_POINT('Ctrl Pts',(-101.585814630166,4.61457347397855,
134.33674523027));
#215708=CARTESIAN_POINT('Ctrl Pts',(-101.864262253979,5.46618489690847,
128.831329428852));
#215709=CARTESIAN_POINT('Ctrl Pts',(-102.142709877791,1.29463943755703,
125.139032901931));
#215710=CARTESIAN_POINT('Ctrl Pts',(-102.421157501604,-4.06661641825637,
126.652895779031));
#215711=CARTESIAN_POINT('Ctrl Pts',(-102.699605125417,-5.69085045094906,
131.981752032413));
#215712=CARTESIAN_POINT('Ctrl Pts',(-102.97805274923,-2.08547093271925,
136.228643094318));
#215713=CARTESIAN_POINT('Ctrl Pts',(-103.256500373043,3.43635449176034,
135.490883551018));
#215714=CARTESIAN_POINT('Ctrl Pts',(-103.534947996856,5.80033801356182,
130.446438381249));
#215715=CARTESIAN_POINT('Ctrl Pts',(-103.813395620669,2.83409426316523,
125.730906261181));
#215716=CARTESIAN_POINT('Ctrl Pts',(-104.091843244482,-2.73654366187847,
125.677630842606));
#215717=CARTESIAN_POINT('Ctrl Pts',(-104.370290868295,-5.79243164924577,
130.335569632546));
#215718=CARTESIAN_POINT('Ctrl Pts',(-104.648738492108,-3.52535792697413,
135.424304436005));
#215719=CARTESIAN_POINT('Ctrl Pts',(-104.92718611592,1.98134750687769,136.267536567122));
#215720=CARTESIAN_POINT('Ctrl Pts',(-105.205633739733,5.66729137611554,
132.090376891579));
#215721=CARTESIAN_POINT('Ctrl Pts',(-105.484081363546,4.14527133327901,
126.731431085605));
#215722=CARTESIAN_POINT('Ctrl Pts',(-105.762528987359,-1.18605055707886,
125.115308545834));
#215723=CARTESIAN_POINT('Ctrl Pts',(-106.040976611172,-5.42744992727162,
128.72714693434));
#215724=CARTESIAN_POINT('Ctrl Pts',(-106.319424234985,-4.68128795997122,
134.247843220201));
#215725=CARTESIAN_POINT('Ctrl Pts',(-106.597871858798,0.366748948912009,
136.604147217717));
#215726=CARTESIAN_POINT('Ctrl Pts',(-106.876319482611,5.07776149042729,
133.630730665021));
#215727=CARTESIAN_POINT('Ctrl Pts',(-107.154767106424,5.12255928467941,
128.060018114567));
#215728=CARTESIAN_POINT('Ctrl Pts',(-107.433214730236,0.45997534724462,
125.011222255784));
#215729=CARTESIAN_POINT('Ctrl Pts',(-107.711662354049,-4.62530346326349,
127.286037540936));
#215730=CARTESIAN_POINT('Ctrl Pts',(-107.990109977862,-5.46015434966779,
132.794019853873));
#215731=CARTESIAN_POINT('Ctrl Pts',(-108.268557601675,-1.2773901320969,
136.473602528901));
#215732=CARTESIAN_POINT('Ctrl Pts',(-108.547005225488,4.07923321289408,
134.943428845277));
#215733=CARTESIAN_POINT('Ctrl Pts',(-108.825452849301,5.6872405168564,129.609653665109));
#215734=CARTESIAN_POINT('Ctrl Pts',(-109.103900473114,2.06895162297316,
125.373755809571));
#215735=CARTESIAN_POINT('Ctrl Pts',(-109.382348096927,-3.45060273851677,
126.128318472786));
#215736=CARTESIAN_POINT('Ctrl Pts',(-109.66079572074,-5.79922175462486,
131.179935429694));
#215737=CARTESIAN_POINT('Ctrl Pts',(-109.939243344552,-2.81863928596571,
135.886417482107));
#215738=CARTESIAN_POINT('Ctrl Pts',(-110.217690968365,2.7521349883118,135.922737548286));
#215739=CARTESIAN_POINT('Ctrl Pts',(-110.496138592178,5.79383165759959,
131.255519261747));
#215740=CARTESIAN_POINT('Ctrl Pts',(-110.774586215991,3.51128007796473,
126.17370822153));
#215741=CARTESIAN_POINT('Ctrl Pts',(-111.053033839804,-1.99796635775128,
125.347240513325));
#215742=CARTESIAN_POINT('Ctrl Pts',(-111.331481463617,-5.67117931677705,
129.535599585778));
#215743=CARTESIAN_POINT('Ctrl Pts',(-111.60992908743,-4.13285553619637,
134.889888064022));
#215744=CARTESIAN_POINT('Ctrl Pts',(-111.888376711243,1.20336058093108,
136.489776408084));
#215745=CARTESIAN_POINT('Ctrl Pts',(-112.166824335056,5.43374711161577,
132.865045388662));
#215746=CARTESIAN_POINT('Ctrl Pts',(-112.445271958868,4.67078550002918,
127.34664573465));
#215747=CARTESIAN_POINT('Ctrl Pts',(-112.723719582681,-0.384399805526852,
125.005717139274));
#215748=CARTESIAN_POINT('Ctrl Pts',(-113.002167206494,-5.08634046877848,
127.993458620965));
#215749=CARTESIAN_POINT('Ctrl Pts',(-113.280614830307,-5.11418272276831,
133.564281717336));
#215750=CARTESIAN_POINT('Ctrl Pts',(-113.55906245412,-0.442340896249408,
136.598872152659));
#215751=CARTESIAN_POINT('Ctrl Pts',(-113.837510077933,4.63599060436829,
134.308589564856));
#215752=CARTESIAN_POINT('Ctrl Pts',(-114.115957701746,5.45407322030374,
128.798091765594));
#215753=CARTESIAN_POINT('Ctrl Pts',(-114.394405325558,1.26012899306928,
125.131257029612));
#215754=CARTESIAN_POINT('Ctrl Pts',(-114.672852949372,-4.09181221807183,
126.677727344441));
#215755=CARTESIAN_POINT('Ctrl Pts',(-114.951300573184,-5.68357789694507,
132.016372040028));
#215756=CARTESIAN_POINT('Ctrl Pts',(-115.229748196997,-2.05241314674147,
136.241237448422));
#215757=CARTESIAN_POINT('Ctrl Pts',(-115.50819582081,3.46481901936097,135.469878655457));
#215758=CARTESIAN_POINT('Ctrl Pts',(-115.786643444623,5.79805177248978,
130.411136708898));
#215759=CARTESIAN_POINT('Ctrl Pts',(-116.065091068436,2.80315819727665,
125.713748324348));
#215760=CARTESIAN_POINT('Ctrl Pts',(-116.343538692249,-2.76770081934284,
125.694383947029));
#215761=CARTESIAN_POINT('Ctrl Pts',(-116.621986316062,-5.79517799268792,
130.370838493694));
#215762=CARTESIAN_POINT('Ctrl Pts',(-116.900433939875,-3.49716970093708,
135.445678693465));
#215763=CARTESIAN_POINT('Ctrl Pts',(-117.178881563688,2.0145666997373,136.255374322477));
#215764=CARTESIAN_POINT('Ctrl Pts',(-117.4573291875,5.67501472040751,132.055854653499));
#215765=CARTESIAN_POINT('Ctrl Pts',(-117.735776811314,4.12040145290537,
126.706273104381));
#215766=CARTESIAN_POINT('Ctrl Pts',(-118.014224435126,-1.22065945701595,
125.122633777175));
#215767=CARTESIAN_POINT('Ctrl Pts',(-118.29267205894,-5.43999395846872,
128.760223848501));
#215768=CARTESIAN_POINT('Ctrl Pts',(-118.571119682752,-4.6602397705682,
134.276275748964));
#215769=CARTESIAN_POINT('Ctrl Pts',(-118.849567306565,0.402047101114997,
136.601807256156));
#215770=CARTESIAN_POINT('Ctrl Pts',(-119.128014930377,5.09487232796628,
133.599768523497));
#215771=CARTESIAN_POINT('Ctrl Pts',(-119.406462554191,5.10575878376697,
128.028886488555));
#215772=CARTESIAN_POINT('Ctrl Pts',(-119.684910178003,0.424702347469154,
125.008529588725));
#215773=CARTESIAN_POINT('Ctrl Pts',(-119.963357801817,-4.64663479828973,
127.314258262312));
#215774=CARTESIAN_POINT('Ctrl Pts',(-120.241805425629,-5.44794156515001,
132.827220499399));
#215775=CARTESIAN_POINT('Ctrl Pts',(-120.520253049442,-1.24285618037906,
136.48127332728));
#215776=CARTESIAN_POINT('Ctrl Pts',(-120.798700673255,4.10435331726091,
134.918520707537));
#215777=CARTESIAN_POINT('Ctrl Pts',(-121.077148297068,5.67986262514396,
129.575055953004));
#215778=CARTESIAN_POINT('Ctrl Pts',(-121.355595920881,2.03585565723516,
125.361262130332));
#215779=CARTESIAN_POINT('Ctrl Pts',(-121.634043544694,-3.47900320259493,
126.149409907283));
#215780=CARTESIAN_POINT('Ctrl Pts',(-121.912491168507,-5.79682807799514,
131.215229979999));
#215781=CARTESIAN_POINT('Ctrl Pts',(-122.19093879232,-2.78765114051323,
135.903481180724));
#215782=CARTESIAN_POINT('Ctrl Pts',(-122.469386416133,2.78324101077128,
135.905889689793));
#215783=CARTESIAN_POINT('Ctrl Pts',(-122.747834039945,5.79647064203949,
131.220242205036));
#215784=CARTESIAN_POINT('Ctrl Pts',(-123.026281663758,3.48302692660634,
126.152419858339));
#215785=CARTESIAN_POINT('Ctrl Pts',(-123.304729287571,-2.03114837905279,
125.359503809431));
#215786=CARTESIAN_POINT('Ctrl Pts',(-123.583176911384,-5.67879755147744,
129.570145171156));
#215787=CARTESIAN_POINT('Ctrl Pts',(-123.861624535197,-4.10790919877744,
134.914970233354));
#215788=CARTESIAN_POINT('Ctrl Pts',(-124.14007215901,1.23794702507767,136.482345873087));
#215789=CARTESIAN_POINT('Ctrl Pts',(-124.418519782823,5.44619040996103,
132.831930447996));
#215790=CARTESIAN_POINT('Ctrl Pts',(-124.696967406636,4.64965086928273,
127.318277401031));
#215791=CARTESIAN_POINT('Ctrl Pts',(-124.975415030448,-0.419690672193134,
125.00816452543));
#215792=CARTESIAN_POINT('Ctrl Pts',(-125.253862654262,-5.10335698895296,
128.024472698579));
#215793=CARTESIAN_POINT('Ctrl Pts',(-125.532310278074,-5.09728754571388,
133.595362064203));
#215794=CARTESIAN_POINT('Ctrl Pts',(-125.810757901887,-0.407059864303788,
136.601457448367));
#215795=CARTESIAN_POINT('Ctrl Pts',(-126.0892055257,4.65723594642128,134.280304048949));
#215796=CARTESIAN_POINT('Ctrl Pts',(-126.367653149513,5.44175944101008,
128.764928445366));
#215797=CARTESIAN_POINT('Ctrl Pts',(-126.646100773326,1.22557185403828,
125.123691376234));
#215798=CARTESIAN_POINT('Ctrl Pts',(-126.924548397139,-4.11685639428078,
126.702711823764));
#215799=CARTESIAN_POINT('Ctrl Pts',(-127.202996020952,-5.67609473587197,
132.050947136115));
#215800=CARTESIAN_POINT('Ctrl Pts',(-127.481443644765,-2.01927930784003,
136.253630337055));
#215801=CARTESIAN_POINT('Ctrl Pts',(-127.759891268577,3.4931551568182,135.44870087741));
#215802=CARTESIAN_POINT('Ctrl Pts',(-128.038338892391,5.79555068247735,
130.375849607603));
#215803=CARTESIAN_POINT('Ctrl Pts',(-128.316786516203,2.77211825933019,
125.696779022025));
#215804=CARTESIAN_POINT('Ctrl Pts',(-128.595234140016,-2.7987554186355,
125.711326403516));
#215805=CARTESIAN_POINT('Ctrl Pts',(-128.873681763829,-5.79770959367839,
130.406123419165));
#215806=CARTESIAN_POINT('Ctrl Pts',(-129.152129387642,-3.46885188599067,
135.466880965177));
#215807=CARTESIAN_POINT('Ctrl Pts',(-129.430577011455,2.04771124208698,
136.243010088514));
#215808=CARTESIAN_POINT('Ctrl Pts',(-129.709024635268,5.68252777494204,
132.021286040849));
#215809=CARTESIAN_POINT('Ctrl Pts',(-129.98747225908,4.09537888954061,126.681266979298));
#215810=CARTESIAN_POINT('Ctrl Pts',(-130.265919882893,-1.25522312496795,
125.130169546993));
#215811=CARTESIAN_POINT('Ctrl Pts',(-130.544367506706,-5.45233640868912,
128.793376508901));
#215812=CARTESIAN_POINT('Ctrl Pts',(-130.822815130519,-4.63901889426667,
134.304579624636));
#215813=CARTESIAN_POINT('Ctrl Pts',(-131.101262754332,0.437330355314798,
136.599252468079));
#215814=CARTESIAN_POINT('Ctrl Pts',(-131.379710378145,5.11179437313754,
133.568702797104));
#215815=CARTESIAN_POINT('Ctrl Pts',(-131.658158001958,5.08876908708517,
127.997857708758));
#215816=CARTESIAN_POINT('Ctrl Pts',(-131.936605625771,0.389413610192037,
125.006051688315));
#215817=CARTESIAN_POINT('Ctrl Pts',(-132.215053249584,-4.66779395055513,
127.342608310716));
#215818=CARTESIAN_POINT('Ctrl Pts',(-132.493500873397,-5.43552690515385,
132.860346187109));
#215819=CARTESIAN_POINT('Ctrl Pts',(-132.77194849721,-1.20827617416795,
136.488733765571));
#215820=CARTESIAN_POINT('Ctrl Pts',(-133.050396121022,4.12932133330617,
134.893460118082));
#215821=CARTESIAN_POINT('Ctrl Pts',(-133.328843744835,5.67227426403318,
129.540503793235));
#215822=CARTESIAN_POINT('Ctrl Pts',(-133.607291368648,2.00268425211708,
125.348970147109));
#215823=CARTESIAN_POINT('Ctrl Pts',(-133.885738992461,-3.50727475093002,
126.170673832692));
#215824=CARTESIAN_POINT('Ctrl Pts',(-134.164186616274,-5.79421959776922,
131.25050930539));
#215825=CARTESIAN_POINT('Ctrl Pts',(-134.442634240087,-2.75655969762259,
135.920355929551));
#215826=CARTESIAN_POINT('Ctrl Pts',(-134.7210818639,2.81424389921159,135.888852792264));
#215827=CARTESIAN_POINT('Ctrl Pts',(-134.999529487713,5.79889483612785,
131.18494973768));
#215828=CARTESIAN_POINT('Ctrl Pts',(-135.277977111526,3.45464471040472,
126.131303874523));
#215829=CARTESIAN_POINT('Ctrl Pts',(-135.556424735338,-2.06425513540386,
125.371968866708));
#215830=CARTESIAN_POINT('Ctrl Pts',(-135.834872359151,-5.68620535624619,
129.604736490841));
#215831=CARTESIAN_POINT('Ctrl Pts',(-136.113319982964,-4.08281064127246,
134.939900082537));
#215832=CARTESIAN_POINT('Ctrl Pts',(-136.391767606777,1.27248759664198,
136.474704938258));
#215833=CARTESIAN_POINT('Ctrl Pts',(-136.67021523059,5.45843189771781,132.798740374984));
#215834=CARTESIAN_POINT('Ctrl Pts',(-136.948662854403,4.62834394401342,
127.290038245509));
#215835=CARTESIAN_POINT('Ctrl Pts',(-137.227110478216,-0.454965987067202,
125.010826691762));
#215836=CARTESIAN_POINT('Ctrl Pts',(-137.505558102029,-5.12018440235748,
128.055589785961));
#215837=CARTESIAN_POINT('Ctrl Pts',(-137.784005725841,-5.0802034867949,
133.626338989485));
#215838=CARTESIAN_POINT('Ctrl Pts',(-138.062453349655,-0.371763748605222,
136.603827930521));
#215839=CARTESIAN_POINT('Ctrl Pts',(-138.340900973467,4.67830871288359,
134.251889730681));
#215840=CARTESIAN_POINT('Ctrl Pts',(-138.61934859728,5.42924401531914,128.731840697047));
#215841=CARTESIAN_POINT('Ctrl Pts',(-138.897796221093,1.19096930099152,
125.116336222143));
#215842=CARTESIAN_POINT('Ctrl Pts',(-139.176243844906,-4.14174801886209,
126.727848291193));
#215843=CARTESIAN_POINT('Ctrl Pts',(-139.454691468719,-5.66840124502105,
132.085476039479));
#215844=CARTESIAN_POINT('Ctrl Pts',(-139.733139092532,-1.98607064380098,
136.265821300996));
#215845=CARTESIAN_POINT('Ctrl Pts',(-140.011586716345,3.52136185412693,
135.427351001626));
#215846=CARTESIAN_POINT('Ctrl Pts',(-140.290034340158,5.79283483620279,
130.340578384942));
#215847=CARTESIAN_POINT('Ctrl Pts',(-140.56848196397,2.7409755995222,125.679998983016));
#215848=CARTESIAN_POINT('Ctrl Pts',(-140.846929587784,-2.82970630901691,
125.72845758426));
#215849=CARTESIAN_POINT('Ctrl Pts',(-141.125377211596,-5.80002635840773,
130.441423101462));
#215850=CARTESIAN_POINT('Ctrl Pts',(-141.403824835409,-3.44040553146196,
135.487910465481));
#215851=CARTESIAN_POINT('Ctrl Pts',(-141.682272459222,2.08077990574355,
136.230444323395));
#215852=CARTESIAN_POINT('Ctrl Pts',(-141.960720083035,5.68983026132012,
131.986672334579));
#215853=CARTESIAN_POINT('Ctrl Pts',(-142.239167706848,4.07020457040501,
126.656413636965));
#215854=CARTESIAN_POINT('Ctrl Pts',(-142.517615330661,-1.289740280165,125.137915576048));
#215855=CARTESIAN_POINT('Ctrl Pts',(-142.796062954474,-5.46447682057862,
128.826603687055));
#215856=CARTESIAN_POINT('Ctrl Pts',(-143.074510578287,-4.61762611741445,
134.332753798405));
#215857=CARTESIAN_POINT('Ctrl Pts',(-143.352958202099,0.472597404077474,
136.596482948152));
#215858=CARTESIAN_POINT('Ctrl Pts',(-143.631405825913,5.12852699888841,
133.537534636997));
#215859=CARTESIAN_POINT('Ctrl Pts',(-143.909853449725,5.07159082419343,
127.966932924958));
#215860=CARTESIAN_POINT('Ctrl Pts',(-144.188301073538,0.354110443050382,
125.003788646376));
#215861=CARTESIAN_POINT('Ctrl Pts',(-144.466748697351,-4.6887801359991,
127.371086635623));
#215862=CARTESIAN_POINT('Ctrl Pts',(-144.745196321164,-5.4229108297093,
132.893395689516));
#215863=CARTESIAN_POINT('Ctrl Pts',(-145.023643944977,-1.17365139483885,
136.495983567324));
#215864=CARTESIAN_POINT('Ctrl Pts',(-145.30209156879,4.15413633583088,134.868248005541));
#215865=CARTESIAN_POINT('Ctrl Pts',(-145.580539192603,5.66447571471356,
129.505998466145));
#215866=CARTESIAN_POINT('Ctrl Pts',(-145.858986816416,1.96943863679757,
125.336880315387));
#215867=CARTESIAN_POINT('Ctrl Pts',(-146.137434440228,-3.53541633590941,
126.192109461069));
#215868=CARTESIAN_POINT('Ctrl Pts',(-146.415882064041,-5.79139641060527,
131.285772098575));
#215869=CARTESIAN_POINT('Ctrl Pts',(-146.694329687854,-2.72536610939861,
135.937041103293));
#215870=CARTESIAN_POINT('Ctrl Pts',(-146.972777311667,2.84514250480927,
135.871627487008));
#215871=CARTESIAN_POINT('Ctrl Pts',(-147.25122493548,5.80110415003576,131.149643167454));
#215872=CARTESIAN_POINT('Ctrl Pts',(-147.529672559293,3.42613448107249,
126.110361052543));
#215873=CARTESIAN_POINT('Ctrl Pts',(-147.808120183106,-2.09728540002206,
125.38463522326));
#215874=CARTESIAN_POINT('Ctrl Pts',(-148.086567806919,-5.69340245658434,
129.639372263039));
#215875=CARTESIAN_POINT('Ctrl Pts',(-148.365015430732,-4.05756079371773,
134.964676687782));
#215876=CARTESIAN_POINT('Ctrl Pts',(-148.643463054544,1.30698101571045,
136.466853886735));
#215877=CARTESIAN_POINT('Ctrl Pts',(-148.921910678358,5.47047112127328,
132.765476399497));
#215878=CARTESIAN_POINT('Ctrl Pts',(-149.20035830217,4.60686551375719,127.261929314495));
#215879=CARTESIAN_POINT('Ctrl Pts',(-149.478805925983,-0.49022444300932,
125.013703539625));
#215880=CARTESIAN_POINT('Ctrl Pts',(-149.757253549796,-5.13682208544599,
128.086808730058));
#215881=CARTESIAN_POINT('Ctrl Pts',(-150.035701173609,-5.06293117906749,
133.657211345319));
#215882=CARTESIAN_POINT('Ctrl Pts',(-150.314148797422,-0.336453857064764,
136.605983511281));
#215883=CARTESIAN_POINT('Ctrl Pts',(-150.592596421235,4.69920812289605,
134.223347662954));
#215884=CARTESIAN_POINT('Ctrl Pts',(-150.871044045047,5.41652740699458,
128.698829746717));
#215885=CARTESIAN_POINT('Ctrl Pts',(-151.14949166886,1.15632261613933,125.109191839888));
#215886=CARTESIAN_POINT('Ctrl Pts',(-151.427939292673,-4.1664861694474,
126.753135815284));
#215887=CARTESIAN_POINT('Ctrl Pts',(-151.706386916486,-5.66049770947745,
132.119957470642));
#215888=CARTESIAN_POINT('Ctrl Pts',(-151.984834540299,-1.95278838518384,
136.277809888502));
#215889=CARTESIAN_POINT('Ctrl Pts',(-152.263282164112,3.54943806607717,
135.405829819234));
#215890=CARTESIAN_POINT('Ctrl Pts',(-152.541729787925,5.78990433430307,
130.3053243479));
#215891=CARTESIAN_POINT('Ctrl Pts',(-152.820177411738,2.70973137185537,
125.663408829112));
#215892=CARTESIAN_POINT('Ctrl Pts',(-153.09862503555,-2.86055234359039,
125.745776854456));
#215893=CARTESIAN_POINT('Ctrl Pts',(-153.377072659364,-5.80212820102742,
130.476736232542));
#215894=CARTESIAN_POINT('Ctrl Pts',(-153.655520283176,-3.41183169144105,
135.508766415124));
#215895=CARTESIAN_POINT('Ctrl Pts',(-153.933967906989,2.1137714653355,136.21767749275));
#215896=CARTESIAN_POINT('Ctrl Pts',(-154.212415530802,5.69692190894542,
131.952014817313));
#215897=CARTESIAN_POINT('Ctrl Pts',(-154.490863154615,4.04487942834225,
126.631713998332));
#215898=CARTESIAN_POINT('Ctrl Pts',(-154.769310778428,-1.32420964356211,
125.145871577308));
#215899=CARTESIAN_POINT('Ctrl Pts',(-155.047758402241,-5.47641474427016,
128.859904151722));
#215900=CARTESIAN_POINT('Ctrl Pts',(-155.326206026054,-4.59606223272787,
134.360797226267));
#215901=CARTESIAN_POINT('Ctrl Pts',(-155.604653649866,0.507846940569522,
136.593498799002));
#215902=CARTESIAN_POINT('Ctrl Pts',(-155.88310127368,5.14506958518534,133.50626519812));
#215903=CARTESIAN_POINT('Ctrl Pts',(-156.161548897493,5.05422463163864,
127.936113283085));
#215904=CARTESIAN_POINT('Ctrl Pts',(-156.439996521305,0.318794154216047,
125.001740546765));
#215905=CARTESIAN_POINT('Ctrl Pts',(-156.718444145118,-4.70959257697085,
127.399692181761));
#215906=CARTESIAN_POINT('Ctrl Pts',(-156.996891768931,-5.41009380630968,
132.926367781962));
#215907=CARTESIAN_POINT('Ctrl Pts',(-157.275339392744,-1.1389831254257,
136.503022463895));
#215908=CARTESIAN_POINT('Ctrl Pts',(-157.553787016557,4.17879740530553,
134.84288530416));
#215909=CARTESIAN_POINT('Ctrl Pts',(-157.83223464037,5.65646726616335,129.471541250343));
#215910=CARTESIAN_POINT('Ctrl Pts',(-158.110682264183,1.93612004320555,
125.324993083158));
#215911=CARTESIAN_POINT('Ctrl Pts',(-158.389129887996,-3.56342691473634,
126.213715998108));
#215912=CARTESIAN_POINT('Ctrl Pts',(-158.667577511808,-5.78835862111754,
131.321017052882));
#215913=CARTESIAN_POINT('Ctrl Pts',(-158.946025135621,-2.69407153173119,
135.95353608367));
#215914=CARTESIAN_POINT('Ctrl Pts',(-159.224472759434,2.87593568260513,
135.854214412314));
#215915=CARTESIAN_POINT('Ctrl Pts',(-159.502920383247,5.80309850189603,
131.114323802656));
#215916=CARTESIAN_POINT('Ctrl Pts',(-159.78136800706,3.39749729506709,126.089592168444));
#215917=CARTESIAN_POINT('Ctrl Pts',(-160.059815630873,-2.13023794895846,
125.39750240973));
#215918=CARTESIAN_POINT('Ctrl Pts',(-160.338263254686,-5.70038858580074,
129.674051204309));
#215919=CARTESIAN_POINT('Ctrl Pts',(-160.616710878499,-4.03216059175559,
134.989299130986));
#215920=CARTESIAN_POINT('Ctrl Pts',(-160.895158502312,1.34142600411673,
136.458793009441));
#215921=CARTESIAN_POINT('Ctrl Pts',(-161.173606126125,5.48230763450959,
132.732139754142));
#215922=CARTESIAN_POINT('Ctrl Pts',(-161.452053749937,4.58521637440516,
127.233951649575));
#215923=CARTESIAN_POINT('Ctrl Pts',(-161.730501373751,-0.525464733504406,
125.016794962416));
#215924=CARTESIAN_POINT('Ctrl Pts',(-162.008948997563,-5.15326942170307,
128.118128374039));
#215925=CARTESIAN_POINT('Ctrl Pts',(-162.287396621376,-5.04547126256333,
133.687977987722));
#215926=CARTESIAN_POINT('Ctrl Pts',(-162.565844245189,-0.301131498102361,
136.607924110772));
#215927=CARTESIAN_POINT('Ctrl Pts',(-162.844291869002,4.71993340202341,
134.194678903404));
#215928=CARTESIAN_POINT('Ctrl Pts',(-163.122739492814,5.40361008725504,
128.665896817606));
#215929=CARTESIAN_POINT('Ctrl Pts',(-163.401187116628,1.12163308332736,
125.102258494207));
#215930=CARTESIAN_POINT('Ctrl Pts',(-163.67963474044,-4.19106992935549,
126.778573459));
#215931=CARTESIAN_POINT('Ctrl Pts',(-163.958082364253,-5.65238442210956,
132.154390151878));
#215932=CARTESIAN_POINT('Ctrl Pts',(-164.236529988066,-1.91943376527495,
136.289595655332));
#215933=CARTESIAN_POINT('Ctrl Pts',(-164.514977611879,3.57738275229458,
135.384138127707));
#215934=CARTESIAN_POINT('Ctrl Pts',(-164.793425235692,5.78675928536899,
130.270088802833));
#215935=CARTESIAN_POINT('Ctrl Pts',(-165.071872859505,2.67838673409632,
125.647009175068));
#215936=CARTESIAN_POINT('Ctrl Pts',(-165.350320483318,-2.89129237934434,
125.763283572333));
#215937=CARTESIAN_POINT('Ctrl Pts',(-165.628768107131,-5.80401504365309,
130.512061503863));
#215938=CARTESIAN_POINT('Ctrl Pts',(-165.907215730944,-3.38313142474212,
135.52944804128));
#215939=CARTESIAN_POINT('Ctrl Pts',(-166.185663354757,2.14668469834846,
136.204710069657));
#215940=CARTESIAN_POINT('Ctrl Pts',(-166.464110978569,5.70380245503433,
131.917314773299));
#215941=CARTESIAN_POINT('Ctrl Pts',(-166.742558602383,4.01940440178476,
126.607168978656));
#215942=CARTESIAN_POINT('Ctrl Pts',(-167.021006226195,-1.3586299378839,
125.15403725596));
#215943=CARTESIAN_POINT('Ctrl Pts',(-167.299453850008,-5.48814973739939,
128.893276668938));
#215944=CARTESIAN_POINT('Ctrl Pts',(-167.577901473821,-4.57432803926507,
134.388708869063));
#215945=CARTESIAN_POINT('Ctrl Pts',(-167.856349097634,0.543077658606429,
136.590300131209));
#215946=CARTESIAN_POINT('Ctrl Pts',(-168.134796721447,5.16142151903669,
133.474895639175));
#215947=CARTESIAN_POINT('Ctrl Pts',(-168.413244345259,5.03667115293141,
127.905399925171));
#215948=CARTESIAN_POINT('Ctrl Pts',(-168.691691969073,0.283466052347084,
124.999907465374));
#215949=CARTESIAN_POINT('Ctrl Pts',(-168.970139592885,-4.7302305022577,
127.42842388914));
#215950=CARTESIAN_POINT('Ctrl Pts',(-169.248587216698,-5.39707630989451,
132.959261242652));
#215951=CARTESIAN_POINT('Ctrl Pts',(-169.527034840511,-1.10427265057399,
136.509850194457));
#215952=CARTESIAN_POINT('Ctrl Pts',(-169.805482464324,4.20330362790601,
134.81737295376));
#215953=CARTESIAN_POINT('Ctrl Pts',(-170.083930088137,5.6482492151383,129.437133422652));
#215954=CARTESIAN_POINT('Ctrl Pts',(-170.36237771195,1.90272970597286,125.313308890908));
#215955=CARTESIAN_POINT('Ctrl Pts',(-170.640825335763,-3.59130544946847,
126.235492643171));
#215956=CARTESIAN_POINT('Ctrl Pts',(-170.919272959575,-5.78510634187241,
131.356242862295));
#215957=CARTESIAN_POINT('Ctrl Pts',(-171.197720583389,-2.66267712425244,
135.969840259458));
#215958=CARTESIAN_POINT('Ctrl Pts',(-171.476168207202,2.90662229154664,
135.836614213432));
#215959=CARTESIAN_POINT('Ctrl Pts',(-171.754615831014,5.80487781780722,
131.07899295206));
#215960=CARTESIAN_POINT('Ctrl Pts',(-172.033063454828,3.36873421355001,
126.068997991823));
#215961=CARTESIAN_POINT('Ctrl Pts',(-172.31151107864,-2.16311156114431,
125.410569949319));
#215962=CARTESIAN_POINT('Ctrl Pts',(-172.589958702453,-5.70716348502144,
129.70877202961));
#215963=CARTESIAN_POINT('Ctrl Pts',(-172.868406326266,-4.00661097660031,
135.013766499754));
#215964=CARTESIAN_POINT('Ctrl Pts',(-173.146853950079,1.3758212854888,136.450522605077));
#215965=CARTESIAN_POINT('Ctrl Pts',(-173.425301573892,5.49394099882038,
132.698731674224));
#215966=CARTESIAN_POINT('Ctrl Pts',(-173.703749197705,4.56339732817417,
127.206106287473));
#215967=CARTESIAN_POINT('Ctrl Pts',(-173.982196821517,-0.560685552710569,
125.02010084558));
#215968=CARTESIAN_POINT('Ctrl Pts',(-174.260644445331,-5.1695258016666,
128.149547557344));
#215969=CARTESIAN_POINT('Ctrl Pts',(-174.539092069143,-5.02782438426607,
133.718637776622));
#215970=CARTESIAN_POINT('Ctrl Pts',(-174.817539692956,-0.265797980601551,
136.609649657082));
#215971=CARTESIAN_POINT('Ctrl Pts',(-175.095987316769,4.74048378228282,
134.165884514362));
#215972=CARTESIAN_POINT('Ctrl Pts',(-175.374434940582,5.39049253475655,
128.633043130058));
#215973=CARTESIAN_POINT('Ctrl Pts',(-175.652882564395,1.08690198798901,
125.095536442018));
#215974=CARTESIAN_POINT('Ctrl Pts',(-175.931330188208,-4.21549838762608,
126.80416027974));
#215975=CARTESIAN_POINT('Ctrl Pts',(-176.209777812021,-5.64406168355824,
132.188772807274));
#215976=CARTESIAN_POINT('Ctrl Pts',(-176.488225435833,-1.886008020042,136.301178164761));
#215977=CARTESIAN_POINT('Ctrl Pts',(-176.766673059646,3.60519487727851,
135.362276730843));
#215978=CARTESIAN_POINT('Ctrl Pts',(-177.045120683459,5.78339980594152,
130.234873055403));
#215979=CARTESIAN_POINT('Ctrl Pts',(-177.323568307272,2.64694284773159,
125.630800628577));
#215980=CARTESIAN_POINT('Ctrl Pts',(-177.602015931085,-2.92192527719638,
125.780977089175));
#215981=CARTESIAN_POINT('Ctrl Pts',(-177.880463554898,-5.80568681636668,
130.547397606436));
#215982=CARTESIAN_POINT('Ctrl Pts',(-178.158911178711,-3.35430579486411,
135.549954577584));
#215983=CARTESIAN_POINT('Ctrl Pts',(-178.437358802524,2.17951838517049,
136.191542534628));
#215984=CARTESIAN_POINT('Ctrl Pts',(-178.715806426336,5.71047164462571,
131.88257348836));
#215985=CARTESIAN_POINT('Ctrl Pts',(-178.99425405015,3.99378043471903,126.582779487459));
#215986=CARTESIAN_POINT('Ctrl Pts',(-179.272701673962,-1.39299988767372,
125.162412309422));
#215987=CARTESIAN_POINT('Ctrl Pts',(-179.551149297775,-5.49968136512185,
128.926720002072));
#215988=CARTESIAN_POINT('Ctrl Pts',(-179.829596921588,-4.55242434239454,
134.416487692516));
#215989=CARTESIAN_POINT('Ctrl Pts',(-180.108044545401,0.578288252700551,
136.5868870633));
#215990=CARTESIAN_POINT('Ctrl Pts',(-180.386492169214,5.17758219451528,
133.443427122574));
#215991=CARTESIAN_POINT('Ctrl Pts',(-180.664939793027,5.01893103852278,
127.874793989312));
#215992=CARTESIAN_POINT('Ctrl Pts',(-180.94338741684,0.248127446539293,
124.998289470128));
#215993=CARTESIAN_POINT('Ctrl Pts',(-181.221835040653,-4.75069314711374,
127.457280693096));
#215994=CARTESIAN_POINT('Ctrl Pts',(-181.500282664465,-5.38385882283189,
132.992074852706));
#215995=CARTESIAN_POINT('Ctrl Pts',(-181.778730288279,-1.06952125649312,
136.516466506004));
#215996=CARTESIAN_POINT('Ctrl Pts',(-182.057177912091,4.22765409554481,
134.791711899713));
#215997=CARTESIAN_POINT('Ctrl Pts',(-182.335625535904,5.63982186616143,
129.402776258069));
#215998=CARTESIAN_POINT('Ctrl Pts',(-182.614073159717,1.86926886239121,
125.301828171599));
#215999=CARTESIAN_POINT('Ctrl Pts',(-182.89252078353,-3.61905090705647,
126.257438589318));
#216000=CARTESIAN_POINT('Ctrl Pts',(-183.170968407343,-5.78163969338434,
131.391448221508));
#216001=CARTESIAN_POINT('Ctrl Pts',(-183.449416031155,-2.63118405029363,
135.985953026497));
#216002=CARTESIAN_POINT('Ctrl Pts',(-183.727863654969,2.93720119453022,
135.818827542541));
#216003=CARTESIAN_POINT('Ctrl Pts',(-184.006311278781,5.80644203183612,
131.04365192486));
#216004=CARTESIAN_POINT('Ctrl Pts',(-184.284758902595,3.33984630234777,
126.048579285806));
#216005=CARTESIAN_POINT('Ctrl Pts',(-184.563206526407,-2.19590501843575,
125.423837357804));
#216006=CARTESIAN_POINT('Ctrl Pts',(-184.84165415022,-5.71372690320071,
129.743533452349));
#216007=CARTESIAN_POINT('Ctrl Pts',(-185.120101774033,-3.98091289500146,
135.03807788744));
#216008=CARTESIAN_POINT('Ctrl Pts',(-185.398549397846,1.41016558529749,
136.442042980103));
#216009=CARTESIAN_POINT('Ctrl Pts',(-185.676997021659,5.50537078312707,
132.665253397689));
#216010=CARTESIAN_POINT('Ctrl Pts',(-185.955444645472,4.54140918357699,
127.178394260007));
#216011=CARTESIAN_POINT('Ctrl Pts',(-186.233892269285,-0.595885595507362,
125.023621066618));
#216012=CARTESIAN_POINT('Ctrl Pts',(-186.512339893098,-5.18559062295048,
128.181065115723));
#216013=CARTESIAN_POINT('Ctrl Pts',(-186.79078751691,-5.00999119808726,
133.749189575911));
#216014=CARTESIAN_POINT('Ctrl Pts',(-187.069235140724,-0.230454613858838,
136.611160086272));
#216015=CARTESIAN_POINT('Ctrl Pts',(-187.347682764536,4.76085850217237,
134.136965562817));
#216016=CARTESIAN_POINT('Ctrl Pts',(-187.626130388349,5.37717523557474,
128.600269901479));
#216017=CARTESIAN_POINT('Ctrl Pts',(-187.904578012162,1.05213061709833,
125.089025932407));
#216018=CARTESIAN_POINT('Ctrl Pts',(-188.183025635975,-4.23977063905356,
126.829895329374));
#216019=CARTESIAN_POINT('Ctrl Pts',(-188.461473259788,-5.63552980222562,
132.223104162766));
#216020=CARTESIAN_POINT('Ctrl Pts',(-188.739920883601,-1.85251238808831,
136.312556987595));
#216021=CARTESIAN_POINT('Ctrl Pts',(-189.018368507414,3.63287341044046,
135.340246438718));
#216022=CARTESIAN_POINT('Ctrl Pts',(-189.296816131227,5.77982602050738,
130.199678410544));
#216023=CARTESIAN_POINT('Ctrl Pts',(-189.575263755039,2.61540087792624,
125.614783790254));
#216024=CARTESIAN_POINT('Ctrl Pts',(-189.853711378852,-2.95244990203274,
125.798856749341));
#216025=CARTESIAN_POINT('Ctrl Pts',(-190.132159002665,-5.80714345722022,
130.582743230867));
#216026=CARTESIAN_POINT('Ctrl Pts',(-190.410606626478,-3.32535586995153,
135.570285264159));
#216027=CARTESIAN_POINT('Ctrl Pts',(-190.689054250291,2.21227130913674,
136.178175375592));
#216028=CARTESIAN_POINT('Ctrl Pts',(-190.967501874104,5.7169292305904,131.847792249846));
#216029=CARTESIAN_POINT('Ctrl Pts',(-191.245949497917,3.96800847665057,
126.558546428502));
#216030=CARTESIAN_POINT('Ctrl Pts',(-191.52439712173,-1.4273182193404,125.170996427354));
#216031=CARTESIAN_POINT('Ctrl Pts',(-191.802844745543,-5.51100920012879,
128.960232911869));
#216032=CARTESIAN_POINT('Ctrl Pts',(-192.081292369355,-4.53035195376586,
134.444132667273));
#216033=CARTESIAN_POINT('Ctrl Pts',(-192.359739993168,0.613477418111232,
136.583259721745));
#216034=CARTESIAN_POINT('Ctrl Pts',(-192.638187616981,5.19355101278185,
133.411860814392));
#216035=CARTESIAN_POINT('Ctrl Pts',(-192.916635240794,5.00100494577841,
127.844296609621));
#216036=CARTESIAN_POINT('Ctrl Pts',(-193.195082864607,0.21277964627773,
124.996886620986));
#216037=CARTESIAN_POINT('Ctrl Pts',(-193.47353048842,-4.77097975328813,
127.486261524329));
#216038=CARTESIAN_POINT('Ctrl Pts',(-193.751978112233,-5.3704418349007,
133.024807396204));
#216039=CARTESIAN_POINT('Ctrl Pts',(-194.030425736046,-1.03473023090876,
136.522871153366));
#216040=CARTESIAN_POINT('Ctrl Pts',(-194.308873359859,4.25184790590635,
134.765903092897));
#216041=CARTESIAN_POINT('Ctrl Pts',(-194.587320983671,5.63118553151129,
129.368471029708));
#216042=CARTESIAN_POINT('Ctrl Pts',(-194.865768607484,1.83573875236439,
125.290551350653));
#216043=CARTESIAN_POINT('Ctrl Pts',(-195.144216231297,-3.64666225938173,
126.279553023333));
#216044=CARTESIAN_POINT('Ctrl Pts',(-195.42266385511,-5.77795880411129,
131.426631825972));
#216045=CARTESIAN_POINT('Ctrl Pts',(-195.701111478923,-2.59959347684268,
136.001873787725));
#216046=CARTESIAN_POINT('Ctrl Pts',(-195.979559102736,2.96767125844341,
135.800855058734));
#216047=CARTESIAN_POINT('Ctrl Pts',(-196.258006726549,5.80779108602021,
131.008302030633));
#216048=CARTESIAN_POINT('Ctrl Pts',(-196.536454350362,3.31083463191258,
126.028336807015));
#216049=CARTESIAN_POINT('Ctrl Pts',(-196.814901974175,-2.22861710565919,
125.437304143558));
#216050=CARTESIAN_POINT('Ctrl Pts',(-197.093349597988,-5.72007859712835,
129.778334184429));
#216051=CARTESIAN_POINT('Ctrl Pts',(-197.3717972218,-3.95506729921131,135.062232393175));
#216052=CARTESIAN_POINT('Ctrl Pts',(-197.650244845613,1.44445763090186,
136.433354448736));
#216053=CARTESIAN_POINT('Ctrl Pts',(-197.928692469426,5.51659656389443,
132.631706165088));
#216054=CARTESIAN_POINT('Ctrl Pts',(-198.207140093239,4.51925275539276,
127.150816594059));
#216055=CARTESIAN_POINT('Ctrl Pts',(-198.485587717052,-0.631063557543924,
125.027355495085));
#216056=CARTESIAN_POINT('Ctrl Pts',(-198.764035340865,-5.2014632902668,
128.212679881281));
#216057=CARTESIAN_POINT('Ctrl Pts',(-199.042482964678,-4.99197236484219,
133.779632253479));
#216058=CARTESIAN_POINT('Ctrl Pts',(-199.320930588491,-0.19510270753564,
136.612455342372));
#216059=CARTESIAN_POINT('Ctrl Pts',(-199.599378212304,4.7810568066993,134.10792312037));
#216060=CARTESIAN_POINT('Ctrl Pts',(-199.877825836116,5.36365868318719,
128.56757834629));
#216061=CARTESIAN_POINT('Ctrl Pts',(-200.156273459929,1.01732025912016,
125.082727206624));
#216062=CARTESIAN_POINT('Ctrl Pts',(-200.434721083742,-4.26388578422093,
126.855777654281));
#216063=CARTESIAN_POINT('Ctrl Pts',(-200.713168707555,-5.62678909426374,
132.257382946195));
#216064=CARTESIAN_POINT('Ctrl Pts',(-200.991616331368,-1.8189481106068,
136.323731702186));
#216065=CARTESIAN_POINT('Ctrl Pts',(-201.270063955181,3.66041732614217,
135.318048067677));
#216066=CARTESIAN_POINT('Ctrl Pts',(-201.548511578994,5.77603806149454,
130.164506172408));
#216067=CARTESIAN_POINT('Ctrl Pts',(-201.826959202806,2.58376199347953,
125.59895925361));
#216068=CARTESIAN_POINT('Ctrl Pts',(-202.10540682662,-2.9828651227522,125.816921890294));
#216069=CARTESIAN_POINT('Ctrl Pts',(-202.383854450432,-5.80838491223743,
130.618097067413));
#216070=CARTESIAN_POINT('Ctrl Pts',(-202.662302074245,-3.29628272275406,
135.590439347642));
#216071=CARTESIAN_POINT('Ctrl Pts',(-202.940749698058,2.24494225657654,
136.164609087875));
#216072=CARTESIAN_POINT('Ctrl Pts',(-203.219197321871,5.72317497363993,
131.812972346589));
#216073=CARTESIAN_POINT('Ctrl Pts',(-203.497644945684,3.94208948256877,
126.534470699752));
#216074=CARTESIAN_POINT('Ctrl Pts',(-203.776092569497,-1.46158366120557,
125.179789291667));
#216075=CARTESIAN_POINT('Ctrl Pts',(-204.05454019331,-5.52213282266317,
128.993814156497));
#216076=CARTESIAN_POINT('Ctrl Pts',(-204.332987817123,-4.5081116912795,
134.471642768938));
#216077=CARTESIAN_POINT('Ctrl Pts',(-204.611435440935,0.648643850890564,
136.579418240959));
#216078=CARTESIAN_POINT('Ctrl Pts',(-204.889883064748,5.20932738210573,
133.380197884332));
#216079=CARTESIAN_POINT('Ctrl Pts',(-205.168330688562,4.98289353895661,
127.813908916192));
#216080=CARTESIAN_POINT('Ctrl Pts',(-205.446778312374,0.177423961388546,
124.995698969927));
#216081=CARTESIAN_POINT('Ctrl Pts',(-205.725225936187,-4.79108956905296,
127.515365308944));
#216082=CARTESIAN_POINT('Ctrl Pts',(-206.00367356,-5.35682584327266,133.057457660231));
#216083=CARTESIAN_POINT('Ctrl Pts',(-206.282121183813,-0.999900863015179,
136.529063899218));
#216084=CARTESIAN_POINT('Ctrl Pts',(-206.560568807626,4.27588416248015,
134.739947489669));
#216085=CARTESIAN_POINT('Ctrl Pts',(-206.839016431439,5.62234053121038,
129.334219008764));
#216086=CARTESIAN_POINT('Ctrl Pts',(-207.117464055252,1.80214061836306,
125.279478845937));
#216087=CARTESIAN_POINT('Ctrl Pts',(-207.395911679064,-3.67413848329639,
126.301835125757));
#216088=CARTESIAN_POINT('Ctrl Pts',(-207.674359302878,-5.77406381044983,
131.461792371951));
#216089=CARTESIAN_POINT('Ctrl Pts',(-207.95280692669,-2.56790657449899,
136.01760195319));
#216090=CARTESIAN_POINT('Ctrl Pts',(-208.231254550503,2.99803135420673,
135.782697427989));
#216091=CARTESIAN_POINT('Ctrl Pts',(-208.509702174316,5.8089249303698,130.972944579282));
#216092=CARTESIAN_POINT('Ctrl Pts',(-208.788149798129,3.28170027728254,
126.008271305542));
#216093=CARTESIAN_POINT('Ctrl Pts',(-209.066597421942,-2.2612466106562,
125.450969807563));
#216094=CARTESIAN_POINT('Ctrl Pts',(-209.345045045754,-5.72621833144002,
129.813172936296));
#216095=CARTESIAN_POINT('Ctrl Pts',(-209.623492669568,-3.92907514694791,
135.086229121905));
#216096=CARTESIAN_POINT('Ctrl Pts',(-209.90194029338,1.4786961515975,136.424457332932));
#216097=CARTESIAN_POINT('Ctrl Pts',(-210.180387917194,5.52761792514773,
132.598091219525));
#216098=CARTESIAN_POINT('Ctrl Pts',(-210.458835541006,4.49692886463537,
127.123374311529));
#216099=CARTESIAN_POINT('Ctrl Pts',(-210.73728316482,-0.666218135288655,
125.031303992602));
#216100=CARTESIAN_POINT('Ctrl Pts',(-211.015730788632,-5.21714321544808,
128.244390682522));
#216101=CARTESIAN_POINT('Ctrl Pts',(-211.294178412445,-4.97376855222533,
133.809964681263));
#216102=CARTESIAN_POINT('Ctrl Pts',(-211.572626036258,-0.159743571609885,
136.613535377387));
#216103=CARTESIAN_POINT('Ctrl Pts',(-211.851073660071,4.80107794740803,
134.0787582632));
#216104=CARTESIAN_POINT('Ctrl Pts',(-212.129521283884,5.34994337845465,
128.534969675892));
#216105=CARTESIAN_POINT('Ctrl Pts',(-212.407968907697,0.982472203965689,
125.076640498072));
#216106=CARTESIAN_POINT('Ctrl Pts',(-212.686416531509,-4.28784292953254,
126.881806295382));
#216107=CARTESIAN_POINT('Ctrl Pts',(-212.964864155322,-5.61783988356258,
132.291607887347));
#216108=CARTESIAN_POINT('Ctrl Pts',(-213.243311779135,-1.78531643133465,
136.334701894451));
#216109=CARTESIAN_POINT('Ctrl Pts',(-213.521759402948,3.68782560373359,
135.295682440288));
#216110=CARTESIAN_POINT('Ctrl Pts',(-213.800207026761,5.77203606926717,
130.129357644311));
#216111=CARTESIAN_POINT('Ctrl Pts',(-214.078654650574,2.55202736678199,
125.583327605028));
#216112=CARTESIAN_POINT('Ctrl Pts',(-214.357102274386,-3.0131698123076,
125.835171842623));
#216113=CARTESIAN_POINT('Ctrl Pts',(-214.6355498982,-5.80941113541564,130.653457806023));
#216114=CARTESIAN_POINT('Ctrl Pts',(-214.913997522012,-3.26708743058812,
135.610416081219));
#216115=CARTESIAN_POINT('Ctrl Pts',(-215.192445145826,2.27753001685547,
136.15084417418));
#216116=CARTESIAN_POINT('Ctrl Pts',(-215.470892769638,5.72920864233609,
131.778115068854));
#216117=CARTESIAN_POINT('Ctrl Pts',(-215.749340393451,3.9160244129115,126.510553193344));
#216118=CARTESIAN_POINT('Ctrl Pts',(-216.027788017264,-1.49579494355069,
125.18879057654));
#216119=CARTESIAN_POINT('Ctrl Pts',(-216.306235641077,-5.53305182053502,
129.02746249159));
#216120=CARTESIAN_POINT('Ctrl Pts',(-216.58468326489,-4.48570437905656,
134.499016978113));
#216121=CARTESIAN_POINT('Ctrl Pts',(-216.863130888703,0.683786247933482,
136.57536276329));
#216122=CARTESIAN_POINT('Ctrl Pts',(-217.141578512516,5.2249107178877,133.348439505674));
#216123=CARTESIAN_POINT('Ctrl Pts',(-217.420026136328,4.96459748918233,
127.78363203505));
#216124=CARTESIAN_POINT('Ctrl Pts',(-217.698473760142,0.142061701988793,
124.994726560962));
#216125=CARTESIAN_POINT('Ctrl Pts',(-217.976921383954,-4.81102184923216,
127.544590968491));
#216126=CARTESIAN_POINT('Ctrl Pts',(-218.255369007768,-5.34301135249269,
133.090024434919));
#216127=CARTESIAN_POINT('Ctrl Pts',(-218.53381663158,-0.965034443427401,
136.535044514085));
#216128=CARTESIAN_POINT('Ctrl Pts',(-218.812264255394,4.29976197459382,
134.713846051821));
#216129=CARTESIAN_POINT('Ctrl Pts',(-219.090711879206,5.61328719301349,
129.300021464458));
#216130=CARTESIAN_POINT('Ctrl Pts',(-219.369159503019,1.76847570537835,
125.268611067748));
#216131=CARTESIAN_POINT('Ctrl Pts',(-219.647607126831,-3.70147856065836,
126.324284070919));
#216132=CARTESIAN_POINT('Ctrl Pts',(-219.926054750645,-5.76995485673049,
131.496928556552));
#216133=CARTESIAN_POINT('Ctrl Pts',(-220.204502374457,-2.5361245174328,
136.033136940081));
#216134=CARTESIAN_POINT('Ctrl Pts',(-220.48294999827,3.02828035681523,135.764355323142));
#216135=CARTESIAN_POINT('Ctrl Pts',(-220.761397622083,5.80984352286985,
130.937580880991));
#216136=CARTESIAN_POINT('Ctrl Pts',(-221.039845245896,3.25244431804234,
125.988383524923));
#216137=CARTESIAN_POINT('Ctrl Pts',(-221.318292869709,-2.29379232432851,
125.464833843433));
#216138=CARTESIAN_POINT('Ctrl Pts',(-221.596740493522,-5.73214587862558,
129.848048416986));
#216139=CARTESIAN_POINT('Ctrl Pts',(-221.875188117335,-3.90293740136003,
135.110067184424));
#216140=CARTESIAN_POINT('Ctrl Pts',(-222.153635741148,1.51287987866345,
136.415351962378));
#216141=CARTESIAN_POINT('Ctrl Pts',(-222.432083364961,5.53843445848603,
132.564409806615));
#216142=CARTESIAN_POINT('Ctrl Pts',(-222.710530988774,4.47443833852516,
127.0960684293));
#216143=CARTESIAN_POINT('Ctrl Pts',(-222.988978612586,-0.701348026075381,
125.035466412855));
#216144=CARTESIAN_POINT('Ctrl Pts',(-223.267426236399,-5.23262981746888,
128.27619634439));
#216145=CARTESIAN_POINT('Ctrl Pts',(-223.545873860212,-4.95538043478568,
133.840185735283));
#216146=CARTESIAN_POINT('Ctrl Pts',(-223.824321484025,-0.124378516327312,
136.614400151295));
#216147=CARTESIAN_POINT('Ctrl Pts',(-224.102769107838,4.82092118240782,
134.049472072021));
#216148=CARTESIAN_POINT('Ctrl Pts',(-224.381216731651,5.33602982960279,
128.502445098609));
#216149=CARTESIAN_POINT('Ctrl Pts',(-224.659664355464,0.947587742942381,
125.070766032295));
#216150=CARTESIAN_POINT('Ctrl Pts',(-224.938111979277,-4.31164118724753,
126.907980288176));
#216151=CARTESIAN_POINT('Ctrl Pts',(-225.216559603089,-5.60868250173869,
132.325777718005));
#216152=CARTESIAN_POINT('Ctrl Pts',(-225.495007226903,-1.75161859650508,
136.345467157888));
#216153=CARTESIAN_POINT('Ctrl Pts',(-225.773454850715,3.71509722759125,
135.273150385318));
#216154=CARTESIAN_POINT('Ctrl Pts',(-226.051902474528,5.7678201921206,130.0942341287));
#216155=CARTESIAN_POINT('Ctrl Pts',(-226.330350098341,2.52019817377184,
125.567889423742));
#216156=CARTESIAN_POINT('Ctrl Pts',(-226.608797722154,-3.04336284774751,
125.853605930069));
#216157=CARTESIAN_POINT('Ctrl Pts',(-226.887245345967,-5.81022208872781,
130.688824136393));
#216158=CARTESIAN_POINT('Ctrl Pts',(-227.16569296978,-3.23777107529596,
135.630214724643));
#216159=CARTESIAN_POINT('Ctrl Pts',(-227.444140593593,2.31003338242206,
136.13688114457));
#216160=CARTESIAN_POINT('Ctrl Pts',(-227.722588217406,5.73503001309909,
131.74322170829));
#216161=CARTESIAN_POINT('Ctrl Pts',(-228.001035841218,3.88981423352964,
126.486794795549));
#216162=CARTESIAN_POINT('Ctrl Pts',(-228.279483465031,-1.52995079866356,
125.197999948425));
#216163=CARTESIAN_POINT('Ctrl Pts',(-228.557931088844,-5.54376578913698,
129.061176670297));
#216164=CARTESIAN_POINT('Ctrl Pts',(-228.836378712657,-4.46313084740822,
134.526254280438));
#216165=CARTESIAN_POINT('Ctrl Pts',(-229.11482633647,0.718903307025501,
136.571093439014));
#216166=CARTESIAN_POINT('Ctrl Pts',(-229.393273960283,5.24030044268158,
133.316586855238));
#216167=CARTESIAN_POINT('Ctrl Pts',(-229.671721584096,4.94611747442232,
127.753467088116));
#216168=CARTESIAN_POINT('Ctrl Pts',(-229.950169207909,0.106694178440453,
124.993969430123));
#216169=CARTESIAN_POINT('Ctrl Pts',(-230.228616831722,-4.83077585522751,
127.57393742));
#216170=CARTESIAN_POINT('Ctrl Pts',(-230.507064455534,-5.32899887446215,
133.122506513493));
#216171=CARTESIAN_POINT('Ctrl Pts',(-230.785512079348,-0.930132264133436,
136.540812776352));
#216172=CARTESIAN_POINT('Ctrl Pts',(-231.06395970316,4.3234804574463,134.687599746553));
#216173=CARTESIAN_POINT('Ctrl Pts',(-231.342407326973,5.60402585239536,
129.265879663993));
#216174=CARTESIAN_POINT('Ctrl Pts',(-231.620854950786,1.73474526087603,
125.257948418793));
#216175=CARTESIAN_POINT('Ctrl Pts',(-231.899302574599,-3.72868147837107,
126.346899026965));
#216176=CARTESIAN_POINT('Ctrl Pts',(-232.177750198412,-5.76563209521201,
131.532039077795));
#216177=CARTESIAN_POINT('Ctrl Pts',(-232.456197822225,-2.50424848333998,
136.048478172742));
#216178=CARTESIAN_POINT('Ctrl Pts',(-232.734645446038,3.05841714538193,
135.745829423867));
#216179=CARTESIAN_POINT('Ctrl Pts',(-233.01309306985,5.81054682948159,130.902212246173));
#216180=CARTESIAN_POINT('Ctrl Pts',(-233.291540693664,3.22306783828139,
125.968674202107));
#216181=CARTESIAN_POINT('Ctrl Pts',(-233.569988317476,-2.32625304068266,
125.478895737432));
#216182=CARTESIAN_POINT('Ctrl Pts',(-233.84843594129,-5.73786101903762,
129.882959334177));
#216183=CARTESIAN_POINT('Ctrl Pts',(-234.126883565102,-3.87665503099142,
135.133745697402));
#216184=CARTESIAN_POINT('Ctrl Pts',(-234.405331188915,1.54700754540913,
136.406038674476));
#216185=CARTESIAN_POINT('Ctrl Pts',(-234.683778812728,5.54904576309872,
132.530663174436));
#216186=CARTESIAN_POINT('Ctrl Pts',(-234.962226436541,4.45178201045685,
127.0688999592));
#216187=CARTESIAN_POINT('Ctrl Pts',(-235.240674060353,-0.736451928153096,
125.039842601604));
#216188=CARTESIAN_POINT('Ctrl Pts',(-235.519121684167,-5.24792252246713,
128.308095688315));
#216189=CARTESIAN_POINT('Ctrl Pts',(-235.797569307979,-4.93680869390195,
133.870294295687));
#216190=CARTESIAN_POINT('Ctrl Pts',(-236.076016931792,-0.0890088521534987,
136.61504963205));
#216191=CARTESIAN_POINT('Ctrl Pts',(-236.354464555605,4.8405857764003,134.020065632043));
#216192=CARTESIAN_POINT('Ctrl Pts',(-236.632912179418,5.32191855220324,
128.470005819654));
#216193=CARTESIAN_POINT('Ctrl Pts',(-236.911359803231,0.912668168706789,
125.065104026974));
#216194=CARTESIAN_POINT('Ctrl Pts',(-237.189807427044,-4.33527967551271,
126.934298662776));
#216195=CARTESIAN_POINT('Ctrl Pts',(-237.468255050857,-5.59931728812211,
132.359891171993));
#216196=CARTESIAN_POINT('Ctrl Pts',(-237.74670267467,-1.71785585480426,
136.356027093583));
#216197=CARTESIAN_POINT('Ctrl Pts',(-238.025150298482,3.7422311871549,135.250452737698));
#216198=CARTESIAN_POINT('Ctrl Pts',(-238.303597922296,5.76339058627568,
130.059136927086));
#216199=CARTESIAN_POINT('Ctrl Pts',(-238.582045546108,2.48827559389159,
125.552645281824));
#216200=CARTESIAN_POINT('Ctrl Pts',(-238.860493169922,-3.07344311025789,
125.87222346955));
#216201=CARTESIAN_POINT('Ctrl Pts',(-239.138940793734,-5.81081774212379,
130.724194748009));
#216202=CARTESIAN_POINT('Ctrl Pts',(-239.417388417547,-3.20833474320591,
135.649834544268));
#216203=CARTESIAN_POINT('Ctrl Pts',(-239.69583604136,2.34245114885216,136.12272051645));
#216204=CARTESIAN_POINT('Ctrl Pts',(-239.974283665173,5.7406388702159,131.708293557882));
#216205=CARTESIAN_POINT('Ctrl Pts',(-240.252731288985,3.86345991565072,
126.463196386742));
#216206=CARTESIAN_POINT('Ctrl Pts',(-240.531178912799,-1.56404996088748,
125.207417066067));
#216207=CARTESIAN_POINT('Ctrl Pts',(-240.809626536611,-5.5542743314588,
129.094955443325));
#216208=CARTESIAN_POINT('Ctrl Pts',(-241.088074160425,-4.44039193280503,
134.553353666625));
#216209=CARTESIAN_POINT('Ctrl Pts',(-241.366521784237,0.753993726891117,
136.566610426332));
#216210=CARTESIAN_POINT('Ctrl Pts',(-241.64496940805,5.25549598621542,133.284641113335));
#216211=CARTESIAN_POINT('Ctrl Pts',(-241.923417031863,4.92745417946037,
127.723415193164));
#216212=CARTESIAN_POINT('Ctrl Pts',(-242.201864655676,0.071322701300089,
124.993427605467));
#216213=CARTESIAN_POINT('Ctrl Pts',(-242.480312279489,-4.85035085504701,
127.603403576029));
#216214=CARTESIAN_POINT('Ctrl Pts',(-242.758759903302,-5.31478892841856,
133.154902692318));
#216215=CARTESIAN_POINT('Ctrl Pts',(-243.037207527115,-0.895195618446729,
136.546368472274));
#216216=CARTESIAN_POINT('Ctrl Pts',(-243.315655150928,4.34703873214009,
134.661209546432));
#216217=CARTESIAN_POINT('Ctrl Pts',(-243.59410277474,5.59455685253872,129.231794872506));
#216218=CARTESIAN_POINT('Ctrl Pts',(-243.872550398553,1.7009505347501,125.247491294183));
#216219=CARTESIAN_POINT('Ctrl Pts',(-244.150998022366,-3.75574622842035,
126.36967915589));
#216220=CARTESIAN_POINT('Ctrl Pts',(-244.429445646179,-5.76109568607594,
131.567122634643));
#216221=CARTESIAN_POINT('Ctrl Pts',(-244.707893269992,-2.47227965339868,
136.063625082699));
#216222=CARTESIAN_POINT('Ctrl Pts',(-244.986340893805,3.08844060317656,
135.727120416648));
#216223=CARTESIAN_POINT('Ctrl Pts',(-245.264788517618,5.81103482414375,
130.866839985428));
#216224=CARTESIAN_POINT('Ctrl Pts',(-245.543236141431,3.1935719265564,125.949144067427));
#216225=CARTESIAN_POINT('Ctrl Pts',(-245.821683765243,-2.35862755687492,
125.49315496849));
#216226=CARTESIAN_POINT('Ctrl Pts',(-246.100131389057,-5.74336354089951,
129.917904394232));
#216227=CARTESIAN_POINT('Ctrl Pts',(-246.378579012869,-3.85022900974501,
135.157263783424));
#216228=CARTESIAN_POINT('Ctrl Pts',(-246.657026636682,1.58107788722132,
136.396517814333));
#216229=CARTESIAN_POINT('Ctrl Pts',(-246.935474260495,5.55945144577998,
132.496852573479));
#216230=CARTESIAN_POINT('Ctrl Pts',(-247.213921884308,4.42896071996899,
127.04186990797));
#216231=CARTESIAN_POINT('Ctrl Pts',(-247.492369508121,-0.77152854073377,
125.044432396689));
#216232=CARTESIAN_POINT('Ctrl Pts',(-247.770817131934,-5.26302076376676,
128.340087532256));
#216233=CARTESIAN_POINT('Ctrl Pts',(-248.049264755747,-4.91805401775627,
133.90028924679));
#216234=CARTESIAN_POINT('Ctrl Pts',(-248.32771237956,-0.0536358897235281,
136.615483795589));
#216235=CARTESIAN_POINT('Ctrl Pts',(-248.606160003372,4.86007100070672,
133.990540032933));
#216236=CARTESIAN_POINT('Ctrl Pts',(-248.884607627186,5.30761006915461,
128.437653041073));
#216237=CARTESIAN_POINT('Ctrl Pts',(-249.163055250998,0.877714775216597,
125.059654691916));
#216238=CARTESIAN_POINT('Ctrl Pts',(-249.441502874812,-4.35875751839529,
126.960760443945));
#216239=CARTESIAN_POINT('Ctrl Pts',(-249.719950498624,-5.58974458974414,
132.393946985223));
#216240=CARTESIAN_POINT('Ctrl Pts',(-249.998398122437,-1.68402945732324,
136.366381310236));
#216241=CARTESIAN_POINT('Ctrl Pts',(-250.27684574625,3.76922647696617,135.227590338499));
#216242=CARTESIAN_POINT('Ctrl Pts',(-250.555293370063,5.75874741587205,
130.024067340013));
#216243=CARTESIAN_POINT('Ctrl Pts',(-250.833740993876,2.45626081004631,
125.537595744144));
#216244=CARTESIAN_POINT('Ctrl Pts',(-251.112188617689,-3.10340948520656,
125.891023771197));
#216245=CARTESIAN_POINT('Ctrl Pts',(-251.390636241501,-5.81119807352532,
130.759568330183));
#216246=CARTESIAN_POINT('Ctrl Pts',(-251.669083865314,-3.17877952510356,
135.669274813107));
#216247=CARTESIAN_POINT('Ctrl Pts',(-251.947531489127,2.37478211491517,
136.10836281449));
#216248=CARTESIAN_POINT('Ctrl Pts',(-252.22597911294,5.74603500580729,131.673331912019));
#216249=CARTESIAN_POINT('Ctrl Pts',(-252.504426736753,3.83696243592119,
126.439758841162));
#216250=CARTESIAN_POINT('Ctrl Pts',(-252.782874360566,-1.59809116681098,
125.217041580908));
#216251=CARTESIAN_POINT('Ctrl Pts',(-253.061321984379,-5.5645770578269,
129.128797558239));
#216252=CARTESIAN_POINT('Ctrl Pts',(-253.339769608192,-4.41748847836656,
134.580314133917));
#216253=CARTESIAN_POINT('Ctrl Pts',(-253.618217232004,0.789056208225191,
136.561913888683));
#216254=CARTESIAN_POINT('Ctrl Pts',(-253.896664855818,5.27049678355612,
133.252603468789));
#216255=CARTESIAN_POINT('Ctrl Pts',(-254.17511247963,4.90860829937749,127.693477454216));
#216256=CARTESIAN_POINT('Ctrl Pts',(-254.453560103444,0.0359485746511809,
124.993101125124));
#216257=CARTESIAN_POINT('Ctrl Pts',(-254.732007727256,-4.86974611083267,
127.632988310607));
#216258=CARTESIAN_POINT('Ctrl Pts',(-255.010455351069,-5.30038206451776,
133.187211835313));
#216259=CARTESIAN_POINT('Ctrl Pts',(-255.288902974882,-0.860225756393269,
136.55171127444));
#216260=CARTESIAN_POINT('Ctrl Pts',(-255.567350598695,4.37043584157037,
134.634676658854));
#216261=CARTESIAN_POINT('Ctrl Pts',(-255.845798222508,5.58488070320316,
129.197767919676));
#216262=CARTESIAN_POINT('Ctrl Pts',(-256.12424584632,1.66709247927321,125.23724089965));
#216263=CARTESIAN_POINT('Ctrl Pts',(-256.402693470134,-3.78267124144458,
126.39262206856));
#216264=CARTESIAN_POINT('Ctrl Pts',(-256.681141093946,-5.75634686702621,
131.602180844355));
#216265=CARTESIAN_POINT('Ctrl Pts',(-256.95958871776,-2.44021719259262,
136.078571600242));
#216266=CARTESIAN_POINT('Ctrl Pts',(-257.238036341572,3.118345804191,135.708239395799));
#216267=CARTESIAN_POINT('Ctrl Pts',(-257.516483965385,5.81131468939531,
130.8314457702));
#216268=CARTESIAN_POINT('Ctrl Pts',(-257.794931589198,3.16394407961038,
125.929830927563));
#216269=CARTESIAN_POINT('Ctrl Pts',(-258.073379213011,-2.39088900078744,
125.507540987923));
#216270=CARTESIAN_POINT('Ctrl Pts',(-258.351826836824,-5.74870171518396,
129.953014515613));
#216271=CARTESIAN_POINT('Ctrl Pts',(-258.630274460636,-3.82356878618261,
135.180370918811));
#216272=CARTESIAN_POINT('Ctrl Pts',(-258.908722084449,1.61491681105698,
136.387261181902));
#216273=CARTESIAN_POINT('Ctrl Pts',(-259.187169708263,5.56997747689423,
132.462088635074));
#216274=CARTESIAN_POINT('Ctrl Pts',(-259.465617332075,4.40535894966821,
127.016664495574));
#216275=CARTESIAN_POINT('Ctrl Pts',(-259.744064955888,-0.805411631290512,
125.046024618449));
#216276=CARTESIAN_POINT('Ctrl Pts',(-260.022512579701,-5.28013240410161,
128.378470706602));
#216277=CARTESIAN_POINT('Ctrl Pts',(-260.254552266212,-4.95911089365773,
132.993351965875));
#216278=CARTESIAN_POINT('Ctrl Pts',(-260.440213228287,-2.45877638613931,
135.28779596926));
#216279=CARTESIAN_POINT('Ctrl Pts',(-260.53305831576,-0.833059752290926,
135.715219187214));
#216280=CARTESIAN_POINT('Ctrl Pts',(-260.579495465929,-0.013892627260139,
135.717527172907));
#216281=CARTESIAN_POINT('',(178.484852205224,2.29534567378642,125.352234455441));
#216282=CARTESIAN_POINT('Ctrl Pts',(178.484852205224,2.2953456737888,125.352234455442));
#216283=CARTESIAN_POINT('Ctrl Pts',(178.474769645589,2.30871694763094,125.378556419204));
#216284=CARTESIAN_POINT('Ctrl Pts',(178.464760721661,2.32210067769615,125.404904734779));
#216285=CARTESIAN_POINT('Ctrl Pts',(178.410116963477,2.39571594247993,125.549964067863));
#216286=CARTESIAN_POINT('Ctrl Pts',(178.366752083918,2.45614810993821,125.669573427325));
#216287=CARTESIAN_POINT('Ctrl Pts',(178.280651552913,2.57861371139863,125.916725903007));
#216288=CARTESIAN_POINT('Ctrl Pts',(178.23809773572,2.6405199714625,126.044243888829));
#216289=CARTESIAN_POINT('Ctrl Pts',(178.119236076123,2.81530092068313,126.41694099985));
#216290=CARTESIAN_POINT('Ctrl Pts',(178.04659616344,2.92444065582699,126.665761747735));
#216291=CARTESIAN_POINT('Ctrl Pts',(177.979076132606,3.02442025815032,126.922107774054));
#216292=CARTESIAN_POINT('',(179.686624807795,-5.92158244890185,130.806643466513));
#216293=CARTESIAN_POINT('Ctrl Pts',(178.484852205224,2.29534567378572,125.35223445544));
#216294=CARTESIAN_POINT('Ctrl Pts',(178.508237305251,2.75521539300514,125.540445630445));
#216295=CARTESIAN_POINT('Ctrl Pts',(178.624438279882,4.91660179655204,126.757108707475));
#216296=CARTESIAN_POINT('Ctrl Pts',(178.833455129117,6.97691126644166,131.352329330672));
#216297=CARTESIAN_POINT('Ctrl Pts',(179.11190275293,3.31016936242742,136.970424136732));
#216298=CARTESIAN_POINT('Ctrl Pts',(179.390350376743,-3.39845647489431,
136.922207797627));
#216299=CARTESIAN_POINT('Ctrl Pts',(179.581924395032,-5.86538284120287,
133.021055300245));
#216300=CARTESIAN_POINT('Ctrl Pts',(179.680682538715,-5.92608698495012,
130.932358269279));
#216301=CARTESIAN_POINT('Ctrl Pts',(179.686624807795,-5.92546899106887,
130.806644964827));
#216302=CARTESIAN_POINT('',(181.436624793272,-5.91313131605275,130.808682171932));
#216303=CARTESIAN_POINT('Ctrl Pts',(179.686624807795,-5.9167495603248,130.80664160337));
#216304=CARTESIAN_POINT('Ctrl Pts',(179.693977154138,-5.91680943647244,
130.651326226339));
#216305=CARTESIAN_POINT('Ctrl Pts',(179.701329500482,-5.91074953815374,
130.495761078002));
#216306=CARTESIAN_POINT('Ctrl Pts',(179.708681846825,-5.89853708827506,
130.340474014242));
#216307=CARTESIAN_POINT('Ctrl Pts',(179.716025830516,-5.88633852899205,
130.185363575961));
#216308=CARTESIAN_POINT('Ctrl Pts',(179.723369814208,-5.86800137290794,
130.030530968938));
#216309=CARTESIAN_POINT('Ctrl Pts',(179.730713797899,-5.84354481501677,
129.876505802743));
#216310=CARTESIAN_POINT('Ctrl Pts',(179.738051104691,-5.81911049219403,
129.722620670976));
#216311=CARTESIAN_POINT('Ctrl Pts',(179.745388411482,-5.78856789958858,
129.569541892852));
#216312=CARTESIAN_POINT('Ctrl Pts',(179.752725718274,-5.75198815284064,
129.417795490325));
#216313=CARTESIAN_POINT('Ctrl Pts',(179.760058027822,-5.71543331957921,
129.266152438212));
#216314=CARTESIAN_POINT('Ctrl Pts',(179.767390337371,-5.6728496059675,129.11584032425));
#216315=CARTESIAN_POINT('Ctrl Pts',(179.774722646919,-5.62435943793095,
128.96737627483));
#216316=CARTESIAN_POINT('Ctrl Pts',(179.782052360326,-5.57588643874756,
128.818964791891));
#216317=CARTESIAN_POINT('Ctrl Pts',(179.789382073733,-5.52151126173289,
128.672400433808));
#216318=CARTESIAN_POINT('Ctrl Pts',(179.796711787139,-5.46140653421223,
128.528186364447));
#216319=CARTESIAN_POINT('Ctrl Pts',(179.804040294966,-5.40131169262705,
128.383996015199));
#216320=CARTESIAN_POINT('Ctrl Pts',(179.811368802792,-5.33548932152652,
128.24215553726));
#216321=CARTESIAN_POINT('Ctrl Pts',(179.818697310619,-5.26416055459471,
128.103148997209));
#216322=CARTESIAN_POINT('Ctrl Pts',(179.826026126248,-5.19282879179809,
127.964136618774));
#216323=CARTESIAN_POINT('Ctrl Pts',(179.833354941878,-5.11599034668846,
127.827958754184));
#216324=CARTESIAN_POINT('Ctrl Pts',(179.840683757508,-5.03391263741617,
127.695075471208));
#216325=CARTESIAN_POINT('Ctrl Pts',(179.848014394317,-4.95181453217909,
127.562159167297));
#216326=CARTESIAN_POINT('Ctrl Pts',(179.855345031126,-4.86447477205808,
127.432539398244));
#216327=CARTESIAN_POINT('Ctrl Pts',(179.862675667936,-4.77220433056239,
127.306647594766));
#216328=CARTESIAN_POINT('Ctrl Pts',(179.870013917591,-4.67983806647012,
127.180625053001));
#216329=CARTESIAN_POINT('Ctrl Pts',(179.877352167246,-4.58253111937658,
127.058338516905));
#216330=CARTESIAN_POINT('Ctrl Pts',(179.884690416902,-4.48063543929967,
126.940187145452));
#216331=CARTESIAN_POINT('Ctrl Pts',(179.892032632595,-4.37868468856922,
126.821971917776));
#216332=CARTESIAN_POINT('Ctrl Pts',(179.899374848289,-4.27214052426441,
126.707896584654));
#216333=CARTESIAN_POINT('Ctrl Pts',(179.906717063983,-4.16139154293925,
126.598323172553));
#216334=CARTESIAN_POINT('Ctrl Pts',(179.914070345708,-4.05047564310977,
126.48858461374));
#216335=CARTESIAN_POINT('Ctrl Pts',(179.921423627433,-3.93534254692211,
126.383361787399));
#216336=CARTESIAN_POINT('Ctrl Pts',(179.928776909158,-3.81641438967868,
126.282976784186));
#216337=CARTESIAN_POINT('Ctrl Pts',(179.934933147562,-3.71684658903447,
126.198933490997));
#216338=CARTESIAN_POINT('Ctrl Pts',(179.941089385965,-3.61461941093371,
126.118280447087));
#216339=CARTESIAN_POINT('Ctrl Pts',(179.947245624368,-3.50999522101216,
126.041182675165));
#216340=CARTESIAN_POINT('Ctrl Pts',(179.954668890774,-3.38383811283284,
125.948217253306));
#216341=CARTESIAN_POINT('Ctrl Pts',(179.962092157179,-3.25379427861745,
125.860126797838));
#216342=CARTESIAN_POINT('Ctrl Pts',(179.969515423585,-3.12027719627839,
125.777254016261));
#216343=CARTESIAN_POINT('Ctrl Pts',(179.976929916306,-2.98691792004263,
125.694479183429));
#216344=CARTESIAN_POINT('Ctrl Pts',(179.984344409027,-2.85009388096072,
125.616909944266));
#216345=CARTESIAN_POINT('Ctrl Pts',(179.991758901748,-2.71025060387357,
125.544848071074));
#216346=CARTESIAN_POINT('Ctrl Pts',(179.999166248101,-2.5705421130023,125.47285565383));
#216347=CARTESIAN_POINT('Ctrl Pts',(180.006573594455,-2.42782050707694,
125.406360204809));
#216348=CARTESIAN_POINT('Ctrl Pts',(180.013980940809,-2.28255910179349,
125.345619507262));
#216349=CARTESIAN_POINT('Ctrl Pts',(180.021382762484,-2.13740603794629,
125.284924112419));
#216350=CARTESIAN_POINT('Ctrl Pts',(180.02878458416,-1.98971728942356,125.229975066268));
#216351=CARTESIAN_POINT('Ctrl Pts',(180.036186405835,-1.83998941521192,
125.180983561525));
#216352=CARTESIAN_POINT('Ctrl Pts',(180.043584320146,-1.69034058117979,
125.132017919016));
#216353=CARTESIAN_POINT('Ctrl Pts',(180.050982234458,-1.53865511912818,
125.089003670412));
#216354=CARTESIAN_POINT('Ctrl Pts',(180.058380148769,-1.38544804064297,
125.052103296376));
#216355=CARTESIAN_POINT('Ctrl Pts',(180.065776833681,-1.23226642239424,
125.015209054514));
#216356=CARTESIAN_POINT('Ctrl Pts',(180.073173518594,-1.07756405213862,
124.984426758055));
#216357=CARTESIAN_POINT('Ctrl Pts',(180.080570203506,-0.921869639997064,
124.959868601201));
#216358=CARTESIAN_POINT('Ctrl Pts',(180.087966560441,-0.76618213150912,
124.935311533282));
#216359=CARTESIAN_POINT('Ctrl Pts',(180.095362917377,-0.609503037337292,
124.916978114377));
#216360=CARTESIAN_POINT('Ctrl Pts',(180.102759274312,-0.452369496104509,
124.904929085503));
#216361=CARTESIAN_POINT('Ctrl Pts',(180.110156763649,-0.295211897325392,
124.892878211893));
#216362=CARTESIAN_POINT('Ctrl Pts',(180.117554252985,-0.137600085177405,
124.887113672636));
#216363=CARTESIAN_POINT('Ctrl Pts',(180.124951742322,0.0199256168518951,
124.887644169037));
#216364=CARTESIAN_POINT('Ctrl Pts',(180.132351824837,0.177506539271902,
124.888174851403));
#216365=CARTESIAN_POINT('Ctrl Pts',(180.139751907352,0.335000918410661,
124.895004961724));
#216366=CARTESIAN_POINT('Ctrl Pts',(180.147151989867,0.491870521751642,
124.908091123018));
#216367=CARTESIAN_POINT('Ctrl Pts',(180.154560209533,0.648912619348167,
124.921191673893));
#216368=CARTESIAN_POINT('Ctrl Pts',(180.1619684292,0.805328196918372,124.940561982845));
#216369=CARTESIAN_POINT('Ctrl Pts',(180.169376648866,0.960585487624677,
124.966106933161));
#216370=CARTESIAN_POINT('Ctrl Pts',(180.176789428168,1.115938336603,124.991667605968));
#216371=CARTESIAN_POINT('Ctrl Pts',(180.184202207471,1.27013111337955,125.023410417793));
#216372=CARTESIAN_POINT('Ctrl Pts',(180.191614986773,1.42264479111333,125.061189684987));
#216373=CARTESIAN_POINT('Ctrl Pts',(180.199038357801,1.57537638754186,125.09902293297));
#216374=CARTESIAN_POINT('Ctrl Pts',(180.20646172883,1.72642373571236,125.142909758842));
#216375=CARTESIAN_POINT('Ctrl Pts',(180.213885099859,1.87528465261602,125.192655169651));
#216376=CARTESIAN_POINT('Ctrl Pts',(180.2178211493,1.95421428262784,125.219031380086));
#216377=CARTESIAN_POINT('Ctrl Pts',(180.221757198741,2.03252957801731,125.247053850963));
#216378=CARTESIAN_POINT('Ctrl Pts',(180.225693248181,2.11015834979351,125.276688204941));
#216379=CARTESIAN_POINT('Ctrl Pts',(180.233116514587,2.25656379065098,125.332577671686));
#216380=CARTESIAN_POINT('Ctrl Pts',(180.240539780992,2.40096865457811,125.394372189534));
#216381=CARTESIAN_POINT('Ctrl Pts',(180.247963047398,2.5428611171387,125.461909129584));
#216382=CARTESIAN_POINT('Ctrl Pts',(180.255377540119,2.68458587459203,125.529366246579));
#216383=CARTESIAN_POINT('Ctrl Pts',(180.26279203284,2.82380380761203,125.602552117214));
#216384=CARTESIAN_POINT('Ctrl Pts',(180.270206525561,2.9600202095537,125.681255024126));
#216385=CARTESIAN_POINT('Ctrl Pts',(180.277613871915,3.09610532099887,125.759882074213));
#216386=CARTESIAN_POINT('Ctrl Pts',(180.285021218268,3.22919433968091,125.844015388928));
#216387=CARTESIAN_POINT('Ctrl Pts',(180.292428564622,3.35881454655656,125.933396092511));
#216388=CARTESIAN_POINT('Ctrl Pts',(180.299830386298,3.48833807779142,126.022710132594));
#216389=CARTESIAN_POINT('Ctrl Pts',(180.307232207973,3.61439764263109,126.11726355784));
#216390=CARTESIAN_POINT('Ctrl Pts',(180.314634029648,3.73654715640086,126.21675275393));
#216391=CARTESIAN_POINT('Ctrl Pts',(180.32203194396,3.8586321883935,126.316189430449));
#216392=CARTESIAN_POINT('Ctrl Pts',(180.329429858271,3.97681099133407,126.420556453577));
#216393=CARTESIAN_POINT('Ctrl Pts',(180.336827772583,4.09066848929571,126.529508354249));
#216394=CARTESIAN_POINT('Ctrl Pts',(180.344224457495,4.20450706620659,126.638442149092));
#216395=CARTESIAN_POINT('Ctrl Pts',(180.351621142407,4.31402549395549,126.751959051452));
#216396=CARTESIAN_POINT('Ctrl Pts',(180.359017827319,4.4188435996499,126.869674886236));
#216397=CARTESIAN_POINT('Ctrl Pts',(180.366414184255,4.52365705759943,126.987385501376));
#216398=CARTESIAN_POINT('Ctrl Pts',(180.37381054119,4.62377035965245,127.109294399949));
#216399=CARTESIAN_POINT('Ctrl Pts',(180.381206898125,4.71884206612648,127.234982504021));
#216400=CARTESIAN_POINT('Ctrl Pts',(180.388604387462,4.81392832832141,127.360689851263));
#216401=CARTESIAN_POINT('Ctrl Pts',(180.396001876799,4.90397123280667,127.490177258346));
#216402=CARTESIAN_POINT('Ctrl Pts',(180.403399366135,4.98867140088571,127.622994839086));
#216403=CARTESIAN_POINT('Ctrl Pts',(180.41079944865,5.07340126047743,127.755858978823));
#216404=CARTESIAN_POINT('Ctrl Pts',(180.418199531165,5.15278445416412,127.892055301928));
#216405=CARTESIAN_POINT('Ctrl Pts',(180.42559961368,5.22656654840633,128.031107531824));
#216406=CARTESIAN_POINT('Ctrl Pts',(180.433007833347,5.30042977364622,128.170312663941));
#216407=CARTESIAN_POINT('Ctrl Pts',(180.440416053013,5.36867942446826,128.312379644405));
#216408=CARTESIAN_POINT('Ctrl Pts',(180.44782427268,5.43110809229362,128.456809669807));
#216409=CARTESIAN_POINT('Ctrl Pts',(180.455237051982,5.49357518392232,128.60132858948));
#216410=CARTESIAN_POINT('Ctrl Pts',(180.462649831284,5.55021401954599,128.748213104701));
#216411=CARTESIAN_POINT('Ctrl Pts',(180.470062610586,5.60086662026004,128.896947797918));
#216412=CARTESIAN_POINT('Ctrl Pts',(180.477485981615,5.65159159578549,129.04589501024));
#216413=CARTESIAN_POINT('Ctrl Pts',(180.484909352643,5.69631314746229,129.196697323519));
#216414=CARTESIAN_POINT('Ctrl Pts',(180.492332723672,5.73492388620217,129.348826838512));
#216415=CARTESIAN_POINT('Ctrl Pts',(180.496268773113,5.75539622633393,129.429489557658));
#216416=CARTESIAN_POINT('Ctrl Pts',(180.500204822554,5.77415145806278,129.510525263669));
#216417=CARTESIAN_POINT('Ctrl Pts',(180.504140871994,5.79117948410592,129.591854640108));
#216418=CARTESIAN_POINT('Ctrl Pts',(180.5115641384,5.82329380979685,129.745239305871));
#216419=CARTESIAN_POINT('Ctrl Pts',(180.518987404805,5.84935868805641,129.900132653963));
#216420=CARTESIAN_POINT('Ctrl Pts',(180.526410671211,5.86923428957744,130.056016167097));
#216421=CARTESIAN_POINT('Ctrl Pts',(180.533825163932,5.88908639978802,130.211715438863));
#216422=CARTESIAN_POINT('Ctrl Pts',(180.541239656653,5.90276374747488,130.368402179512));
#216423=CARTESIAN_POINT('Ctrl Pts',(180.548654149374,5.91017705542789,130.525545739925));
#216424=CARTESIAN_POINT('Ctrl Pts',(180.556061495727,5.91758321815559,130.682537839459));
#216425=CARTESIAN_POINT('Ctrl Pts',(180.563468842081,5.91873734318499,130.839985511826));
#216426=CARTESIAN_POINT('Ctrl Pts',(180.570876188435,5.91360171383272,130.997351116438));
#216427=CARTESIAN_POINT('Ctrl Pts',(180.57827801011,5.90846991482658,131.154599351844));
#216428=CARTESIAN_POINT('Ctrl Pts',(180.585679831786,5.89705771424754,131.311765269877));
#216429=CARTESIAN_POINT('Ctrl Pts',(180.593081653461,5.87937943175644,131.468309455911));
#216430=CARTESIAN_POINT('Ctrl Pts',(180.600479567773,5.86171048149293,131.624771003489));
#216431=CARTESIAN_POINT('Ctrl Pts',(180.607877482084,5.83778207877467,131.780611102708));
#216432=CARTESIAN_POINT('Ctrl Pts',(180.615275396395,5.80766051783306,131.935293803967));
#216433=CARTESIAN_POINT('Ctrl Pts',(180.622672081308,5.77754396254863,132.089950799766));
#216434=CARTESIAN_POINT('Ctrl Pts',(180.63006876622,5.74123636296223,132.243450413284));
#216435=CARTESIAN_POINT('Ctrl Pts',(180.637465451132,5.69885544372551,132.395265138277));
#216436=CARTESIAN_POINT('Ctrl Pts',(180.644861808067,5.65647640370319,132.547073131647));
#216437=CARTESIAN_POINT('Ctrl Pts',(180.652258165003,5.60802467985748,132.697196025489));
#216438=CARTESIAN_POINT('Ctrl Pts',(180.659654521938,5.55366829783429,132.84512003507));
#216439=CARTESIAN_POINT('Ctrl Pts',(180.667052011275,5.49930359371009,132.993066692195));
#216440=CARTESIAN_POINT('Ctrl Pts',(180.674449500611,5.4390325601511,133.138813444321));
#216441=CARTESIAN_POINT('Ctrl Pts',(180.681846989948,5.37307187764845,133.281865241199));
#216442=CARTESIAN_POINT('Ctrl Pts',(180.689247072463,5.30708807273077,133.424967184663));
#216443=CARTESIAN_POINT('Ctrl Pts',(180.696647154978,5.23541080405183,133.56537195318));
#216444=CARTESIAN_POINT('Ctrl Pts',(180.704047237493,5.15830324904222,133.702608045482));
#216445=CARTESIAN_POINT('Ctrl Pts',(180.71145545716,5.08111090634927,133.839995042975));
#216446=CARTESIAN_POINT('Ctrl Pts',(180.718863676826,4.99847653549861,133.974206080262));
#216447=CARTESIAN_POINT('Ctrl Pts',(180.726271896493,4.91070768452162,134.104797043204));
#216448=CARTESIAN_POINT('Ctrl Pts',(180.733684675795,4.82288481328128,134.235468382706));
#216449=CARTESIAN_POINT('Ctrl Pts',(180.741097455097,4.72992138477512,134.362514907542));
#216450=CARTESIAN_POINT('Ctrl Pts',(180.748510234399,4.6321656429306,134.485525109809));
#216451=CARTESIAN_POINT('Ctrl Pts',(180.755933605427,4.53427022309773,134.608711074823));
#216452=CARTESIAN_POINT('Ctrl Pts',(180.763356976456,4.43156905705897,134.727848916707));
#216453=CARTESIAN_POINT('Ctrl Pts',(180.770780347485,4.32444823497244,134.842562943545));
#216454=CARTESIAN_POINT('Ctrl Pts',(180.774716396926,4.26765020477355,134.9033870731));
#216455=CARTESIAN_POINT('Ctrl Pts',(180.778652446367,4.20961023112803,134.962968159235));
#216456=CARTESIAN_POINT('Ctrl Pts',(180.782588495807,4.15038958737084,135.02125483435));
#216457=CARTESIAN_POINT('Ctrl Pts',(180.790011762213,4.03870130145738,135.131181684552));
#216458=CARTESIAN_POINT('Ctrl Pts',(180.797435028618,3.92247384426901,135.236834442952));
#216459=CARTESIAN_POINT('Ctrl Pts',(180.804858295024,3.80206787792984,135.337815195933));
#216460=CARTESIAN_POINT('Ctrl Pts',(180.812272787745,3.68180422144385,135.43867659805));
#216461=CARTESIAN_POINT('Ctrl Pts',(180.819687280466,3.5573721694491,135.534876748629));
#216462=CARTESIAN_POINT('Ctrl Pts',(180.827101773187,3.42916991556503,135.626053707414));
#216463=CARTESIAN_POINT('Ctrl Pts',(180.83450911954,3.30109122784012,135.717142786413));
#216464=CARTESIAN_POINT('Ctrl Pts',(180.841916465894,3.16924987469744,135.803218097274));
#216465=CARTESIAN_POINT('Ctrl Pts',(180.849323812248,3.03407780160299,135.883957300012));
#216466=CARTESIAN_POINT('Ctrl Pts',(180.856725633923,2.89900654493989,135.964636284407));
#216467=CARTESIAN_POINT('Ctrl Pts',(180.864127455599,2.76060983375698,136.039986894538));
#216468=CARTESIAN_POINT('Ctrl Pts',(180.871529277274,2.61934923298189,136.109729611159));
#216469=CARTESIAN_POINT('Ctrl Pts',(180.878927191586,2.47816320257805,136.179435511143));
#216470=CARTESIAN_POINT('Ctrl Pts',(180.886325105897,2.33411662733151,136.243539248482));
#216471=CARTESIAN_POINT('Ctrl Pts',(180.893723020208,2.18769625047188,136.301806904541));
#216472=CARTESIAN_POINT('Ctrl Pts',(180.901119705121,2.04130020602305,136.360064877571));
#216473=CARTESIAN_POINT('Ctrl Pts',(180.908516390033,1.8925314893964,136.412488556298));
#216474=CARTESIAN_POINT('Ctrl Pts',(180.915913074945,1.74189753958409,136.458891855794));
#216475=CARTESIAN_POINT('Ctrl Pts',(180.92330943188,1.59127026903901,136.505293097718));
#216476=CARTESIAN_POINT('Ctrl Pts',(180.930705788816,1.43877828651029,136.5456743813));
#216477=CARTESIAN_POINT('Ctrl Pts',(180.938102145751,1.28494467561209,136.579899358075));
#216478=CARTESIAN_POINT('Ctrl Pts',(180.945499635088,1.13108751239619,136.61412957478));
#216479=CARTESIAN_POINT('Ctrl Pts',(180.952897124424,0.97588867623078,136.642201526869));
#216480=CARTESIAN_POINT('Ctrl Pts',(180.960294613761,0.819881788008743,
136.664029927023));
#216481=CARTESIAN_POINT('Ctrl Pts',(180.967694696276,0.663820211813073,
136.685865979089));
#216482=CARTESIAN_POINT('Ctrl Pts',(180.975094778791,0.50695038905536,136.701454069904));
#216483=CARTESIAN_POINT('Ctrl Pts',(180.982494861306,0.34981126093449,136.710760760142));
#216484=CARTESIAN_POINT('Ctrl Pts',(180.989903080972,0.192499342187787,
136.720077684043));
#216485=CARTESIAN_POINT('Ctrl Pts',(180.997311300639,0.0349178995625732,
136.72309939146));
#216486=CARTESIAN_POINT('Ctrl Pts',(181.004719520305,-0.122393183915837,
136.719844576722));
#216487=CARTESIAN_POINT('Ctrl Pts',(181.012132299607,-0.279801089741335,
136.7165877587));
#216488=CARTESIAN_POINT('Ctrl Pts',(181.01954507891,-0.436937933096332,
136.707046743394));
#216489=CARTESIAN_POINT('Ctrl Pts',(181.026957858212,-0.593269266378005,
136.691292088211));
#216490=CARTESIAN_POINT('Ctrl Pts',(181.03438122924,-0.749823973199911,
136.675514922038));
#216491=CARTESIAN_POINT('Ctrl Pts',(181.041804600269,-0.905570502595506,
136.653506436043));
#216492=CARTESIAN_POINT('Ctrl Pts',(181.049227971298,-1.05998408315404,
136.625388388154));
#216493=CARTESIAN_POINT('Ctrl Pts',(181.053164020739,-1.14185786866959,
136.61047952448));
#216494=CARTESIAN_POINT('Ctrl Pts',(181.05710007018,-1.22335714732034,136.59385388328));
#216495=CARTESIAN_POINT('Ctrl Pts',(181.06103611962,-1.30440558235503,136.575535250101));
#216496=CARTESIAN_POINT('Ctrl Pts',(181.068459386026,-1.45726040139478,
136.540986879633));
#216497=CARTESIAN_POINT('Ctrl Pts',(181.075882652431,-1.60897283890215,
136.500309324795));
#216498=CARTESIAN_POINT('Ctrl Pts',(181.083305918837,-1.75901317219453,
136.453590938817));
#216499=CARTESIAN_POINT('Ctrl Pts',(181.090720411558,-1.90887617027225,
136.406927770093));
#216500=CARTESIAN_POINT('Ctrl Pts',(181.098134904279,-2.05707064500866,
136.354238091858));
#216501=CARTESIAN_POINT('Ctrl Pts',(181.105549397,-2.20307685243817,136.295661278134));
#216502=CARTESIAN_POINT('Ctrl Pts',(181.112956743353,-2.34894233358859,
136.237140922947));
#216503=CARTESIAN_POINT('Ctrl Pts',(181.120364089707,-2.49262340217373,
136.172744866634));
#216504=CARTESIAN_POINT('Ctrl Pts',(181.127771436061,-2.6336153873598,136.102662284512));
#216505=CARTESIAN_POINT('Ctrl Pts',(181.135173257736,-2.77450221540357,
136.032631972624));
#216506=CARTESIAN_POINT('Ctrl Pts',(181.142575079412,-2.91270362066783,
135.956923745224));
#216507=CARTESIAN_POINT('Ctrl Pts',(181.149976901087,-3.04773494857795,
135.875774842979));
#216508=CARTESIAN_POINT('Ctrl Pts',(181.157374815399,-3.1826949945026,135.794668778606));
#216509=CARTESIAN_POINT('Ctrl Pts',(181.16477272971,-3.31448797669285,135.708127951092));
#216510=CARTESIAN_POINT('Ctrl Pts',(181.172170644021,-3.44265399617015,
135.616435432566));
#216511=CARTESIAN_POINT('Ctrl Pts',(181.179567328934,-3.57079871677919,
135.524758151673));
#216512=CARTESIAN_POINT('Ctrl Pts',(181.186964013846,-3.69531736762194,
135.427931095897));
#216513=CARTESIAN_POINT('Ctrl Pts',(181.194360698758,-3.81577910700978,
135.326280604586));
#216514=CARTESIAN_POINT('Ctrl Pts',(181.201757055694,-3.93623550499821,
135.224634620564));
#216515=CARTESIAN_POINT('Ctrl Pts',(181.209153412629,-4.0526350639138,135.118165867008));
#216516=CARTESIAN_POINT('Ctrl Pts',(181.216549769564,-4.16458033046145,
135.007240729303));
#216517=CARTESIAN_POINT('Ctrl Pts',(181.223947258901,-4.27654273611478,
134.896298608676));
#216518=CARTESIAN_POINT('Ctrl Pts',(181.231344748238,-4.38404922633616,
134.78089900815));
#216519=CARTESIAN_POINT('Ctrl Pts',(181.238742237574,-4.48673961136266,
134.661444778215));
#216520=CARTESIAN_POINT('Ctrl Pts',(181.246142320089,-4.58946599434432,
134.541948673785));
#216521=CARTESIAN_POINT('Ctrl Pts',(181.253542402604,-4.68737266758336,
134.418395392961));
#216522=CARTESIAN_POINT('Ctrl Pts',(181.260942485119,-4.78014018674565,
134.291220287464));
#216523=CARTESIAN_POINT('Ctrl Pts',(181.268350704786,-4.87300971333234,
134.163905339864));
#216524=CARTESIAN_POINT('Ctrl Pts',(181.275758924452,-4.96072858024092,
134.032960915913));
#216525=CARTESIAN_POINT('Ctrl Pts',(181.283167144119,-5.04302069557768,
133.898851339232));
#216526=CARTESIAN_POINT('Ctrl Pts',(181.290579923421,-5.12536346033855,
133.764659220344));
#216527=CARTESIAN_POINT('Ctrl Pts',(181.297992702723,-5.20227263606082,
133.627298391857));
#216528=CARTESIAN_POINT('Ctrl Pts',(181.305405482025,-5.27351870270403,
133.487256637678));
#216529=CARTESIAN_POINT('Ctrl Pts',(181.312828853054,-5.34486656906833,
133.347014785273));
#216530=CARTESIAN_POINT('Ctrl Pts',(181.320252224083,-5.4105350099472,133.204084694854));
#216531=CARTESIAN_POINT('Ctrl Pts',(181.327675595111,-5.47034281196722,
133.058973684604));
#216532=CARTESIAN_POINT('Ctrl Pts',(181.331611644552,-5.50205434366603,
132.982032345081));
#216533=CARTESIAN_POINT('Ctrl Pts',(181.335547693993,-5.53211907170173,
132.904478128601));
#216534=CARTESIAN_POINT('Ctrl Pts',(181.339483743433,-5.56051574565194,
132.826388116107));
#216535=CARTESIAN_POINT('Ctrl Pts',(181.348080014218,-5.622533640077,132.655840742883));
#216536=CARTESIAN_POINT('Ctrl Pts',(181.356676285003,-5.67674712583689,
132.482312359138));
#216537=CARTESIAN_POINT('Ctrl Pts',(181.365272555788,-5.7229002646624,132.306473503879));
#216538=CARTESIAN_POINT('Ctrl Pts',(181.373836240798,-5.76887845136683,
132.13130119875));
#216539=CARTESIAN_POINT('Ctrl Pts',(181.382399925807,-5.8068571937891,131.953836020863));
#216540=CARTESIAN_POINT('Ctrl Pts',(181.390963610817,-5.83663002103799,
131.774762884679));
#216541=CARTESIAN_POINT('Ctrl Pts',(181.399463586485,-5.86618135400975,
131.597021959055));
#216542=CARTESIAN_POINT('Ctrl Pts',(181.407963562153,-5.88764834009424,
131.417697041437));
#216543=CARTESIAN_POINT('Ctrl Pts',(181.416463537821,-5.90087621830845,
131.237477713398));
#216544=CARTESIAN_POINT('Ctrl Pts',(181.423183949748,-5.91133469418984,
131.094989291209));
#216545=CARTESIAN_POINT('Ctrl Pts',(181.429904361675,-5.91664371146173,
130.95194217167));
#216546=CARTESIAN_POINT('Ctrl Pts',(181.436624773602,-5.91674841954496,
130.808685234569));
#216547=CARTESIAN_POINT('',(183.186624807795,-5.9097261727316,130.800419732287));
#216548=CARTESIAN_POINT('Ctrl Pts',(181.436624807795,-5.91046065331948,
130.808679910655));
#216549=CARTESIAN_POINT('Ctrl Pts',(181.497060327612,-5.90180348691877,
129.521756724088));
#216550=CARTESIAN_POINT('Ctrl Pts',(181.650311722033,-4.85487069311502,
126.24557662955));
#216551=CARTESIAN_POINT('Ctrl Pts',(181.89637899106,0.558585749835051,123.828291345372));
#216552=CARTESIAN_POINT('Ctrl Pts',(182.174826614872,6.17109389324245,127.503578787286));
#216553=CARTESIAN_POINT('Ctrl Pts',(182.453274238685,6.11266822346165,134.212123479067));
#216554=CARTESIAN_POINT('Ctrl Pts',(182.731721862497,0.436999076760051,
137.789100579601));
#216555=CARTESIAN_POINT('Ctrl Pts',(182.976172052201,-4.89824093256168,
135.294398866638));
#216556=CARTESIAN_POINT('Ctrl Pts',(183.1278063673,-5.90209859011289,132.053299422131));
#216557=CARTESIAN_POINT('Ctrl Pts',(183.186624807795,-5.9097261727316,130.800419732287));
#216558=CARTESIAN_POINT('',(184.936624807795,-5.92486718842363,130.801517542038));
#216559=CARTESIAN_POINT('Ctrl Pts',(183.186624807795,-5.9097261727316,130.800419732287));
#216560=CARTESIAN_POINT('Ctrl Pts',(183.220622241905,-5.91413496418055,
130.076247273033));
#216561=CARTESIAN_POINT('Ctrl Pts',(183.347435550617,-5.4548282023846,127.380421002293));
#216562=CARTESIAN_POINT('Ctrl Pts',(183.567064733937,-1.42373941229825,
123.952315184543));
#216563=CARTESIAN_POINT('Ctrl Pts',(183.845512357749,4.99525395369783,125.90283040054));
#216564=CARTESIAN_POINT('Ctrl Pts',(184.123959981563,6.82385296796736,132.357612432922));
#216565=CARTESIAN_POINT('Ctrl Pts',(184.402407605375,2.38166446842562,137.385031927559));
#216566=CARTESIAN_POINT('Ctrl Pts',(184.673295880787,-4.06914253102304,
136.392824298985));
#216567=CARTESIAN_POINT('Ctrl Pts',(184.851368281593,-5.91419482002716,
132.605670887374));
#216568=CARTESIAN_POINT('Ctrl Pts',(184.936624807795,-5.92486718842363,
130.801517542038));
#216569=CARTESIAN_POINT('',(186.686624807795,-5.91810304431807,130.809680029163));
#216570=CARTESIAN_POINT('Ctrl Pts',(184.936624807795,-5.92486718842363,
130.801517542038));
#216571=CARTESIAN_POINT('Ctrl Pts',(184.944184156197,-5.92581346379487,
130.641550624367));
#216572=CARTESIAN_POINT('Ctrl Pts',(185.044559379204,-5.84727879099301,
128.518407035367));
#216573=CARTESIAN_POINT('Ctrl Pts',(185.237750476814,-3.29138665363019,
124.628250642296));
#216574=CARTESIAN_POINT('Ctrl Pts',(185.516198100626,3.4170613558443,124.696885507443));
#216575=CARTESIAN_POINT('Ctrl Pts',(185.794645724439,6.98539691202545,130.377991632052));
#216576=CARTESIAN_POINT('Ctrl Pts',(186.073093348252,4.13449396166582,136.450910025061));
#216577=CARTESIAN_POINT('Ctrl Pts',(186.351540972065,-2.5158069582057,137.334925361857));
#216578=CARTESIAN_POINT('Ctrl Pts',(186.55605145858,-5.7022149293107,133.576472626177));
#216579=CARTESIAN_POINT('Ctrl Pts',(186.667746070489,-5.92222955506447,
131.210299569289));
#216580=CARTESIAN_POINT('Ctrl Pts',(186.686624807795,-5.91851213263273,
130.809680396867));
#216581=CARTESIAN_POINT('',(188.436624807759,-5.91674998742092,130.804746434304));
#216582=CARTESIAN_POINT('Ctrl Pts',(186.686624807795,-5.91674760990531,
130.809678810848));
#216583=CARTESIAN_POINT('Ctrl Pts',(186.693927872074,-5.91688686513407,
130.654750624113));
#216584=CARTESIAN_POINT('Ctrl Pts',(186.701230936354,-5.91093684901184,
130.499626658566));
#216585=CARTESIAN_POINT('Ctrl Pts',(186.708534000633,-5.89887823475046,
130.344832452937));
#216586=CARTESIAN_POINT('Ctrl Pts',(186.71583126983,-5.88682918916652,130.190161078655));
#216587=CARTESIAN_POINT('Ctrl Pts',(186.723128539027,-5.86868122137412,
130.035819325382));
#216588=CARTESIAN_POINT('Ctrl Pts',(186.730425808224,-5.84446706708341,
129.882332817401));
#216589=CARTESIAN_POINT('Ctrl Pts',(186.737842908702,-5.81985528279573,
129.726325848082));
#216590=CARTESIAN_POINT('Ctrl Pts',(186.745260009179,-5.78897632400346,
129.57120286325));
#216591=CARTESIAN_POINT('Ctrl Pts',(186.752677109657,-5.75191958714079,
129.417511085149));
#216592=CARTESIAN_POINT('Ctrl Pts',(186.759968840886,-5.71548921030546,
129.266417117715));
#216593=CARTESIAN_POINT('Ctrl Pts',(186.767260572116,-5.67308835349849,
129.116706741788));
#216594=CARTESIAN_POINT('Ctrl Pts',(186.774552303345,-5.62485348468246,
128.968889604895));
#216595=CARTESIAN_POINT('Ctrl Pts',(186.781843715033,-5.57662072963386,
128.821078945703));
#216596=CARTESIAN_POINT('Ctrl Pts',(186.789135126721,-5.52255459037707,
128.675161726577));
#216597=CARTESIAN_POINT('Ctrl Pts',(186.796426538409,-5.46284118724312,
128.531631701602));
#216598=CARTESIAN_POINT('Ctrl Pts',(186.803719166403,-5.40311782310642,
128.388077733878));
#216599=CARTESIAN_POINT('Ctrl Pts',(186.811011794397,-5.33774546886925,
128.246912107963));
#216600=CARTESIAN_POINT('Ctrl Pts',(186.818304422391,-5.26695796755661,
128.108607600227));
#216601=CARTESIAN_POINT('Ctrl Pts',(186.8258154055,-5.19405095418979,127.966161993203));
#216602=CARTESIAN_POINT('Ctrl Pts',(186.833326388608,-5.11539964036747,
127.826751909787));
#216603=CARTESIAN_POINT('Ctrl Pts',(186.840837371716,-5.03130930734334,
127.690864637748));
#216604=CARTESIAN_POINT('Ctrl Pts',(186.84814077682,-4.949542944875,127.558732827339));
#216605=CARTESIAN_POINT('Ctrl Pts',(186.855444181923,-4.86263449198645,
127.429931967507));
#216606=CARTESIAN_POINT('Ctrl Pts',(186.862747587026,-4.77090702822886,
127.30487827149));
#216607=CARTESIAN_POINT('Ctrl Pts',(186.870362359137,-4.6752689357269,127.174493145188));
#216608=CARTESIAN_POINT('Ctrl Pts',(186.877977131248,-4.57439219292684,
127.048182094909));
#216609=CARTESIAN_POINT('Ctrl Pts',(186.885591903359,-4.46868683856503,
126.926375509119));
#216610=CARTESIAN_POINT('Ctrl Pts',(186.89320667547,-4.3629814842032,126.80456892333));
#216611=CARTESIAN_POINT('Ctrl Pts',(186.900821447581,-4.25244789244555,
126.687267089292));
#216612=CARTESIAN_POINT('Ctrl Pts',(186.908436219692,-4.13753558760197,
126.574853574916));
#216613=CARTESIAN_POINT('Ctrl Pts',(186.915859486097,-4.02551323950221,
126.465267174611));
#216614=CARTESIAN_POINT('Ctrl Pts',(186.923282752503,-3.9089647500179,126.359968661986));
#216615=CARTESIAN_POINT('Ctrl Pts',(186.930706018908,-3.78825199071475,
126.259354851085));
#216616=CARTESIAN_POINT('Ctrl Pts',(186.938120511629,-3.66768190386831,
126.158859957352));
#216617=CARTESIAN_POINT('Ctrl Pts',(186.94553500435,-3.54295762806711,126.063038980729));
#216618=CARTESIAN_POINT('Ctrl Pts',(186.952949497071,-3.4144784567078,125.972252647831));
#216619=CARTESIAN_POINT('Ctrl Pts',(186.960356843425,-3.28612311841112,
125.881553818218));
#216620=CARTESIAN_POINT('Ctrl Pts',(186.967764189779,-3.15402039231062,
125.795880185779));
#216621=CARTESIAN_POINT('Ctrl Pts',(186.975171536132,-3.01860320296358,
125.715552774313));
#216622=CARTESIAN_POINT('Ctrl Pts',(186.982573357808,-2.88328701286552,
125.63528527406));
#216623=CARTESIAN_POINT('Ctrl Pts',(186.989975179483,-2.74466160138934,
125.560356244931));
#216624=CARTESIAN_POINT('Ctrl Pts',(186.997377001159,-2.60318938208514,
125.491043800031));
#216625=CARTESIAN_POINT('Ctrl Pts',(187.00477491547,-2.46179184486368,125.421767944631));
#216626=CARTESIAN_POINT('Ctrl Pts',(187.012172829781,-2.3175508271054,125.358102932441));
#216627=CARTESIAN_POINT('Ctrl Pts',(187.019570744093,-2.17095378175324,
125.300281199535));
#216628=CARTESIAN_POINT('Ctrl Pts',(187.026967429005,-2.02438109817091,
125.242469075553));
#216629=CARTESIAN_POINT('Ctrl Pts',(187.034364113917,-1.87545351098578,
125.190498440448));
#216630=CARTESIAN_POINT('Ctrl Pts',(187.041760798829,-1.72467902321808,
125.144553833817));
#216631=CARTESIAN_POINT('Ctrl Pts',(187.049157155765,-1.573911220949,125.098611264417));
#216632=CARTESIAN_POINT('Ctrl Pts',(187.0565535127,-1.42129703801589,125.058694301019));
#216633=CARTESIAN_POINT('Ctrl Pts',(187.063949869636,-1.2673599706079,125.024937699367));
#216634=CARTESIAN_POINT('Ctrl Pts',(187.071347358972,-1.11339933504184,
124.991175929494));
#216635=CARTESIAN_POINT('Ctrl Pts',(187.078744848309,-0.958115776379954,
124.963576479304));
#216636=CARTESIAN_POINT('Ctrl Pts',(187.086142337645,-0.802043172628662,
124.942223011561));
#216637=CARTESIAN_POINT('Ctrl Pts',(187.09354242016,-0.645915857868791,
124.920862058393));
#216638=CARTESIAN_POINT('Ctrl Pts',(187.100942502675,-0.488999316935465,
124.905751497561));
#216639=CARTESIAN_POINT('Ctrl Pts',(187.10834258519,-0.331832590309043,
124.896923127883));
#216640=CARTESIAN_POINT('Ctrl Pts',(187.115750804857,-0.174493042708975,
124.888085050506));
#216641=CARTESIAN_POINT('Ctrl Pts',(187.123159024523,-0.016903132952331,
124.885542980791));
#216642=CARTESIAN_POINT('Ctrl Pts',(187.13056724419,0.140397315335382,124.889276581278));
#216643=CARTESIAN_POINT('Ctrl Pts',(187.137980023492,0.297794579424681,
124.893012479734));
#216644=CARTESIAN_POINT('Ctrl Pts',(187.145392802794,0.454901655364147,
124.903031721345));
#216645=CARTESIAN_POINT('Ctrl Pts',(187.152805582096,0.611184312778971,
124.919262122357));
#216646=CARTESIAN_POINT('Ctrl Pts',(187.160228953124,0.767690274183362,
124.935515714127));
#216647=CARTESIAN_POINT('Ctrl Pts',(187.167652324153,0.923369095910833,
124.957998137041));
#216648=CARTESIAN_POINT('Ctrl Pts',(187.175075695182,1.07769637957054,124.986586036512));
#216649=CARTESIAN_POINT('Ctrl Pts',(187.179011744623,1.15952440839869,125.001744026769));
#216650=CARTESIAN_POINT('Ctrl Pts',(187.182947794064,1.24097270681647,125.01861764673));
#216651=CARTESIAN_POINT('Ctrl Pts',(187.186883843504,1.32196501082129,125.037182878614));
#216652=CARTESIAN_POINT('Ctrl Pts',(187.19430710991,1.47471396849223,125.072196326546));
#216653=CARTESIAN_POINT('Ctrl Pts',(187.201730376315,1.62630189479336,125.113335453442));
#216654=CARTESIAN_POINT('Ctrl Pts',(187.209153642721,1.77619933841254,125.160510294185));
#216655=CARTESIAN_POINT('Ctrl Pts',(187.216568135442,1.92591961570148,125.207629378185));
#216656=CARTESIAN_POINT('Ctrl Pts',(187.223982628163,2.07395303475566,125.260769865369));
#216657=CARTESIAN_POINT('Ctrl Pts',(187.231397120884,2.21978027822349,125.319790800442));
#216658=CARTESIAN_POINT('Ctrl Pts',(187.238804467237,2.36546696790406,125.378754848915));
#216659=CARTESIAN_POINT('Ctrl Pts',(187.246211813591,2.50895137152433,125.443587922699));
#216660=CARTESIAN_POINT('Ctrl Pts',(187.253619159945,2.64972939637269,125.514099311307));
#216661=CARTESIAN_POINT('Ctrl Pts',(187.26102098162,2.79040242365833,125.584558109861));
#216662=CARTESIAN_POINT('Ctrl Pts',(187.268422803296,2.92837275898145,125.660686624124));
#216663=CARTESIAN_POINT('Ctrl Pts',(187.275824624971,3.0631564720913,125.742246139407));
#216664=CARTESIAN_POINT('Ctrl Pts',(187.283222539282,3.19786903392806,125.823762600057));
#216665=CARTESIAN_POINT('Ctrl Pts',(187.290620453594,3.3293980051506,125.910704159221));
#216666=CARTESIAN_POINT('Ctrl Pts',(187.298018367905,3.45728435048477,126.002786346309));
#216667=CARTESIAN_POINT('Ctrl Pts',(187.305415052817,3.58514944342875,126.094853231009));
#216668=CARTESIAN_POINT('Ctrl Pts',(187.31281173773,3.70937280925888,126.192058830229));
#216669=CARTESIAN_POINT('Ctrl Pts',(187.320208422642,3.82952460154685,126.2940754948));
#216670=CARTESIAN_POINT('Ctrl Pts',(187.327604779577,3.94967106617857,126.396087635844));
#216671=CARTESIAN_POINT('Ctrl Pts',(187.335001136513,4.06574603167699,126.502910176461));
#216672=CARTESIAN_POINT('Ctrl Pts',(187.342397493448,4.17735316173905,126.614175523252));
#216673=CARTESIAN_POINT('Ctrl Pts',(187.349794982785,4.28897737913757,126.725457905052));
#216674=CARTESIAN_POINT('Ctrl Pts',(187.357192472121,4.39613213470813,126.841184183831));
#216675=CARTESIAN_POINT('Ctrl Pts',(187.364589961458,4.4984584664945,126.96095041467));
#216676=CARTESIAN_POINT('Ctrl Pts',(187.371990043973,4.6008206686173,127.080758629375));
#216677=CARTESIAN_POINT('Ctrl Pts',(187.379390126488,4.69835083467273,127.204609332144));
#216678=CARTESIAN_POINT('Ctrl Pts',(187.386790209003,4.79073084686722,127.332066200991));
#216679=CARTESIAN_POINT('Ctrl Pts',(187.394198428669,4.88321244038255,127.45966322177));
#216680=CARTESIAN_POINT('Ctrl Pts',(187.401606648336,4.97053235119977,127.590874025252));
#216681=CARTESIAN_POINT('Ctrl Pts',(187.409014868002,5.05241590194538,127.725233449638));
#216682=CARTESIAN_POINT('Ctrl Pts',(187.416427647304,5.13434985065019,127.859675570009));
#216683=CARTESIAN_POINT('Ctrl Pts',(187.423840426606,5.21084059102242,127.997269847324));
#216684=CARTESIAN_POINT('Ctrl Pts',(187.431253205909,5.28166008873117,128.137527801358));
#216685=CARTESIAN_POINT('Ctrl Pts',(187.438676576937,5.35258077665936,128.277986162534));
#216686=CARTESIAN_POINT('Ctrl Pts',(187.446099947966,5.41781388333707,128.421115463055));
#216687=CARTESIAN_POINT('Ctrl Pts',(187.453523318995,5.47717974033229,128.566407835537));
#216688=CARTESIAN_POINT('Ctrl Pts',(187.457459368436,5.50865694217581,128.64344533767));
#216689=CARTESIAN_POINT('Ctrl Pts',(187.461395417877,5.53848548259736,128.721090701616));
#216690=CARTESIAN_POINT('Ctrl Pts',(187.465331467317,5.56664434588085,128.799266782113));
#216691=CARTESIAN_POINT('Ctrl Pts',(187.472754733723,5.61975108322465,128.946704430135));
#216692=CARTESIAN_POINT('Ctrl Pts',(187.480178000128,5.66707654755361,129.096476348691));
#216693=CARTESIAN_POINT('Ctrl Pts',(187.487601266534,5.70841024769987,129.248088467055));
#216694=CARTESIAN_POINT('Ctrl Pts',(187.495015759255,5.74969509484514,129.399521392486));
#216695=CARTESIAN_POINT('Ctrl Pts',(187.502430251976,5.78500217687627,129.552789831813));
#216696=CARTESIAN_POINT('Ctrl Pts',(187.509844744697,5.81416937976279,129.707380678858));
#216697=CARTESIAN_POINT('Ctrl Pts',(187.517252091051,5.84330847020106,129.861822525424));
#216698=CARTESIAN_POINT('Ctrl Pts',(187.524659437404,5.86631939401667,130.017583877895));
#216699=CARTESIAN_POINT('Ctrl Pts',(187.532066783758,5.88309012691937,130.17413754512));
#216700=CARTESIAN_POINT('Ctrl Pts',(187.539468605433,5.89984835157674,130.330574448713));
#216701=CARTESIAN_POINT('Ctrl Pts',(187.546870427109,5.91037561281063,130.487802120845));
#216702=CARTESIAN_POINT('Ctrl Pts',(187.554272248784,5.91461117192879,130.64528438617));
#216703=CARTESIAN_POINT('Ctrl Pts',(187.561670163096,5.91884449512825,130.802683517833));
#216704=CARTESIAN_POINT('Ctrl Pts',(187.569068077407,5.91679272080989,130.960336602811));
#216705=CARTESIAN_POINT('Ctrl Pts',(187.576465991718,5.90844706236015,131.117703678424));
#216706=CARTESIAN_POINT('Ctrl Pts',(187.583862676631,5.90010279080743,131.275044602484));
#216707=CARTESIAN_POINT('Ctrl Pts',(187.591259361543,5.88546673073356,131.432099239102));
#216708=CARTESIAN_POINT('Ctrl Pts',(187.598656046455,5.86458220017064,131.588328843926));
#216709=CARTESIAN_POINT('Ctrl Pts',(187.60605240339,5.84369859564966,131.744551521365));
#216710=CARTESIAN_POINT('Ctrl Pts',(187.613448760326,5.81656712099775,131.899948869742));
#216711=CARTESIAN_POINT('Ctrl Pts',(187.620845117261,5.78328281349836,132.053988746889));
#216712=CARTESIAN_POINT('Ctrl Pts',(187.628242606598,5.74999341008647,132.208052207934));
#216713=CARTESIAN_POINT('Ctrl Pts',(187.635640095934,5.71054937699733,132.360757419028));
#216714=CARTESIAN_POINT('Ctrl Pts',(187.643037585271,5.66509653682644,132.511584033214));
#216715=CARTESIAN_POINT('Ctrl Pts',(187.650437667786,5.61962776323287,132.662463519436));
#216716=CARTESIAN_POINT('Ctrl Pts',(187.657837750301,5.56814609641887,132.811462740405));
#216717=CARTESIAN_POINT('Ctrl Pts',(187.665237832816,5.51084667598898,132.958078211923));
#216718=CARTESIAN_POINT('Ctrl Pts',(187.672646052482,5.45348424895594,133.104854902223));
#216719=CARTESIAN_POINT('Ctrl Pts',(187.680054272149,5.39029142860743,133.249242260506));
#216720=CARTESIAN_POINT('Ctrl Pts',(187.687462491815,5.3215110989095,133.390757761603));
#216721=CARTESIAN_POINT('Ctrl Pts',(187.694875271117,5.2526884360661,133.53236036313));
#216722=CARTESIAN_POINT('Ctrl Pts',(187.702288050419,5.17827158724947,133.671087257152));
#216723=CARTESIAN_POINT('Ctrl Pts',(187.709700829722,5.09854826658263,133.806482556433));
#216724=CARTESIAN_POINT('Ctrl Pts',(187.71712420075,5.01871103349667,133.942071314867));
#216725=CARTESIAN_POINT('Ctrl Pts',(187.724547571779,4.93355238690208,134.074318658072));
#216726=CARTESIAN_POINT('Ctrl Pts',(187.731970942808,4.84340249483737,134.20279891118));
#216727=CARTESIAN_POINT('Ctrl Pts',(187.735906992249,4.79560285894802,134.270922224219));
#216728=CARTESIAN_POINT('Ctrl Pts',(187.739843041689,4.74640066993037,134.337987035869));
#216729=CARTESIAN_POINT('Ctrl Pts',(187.74377909113,4.69584947277127,134.403933966114));
#216730=CARTESIAN_POINT('Ctrl Pts',(187.751202357536,4.6005114925774,134.528307818423));
#216731=CARTESIAN_POINT('Ctrl Pts',(187.758625623941,4.50008470519337,134.649079452252));
#216732=CARTESIAN_POINT('Ctrl Pts',(187.766048890346,4.39487101069584,134.765804718124));
#216733=CARTESIAN_POINT('Ctrl Pts',(187.773463383067,4.28978167004782,134.882392024425));
#216734=CARTESIAN_POINT('Ctrl Pts',(187.780877875788,4.17991693151612,134.994942207732));
#216735=CARTESIAN_POINT('Ctrl Pts',(187.788292368509,4.06562085926568,135.103041530498));
#216736=CARTESIAN_POINT('Ctrl Pts',(187.795699714863,3.95143494987295,135.211036663066));
#216737=CARTESIAN_POINT('Ctrl Pts',(187.803107061217,3.83282647904385,135.314589220668));
#216738=CARTESIAN_POINT('Ctrl Pts',(187.810514407571,3.71017843575953,135.413319994402));
#216739=CARTESIAN_POINT('Ctrl Pts',(187.817916229246,3.58762186801298,135.511977131));
#216740=CARTESIAN_POINT('Ctrl Pts',(187.825318050921,3.4610320163687,135.60581941131));
#216741=CARTESIAN_POINT('Ctrl Pts',(187.832719872597,3.33082714958386,135.69450591828));
#216742=CARTESIAN_POINT('Ctrl Pts',(187.840117786908,3.20069101693379,135.783145608334));
#216743=CARTESIAN_POINT('Ctrl Pts',(187.847515701219,3.06694397743706,135.866634735812));
#216744=CARTESIAN_POINT('Ctrl Pts',(187.854913615531,2.93003556760929,135.944674045271));
#216745=CARTESIAN_POINT('Ctrl Pts',(187.862310300443,2.79314990947657,136.022700386012));
#216746=CARTESIAN_POINT('Ctrl Pts',(187.869706985355,2.65310424769539,136.095278521522));
#216747=CARTESIAN_POINT('Ctrl Pts',(187.877103670267,2.51037525760295,136.162153692006));
#216748=CARTESIAN_POINT('Ctrl Pts',(187.884500027203,2.36765259626331,136.229025897175));
#216749=CARTESIAN_POINT('Ctrl Pts',(187.891896384138,2.22224718122004,136.290195481735));
#216750=CARTESIAN_POINT('Ctrl Pts',(187.899292741074,2.0746580887224,136.345454767407));
#216751=CARTESIAN_POINT('Ctrl Pts',(187.90669023041,1.92704639995784,136.400722513416));
#216752=CARTESIAN_POINT('Ctrl Pts',(187.914087719747,1.77725071766979,136.450078027893));
#216753=CARTESIAN_POINT('Ctrl Pts',(187.921485209083,1.62578764516406,136.493362735278));
#216754=CARTESIAN_POINT('Ctrl Pts',(187.928885291598,1.47427147751353,136.53666261605));
#216755=CARTESIAN_POINT('Ctrl Pts',(187.936285374113,1.32108711461301,136.573887350165));
#216756=CARTESIAN_POINT('Ctrl Pts',(187.943685456628,1.16676362970169,136.60492896859));
#216757=CARTESIAN_POINT('Ctrl Pts',(187.951093676295,1.01227045025355,136.636004720467));
#216758=CARTESIAN_POINT('Ctrl Pts',(187.958501895961,0.856636013498965,
136.660883705003));
#216759=CARTESIAN_POINT('Ctrl Pts',(187.965910115627,0.700397566244245,
136.679509450719));
#216760=CARTESIAN_POINT('Ctrl Pts',(187.973322894929,0.544062956832329,
136.698146660271));
#216761=CARTESIAN_POINT('Ctrl Pts',(187.980735674231,0.387123967424787,
136.710522932578));
#216762=CARTESIAN_POINT('Ctrl Pts',(187.988148453534,0.23011966537511,136.716633911495));
#216763=CARTESIAN_POINT('Ctrl Pts',(187.995571824562,0.072891028215697,
136.722753622065));
#216764=CARTESIAN_POINT('Ctrl Pts',(188.002995195591,-0.0844027356615752,
136.72259016019));
#216765=CARTESIAN_POINT('Ctrl Pts',(188.01041856662,-0.241225030045429,
136.716191217928));
#216766=CARTESIAN_POINT('Ctrl Pts',(188.014354616061,-0.324375973428068,
136.7127983452));
#216767=CARTESIAN_POINT('Ctrl Pts',(188.018290665501,-0.407394483839031,
136.707653318947));
#216768=CARTESIAN_POINT('Ctrl Pts',(188.022226714942,-0.490201660815617,
136.700769091733));
#216769=CARTESIAN_POINT('Ctrl Pts',(188.029649981348,-0.646373412268205,
136.687785654058));
#216770=CARTESIAN_POINT('Ctrl Pts',(188.037073247753,-0.80226513988054,
136.668573771693));
#216771=CARTESIAN_POINT('Ctrl Pts',(188.044496514159,-0.957339983753277,
136.643147368083));
#216772=CARTESIAN_POINT('Ctrl Pts',(188.051911006879,-1.11223154203839,
136.61775101637));
#216773=CARTESIAN_POINT('Ctrl Pts',(188.0593254996,-1.26630777361279,136.58615482358));
#216774=CARTESIAN_POINT('Ctrl Pts',(188.066739992321,-1.41903461427524,
136.548424625391));
#216775=CARTESIAN_POINT('Ctrl Pts',(188.074147338675,-1.57161425105952,
136.510730792987));
#216776=CARTESIAN_POINT('Ctrl Pts',(188.081554685029,-1.72284672618799,
136.466914814107));
#216777=CARTESIAN_POINT('Ctrl Pts',(188.088962031383,-1.87220598557174,
136.417093936555));
#216778=CARTESIAN_POINT('Ctrl Pts',(188.096363853058,-2.02145384718316,
136.367310217293));
#216779=CARTESIAN_POINT('Ctrl Pts',(188.103765674734,-2.16883092230147,
136.311530634628));
#216780=CARTESIAN_POINT('Ctrl Pts',(188.111167496409,-2.31382430327432,
136.249922815914));
#216781=CARTESIAN_POINT('Ctrl Pts',(188.11856541072,-2.45874114337115,136.188347519488));
#216782=CARTESIAN_POINT('Ctrl Pts',(188.125963325032,-2.60127645265397,
136.120950259984));
#216783=CARTESIAN_POINT('Ctrl Pts',(188.133361239343,-2.7409354735747,136.047947490328));
#216784=CARTESIAN_POINT('Ctrl Pts',(188.140757924255,-2.88057128569987,
135.974956852407));
#216785=CARTESIAN_POINT('Ctrl Pts',(188.148154609167,-3.01733142762264,
135.896362725914));
#216786=CARTESIAN_POINT('Ctrl Pts',(188.15555129408,-3.1507439080487,135.812428447418));
#216787=CARTESIAN_POINT('Ctrl Pts',(188.162947651015,-3.28415047282601,
135.728497890655));
#216788=CARTESIAN_POINT('Ctrl Pts',(188.170344007951,-3.41420935528581,
135.639227851488));
#216789=CARTESIAN_POINT('Ctrl Pts',(188.177740364886,-3.54047606690486,
135.544925961718));
#216790=CARTESIAN_POINT('Ctrl Pts',(188.185137854223,-3.66676211027926,
135.450609634088));
#216791=CARTESIAN_POINT('Ctrl Pts',(188.192535343559,-3.78925452766934,
135.351260145295));
#216792=CARTESIAN_POINT('Ctrl Pts',(188.199932832896,-3.90754066825958,
135.247226414368));
#216793=CARTESIAN_POINT('Ctrl Pts',(188.207332915411,-4.02586827387267,
135.143156214579));
#216794=CARTESIAN_POINT('Ctrl Pts',(188.214732997926,-4.13998638682651,
135.034398749718));
#216795=CARTESIAN_POINT('Ctrl Pts',(188.222133080441,-4.24951819270741,
134.921340784187));
#216796=CARTESIAN_POINT('Ctrl Pts',(188.229541300107,-4.35917044006939,
134.808158499799));
#216797=CARTESIAN_POINT('Ctrl Pts',(188.236949519774,-4.4642260490177,134.690666539206));
#216798=CARTESIAN_POINT('Ctrl Pts',(188.24435773944,-4.56434711347478,134.569286379147));
#216799=CARTESIAN_POINT('Ctrl Pts',(188.251770518742,-4.66452980077634,
134.447831511624));
#216800=CARTESIAN_POINT('Ctrl Pts',(188.259183298044,-4.75977166640558,
134.322483972582));
#216801=CARTESIAN_POINT('Ctrl Pts',(188.266596077347,-4.84977766634151,
134.193694940048));
#216802=CARTESIAN_POINT('Ctrl Pts',(188.274019448375,-4.93991227107106,
134.064721887705));
#216803=CARTESIAN_POINT('Ctrl Pts',(188.281442819404,-5.02479586745561,
133.932297834228));
#216804=CARTESIAN_POINT('Ctrl Pts',(188.288866190433,-5.10417853681512,
133.796900011929));
#216805=CARTESIAN_POINT('Ctrl Pts',(188.292802239874,-5.14626913287155,
133.725108837719));
#216806=CARTESIAN_POINT('Ctrl Pts',(188.296738289315,-5.18681400928749,
133.652482001339));
#216807=CARTESIAN_POINT('Ctrl Pts',(188.300674338755,-5.22578141579513,
133.579092885161));
#216808=CARTESIAN_POINT('Ctrl Pts',(188.308522635262,-5.30348058216972,
133.432758457005));
#216809=CARTESIAN_POINT('Ctrl Pts',(188.316370931769,-5.37511838685106,
133.282990724991));
#216810=CARTESIAN_POINT('Ctrl Pts',(188.324219228275,-5.44039662476336,
133.130304539453));
#216811=CARTESIAN_POINT('Ctrl Pts',(188.332053990155,-5.50556228836188,
132.977881665902));
#216812=CARTESIAN_POINT('Ctrl Pts',(188.339888752035,-5.56439012663925,
132.822550655319));
#216813=CARTESIAN_POINT('Ctrl Pts',(188.347723513915,-5.61662765213832,
132.664850977588));
#216814=CARTESIAN_POINT('Ctrl Pts',(188.355539641514,-5.6687409353559,132.507526374433));
#216815=CARTESIAN_POINT('Ctrl Pts',(188.363355769114,-5.71429507358988,
132.347844634376));
#216816=CARTESIAN_POINT('Ctrl Pts',(188.371171896713,-5.75308575484795,
132.1863645466));
#216817=CARTESIAN_POINT('Ctrl Pts',(188.378976980979,-5.7918216291147,132.025112612533));
#216818=CARTESIAN_POINT('Ctrl Pts',(188.386782065244,-5.82381301965768,
131.862067694374));
#216819=CARTESIAN_POINT('Ctrl Pts',(188.39458714951,-5.8489048080885,131.697805136503));
#216820=CARTESIAN_POINT('Ctrl Pts',(188.402376866656,-5.87394719429565,
131.533865988645));
#216821=CARTESIAN_POINT('Ctrl Pts',(188.410166583802,-5.89211702687552,
131.368714288067));
#216822=CARTESIAN_POINT('Ctrl Pts',(188.417956300948,-5.90330990566078,
131.20293648265));
#216823=CARTESIAN_POINT('Ctrl Pts',(188.424179136552,-5.91225136570458,
131.070504455847));
#216824=CARTESIAN_POINT('Ctrl Pts',(188.430401972156,-5.91674131959235,
130.937673208914));
#216825=CARTESIAN_POINT('Ctrl Pts',(188.436624807759,-5.91674998742092,
130.804746434304));
#216826=CARTESIAN_POINT('',(190.186624807795,-5.9167474892903,130.798909885783));
#216827=CARTESIAN_POINT('Ctrl Pts',(188.436624807795,-5.91674998742097,
130.80474643354));
#216828=CARTESIAN_POINT('Ctrl Pts',(188.444336312247,-5.91676072880488,
130.640020016287));
#216829=CARTESIAN_POINT('Ctrl Pts',(188.452047816698,-5.9098880006331,130.475412038668));
#216830=CARTESIAN_POINT('Ctrl Pts',(188.45975932115,-5.89618734660479,130.311506342716));
#216831=CARTESIAN_POINT('Ctrl Pts',(188.467479281045,-5.88247167020258,
130.147420928874));
#216832=CARTESIAN_POINT('Ctrl Pts',(188.47519924094,-5.86191315565751,129.984039656638));
#216833=CARTESIAN_POINT('Ctrl Pts',(188.482919200835,-5.83461887000143,
129.821938506494));
#216834=CARTESIAN_POINT('Ctrl Pts',(188.490936097646,-5.80627474974523,
129.65360237375));
#216835=CARTESIAN_POINT('Ctrl Pts',(188.498952994457,-5.77066650315088,
129.486647185334));
#216836=CARTESIAN_POINT('Ctrl Pts',(188.506969891268,-5.72797103557548,
129.321701392353));
#216837=CARTESIAN_POINT('Ctrl Pts',(188.514715160958,-5.6867221685032,129.162344264416));
#216838=CARTESIAN_POINT('Ctrl Pts',(188.522460430647,-5.63885863849107,
129.004862872487));
#216839=CARTESIAN_POINT('Ctrl Pts',(188.530205700337,-5.5845895056426,128.849804244379));
#216840=CARTESIAN_POINT('Ctrl Pts',(188.538358410709,-5.52746553966337,
128.686588741718));
#216841=CARTESIAN_POINT('Ctrl Pts',(188.546511121081,-5.46324405110737,
128.526058178221));
#216842=CARTESIAN_POINT('Ctrl Pts',(188.554663831453,-5.39222426567471,
128.368822067026));
#216843=CARTESIAN_POINT('Ctrl Pts',(188.562816541824,-5.32120448024206,
128.21158595583));
#216844=CARTESIAN_POINT('Ctrl Pts',(188.570969252196,-5.24338665044448,
128.057644630733));
#216845=CARTESIAN_POINT('Ctrl Pts',(188.579121962568,-5.15912334327355,
127.907573277876));
#216846=CARTESIAN_POINT('Ctrl Pts',(188.586545228974,-5.08239929092767,
127.770929194955));
#216847=CARTESIAN_POINT('Ctrl Pts',(188.593968495379,-5.00012675873199,
127.637128755464));
#216848=CARTESIAN_POINT('Ctrl Pts',(188.601391761784,-4.91254156507233,
127.506654455104));
#216849=CARTESIAN_POINT('Ctrl Pts',(188.608806254505,-4.82505988983811,
127.376334364533));
#216850=CARTESIAN_POINT('Ctrl Pts',(188.616220747226,-4.73227825779838,
127.249332894892));
#216851=CARTESIAN_POINT('Ctrl Pts',(188.623635239947,-4.6344785403192,127.126108420962));
#216852=CARTESIAN_POINT('Ctrl Pts',(188.631042586301,-4.53677308588965,
127.00300271542));
#216853=CARTESIAN_POINT('Ctrl Pts',(188.638449932655,-4.43405940528752,
126.883667048682));
#216854=CARTESIAN_POINT('Ctrl Pts',(188.645857279009,-4.32666280054533,
126.76853113989));
#216855=CARTESIAN_POINT('Ctrl Pts',(188.653259100684,-4.21934629624284,
126.653481103803));
#216856=CARTESIAN_POINT('Ctrl Pts',(188.66066092236,-4.10735407577181,126.542624860554));
#216857=CARTESIAN_POINT('Ctrl Pts',(188.668062744035,-3.99105179769123,
126.436359231274));
#216858=CARTESIAN_POINT('Ctrl Pts',(188.675460658346,-3.87481091467824,
126.330149698793));
#216859=CARTESIAN_POINT('Ctrl Pts',(188.682858572658,-3.75426478020397,
126.22852620523));
#216860=CARTESIAN_POINT('Ctrl Pts',(188.690256486969,-3.62981591611858,
126.131848768722));
#216861=CARTESIAN_POINT('Ctrl Pts',(188.697653171881,-3.50538773317637,
126.035187398249));
#216862=CARTESIAN_POINT('Ctrl Pts',(188.705049856793,-3.3770584023365,125.943470682302));
#216863=CARTESIAN_POINT('Ctrl Pts',(188.712446541706,-3.24526362374814,
125.857018444755));
#216864=CARTESIAN_POINT('Ctrl Pts',(188.719842898641,-3.11347468907845,
125.77057004059));
#216865=CARTESIAN_POINT('Ctrl Pts',(188.727239255577,-2.97822092432744,
125.689385855431));
#216866=CARTESIAN_POINT('Ctrl Pts',(188.734635612512,-2.83996688492409,
125.613742286863));
#216867=CARTESIAN_POINT('Ctrl Pts',(188.742033101849,-2.70169167847449,
125.53808713707));
#216868=CARTESIAN_POINT('Ctrl Pts',(188.749430591185,-2.56041561025224,
125.467974472102));
#216869=CARTESIAN_POINT('Ctrl Pts',(188.756828080522,-2.41662755324927,
125.403634570878));
#216870=CARTESIAN_POINT('Ctrl Pts',(188.764228163037,-2.27278909156605,
125.339272115401));
#216871=CARTESIAN_POINT('Ctrl Pts',(188.771628245552,-2.1264372284147,125.280686605083));
#216872=CARTESIAN_POINT('Ctrl Pts',(188.779028328067,-1.97808036179923,
125.228059993966));
#216873=CARTESIAN_POINT('Ctrl Pts',(188.786436547733,-1.82956036155703,
125.175375514479));
#216874=CARTESIAN_POINT('Ctrl Pts',(188.7938447674,-1.67903130693944,125.128663144689));
#216875=CARTESIAN_POINT('Ctrl Pts',(188.801252987066,-1.52701699451342,
125.088055022082));
#216876=CARTESIAN_POINT('Ctrl Pts',(188.808665766368,-1.37490911981405,
125.047421905852));
#216877=CARTESIAN_POINT('Ctrl Pts',(188.81607854567,-1.22131452911263,125.012900604892));
#216878=CARTESIAN_POINT('Ctrl Pts',(188.823491324972,-1.06676621647483,
124.984571927082));
#216879=CARTESIAN_POINT('Ctrl Pts',(188.830914696001,-0.911997077960795,
124.956202771929));
#216880=CARTESIAN_POINT('Ctrl Pts',(188.83833806703,-0.75627186444372,124.934043964435));
#216881=CARTESIAN_POINT('Ctrl Pts',(188.845761438059,-0.600128509702636,
124.918124440318));
#216882=CARTESIAN_POINT('Ctrl Pts',(188.8496974875,-0.517337556408728,124.909683526647));
#216883=CARTESIAN_POINT('Ctrl Pts',(188.853633536941,-0.434429058316661,
124.90299582822));
#216884=CARTESIAN_POINT('Ctrl Pts',(188.857569586381,-0.3514829554707,124.898059719837));
#216885=CARTESIAN_POINT('Ctrl Pts',(188.864992852787,-0.195049194165717,
124.888750373478));
#216886=CARTESIAN_POINT('Ctrl Pts',(188.872416119192,-0.0380087817261698,
124.885646179091));
#216887=CARTESIAN_POINT('Ctrl Pts',(188.879839385598,0.1191048789509,124.888809536702));
#216888=CARTESIAN_POINT('Ctrl Pts',(188.887253878319,0.276032844328527,
124.891969155487));
#216889=CARTESIAN_POINT('Ctrl Pts',(188.89466837104,0.433033516041292,124.90138157371));
#216890=CARTESIAN_POINT('Ctrl Pts',(188.902082863761,0.589568892045253,
124.917057407774));
#216891=CARTESIAN_POINT('Ctrl Pts',(188.909490210115,0.745953393360701,
124.932718132878));
#216892=CARTESIAN_POINT('Ctrl Pts',(188.916897556468,0.901873122835364,
124.954630218564));
#216893=CARTESIAN_POINT('Ctrl Pts',(188.924304902822,1.05679071189202,124.98275225271));
#216894=CARTESIAN_POINT('Ctrl Pts',(188.931706724498,1.21159275756575,125.010853312383));
#216895=CARTESIAN_POINT('Ctrl Pts',(188.939108546173,1.36539378534926,125.045155031959));
#216896=CARTESIAN_POINT('Ctrl Pts',(188.946510367848,1.51766229100495,125.085564264052));
#216897=CARTESIAN_POINT('Ctrl Pts',(188.95390828216,1.66985041530155,125.125952164426));
#216898=CARTESIAN_POINT('Ctrl Pts',(188.961306196471,1.8205072687502,125.17244106084));
#216899=CARTESIAN_POINT('Ctrl Pts',(188.968704110782,1.96911238500255,125.22488689886));
#216900=CARTESIAN_POINT('Ctrl Pts',(188.976100795695,2.11769280578066,125.277324021333));
#216901=CARTESIAN_POINT('Ctrl Pts',(188.983497480607,2.26422181439622,125.33571599657));
#216902=CARTESIAN_POINT('Ctrl Pts',(188.990894165519,2.40819482739287,125.39986913031));
#216903=CARTESIAN_POINT('Ctrl Pts',(188.998290522454,2.55216145647515,125.464019419434));
#216904=CARTESIAN_POINT('Ctrl Pts',(189.00568687939,2.69357197430951,125.533930207192));
#216905=CARTESIAN_POINT('Ctrl Pts',(189.013083236325,2.83194273622357,125.609360049592));
#216906=CARTESIAN_POINT('Ctrl Pts',(189.020480725662,2.97033468305507,125.684801440493));
#216907=CARTESIAN_POINT('Ctrl Pts',(189.027878214998,3.10568561952156,125.765763389823));
#216908=CARTESIAN_POINT('Ctrl Pts',(189.035275704335,3.23753755765109,125.851959066268));
#216909=CARTESIAN_POINT('Ctrl Pts',(189.04267578685,3.36943571627262,125.938184958474));
#216910=CARTESIAN_POINT('Ctrl Pts',(189.050075869365,3.49783212220785,126.029648026486));
#216911=CARTESIAN_POINT('Ctrl Pts',(189.05747595188,3.62229889082746,126.126018891269));
#216912=CARTESIAN_POINT('Ctrl Pts',(189.064884171547,3.74690252345494,126.222495725726));
#216913=CARTESIAN_POINT('Ctrl Pts',(189.072292391213,3.86756759402008,126.323890905695));
#216914=CARTESIAN_POINT('Ctrl Pts',(189.079700610879,3.98389980667395,126.429835169831));
#216915=CARTESIAN_POINT('Ctrl Pts',(189.087113390182,4.10030361986379,126.535844640893));
#216916=CARTESIAN_POINT('Ctrl Pts',(189.094526169484,4.21236899608596,126.646408513676));
#216917=CARTESIAN_POINT('Ctrl Pts',(189.101938948786,4.31973985307035,126.761122043812));
#216918=CARTESIAN_POINT('Ctrl Pts',(189.109362319814,4.42726412657015,126.875999482018));
#216919=CARTESIAN_POINT('Ctrl Pts',(189.116785690843,4.53008024059027,126.995038137808));
#216920=CARTESIAN_POINT('Ctrl Pts',(189.124209061872,4.627873084345,127.11780107272));
#216921=CARTESIAN_POINT('Ctrl Pts',(189.128145111313,4.6797251966109,127.182892926467));
#216922=CARTESIAN_POINT('Ctrl Pts',(189.132081160754,4.73016581507376,127.249031329645));
#216923=CARTESIAN_POINT('Ctrl Pts',(189.136017210194,4.77915309751256,127.316148147971));
#216924=CARTESIAN_POINT('Ctrl Pts',(189.1434404766,4.87154158335144,127.442728372691));
#216925=CARTESIAN_POINT('Ctrl Pts',(189.150863743005,4.95903740885353,127.573173026402));
#216926=CARTESIAN_POINT('Ctrl Pts',(189.158287009411,5.04129975781475,127.707067070878));
#216927=CARTESIAN_POINT('Ctrl Pts',(189.165701502132,5.12346487951111,127.840802863713));
#216928=CARTESIAN_POINT('Ctrl Pts',(189.173115994853,5.20040864350211,127.977979617276));
#216929=CARTESIAN_POINT('Ctrl Pts',(189.180530487574,5.27183131466145,128.118150433635));
#216930=CARTESIAN_POINT('Ctrl Pts',(189.187937833927,5.34318514596105,128.258186148084));
#216931=CARTESIAN_POINT('Ctrl Pts',(189.195345180281,5.40902831002284,128.401209849912));
#216932=CARTESIAN_POINT('Ctrl Pts',(189.202752526635,5.46910518719545,128.546747051454));
#216933=CARTESIAN_POINT('Ctrl Pts',(189.21015434831,5.52913725676648,128.692175705861));
#216934=CARTESIAN_POINT('Ctrl Pts',(189.217556169986,5.58341146092722,128.840113783703));
#216935=CARTESIAN_POINT('Ctrl Pts',(189.224957991661,5.6317188761904,128.990063766976));
#216936=CARTESIAN_POINT('Ctrl Pts',(189.232355905972,5.68000079034474,129.139934592819));
#216937=CARTESIAN_POINT('Ctrl Pts',(189.239753820284,5.72232207444452,129.291814854514));
#216938=CARTESIAN_POINT('Ctrl Pts',(189.247151734595,5.75852260079111,129.445188804042));
#216939=CARTESIAN_POINT('Ctrl Pts',(189.254548419507,5.79471711126733,129.598537265604));
#216940=CARTESIAN_POINT('Ctrl Pts',(189.26194510442,5.82479279708112,129.753378559388));
#216941=CARTESIAN_POINT('Ctrl Pts',(189.269341789332,5.84863987901503,129.909183468564));
#216942=CARTESIAN_POINT('Ctrl Pts',(189.276738146267,5.8724859035443,130.064981469187));
#216943=CARTESIAN_POINT('Ctrl Pts',(189.284134503203,5.89010381686027,130.221742631245));
#216944=CARTESIAN_POINT('Ctrl Pts',(189.291530860138,5.90143533087373,130.3789295444));
#216945=CARTESIAN_POINT('Ctrl Pts',(189.298928349475,5.91276857977092,130.536140523273));
#216946=CARTESIAN_POINT('Ctrl Pts',(189.306325838811,5.9178134861293,130.693777010678));
#216947=CARTESIAN_POINT('Ctrl Pts',(189.313723328148,5.91656381556915,130.851298649032));
#216948=CARTESIAN_POINT('Ctrl Pts',(189.321123410663,5.91531370693891,131.008875506353));
#216949=CARTESIAN_POINT('Ctrl Pts',(189.328523493178,5.90776463111646,131.166337061412));
#216950=CARTESIAN_POINT('Ctrl Pts',(189.335923575693,5.89396242191814,131.323145285339));
#216951=CARTESIAN_POINT('Ctrl Pts',(189.343331795359,5.88014503577195,131.480125936029));
#216952=CARTESIAN_POINT('Ctrl Pts',(189.350740015026,5.86006081725151,131.636451448796));
#216953=CARTESIAN_POINT('Ctrl Pts',(189.358148234692,5.83380730984865,131.791590496599));
#216954=CARTESIAN_POINT('Ctrl Pts',(189.365561013994,5.80753764385015,131.946825029897));
#216955=CARTESIAN_POINT('Ctrl Pts',(189.372973793296,5.77509119954317,132.100871278681));
#216956=CARTESIAN_POINT('Ctrl Pts',(189.380386572599,5.7366160286638,132.253210886634));
#216957=CARTESIAN_POINT('Ctrl Pts',(189.387809943627,5.69808588265588,132.405768164563));
#216958=CARTESIAN_POINT('Ctrl Pts',(189.395233314656,5.65350991124101,132.556613574327));
#216959=CARTESIAN_POINT('Ctrl Pts',(189.402656685685,5.60308539804483,132.705245828387));
#216960=CARTESIAN_POINT('Ctrl Pts',(189.406592735126,5.57634911122828,132.784054215872));
#216961=CARTESIAN_POINT('Ctrl Pts',(189.410528784567,5.54796938585717,132.862240759177));
#216962=CARTESIAN_POINT('Ctrl Pts',(189.414464834007,5.51798092849068,132.93973342701));
#216963=CARTESIAN_POINT('Ctrl Pts',(189.421888100413,5.46142363380593,133.085882180079));
#216964=CARTESIAN_POINT('Ctrl Pts',(189.429311366818,5.39897048314281,133.230003417703));
#216965=CARTESIAN_POINT('Ctrl Pts',(189.436734633224,5.33078644043194,133.371586063258));
#216966=CARTESIAN_POINT('Ctrl Pts',(189.444149125945,5.26268298559709,133.513001369884));
#216967=CARTESIAN_POINT('Ctrl Pts',(189.451563618666,5.18886228167012,133.651883723719));
#216968=CARTESIAN_POINT('Ctrl Pts',(189.458978111387,5.10953830238054,133.787739389865));
#216969=CARTESIAN_POINT('Ctrl Pts',(189.466385457741,5.03029077852894,133.923464113205));
#216970=CARTESIAN_POINT('Ctrl Pts',(189.473792804094,4.94555072602297,134.056167636292));
#216971=CARTESIAN_POINT('Ctrl Pts',(189.481200150448,4.85557917610903,134.1853784269));
#216972=CARTESIAN_POINT('Ctrl Pts',(189.488601972123,4.76567473037149,134.314492847226));
#216973=CARTESIAN_POINT('Ctrl Pts',(189.496003793799,4.67054676872829,134.440119416974));
#216974=CARTESIAN_POINT('Ctrl Pts',(189.503405615474,4.57050093892078,134.561813442263));
#216975=CARTESIAN_POINT('Ctrl Pts',(189.510803529786,4.470507922528,134.683443226223));
#216976=CARTESIAN_POINT('Ctrl Pts',(189.518201444097,4.36560244470111,134.801144312466));
#216977=CARTESIAN_POINT('Ctrl Pts',(189.525599358408,4.25613186592361,134.914503206622));
#216978=CARTESIAN_POINT('Ctrl Pts',(189.53299604332,4.1466794791702,135.027843262585));
#216979=CARTESIAN_POINT('Ctrl Pts',(189.540392728233,4.03266375619807,135.136842290347));
#216980=CARTESIAN_POINT('Ctrl Pts',(189.547789413145,3.9144706037665,135.241121874919));
#216981=CARTESIAN_POINT('Ctrl Pts',(189.55518577008,3.79628269214324,135.345396835624));
#216982=CARTESIAN_POINT('Ctrl Pts',(189.562582127016,3.67391799928616,135.444952522259));
#216983=CARTESIAN_POINT('Ctrl Pts',(189.569978483951,3.5477971575957,135.539449411987));
#216984=CARTESIAN_POINT('Ctrl Pts',(189.577375973288,3.42165700648274,135.633960769431));
#216985=CARTESIAN_POINT('Ctrl Pts',(189.584773462624,3.2917598602477,135.723411563957));
#216986=CARTESIAN_POINT('Ctrl Pts',(189.592170951961,3.15855696719353,135.807504473932));
#216987=CARTESIAN_POINT('Ctrl Pts',(189.599571034476,3.02530738007121,135.891626862547));
#216988=CARTESIAN_POINT('Ctrl Pts',(189.606971116991,2.88875005437881,135.970387427978));
#216989=CARTESIAN_POINT('Ctrl Pts',(189.614371199506,2.74936242334025,136.043533913767));
#216990=CARTESIAN_POINT('Ctrl Pts',(189.621779419172,2.6098215212719,136.116760831637));
#216991=CARTESIAN_POINT('Ctrl Pts',(189.629187638839,2.46744442931756,136.184361167894));
#216992=CARTESIAN_POINT('Ctrl Pts',(189.636595858505,2.3227308926061,136.246129793398));
#216993=CARTESIAN_POINT('Ctrl Pts',(189.644008637807,2.17792828712777,136.307936436459));
#216994=CARTESIAN_POINT('Ctrl Pts',(189.651421417109,2.03078671951321,136.363904084189));
#216995=CARTESIAN_POINT('Ctrl Pts',(189.658834196411,1.88182232319197,136.413877112455));
#216996=CARTESIAN_POINT('Ctrl Pts',(189.66625756744,1.73264507955527,136.463921544528));
#216997=CARTESIAN_POINT('Ctrl Pts',(189.673680938469,1.58164016277834,136.507954145901));
#216998=CARTESIAN_POINT('Ctrl Pts',(189.681104309498,1.42933595688406,136.545869938717));
#216999=CARTESIAN_POINT('Ctrl Pts',(189.685040358939,1.3485806124279,136.565973801845));
#217000=CARTESIAN_POINT('Ctrl Pts',(189.688976408379,1.26746012441086,136.584358871603));
#217001=CARTESIAN_POINT('Ctrl Pts',(189.69291245782,1.18605385454001,136.601015412931));
#217002=CARTESIAN_POINT('Ctrl Pts',(189.700335724226,1.03252417016951,136.632429130043));
#217003=CARTESIAN_POINT('Ctrl Pts',(189.707758990631,0.877513437794605,
136.657786574917));
#217004=CARTESIAN_POINT('Ctrl Pts',(189.715182257037,0.721540807687306,
136.676950286983));
#217005=CARTESIAN_POINT('Ctrl Pts',(189.722596749758,0.56575252427599,136.696091349132));
#217006=CARTESIAN_POINT('Ctrl Pts',(189.730011242479,0.409004972998288,
136.709053204846));
#217007=CARTESIAN_POINT('Ctrl Pts',(189.7374257352,0.251829205035335,136.715749000509));
#217008=CARTESIAN_POINT('Ctrl Pts',(189.744833081553,0.0948049289951359,
136.722438342512));
#217009=CARTESIAN_POINT('Ctrl Pts',(189.752240427907,-0.0626463716075346,
136.722873632068));
#217010=CARTESIAN_POINT('Ctrl Pts',(189.759647774261,-0.219986889591926,
136.717019607471));
#217011=CARTESIAN_POINT('Ctrl Pts',(189.767049595936,-0.377210057081186,
136.711169949027));
#217012=CARTESIAN_POINT('Ctrl Pts',(189.774451417612,-0.534322235037135,
136.699040330281));
#217013=CARTESIAN_POINT('Ctrl Pts',(189.781853239287,-0.690784079832339,
136.68064753343));
#217014=CARTESIAN_POINT('Ctrl Pts',(189.789251153599,-0.847163329639719,
136.662264445992));
#217015=CARTESIAN_POINT('Ctrl Pts',(189.79664906791,-1.00289256018978,136.637624808542));
#217016=CARTESIAN_POINT('Ctrl Pts',(189.804046982221,-1.15743613013174,
136.606797361484));
#217017=CARTESIAN_POINT('Ctrl Pts',(189.811443667134,-1.31195401773457,
136.575975037388));
#217018=CARTESIAN_POINT('Ctrl Pts',(189.818840352046,-1.4652862700588,136.538967017513));
#217019=CARTESIAN_POINT('Ctrl Pts',(189.826237036958,-1.61690592382758,
136.4958934336));
#217020=CARTESIAN_POINT('Ctrl Pts',(189.833633393893,-1.76851885462208,
136.452821759614));
#217021=CARTESIAN_POINT('Ctrl Pts',(189.841029750829,-1.91841897876412,
136.403685158374));
#217022=CARTESIAN_POINT('Ctrl Pts',(189.848426107764,-2.0660932839906,136.348653999445));
#217023=CARTESIAN_POINT('Ctrl Pts',(189.855823597101,-2.21379019853027,
136.293614415105));
#217024=CARTESIAN_POINT('Ctrl Pts',(189.863221086437,-2.35926026579751,
136.232678606497));
#217025=CARTESIAN_POINT('Ctrl Pts',(189.870618575774,-2.50200942995244,
136.166065511994));
#217026=CARTESIAN_POINT('Ctrl Pts',(189.878018658289,-2.64480863460694,
136.099429066372));
#217027=CARTESIAN_POINT('Ctrl Pts',(189.885418740804,-2.78488469905547,
136.027111530211));
#217028=CARTESIAN_POINT('Ctrl Pts',(189.892818823319,-2.92176732847544,
135.949378230826));
#217029=CARTESIAN_POINT('Ctrl Pts',(189.900227042986,-3.05880047441704,
135.871559455687));
#217030=CARTESIAN_POINT('Ctrl Pts',(189.907635262652,-3.19263284780672,
135.788313208874));
#217031=CARTESIAN_POINT('Ctrl Pts',(189.915043482319,-3.32282174323811,
135.699949062806));
#217032=CARTESIAN_POINT('Ctrl Pts',(189.922456261621,-3.45309076776235,
135.611530530079));
#217033=CARTESIAN_POINT('Ctrl Pts',(189.929869040923,-3.579711546312,135.517988042663));
#217034=CARTESIAN_POINT('Ctrl Pts',(189.937281820225,-3.70227416517129,
135.419671719583));
#217035=CARTESIAN_POINT('Ctrl Pts',(189.944705191254,-3.82501190724813,
135.321214917531));
#217036=CARTESIAN_POINT('Ctrl Pts',(189.952128562282,-3.94367962786938,
135.217970900963));
#217037=CARTESIAN_POINT('Ctrl Pts',(189.959551933311,-4.05790340171897,
135.110327471226));
#217038=CARTESIAN_POINT('Ctrl Pts',(189.963487982752,-4.1184675873743,135.053252341912));
#217039=CARTESIAN_POINT('Ctrl Pts',(189.967424032192,-4.17778307250271,
134.994940957179));
#217040=CARTESIAN_POINT('Ctrl Pts',(189.971360081633,-4.23579876978104,
134.935454824241));
#217041=CARTESIAN_POINT('Ctrl Pts',(189.97868580183,-4.34377677455446,134.824740065172));
#217042=CARTESIAN_POINT('Ctrl Pts',(189.986011522027,-4.44759549208393,
134.709599597571));
#217043=CARTESIAN_POINT('Ctrl Pts',(189.993337242224,-4.54686303201109,
134.590383217952));
#217044=CARTESIAN_POINT('Ctrl Pts',(190.000654105557,-4.6460105565541,134.471310972051));
#217045=CARTESIAN_POINT('Ctrl Pts',(190.00797096889,-4.74061760854022,134.348172911224));
#217046=CARTESIAN_POINT('Ctrl Pts',(190.015287832222,-4.83032801012746,
134.221356648743));
#217047=CARTESIAN_POINT('Ctrl Pts',(190.022596306275,-4.91993555265535,
134.094685789707));
#217048=CARTESIAN_POINT('Ctrl Pts',(190.029904780328,-5.00465740532908,
133.964345439033));
#217049=CARTESIAN_POINT('Ctrl Pts',(190.037213254381,-5.08417700870137,
133.830756941033));
#217050=CARTESIAN_POINT('Ctrl Pts',(190.044516984866,-5.16364499985177,
133.697255148686));
#217051=CARTESIAN_POINT('Ctrl Pts',(190.051820715352,-5.23791726272298,
133.560509731128));
#217052=CARTESIAN_POINT('Ctrl Pts',(190.059124445837,-5.30671991172705,
133.420971849862));
#217053=CARTESIAN_POINT('Ctrl Pts',(190.06642496806,-5.3754923382356,133.281495262502));
#217054=CARTESIAN_POINT('Ctrl Pts',(190.073725490283,-5.43879976191837,
133.139228995741));
#217055=CARTESIAN_POINT('Ctrl Pts',(190.081026012506,-5.49641386784294,
132.994649446895));
#217056=CARTESIAN_POINT('Ctrl Pts',(190.088324859137,-5.55401475037018,
132.850103081465));
#217057=CARTESIAN_POINT('Ctrl Pts',(190.095623705769,-5.60592477449524,
132.703244847386));
#217058=CARTESIAN_POINT('Ctrl Pts',(190.1029225524,-5.65196358703582,132.554571511522));
#217059=CARTESIAN_POINT('Ctrl Pts',(190.110223624323,-5.69801643600718,
132.405852847751));
#217060=CARTESIAN_POINT('Ctrl Pts',(190.117524696245,-5.73819437761977,
132.255318341899));
#217061=CARTESIAN_POINT('Ctrl Pts',(190.124825768168,-5.77236675875697,
132.103480536934));
#217062=CARTESIAN_POINT('Ctrl Pts',(190.132127831751,-5.80654378132449,
131.951622108746));
#217063=CARTESIAN_POINT('Ctrl Pts',(190.139429895335,-5.83471354286302,
131.79846040554));
#217064=CARTESIAN_POINT('Ctrl Pts',(190.146731958918,-5.85679658929349,
131.644517908875));
#217065=CARTESIAN_POINT('Ctrl Pts',(190.154040273153,-5.87889853906686,
131.490443635655));
#217066=CARTESIAN_POINT('Ctrl Pts',(190.161348587387,-5.89490331910291,
131.33558761541));
#217067=CARTESIAN_POINT('Ctrl Pts',(190.168656901621,-5.90478335808391,
131.180477695875));
#217068=CARTESIAN_POINT('Ctrl Pts',(190.174646203679,-5.91288023732375,
131.053362176412));
#217069=CARTESIAN_POINT('Ctrl Pts',(190.180635505737,-5.91686463980822,
130.926076303123));
#217070=CARTESIAN_POINT('Ctrl Pts',(190.186624807795,-5.9167474892903,130.798909885783));
#217071=CARTESIAN_POINT('',(191.936624807795,-5.92167388468568,130.806439789968));
#217072=CARTESIAN_POINT('Ctrl Pts',(190.186624807795,-5.91709367293974,
130.798909566865));
#217073=CARTESIAN_POINT('Ctrl Pts',(190.207685773679,-5.92124324054971,
130.351707301601));
#217074=CARTESIAN_POINT('Ctrl Pts',(190.321562614164,-5.67042057656234,
127.938289561738));
#217075=CARTESIAN_POINT('Ctrl Pts',(190.52825532926,-2.36162413690314,124.216470821409));
#217076=CARTESIAN_POINT('Ctrl Pts',(190.80670295307,4.26606273237082,125.256543993538));
#217077=CARTESIAN_POINT('Ctrl Pts',(191.085150576885,6.97344635934664,131.394789617243));
#217078=CARTESIAN_POINT('Ctrl Pts',(191.363598200697,3.27257345387652,136.990459834304));
#217079=CARTESIAN_POINT('Ctrl Pts',(191.64204582451,-3.43563458160472,136.901407078928));
#217080=CARTESIAN_POINT('Ctrl Pts',(191.833054693543,-5.87156050063434,
132.996862586964));
#217081=CARTESIAN_POINT('Ctrl Pts',(191.931247687971,-5.92616743922034,
130.920188992212));
#217082=CARTESIAN_POINT('Ctrl Pts',(191.936624807795,-5.92565178765728,
130.806441186659));
#217083=CARTESIAN_POINT('',(193.686624807763,-5.91674833022066,130.808805764476));
#217084=CARTESIAN_POINT('Ctrl Pts',(191.936624807795,-5.91674963529206,
130.806438061004));
#217085=CARTESIAN_POINT('Ctrl Pts',(191.943982571507,-5.91680420246894,
130.651025731606));
#217086=CARTESIAN_POINT('Ctrl Pts',(191.95134033522,-5.91073134974623,130.495363673782));
#217087=CARTESIAN_POINT('Ctrl Pts',(191.958698098932,-5.89849824070525,
130.3399803134));
#217088=CARTESIAN_POINT('Ctrl Pts',(191.966047433817,-5.88627914553708,
130.184774955408));
#217089=CARTESIAN_POINT('Ctrl Pts',(191.973396768702,-5.86791386650228,
130.029848035039));
#217090=CARTESIAN_POINT('Ctrl Pts',(191.980746103587,-5.84342153691622,
129.875729741274));
#217091=CARTESIAN_POINT('Ctrl Pts',(191.988088691781,-5.81895169129261,
129.721752928126));
#217092=CARTESIAN_POINT('Ctrl Pts',(191.995431279975,-5.7883660488743,129.568583637425));
#217093=CARTESIAN_POINT('Ctrl Pts',(192.00277386817,-5.7517356631725,129.416748487506));
#217094=CARTESIAN_POINT('Ctrl Pts',(192.010111385737,-5.71513057359504,
129.265018191543));
#217095=CARTESIAN_POINT('Ctrl Pts',(192.017448903304,-5.67248913923677,
129.114620570674));
#217096=CARTESIAN_POINT('Ctrl Pts',(192.024786420871,-5.62393372693014,
128.966073371895));
#217097=CARTESIAN_POINT('Ctrl Pts',(192.032121243465,-5.57539614838435,
128.817580732537));
#217098=CARTESIAN_POINT('Ctrl Pts',(192.03945606606,-5.52094902955856,128.670937524576));
#217099=CARTESIAN_POINT('Ctrl Pts',(192.046790888654,-5.46076494507694,
128.52664755901));
#217100=CARTESIAN_POINT('Ctrl Pts',(192.054124432835,-5.40059135029389,
128.382382742256));
#217101=CARTESIAN_POINT('Ctrl Pts',(192.061457977017,-5.33468292520694,
128.240470702987));
#217102=CARTESIAN_POINT('Ctrl Pts',(192.068791521199,-5.2632607654466,128.101396193566));
#217103=CARTESIAN_POINT('Ctrl Pts',(192.076125297015,-5.19183634977695,
127.962317291398));
#217104=CARTESIAN_POINT('Ctrl Pts',(192.083459072831,-5.11489802642811,
127.826076435999));
#217105=CARTESIAN_POINT('Ctrl Pts',(192.090792848647,-5.03271319836429,
127.693134424325));
#217106=CARTESIAN_POINT('Ctrl Pts',(192.098128366077,-4.95050885317121,
127.560160841782));
#217107=CARTESIAN_POINT('Ctrl Pts',(192.105463883507,-4.86305572373874,
127.43048798552));
#217108=CARTESIAN_POINT('Ctrl Pts',(192.112799400937,-4.77066480062535,
127.304548062218));
#217109=CARTESIAN_POINT('Ctrl Pts',(192.120142509709,-4.67817826447584,
127.178477806865));
#217110=CARTESIAN_POINT('Ctrl Pts',(192.12748561848,-4.58074395310877,127.056148507902));
#217111=CARTESIAN_POINT('Ctrl Pts',(192.134828727252,-4.47871388483845,
126.937960159743));
#217112=CARTESIAN_POINT('Ctrl Pts',(192.142175724157,-4.37662979224858,
126.81970923155));
#217113=CARTESIAN_POINT('Ctrl Pts',(192.149522721062,-4.26994535451669,
126.705603899663));
#217114=CARTESIAN_POINT('Ctrl Pts',(192.156869717967,-4.15904929270293,
126.596007074508));
#217115=CARTESIAN_POINT('Ctrl Pts',(192.164227936362,-4.04798385296286,
126.486242855825));
#217116=CARTESIAN_POINT('Ctrl Pts',(192.171586154757,-3.93269421798494,
126.381001158029));
#217117=CARTESIAN_POINT('Ctrl Pts',(192.178944373152,-3.81360275633488,
126.280605034052));
#217118=CARTESIAN_POINT('Ctrl Pts',(192.18560993948,-3.70572174572714,126.189659510622));
#217119=CARTESIAN_POINT('Ctrl Pts',(192.192275505808,-3.59472154676677,
126.102689823874));
#217120=CARTESIAN_POINT('Ctrl Pts',(192.198941072137,-3.48093537284348,
126.019904588655));
#217121=CARTESIAN_POINT('Ctrl Pts',(192.206364338542,-3.35421469515357,
125.927708843354));
#217122=CARTESIAN_POINT('Ctrl Pts',(192.213787604947,-3.22363703874374,
125.840411633728));
#217123=CARTESIAN_POINT('Ctrl Pts',(192.221210871353,-3.08961796002339,
125.758353143969));
#217124=CARTESIAN_POINT('Ctrl Pts',(192.228625364074,-2.95575728072412,
125.676391640529));
#217125=CARTESIAN_POINT('Ctrl Pts',(192.236039856795,-2.8184635906989,125.599656725305));
#217126=CARTESIAN_POINT('Ctrl Pts',(192.243454349516,-2.67818424350777,
125.528447452973));
#217127=CARTESIAN_POINT('Ctrl Pts',(192.25086169587,-2.53804010283326,125.457306814819));
#217128=CARTESIAN_POINT('Ctrl Pts',(192.258269042224,-2.39491636453648,
125.39168138473));
#217129=CARTESIAN_POINT('Ctrl Pts',(192.265676388577,-2.24928790474382,
125.331826059971));
#217130=CARTESIAN_POINT('Ctrl Pts',(192.273078210253,-2.10376806015,125.272015377571));
#217131=CARTESIAN_POINT('Ctrl Pts',(192.280480031928,-1.95574755751648,
125.21796637283));
#217132=CARTESIAN_POINT('Ctrl Pts',(192.287881853604,-1.80572423221982,
125.169887211854));
#217133=CARTESIAN_POINT('Ctrl Pts',(192.295279767915,-1.65578010306985,
125.121833431494));
#217134=CARTESIAN_POINT('Ctrl Pts',(192.302677682226,-1.5038356114583,125.079743332305));
#217135=CARTESIAN_POINT('Ctrl Pts',(192.310075596538,-1.35040674849502,
125.04377625692));
#217136=CARTESIAN_POINT('Ctrl Pts',(192.31747228145,-1.19700338262484,125.007815158611));
#217137=CARTESIAN_POINT('Ctrl Pts',(192.324868966362,-1.04211649807024,
124.977975149715));
#217138=CARTESIAN_POINT('Ctrl Pts',(192.332265651274,-0.886275478114352,
124.954365203944));
#217139=CARTESIAN_POINT('Ctrl Pts',(192.33966200821,-0.73044136831249,124.930756305064));
#217140=CARTESIAN_POINT('Ctrl Pts',(192.347058365145,-0.573653576316578,
124.913376975953));
#217141=CARTESIAN_POINT('Ctrl Pts',(192.354454722081,-0.416449600545396,
124.902284686785));
#217142=CARTESIAN_POINT('Ctrl Pts',(192.361852211417,-0.259221556444396,
124.891190699359));
#217143=CARTESIAN_POINT('Ctrl Pts',(192.369249700754,-0.10157757409154,
124.886385694742));
#217144=CARTESIAN_POINT('Ctrl Pts',(192.37664719009,0.0559419800692496,
124.887875084974));
#217145=CARTESIAN_POINT('Ctrl Pts',(192.384047272605,0.213516752465648,
124.88936499731));
#217146=CARTESIAN_POINT('Ctrl Pts',(192.39144735512,0.370966636778287,124.897153694073));
#217147=CARTESIAN_POINT('Ctrl Pts',(192.398847437635,0.527753674510833,
124.911194522712));
#217148=CARTESIAN_POINT('Ctrl Pts',(192.406255657302,0.684713115709465,
124.925250790685));
#217149=CARTESIAN_POINT('Ctrl Pts',(192.413663876968,0.841007882692738,
124.945572886768));
#217150=CARTESIAN_POINT('Ctrl Pts',(192.421072096635,0.996106797477932,
124.972062458991));
#217151=CARTESIAN_POINT('Ctrl Pts',(192.428484875937,1.15130117305738,124.998568335104));
#217152=CARTESIAN_POINT('Ctrl Pts',(192.435897655239,1.30529786549359,125.031249174006));
#217153=CARTESIAN_POINT('Ctrl Pts',(192.443310434541,1.45757874437968,125.069956135283));
#217154=CARTESIAN_POINT('Ctrl Pts',(192.45073380557,1.61007720932673,125.108718402881));
#217155=CARTESIAN_POINT('Ctrl Pts',(192.458157176598,1.76085460737413,125.153523883713));
#217156=CARTESIAN_POINT('Ctrl Pts',(192.465580547627,1.90940995179483,125.204174531507));
#217157=CARTESIAN_POINT('Ctrl Pts',(192.469516597068,1.9881775599421,125.231030720313));
#217158=CARTESIAN_POINT('Ctrl Pts',(192.473452646509,2.06632082359468,125.259529399429));
#217159=CARTESIAN_POINT('Ctrl Pts',(192.477388695949,2.14376776436376,125.289635752718));
#217160=CARTESIAN_POINT('Ctrl Pts',(192.484811962355,2.28983027762013,125.346415395433));
#217161=CARTESIAN_POINT('Ctrl Pts',(192.49223522876,2.43385630529008,125.409087801767));
#217162=CARTESIAN_POINT('Ctrl Pts',(192.499658495166,2.57533502238865,125.477487230207));
#217163=CARTESIAN_POINT('Ctrl Pts',(192.507072987887,2.71664652339273,125.545805816202));
#217164=CARTESIAN_POINT('Ctrl Pts',(192.514487480608,2.85541637385971,125.619837789946));
#217165=CARTESIAN_POINT('Ctrl Pts',(192.521901973329,2.99115116509402,125.699368426577));
#217166=CARTESIAN_POINT('Ctrl Pts',(192.529309319682,3.1267551300262,125.778822408586));
#217167=CARTESIAN_POINT('Ctrl Pts',(192.536716666036,3.25932953951027,125.863764315137));
#217168=CARTESIAN_POINT('Ctrl Pts',(192.54412401239,3.38840325911156,125.953932397693));
#217169=CARTESIAN_POINT('Ctrl Pts',(192.551525834065,3.51738071066331,126.044033229491));
#217170=CARTESIAN_POINT('Ctrl Pts',(192.558927655741,3.64286236637453,126.139352263232));
#217171=CARTESIAN_POINT('Ctrl Pts',(192.566329477416,3.76440399802195,126.239583174779));
#217172=CARTESIAN_POINT('Ctrl Pts',(192.573727391728,3.88588146878789,126.339761175208));
#217173=CARTESIAN_POINT('Ctrl Pts',(192.581125306039,4.00342277045593,126.444845652573));
#217174=CARTESIAN_POINT('Ctrl Pts',(192.58852322035,4.11661493775789,126.554488617525));
#217175=CARTESIAN_POINT('Ctrl Pts',(192.595919905262,4.22978829457512,126.664113361806));
#217176=CARTESIAN_POINT('Ctrl Pts',(192.603316590175,4.33861368359645,126.778294830715));
#217177=CARTESIAN_POINT('Ctrl Pts',(192.610713275087,4.44271327755592,126.896646542057));
#217178=CARTESIAN_POINT('Ctrl Pts',(192.618109632022,4.54680825563025,127.01499300556));
#217179=CARTESIAN_POINT('Ctrl Pts',(192.625505988958,4.64617760874819,127.137509063529));
#217180=CARTESIAN_POINT('Ctrl Pts',(192.632902345893,4.74048245459971,127.263773567354));
#217181=CARTESIAN_POINT('Ctrl Pts',(192.64029983523,4.83480173876412,127.390057402596));
#217182=CARTESIAN_POINT('Ctrl Pts',(192.647697324566,4.92405474836339,127.520090527295));
#217183=CARTESIAN_POINT('Ctrl Pts',(192.655094813903,5.00794484883268,127.653421241197));
#217184=CARTESIAN_POINT('Ctrl Pts',(192.662494896418,5.09186435684631,127.786798693974));
#217185=CARTESIAN_POINT('Ctrl Pts',(192.669894978933,5.1704170140703,127.923475721708));
#217186=CARTESIAN_POINT('Ctrl Pts',(192.677295061448,5.24335129090999,128.062974507837));
#217187=CARTESIAN_POINT('Ctrl Pts',(192.684703281114,5.31636576648502,128.202626687223));
#217188=CARTESIAN_POINT('Ctrl Pts',(192.692111500781,5.38374935076555,128.345106490511));
#217189=CARTESIAN_POINT('Ctrl Pts',(192.699519720447,5.4452976753735,128.48991386098));
#217190=CARTESIAN_POINT('Ctrl Pts',(192.706932499749,5.50688388194844,128.634810357969));
#217191=CARTESIAN_POINT('Ctrl Pts',(192.714345279052,5.56262754045087,128.782036928429));
#217192=CARTESIAN_POINT('Ctrl Pts',(192.721758058354,5.61237381239609,128.931077202695));
#217193=CARTESIAN_POINT('Ctrl Pts',(192.729181429382,5.66219116414747,129.080330432694));
#217194=CARTESIAN_POINT('Ctrl Pts',(192.736604800411,5.70599391075369,129.231402184733));
#217195=CARTESIAN_POINT('Ctrl Pts',(192.74402817144,5.74367787858866,129.383763915644));
#217196=CARTESIAN_POINT('Ctrl Pts',(192.747964220881,5.76365882254902,129.464549761242));
#217197=CARTESIAN_POINT('Ctrl Pts',(192.751900270321,5.7819204194436,129.545698134267));
#217198=CARTESIAN_POINT('Ctrl Pts',(192.755836319762,5.79845305499836,129.627129658289));
#217199=CARTESIAN_POINT('Ctrl Pts',(192.763259586168,5.82963308968896,129.780706971204));
#217200=CARTESIAN_POINT('Ctrl Pts',(192.770682852573,5.85475460525286,129.935756113794));
#217201=CARTESIAN_POINT('Ctrl Pts',(192.778106118978,5.87368093133555,130.091757727195));
#217202=CARTESIAN_POINT('Ctrl Pts',(192.785520611699,5.89258488807253,130.247574959644));
#217203=CARTESIAN_POINT('Ctrl Pts',(192.79293510442,5.90530818568646,130.404342055148));
#217204=CARTESIAN_POINT('Ctrl Pts',(192.800349597141,5.91176477883311,130.561527830965));
#217205=CARTESIAN_POINT('Ctrl Pts',(192.807756943495,5.91821514887222,130.718562105214));
#217206=CARTESIAN_POINT('Ctrl Pts',(192.815164289849,5.91841082384763,130.876013885927));
#217207=CARTESIAN_POINT('Ctrl Pts',(192.822571636203,5.91231736054565,131.033345312885));
#217208=CARTESIAN_POINT('Ctrl Pts',(192.829973457878,5.90622844197851,131.190559396129));
#217209=CARTESIAN_POINT('Ctrl Pts',(192.837375279553,5.89385973928897,131.347652932937));
#217210=CARTESIAN_POINT('Ctrl Pts',(192.844777101229,5.8752288554425,131.504086605847));
#217211=CARTESIAN_POINT('Ctrl Pts',(192.85217501554,5.8566078066946,131.660437698638));
#217212=CARTESIAN_POINT('Ctrl Pts',(192.859572929851,5.83173120439777,131.816129251521));
#217213=CARTESIAN_POINT('Ctrl Pts',(192.866970844163,5.80066860403245,131.970625728376));
#217214=CARTESIAN_POINT('Ctrl Pts',(192.874367529075,5.76961116570776,132.125096530719));
#217215=CARTESIAN_POINT('Ctrl Pts',(192.881764213987,5.73236984310127,132.278372285581));
#217216=CARTESIAN_POINT('Ctrl Pts',(192.889160898899,5.6890655697637,132.429926213114));
#217217=CARTESIAN_POINT('Ctrl Pts',(192.896557255835,5.64576321658296,132.581473420587));
#217218=CARTESIAN_POINT('Ctrl Pts',(192.90395361277,5.5963985497707,132.731298593605));
#217219=CARTESIAN_POINT('Ctrl Pts',(192.911349969705,5.54114271941322,132.878888979771));
#217220=CARTESIAN_POINT('Ctrl Pts',(192.918747459042,5.48587842924699,133.026501962402));
#217221=CARTESIAN_POINT('Ctrl Pts',(192.926144948379,5.42472131052274,133.17187912729));
#217222=CARTESIAN_POINT('Ctrl Pts',(192.933542437715,5.35789105322837,133.314526752354));
#217223=CARTESIAN_POINT('Ctrl Pts',(192.94094252023,5.29103736869093,133.457224382321));
#217224=CARTESIAN_POINT('Ctrl Pts',(192.948342602745,5.21850674434839,133.597190229583));
#217225=CARTESIAN_POINT('Ctrl Pts',(192.95574268526,5.14056522291733,133.733954403645));
#217226=CARTESIAN_POINT('Ctrl Pts',(192.963150904926,5.06253799677085,133.870868963976));
#217227=CARTESIAN_POINT('Ctrl Pts',(192.970559124593,4.97908817626604,134.004574495774));
#217228=CARTESIAN_POINT('Ctrl Pts',(192.977967344259,4.89052600718495,134.13462876526));
#217229=CARTESIAN_POINT('Ctrl Pts',(192.985380123561,4.80190932956638,134.26476308098));
#217230=CARTESIAN_POINT('Ctrl Pts',(192.992792902864,4.70817425520031,134.391241357163));
#217231=CARTESIAN_POINT('Ctrl Pts',(193.000205682166,4.60967152652743,134.51365421339));
#217232=CARTESIAN_POINT('Ctrl Pts',(193.007629053194,4.51102805253667,134.636241978846));
#217233=CARTESIAN_POINT('Ctrl Pts',(193.015052424223,4.40760356345385,134.754752442234));
#217234=CARTESIAN_POINT('Ctrl Pts',(193.022475795252,4.29978642922707,134.868812268839));
#217235=CARTESIAN_POINT('Ctrl Pts',(193.026411844693,4.24261919762311,134.929289525733));
#217236=CARTESIAN_POINT('Ctrl Pts',(193.030347894133,4.18421761234096,134.988516202176));
#217237=CARTESIAN_POINT('Ctrl Pts',(193.034283943574,4.12464325826948,135.046441304506));
#217238=CARTESIAN_POINT('Ctrl Pts',(193.04170720998,4.01228788574312,135.155686239721));
#217239=CARTESIAN_POINT('Ctrl Pts',(193.049130476385,3.89541944365211,135.260629531099));
#217240=CARTESIAN_POINT('Ctrl Pts',(193.05655374279,3.77440100965145,135.360875467848));
#217241=CARTESIAN_POINT('Ctrl Pts',(193.063968235512,3.65352560938941,135.461002922225));
#217242=CARTESIAN_POINT('Ctrl Pts',(193.071382728233,3.52851026521044,135.55644383722));
#217243=CARTESIAN_POINT('Ctrl Pts',(193.078797220954,3.39975536658942,135.6468387032));
#217244=CARTESIAN_POINT('Ctrl Pts',(193.086204567307,3.27112456678774,135.737146443204));
#217245=CARTESIAN_POINT('Ctrl Pts',(193.093611913661,3.13876169151149,135.822417603552));
#217246=CARTESIAN_POINT('Ctrl Pts',(193.101019260015,3.0031006403987,135.902332479605));
#217247=CARTESIAN_POINT('Ctrl Pts',(193.10842108169,2.86754077041626,135.982187752127));
#217248=CARTESIAN_POINT('Ctrl Pts',(193.115822903366,2.72868794285352,136.056694506122));
#217249=CARTESIAN_POINT('Ctrl Pts',(193.123224725041,2.58700541559937,136.125576037201));
#217250=CARTESIAN_POINT('Ctrl Pts',(193.130622639352,2.44539768144717,136.194421206256));
#217251=CARTESIAN_POINT('Ctrl Pts',(193.138020553664,2.30096355740562,136.257646903513));
#217252=CARTESIAN_POINT('Ctrl Pts',(193.145418467975,2.15419120161526,136.315022177613));
#217253=CARTESIAN_POINT('Ctrl Pts',(193.152815152887,2.00744323672871,136.372387916984));
#217254=CARTESIAN_POINT('Ctrl Pts',(193.1602118378,1.85835815862988,136.423905027017));
#217255=CARTESIAN_POINT('Ctrl Pts',(193.167608522712,1.70744452966099,136.46939051516));
#217256=CARTESIAN_POINT('Ctrl Pts',(193.175004879647,1.55653759236051,136.514873986428));
#217257=CARTESIAN_POINT('Ctrl Pts',(193.182401236583,1.40380262282025,136.554326259858));
#217258=CARTESIAN_POINT('Ctrl Pts',(193.189797593518,1.24976352495471,136.58761417367));
#217259=CARTESIAN_POINT('Ctrl Pts',(193.197195082855,1.09570084331009,136.620907183947));
#217260=CARTESIAN_POINT('Ctrl Pts',(193.204592572191,0.94033400067869,136.648033876561));
#217261=CARTESIAN_POINT('Ctrl Pts',(193.211990061528,0.78419712723474,136.668912214077));
#217262=CARTESIAN_POINT('Ctrl Pts',(193.219390144043,0.628005520252473,
136.689797870461));
#217263=CARTESIAN_POINT('Ctrl Pts',(193.226790226558,0.471043714796622,
136.704430761329));
#217264=CARTESIAN_POINT('Ctrl Pts',(193.234190309073,0.313850845635412,
136.712780728661));
#217265=CARTESIAN_POINT('Ctrl Pts',(193.241598528739,0.156485126754066,
136.721139877641));
#217266=CARTESIAN_POINT('Ctrl Pts',(193.249006748406,-0.00111179024260466,
136.723202286104));
#217267=CARTESIAN_POINT('Ctrl Pts',(193.256414968072,-0.15840014612975,
136.718989934455));
#217268=CARTESIAN_POINT('Ctrl Pts',(193.263827747375,-0.315785310375573,
136.714774990174));
#217269=CARTESIAN_POINT('Ctrl Pts',(193.271240526677,-0.472861163480505,
136.704277615075));
#217270=CARTESIAN_POINT('Ctrl Pts',(193.278653305979,-0.629093697246785,
136.687571618591));
#217271=CARTESIAN_POINT('Ctrl Pts',(193.286076677007,-0.785549463383723,
136.670841751796));
#217272=CARTESIAN_POINT('Ctrl Pts',(193.293500048036,-0.941159135255626,
136.647885600237));
#217273=CARTESIAN_POINT('Ctrl Pts',(193.300923419065,-1.09539869234955,
136.618828114018));
#217274=CARTESIAN_POINT('Ctrl Pts',(193.304859468506,-1.17718020644852,
136.6034211376));
#217275=CARTESIAN_POINT('Ctrl Pts',(193.308795517947,-1.25857677010934,
136.586299695192));
#217276=CARTESIAN_POINT('Ctrl Pts',(193.312731567387,-1.33951219278451,
136.567488036588));
#217277=CARTESIAN_POINT('Ctrl Pts',(193.320154833793,-1.49215387404138,
136.532009835551));
#217278=CARTESIAN_POINT('Ctrl Pts',(193.327578100198,-1.64361588484665,
136.490409517706));
#217279=CARTESIAN_POINT('Ctrl Pts',(193.335001366604,-1.79336905016339,
136.442778659217));
#217280=CARTESIAN_POINT('Ctrl Pts',(193.342415859325,-1.94294521967514,
136.395204096447));
#217281=CARTESIAN_POINT('Ctrl Pts',(193.349830352046,-2.0908162116855,136.3416132926));
#217282=CARTESIAN_POINT('Ctrl Pts',(193.357244844767,-2.23646314026778,
136.282148782941));
#217283=CARTESIAN_POINT('Ctrl Pts',(193.364652191121,-2.38196968885627,
136.222741587416));
#217284=CARTESIAN_POINT('Ctrl Pts',(193.372059537474,-2.52525609829113,
136.157472096766));
#217285=CARTESIAN_POINT('Ctrl Pts',(193.379466883828,-2.66581885865279,
136.08653255488));
#217286=CARTESIAN_POINT('Ctrl Pts',(193.386868705504,-2.80627678200372,
136.015645922381));
#217287=CARTESIAN_POINT('Ctrl Pts',(193.394270527179,-2.94401476924652,
135.9390978265));
#217288=CARTESIAN_POINT('Ctrl Pts',(193.401672348854,-3.07854961893739,
135.857128453737));
#217289=CARTESIAN_POINT('Ctrl Pts',(193.409070263166,-3.21301344872921,
135.775202351967));
#217290=CARTESIAN_POINT('Ctrl Pts',(193.416468177477,-3.34427719051927,
135.687860866565));
#217291=CARTESIAN_POINT('Ctrl Pts',(193.423866091788,-3.47188267699022,
135.595389863951));
#217292=CARTESIAN_POINT('Ctrl Pts',(193.4312627767,-3.59946695774474,135.502934228339));
#217293=CARTESIAN_POINT('Ctrl Pts',(193.438659461613,-3.72339388777422,
135.405350986174));
#217294=CARTESIAN_POINT('Ctrl Pts',(193.446056146525,-3.84323461989282,
135.302969093412));
#217295=CARTESIAN_POINT('Ctrl Pts',(193.45345250346,-3.96307003814781,135.200591740371));
#217296=CARTESIAN_POINT('Ctrl Pts',(193.460848860396,-4.07881933492679,
135.093416402282));
#217297=CARTESIAN_POINT('Ctrl Pts',(193.468245217331,-4.19008729459038,
134.981811877151));
#217298=CARTESIAN_POINT('Ctrl Pts',(193.475642706668,-4.30137228966243,
134.870190265084));
#217299=CARTESIAN_POINT('Ctrl Pts',(193.483040196004,-4.40817431791499,
134.754138380124));
#217300=CARTESIAN_POINT('Ctrl Pts',(193.490437685341,-4.51013564852389,
134.634061257879));
#217301=CARTESIAN_POINT('Ctrl Pts',(193.497837767856,-4.61213272151835,
134.513942042786));
#217302=CARTESIAN_POINT('Ctrl Pts',(193.505237850371,-4.70928547688403,
134.389795065409));
#217303=CARTESIAN_POINT('Ctrl Pts',(193.512637932886,-4.80127712631488,
134.262057613953));
#217304=CARTESIAN_POINT('Ctrl Pts',(193.520046152552,-4.89336993002218,
134.134179702037));
#217305=CARTESIAN_POINT('Ctrl Pts',(193.527454372219,-4.98029007582845,
134.002703734542));
#217306=CARTESIAN_POINT('Ctrl Pts',(193.534862591885,-5.06176430342499,
133.868095707138));
#217307=CARTESIAN_POINT('Ctrl Pts',(193.542275371188,-5.14328867704949,
133.733404830738));
#217308=CARTESIAN_POINT('Ctrl Pts',(193.54968815049,-5.21936027347246,133.595578379247));
#217309=CARTESIAN_POINT('Ctrl Pts',(193.557100929792,-5.28975254618504,
133.455105524687));
#217310=CARTESIAN_POINT('Ctrl Pts',(193.564524300821,-5.36024539867765,
133.314431955926));
#217311=CARTESIAN_POINT('Ctrl Pts',(193.571947671849,-5.42504256684365,
133.171104771232));
#217312=CARTESIAN_POINT('Ctrl Pts',(193.579371042878,-5.48396592885686,
133.025632382487));
#217313=CARTESIAN_POINT('Ctrl Pts',(193.583307092319,-5.51520850924322,
132.948499431412));
#217314=CARTESIAN_POINT('Ctrl Pts',(193.58724314176,-5.54480058572185,132.870763639298));
#217315=CARTESIAN_POINT('Ctrl Pts',(193.591179191201,-5.57272137747765,
132.792502215014));
#217316=CARTESIAN_POINT('Ctrl Pts',(193.59982438893,-5.63404702115283,132.62060765482));
#217317=CARTESIAN_POINT('Ctrl Pts',(193.60846958666,-5.6874596691831,132.445749915596));
#217318=CARTESIAN_POINT('Ctrl Pts',(193.61711478439,-5.7327048543804,132.268609781835));
#217319=CARTESIAN_POINT('Ctrl Pts',(193.625725250551,-5.77776826973561,
132.092181298032));
#217320=CARTESIAN_POINT('Ctrl Pts',(193.634335716713,-5.81472962923724,
131.913488824043));
#217321=CARTESIAN_POINT('Ctrl Pts',(193.642946182875,-5.84338413695381,
131.733226803029));
#217322=CARTESIAN_POINT('Ctrl Pts',(193.651489290023,-5.87181448266578,
131.554374957907));
#217323=CARTESIAN_POINT('Ctrl Pts',(193.660032397172,-5.89206736515099,
131.373978144609));
#217324=CARTESIAN_POINT('Ctrl Pts',(193.668575504321,-5.90398986112245,
131.192734512496));
#217325=CARTESIAN_POINT('Ctrl Pts',(193.674591938801,-5.91238621090631,
131.065094718366));
#217326=CARTESIAN_POINT('Ctrl Pts',(193.680608373282,-5.91665199363111,
130.937035352127));
#217327=CARTESIAN_POINT('Ctrl Pts',(193.686624807763,-5.91674833022066,
130.808805764476));
#217328=CARTESIAN_POINT('',(195.436626015881,-5.91264468443637,130.800534531502));
#217329=CARTESIAN_POINT('Ctrl Pts',(193.686624807795,-5.91674833022117,
130.808805763797));
#217330=CARTESIAN_POINT('Ctrl Pts',(193.694249891429,-5.91687042486749,
130.646290683926));
#217331=CARTESIAN_POINT('Ctrl Pts',(193.701874975063,-5.91029198571113,
130.483707620702));
#217332=CARTESIAN_POINT('Ctrl Pts',(193.709500058697,-5.89702633263468,
130.321648493507));
#217333=CARTESIAN_POINT('Ctrl Pts',(193.716903394445,-5.8841464629385,130.164302267934));
#217334=CARTESIAN_POINT('Ctrl Pts',(193.724306730192,-5.86496295699468,
130.007450318832));
#217335=CARTESIAN_POINT('Ctrl Pts',(193.731710065939,-5.839540805705,129.851630991173));
#217336=CARTESIAN_POINT('Ctrl Pts',(193.739114086533,-5.81411630273351,
129.695797249413));
#217337=CARTESIAN_POINT('Ctrl Pts',(193.746518107128,-5.78245206455313,
129.540996686389));
#217338=CARTESIAN_POINT('Ctrl Pts',(193.753922127722,-5.74466447835844,
129.387758840923));
#217339=CARTESIAN_POINT('Ctrl Pts',(193.761328280158,-5.70686601197486,
129.234476873648));
#217340=CARTESIAN_POINT('Ctrl Pts',(193.768734432594,-5.66294077563007,
129.082758880831));
#217341=CARTESIAN_POINT('Ctrl Pts',(193.776140585029,-5.61305539489754,
128.933120468277));
#217342=CARTESIAN_POINT('Ctrl Pts',(193.783931104195,-5.56058104765214,
128.775716076322));
#217343=CARTESIAN_POINT('Ctrl Pts',(193.79172162336,-5.50151156375219,128.620613319595));
#217344=CARTESIAN_POINT('Ctrl Pts',(193.799512142525,-5.43609843388967,
128.468388789919));
#217345=CARTESIAN_POINT('Ctrl Pts',(193.806931140232,-5.37380478565584,
128.32342368392));
#217346=CARTESIAN_POINT('Ctrl Pts',(193.814350137939,-5.3057587036248,128.181068965662));
#217347=CARTESIAN_POINT('Ctrl Pts',(193.821769135646,-5.23222448513309,
128.041797043696));
#217348=CARTESIAN_POINT('Ctrl Pts',(193.829193605055,-5.15863603325452,
127.902422405087));
#217349=CARTESIAN_POINT('Ctrl Pts',(193.836618074465,-5.07955156595895,
127.766135413061));
#217350=CARTESIAN_POINT('Ctrl Pts',(193.844042543874,-4.99527888296432,
127.633379784462));
#217351=CARTESIAN_POINT('Ctrl Pts',(193.851477405336,-4.91088824323663,
127.500438337403));
#217352=CARTESIAN_POINT('Ctrl Pts',(193.858912266798,-4.82129510231583,
127.371038424274));
#217353=CARTESIAN_POINT('Ctrl Pts',(193.86634712826,-4.72684806539047,127.245591458262));
#217354=CARTESIAN_POINT('Ctrl Pts',(193.867440357178,-4.71296048557474,
127.227145620151));
#217355=CARTESIAN_POINT('Ctrl Pts',(193.868533586096,-4.69896802508309,
127.20878518446));
#217356=CARTESIAN_POINT('Ctrl Pts',(193.869626815014,-4.68487185884326,
127.190511391503));
#217357=CARTESIAN_POINT('Ctrl Pts',(193.877050081419,-4.58915576902482,
127.066428291302));
#217358=CARTESIAN_POINT('Ctrl Pts',(193.884473347825,-4.48836185950119,
126.945962881474));
#217359=CARTESIAN_POINT('Ctrl Pts',(193.89189661423,-4.38279338078887,126.82955839056));
#217360=CARTESIAN_POINT('Ctrl Pts',(193.899311106951,-4.27734967525132,
126.713291480087));
#217361=CARTESIAN_POINT('Ctrl Pts',(193.906725599672,-4.16714288156309,
126.601076208577));
#217362=CARTESIAN_POINT('Ctrl Pts',(193.914140092393,-4.0525183215702,126.493325264447));
#217363=CARTESIAN_POINT('Ctrl Pts',(193.921547438747,-3.93800424104399,
126.385678174735));
#217364=CARTESIAN_POINT('Ctrl Pts',(193.928954785101,-3.81908114123644,
126.282487100167));
#217365=CARTESIAN_POINT('Ctrl Pts',(193.936362131454,-3.69613316353616,
126.184130082202));
#217366=CARTESIAN_POINT('Ctrl Pts',(193.94376395313,-3.57327688507596,126.085846422612));
#217367=CARTESIAN_POINT('Ctrl Pts',(193.951165774805,-3.44640199616621,
125.992389872936));
#217368=CARTESIAN_POINT('Ctrl Pts',(193.958567596481,-3.31592780126095,
125.904100075582));
#217369=CARTESIAN_POINT('Ctrl Pts',(193.965965510792,-3.18552248266734,
125.815856885725));
#217370=CARTESIAN_POINT('Ctrl Pts',(193.973363425103,-3.05152195049331,
125.732775224944));
#217371=CARTESIAN_POINT('Ctrl Pts',(193.980761339415,-2.91437665000294,
125.655152979063));
#217372=CARTESIAN_POINT('Ctrl Pts',(193.988158024327,-2.77725414057385,
125.577543632592));
#217373=CARTESIAN_POINT('Ctrl Pts',(193.995554709239,-2.63698822459584,
125.505392084079));
#217374=CARTESIAN_POINT('Ctrl Pts',(194.002951394151,-2.49405635059935,
125.438951641306));
#217375=CARTESIAN_POINT('Ctrl Pts',(194.010347751087,-2.35113081435208,
125.372514144571));
#217376=CARTESIAN_POINT('Ctrl Pts',(194.017744108022,-2.20553989364301,
125.31178740741));
#217377=CARTESIAN_POINT('Ctrl Pts',(194.025140464957,-2.057783294511,125.256977588125));
#217378=CARTESIAN_POINT('Ctrl Pts',(194.032537954294,-1.9100040734663,125.202159377317));
#217379=CARTESIAN_POINT('Ctrl Pts',(194.039935443631,-1.76005886381328,
125.15326001798));
#217380=CARTESIAN_POINT('Ctrl Pts',(194.047332932967,-1.60846474911433,
125.110436512579));
#217381=CARTESIAN_POINT('Ctrl Pts',(194.054733015482,-1.45681749333343,
125.067597995464));
#217382=CARTESIAN_POINT('Ctrl Pts',(194.062133097997,-1.30352054068615,
125.030839674279));
#217383=CARTESIAN_POINT('Ctrl Pts',(194.069533180512,-1.14910329058166,
125.000267907239));
#217384=CARTESIAN_POINT('Ctrl Pts',(194.076941400178,-0.994516242836139,
124.969662523398));
#217385=CARTESIAN_POINT('Ctrl Pts',(194.084349619845,-0.838806803898584,
124.945257351789));
#217386=CARTESIAN_POINT('Ctrl Pts',(194.091757839511,-0.68251238996658,
124.927107228436));
#217387=CARTESIAN_POINT('Ctrl Pts',(194.099170618813,-0.526121779430448,
124.908945933984));
#217388=CARTESIAN_POINT('Ctrl Pts',(194.106583398116,-0.369145847837443,
124.897047387302));
#217389=CARTESIAN_POINT('Ctrl Pts',(194.113996177418,-0.212123673302736,
124.891414303779));
#217390=CARTESIAN_POINT('Ctrl Pts',(194.121419548446,-0.0548771381217091,
124.885773171442));
#217391=CARTESIAN_POINT('Ctrl Pts',(194.128842919475,0.102415399659899,
124.886415380671));
#217392=CARTESIAN_POINT('Ctrl Pts',(194.136266290504,0.259217491474521,
124.893291606413));
#217393=CARTESIAN_POINT('Ctrl Pts',(194.140202339945,0.342357722969995,
124.896937546294));
#217394=CARTESIAN_POINT('Ctrl Pts',(194.144138389385,0.425360189154594,
124.902335228505));
#217395=CARTESIAN_POINT('Ctrl Pts',(194.148074438826,0.508146029354237,
124.909471460393));
#217396=CARTESIAN_POINT('Ctrl Pts',(194.155497705232,0.664277540311929,
124.922930171021));
#217397=CARTESIAN_POINT('Ctrl Pts',(194.162920971637,0.820110071483281,
124.942616445193));
#217398=CARTESIAN_POINT('Ctrl Pts',(194.170344238043,0.975106807833801,
124.968514725511));
#217399=CARTESIAN_POINT('Ctrl Pts',(194.177758730764,1.12992035091363,124.994382396213));
#217400=CARTESIAN_POINT('Ctrl Pts',(194.185173223485,1.28389970087569,125.0264473977));
#217401=CARTESIAN_POINT('Ctrl Pts',(194.192587716206,1.43651099637365,125.064642269093));
#217402=CARTESIAN_POINT('Ctrl Pts',(194.199995062559,1.58897519935966,125.102800326831));
#217403=CARTESIAN_POINT('Ctrl Pts',(194.207402408913,1.74007361322188,125.147076402391));
#217404=CARTESIAN_POINT('Ctrl Pts',(194.214809755267,1.88928054317001,125.197351647384));
#217405=CARTESIAN_POINT('Ctrl Pts',(194.222211576942,2.03837618896044,125.247589395203));
#217406=CARTESIAN_POINT('Ctrl Pts',(194.229613398618,2.18558280757734,125.303817284624));
#217407=CARTESIAN_POINT('Ctrl Pts',(194.237015220293,2.33038800394414,125.365866127951));
#217408=CARTESIAN_POINT('Ctrl Pts',(194.244413134605,2.47511675877508,125.427882216177));
#217409=CARTESIAN_POINT('Ctrl Pts',(194.251811048916,2.61744627377012,125.495712991953));
#217410=CARTESIAN_POINT('Ctrl Pts',(194.259208963227,2.75688245248113,125.569140497485));
#217411=CARTESIAN_POINT('Ctrl Pts',(194.26660564814,2.89629545942845,125.642555800698));
#217412=CARTESIAN_POINT('Ctrl Pts',(194.274002333052,3.03281575440156,125.721565813977));
#217413=CARTESIAN_POINT('Ctrl Pts',(194.281399017964,3.16597214979834,125.805905765394));
#217414=CARTESIAN_POINT('Ctrl Pts',(194.2887953749,3.29912264090107,125.89024197709));
#217415=CARTESIAN_POINT('Ctrl Pts',(194.296191731835,3.42890921364481,125.979907457263));
#217416=CARTESIAN_POINT('Ctrl Pts',(194.30358808877,3.55488831789053,126.07459322267));
#217417=CARTESIAN_POINT('Ctrl Pts',(194.310985578107,3.68088670985897,126.169293484709));
#217418=CARTESIAN_POINT('Ctrl Pts',(194.318383067444,3.80307617420363,126.269015338105));
#217419=CARTESIAN_POINT('Ctrl Pts',(194.32578055678,3.92104512400985,126.373408609478));
#217420=CARTESIAN_POINT('Ctrl Pts',(194.333180639295,4.03905542764841,126.477838475751));
#217421=CARTESIAN_POINT('Ctrl Pts',(194.34058072181,4.15284199170322,126.586942773136));
#217422=CARTESIAN_POINT('Ctrl Pts',(194.347980804325,4.26202918068377,126.700333592131));
#217423=CARTESIAN_POINT('Ctrl Pts',(194.355389023992,4.37133643220337,126.813849095989));
#217424=CARTESIAN_POINT('Ctrl Pts',(194.362797243658,4.47603394942869,126.931660265503));
#217425=CARTESIAN_POINT('Ctrl Pts',(194.370205463325,4.57578511067753,127.053344597419));
#217426=CARTESIAN_POINT('Ctrl Pts',(194.377618242627,4.67559766710175,127.17510382401));
#217427=CARTESIAN_POINT('Ctrl Pts',(194.385031021929,4.77045757678608,127.300740665929));
#217428=CARTESIAN_POINT('Ctrl Pts',(194.392443801231,4.86007117030686,127.429803049224));
#217429=CARTESIAN_POINT('Ctrl Pts',(194.39986717226,4.94981280793254,127.559049842905));
#217430=CARTESIAN_POINT('Ctrl Pts',(194.407290543289,5.03429295787514,127.691731639473));
#217431=CARTESIAN_POINT('Ctrl Pts',(194.414713914317,5.11326315514323,127.827370448158));
#217432=CARTESIAN_POINT('Ctrl Pts',(194.418649963758,5.15513504859709,127.899289399128));
#217433=CARTESIAN_POINT('Ctrl Pts',(194.422586013199,5.19545868610213,127.972039303758));
#217434=CARTESIAN_POINT('Ctrl Pts',(194.426522062639,5.23420254088829,128.04554668338));
#217435=CARTESIAN_POINT('Ctrl Pts',(194.433945329045,5.30727224186316,128.184179307264));
#217436=CARTESIAN_POINT('Ctrl Pts',(194.44136859545,5.37494091137785,128.325926541199));
#217437=CARTESIAN_POINT('Ctrl Pts',(194.448791861856,5.4369314766717,128.470328338338));
#217438=CARTESIAN_POINT('Ctrl Pts',(194.456206354577,5.49884877426541,128.614559464546));
#217439=CARTESIAN_POINT('Ctrl Pts',(194.463620847298,5.55510118019554,128.761438569126));
#217440=CARTESIAN_POINT('Ctrl Pts',(194.471035340019,5.60545688611216,128.910480035154));
#217441=CARTESIAN_POINT('Ctrl Pts',(194.478442686372,5.6557640573036,129.059377849406));
#217442=CARTESIAN_POINT('Ctrl Pts',(194.485850032726,5.70018572444837,129.21043352466));
#217443=CARTESIAN_POINT('Ctrl Pts',(194.49325737908,5.73853772718516,129.363140538545));
#217444=CARTESIAN_POINT('Ctrl Pts',(194.500659200755,5.77686112555123,129.515733657777));
#217445=CARTESIAN_POINT('Ctrl Pts',(194.508061022431,5.80912378280913,129.669975302801));
#217446=CARTESIAN_POINT('Ctrl Pts',(194.515462844106,5.83519107930323,129.825342931045));
#217447=CARTESIAN_POINT('Ctrl Pts',(194.522860758417,5.86124461507446,129.980628541928));
#217448=CARTESIAN_POINT('Ctrl Pts',(194.530258672729,5.88110924179336,130.13703858504));
#217449=CARTESIAN_POINT('Ctrl Pts',(194.53765658704,5.8947012623256,130.294039551533));
#217450=CARTESIAN_POINT('Ctrl Pts',(194.545053271952,5.90829102411064,130.451014427314));
#217451=CARTESIAN_POINT('Ctrl Pts',(194.552449956865,5.91561021638582,130.608579660035));
#217452=CARTESIAN_POINT('Ctrl Pts',(194.559846641777,5.91662691086489,130.766195710526));
#217453=CARTESIAN_POINT('Ctrl Pts',(194.567242998712,5.91764356026267,130.923804772156));
#217454=CARTESIAN_POINT('Ctrl Pts',(194.574639355648,5.91235826511605,131.081464273787));
#217455=CARTESIAN_POINT('Ctrl Pts',(194.582035712583,5.90079123209493,131.238634031134));
#217456=CARTESIAN_POINT('Ctrl Pts',(194.58943320192,5.88922242813151,131.395827851571));
#217457=CARTESIAN_POINT('Ctrl Pts',(194.596830691256,5.87136999872203,131.552531406112));
#217458=CARTESIAN_POINT('Ctrl Pts',(194.604228180593,5.84730608186697,131.708209137763));
#217459=CARTESIAN_POINT('Ctrl Pts',(194.611628263108,5.82323372944323,131.863941442));
#217460=CARTESIAN_POINT('Ctrl Pts',(194.619028345623,5.79294561132196,132.0186468387));
#217461=CARTESIAN_POINT('Ctrl Pts',(194.626428428138,5.75656504659628,132.171799620522));
#217462=CARTESIAN_POINT('Ctrl Pts',(194.633836647804,5.72014447769965,132.325120809573));
#217463=CARTESIAN_POINT('Ctrl Pts',(194.641244867471,5.67761816964086,132.476885610823));
#217464=CARTESIAN_POINT('Ctrl Pts',(194.648653087137,5.62915963413416,132.626582441586));
#217465=CARTESIAN_POINT('Ctrl Pts',(194.656065866439,5.58067127320736,132.776371408251));
#217466=CARTESIAN_POINT('Ctrl Pts',(194.663478645741,5.52624353814764,132.924089518748));
#217467=CARTESIAN_POINT('Ctrl Pts',(194.670891425043,5.46609803607665,133.069245343661));
#217468=CARTESIAN_POINT('Ctrl Pts',(194.678314796072,5.4058665952918,133.214608574024));
#217469=CARTESIAN_POINT('Ctrl Pts',(194.685738167101,5.33990122668302,133.35740186875));
#217470=CARTESIAN_POINT('Ctrl Pts',(194.69316153813,5.26846977602395,133.49715782152));
#217471=CARTESIAN_POINT('Ctrl Pts',(194.697097587571,5.23059510690934,133.571259781079));
#217472=CARTESIAN_POINT('Ctrl Pts',(194.701033637011,5.19118446278821,133.644508299809));
#217473=CARTESIAN_POINT('Ctrl Pts',(194.704969686452,5.15028262235604,133.716837136331));
#217474=CARTESIAN_POINT('Ctrl Pts',(194.712392952858,5.07314302780579,133.853247064702));
#217475=CARTESIAN_POINT('Ctrl Pts',(194.719816219263,4.99046363417835,133.986796475152));
#217476=CARTESIAN_POINT('Ctrl Pts',(194.727239485669,4.90248172731818,134.117003591961));
#217477=CARTESIAN_POINT('Ctrl Pts',(194.73465397839,4.81460380776549,134.247056814772));
#217478=CARTESIAN_POINT('Ctrl Pts',(194.742068471111,4.7214360566969,134.373775300779));
#217479=CARTESIAN_POINT('Ctrl Pts',(194.749482963832,4.62326173930799,134.496701535243));
#217480=CARTESIAN_POINT('Ctrl Pts',(194.756890310185,4.52518204602216,134.619509288774));
#217481=CARTESIAN_POINT('Ctrl Pts',(194.764297656539,4.4221056244628,134.738531777645));
#217482=CARTESIAN_POINT('Ctrl Pts',(194.771705002893,4.31435908307288,134.853340274814));
#217483=CARTESIAN_POINT('Ctrl Pts',(194.779106824568,4.2066929031187,134.968063143474));
#217484=CARTESIAN_POINT('Ctrl Pts',(194.786508646244,4.0943637931164,135.078578007448));
#217485=CARTESIAN_POINT('Ctrl Pts',(194.793910467919,3.97773861771825,135.184489160384));
#217486=CARTESIAN_POINT('Ctrl Pts',(194.801308382231,3.86117500784292,135.290344403647));
#217487=CARTESIAN_POINT('Ctrl Pts',(194.808706296542,3.74032012477287,135.39160052553));
#217488=CARTESIAN_POINT('Ctrl Pts',(194.816104210853,3.61557758426522,135.487898734701));
#217489=CARTESIAN_POINT('Ctrl Pts',(194.823500895765,3.49085577370419,135.584180940857));
#217490=CARTESIAN_POINT('Ctrl Pts',(194.830897580678,3.36224788314285,135.675506641639));
#217491=CARTESIAN_POINT('Ctrl Pts',(194.83829426559,3.23019058414608,135.761557340775));
#217492=CARTESIAN_POINT('Ctrl Pts',(194.845690622525,3.09813914070806,135.847604224333));
#217493=CARTESIAN_POINT('Ctrl Pts',(194.853086979461,2.96263890570939,135.928376367518));
#217494=CARTESIAN_POINT('Ctrl Pts',(194.860483336396,2.82415527368646,136.003598787972));
#217495=CARTESIAN_POINT('Ctrl Pts',(194.867880825733,2.68565043946621,136.078832725171));
#217496=CARTESIAN_POINT('Ctrl Pts',(194.875278315069,2.54416162679036,136.148515069628));
#217497=CARTESIAN_POINT('Ctrl Pts',(194.882675804406,2.40017840727624,136.212417031449));
#217498=CARTESIAN_POINT('Ctrl Pts',(194.890075886921,2.25614471466828,136.276341394004));
#217499=CARTESIAN_POINT('Ctrl Pts',(194.897475969436,2.10961521526799,136.33448118823));
#217500=CARTESIAN_POINT('Ctrl Pts',(194.904876051951,1.96109885853,136.386656008315));
#217501=CARTESIAN_POINT('Ctrl Pts',(194.912284271617,1.81241919278925,136.438888199978));
#217502=CARTESIAN_POINT('Ctrl Pts',(194.919692491284,1.66174865902651,136.485142194737));
#217503=CARTESIAN_POINT('Ctrl Pts',(194.92710071095,1.50961145356359,136.525287449974));
#217504=CARTESIAN_POINT('Ctrl Pts',(194.934513490252,1.35738061018877,136.565457413946));
#217505=CARTESIAN_POINT('Ctrl Pts',(194.941926269555,1.20368165996157,136.599511065906));
#217506=CARTESIAN_POINT('Ctrl Pts',(194.949339048857,1.04904784043026,136.627369220598));
#217507=CARTESIAN_POINT('Ctrl Pts',(194.956762419885,0.894193072846361,
136.655267180328));
#217508=CARTESIAN_POINT('Ctrl Pts',(194.964185790914,0.738401136849904,
136.676951911201));
#217509=CARTESIAN_POINT('Ctrl Pts',(194.971609161943,0.582210051798615,
136.692396114919));
#217510=CARTESIAN_POINT('Ctrl Pts',(194.975545211384,0.499393790750225,
136.700585002308));
#217511=CARTESIAN_POINT('Ctrl Pts',(194.979481260825,0.416465321632257,
136.70702032481));
#217512=CARTESIAN_POINT('Ctrl Pts',(194.983417310265,0.333504579172153,
136.711703950924));
#217513=CARTESIAN_POINT('Ctrl Pts',(194.990840576671,0.177043208009956,
136.720537123605));
#217514=CARTESIAN_POINT('Ctrl Pts',(194.998263843076,0.0199940748712888,
136.723163326617));
#217515=CARTESIAN_POINT('Ctrl Pts',(195.005687109482,-0.137109229893286,
136.71952178372));
#217516=CARTESIAN_POINT('Ctrl Pts',(195.013101602203,-0.294026851598554,
136.715884544824));
#217517=CARTESIAN_POINT('Ctrl Pts',(195.020516094924,-0.450998147931574,
136.70599431416));
#217518=CARTESIAN_POINT('Ctrl Pts',(195.027930587645,-0.607485087027711,
136.689842112868));
#217519=CARTESIAN_POINT('Ctrl Pts',(195.035337933998,-0.763821198120527,
136.673705479675));
#217520=CARTESIAN_POINT('Ctrl Pts',(195.042745280352,-0.919673512534122,
136.651318929462));
#217521=CARTESIAN_POINT('Ctrl Pts',(195.050152626706,-1.07450479022457,
136.622725509723));
#217522=CARTESIAN_POINT('Ctrl Pts',(195.057554448381,-1.22922058890767,
136.594153416035));
#217523=CARTESIAN_POINT('Ctrl Pts',(195.064956270057,-1.38291650166136,
136.559383737918));
#217524=CARTESIAN_POINT('Ctrl Pts',(195.072358091732,-1.53506131021855,
136.518511240044));
#217525=CARTESIAN_POINT('Ctrl Pts',(195.079756006044,-1.68712580271452,
136.477660318445));
#217526=CARTESIAN_POINT('Ctrl Pts',(195.087153920355,-1.83764046212198,
136.430713089725));
#217527=CARTESIAN_POINT('Ctrl Pts',(195.094551834666,-1.98608526295548,
136.377815191775));
#217528=CARTESIAN_POINT('Ctrl Pts',(195.101948519579,-2.13450539495601,
136.324926084496));
#217529=CARTESIAN_POINT('Ctrl Pts',(195.109345204491,-2.28085599977257,
136.266088395828));
#217530=CARTESIAN_POINT('Ctrl Pts',(195.116741889403,-2.42463308582467,
136.201497354913));
#217531=CARTESIAN_POINT('Ctrl Pts',(195.124138246339,-2.56840379665031,
136.136909178033));
#217532=CARTESIAN_POINT('Ctrl Pts',(195.131534603274,-2.70960087509142,
136.066568309123));
#217533=CARTESIAN_POINT('Ctrl Pts',(195.138930960209,-2.84774141358831,
135.990717663107));
#217534=CARTESIAN_POINT('Ctrl Pts',(195.146328449546,-2.98590310175456,
135.914855404164));
#217535=CARTESIAN_POINT('Ctrl Pts',(195.153725938883,-3.1210069909607,135.833481868153));
#217536=CARTESIAN_POINT('Ctrl Pts',(195.161123428219,-3.25259596837197,
135.746885279015));
#217537=CARTESIAN_POINT('Ctrl Pts',(195.168523510734,-3.38423107409569,
135.660258333577));
#217538=CARTESIAN_POINT('Ctrl Pts',(195.175923593249,-3.51234850319129,
135.568404894722));
#217539=CARTESIAN_POINT('Ctrl Pts',(195.183323675764,-3.63652137552785,
135.471655642292));
#217540=CARTESIAN_POINT('Ctrl Pts',(195.190731895431,-3.76083078870214,
135.374800004113));
#217541=CARTESIAN_POINT('Ctrl Pts',(195.198140115097,-3.88118668830531,
135.273038030831));
#217542=CARTESIAN_POINT('Ctrl Pts',(195.205548334764,-3.99719590421933,
135.166740182184));
#217543=CARTESIAN_POINT('Ctrl Pts',(195.212961114066,-4.11327652186949,
135.060376908984));
#217544=CARTESIAN_POINT('Ctrl Pts',(195.220373893368,-4.2250048606152,134.949472459869));
#217545=CARTESIAN_POINT('Ctrl Pts',(195.22778667267,-4.33202607173832,134.834432661125));
#217546=CARTESIAN_POINT('Ctrl Pts',(195.235210043698,-4.43920019978721,
134.719228488122));
#217547=CARTESIAN_POINT('Ctrl Pts',(195.242633414727,-4.54165352484936,
134.599877446827));
#217548=CARTESIAN_POINT('Ctrl Pts',(195.250056785756,-4.63907226748901,
134.476817432767));
#217549=CARTESIAN_POINT('Ctrl Pts',(195.253992835197,-4.6907260223665,134.411568060529));
#217550=CARTESIAN_POINT('Ctrl Pts',(195.257928884637,-4.7409651046425,134.345276439808));
#217551=CARTESIAN_POINT('Ctrl Pts',(195.261864934078,-4.78974787966705,
134.278010831926));
#217552=CARTESIAN_POINT('Ctrl Pts',(195.269344497194,-4.88244840344199,
134.150187905093));
#217553=CARTESIAN_POINT('Ctrl Pts',(195.27682406031,-4.97016722581075,134.018460598548));
#217554=CARTESIAN_POINT('Ctrl Pts',(195.284303623426,-5.05256043017122,
133.883250622416));
#217555=CARTESIAN_POINT('Ctrl Pts',(195.291774119838,-5.13485375774175,
133.748204547404));
#217556=CARTESIAN_POINT('Ctrl Pts',(195.29924461625,-5.21183412944589,133.609684515291));
#217557=CARTESIAN_POINT('Ctrl Pts',(195.306715112662,-5.28319868593022,
133.468144056114));
#217558=CARTESIAN_POINT('Ctrl Pts',(195.314177953125,-5.35449010624771,
133.326748651109));
#217559=CARTESIAN_POINT('Ctrl Pts',(195.321640793587,-5.42017700590164,
133.182339305798));
#217560=CARTESIAN_POINT('Ctrl Pts',(195.329103634049,-5.48000059220959,
133.03539716408));
#217561=CARTESIAN_POINT('Ctrl Pts',(195.336560224284,-5.53977407546993,
132.888578088357));
#217562=CARTESIAN_POINT('Ctrl Pts',(195.344016814518,-5.59369388645601,
132.739230777314));
#217563=CARTESIAN_POINT('Ctrl Pts',(195.351473404753,-5.64154786489769,
132.587859496334));
#217564=CARTESIAN_POINT('Ctrl Pts',(195.358924751708,-5.68936819367592,
132.436594655673));
#217565=CARTESIAN_POINT('Ctrl Pts',(195.366376098664,-5.73113107811833,
132.28330902832));
#217566=CARTESIAN_POINT('Ctrl Pts',(195.373827445619,-5.76667310995969,
132.128525186405));
#217567=CARTESIAN_POINT('Ctrl Pts',(195.381275645374,-5.80220013002815,
131.97380672004));
#217568=CARTESIAN_POINT('Ctrl Pts',(195.388723845128,-5.83151144890194,
131.817591655312));
#217569=CARTESIAN_POINT('Ctrl Pts',(195.396172044882,-5.85449396429676,
131.660416097376));
#217570=CARTESIAN_POINT('Ctrl Pts',(195.403619442704,-5.87747400521164,
131.503257462208));
#217571=CARTESIAN_POINT('Ctrl Pts',(195.411066840526,-5.89412654082032,
131.345138900639));
#217572=CARTESIAN_POINT('Ctrl Pts',(195.418514238348,-5.90438986155658,
131.186605205818));
#217573=CARTESIAN_POINT('Ctrl Pts',(195.424551094831,-5.91270930356792,
131.058097882038));
#217574=CARTESIAN_POINT('Ctrl Pts',(195.430587951313,-5.91683153852153,
130.929318034017));
#217575=CARTESIAN_POINT('Ctrl Pts',(195.436624807795,-5.91674877781543,
130.800557629312));
#217576=CARTESIAN_POINT('',(197.186623444831,-5.92116344383671,130.801362336707));
#217577=CARTESIAN_POINT('Ctrl Pts',(195.436626945312,-5.90948723714756,
130.800516761409));
#217578=CARTESIAN_POINT('Ctrl Pts',(195.471188816171,-5.9137909198465,130.064246680543));
#217579=CARTESIAN_POINT('Ctrl Pts',(195.598566561638,-5.44429779229546,
127.356026198653));
#217580=CARTESIAN_POINT('Ctrl Pts',(195.818760181701,-1.38200268831043,
123.943775431166));
#217581=CARTESIAN_POINT('Ctrl Pts',(196.097207805517,5.0249984088633,125.933328743181));
#217582=CARTESIAN_POINT('Ctrl Pts',(196.375655429329,6.81427145311116,132.39912238462));
#217583=CARTESIAN_POINT('Ctrl Pts',(196.654103053143,2.34156192761705,137.399407870579));
#217584=CARTESIAN_POINT('Ctrl Pts',(196.924425368086,-4.08962105397609,
136.370105731155));
#217585=CARTESIAN_POINT('Ctrl Pts',(197.101931808425,-5.91344458449586,
132.593748677927));
#217586=CARTESIAN_POINT('Ctrl Pts',(197.18662237416,-5.92463101698242,130.801383223244));
#217587=CARTESIAN_POINT('',(198.936625519421,-5.91828595945227,130.809611426597));
#217588=CARTESIAN_POINT('Ctrl Pts',(197.186624807795,-5.91674922678536,
130.801335748166));
#217589=CARTESIAN_POINT('Ctrl Pts',(197.194749305453,-5.91666143946249,
130.629620706627));
#217590=CARTESIAN_POINT('Ctrl Pts',(197.20287380311,-5.90909912685711,130.458101858393));
#217591=CARTESIAN_POINT('Ctrl Pts',(197.210998300767,-5.89410901923282,
130.287244158827));
#217592=CARTESIAN_POINT('Ctrl Pts',(197.218421567172,-5.88041271860844,
130.131133310534));
#217593=CARTESIAN_POINT('Ctrl Pts',(197.225844833577,-5.86048931664855,
129.975330918972));
#217594=CARTESIAN_POINT('Ctrl Pts',(197.233268099982,-5.83435518767231,
129.820373774879));
#217595=CARTESIAN_POINT('Ctrl Pts',(197.240682592703,-5.80825194706619,
129.665599777262));
#217596=CARTESIAN_POINT('Ctrl Pts',(197.248097085424,-5.77595265235115,
129.511669403079));
#217597=CARTESIAN_POINT('Ctrl Pts',(197.255511578145,-5.73752557677412,
129.359116410395));
#217598=CARTESIAN_POINT('Ctrl Pts',(197.262918924498,-5.69913553865926,
129.206710454028));
#217599=CARTESIAN_POINT('Ctrl Pts',(197.270326270852,-5.65462956830657,
129.055679595785));
#217600=CARTESIAN_POINT('Ctrl Pts',(197.277733617205,-5.60412731398305,
128.906549348981));
#217601=CARTESIAN_POINT('Ctrl Pts',(197.285135438881,-5.55366272614622,
128.757530329141));
#217602=CARTESIAN_POINT('Ctrl Pts',(197.292537260556,-5.49721087842226,
128.610409450263));
#217603=CARTESIAN_POINT('Ctrl Pts',(197.299939082232,-5.43494173808804,
128.465698849356));
#217604=CARTESIAN_POINT('Ctrl Pts',(197.307336996543,-5.37270546914825,
128.321064640048));
#217605=CARTESIAN_POINT('Ctrl Pts',(197.314734910855,-5.3046581706263,128.178838516762));
#217606=CARTESIAN_POINT('Ctrl Pts',(197.322132825166,-5.23101855199436,
128.03951424368));
#217607=CARTESIAN_POINT('Ctrl Pts',(197.329529510078,-5.15739117093109,
127.900213123764));
#217608=CARTESIAN_POINT('Ctrl Pts',(197.336926194991,-5.07817348849507,
127.76381322667));
#217609=CARTESIAN_POINT('Ctrl Pts',(197.344322879903,-4.9936309933754,127.630785336515));
#217610=CARTESIAN_POINT('Ctrl Pts',(197.351719236839,-4.90909224695859,
127.497763344956));
#217611=CARTESIAN_POINT('Ctrl Pts',(197.359115593775,-4.81922935754628,
127.368113378099));
#217612=CARTESIAN_POINT('Ctrl Pts',(197.36651195071,-4.72435198303289,127.242278515352));
#217613=CARTESIAN_POINT('Ctrl Pts',(197.373909440047,-4.62946008255125,
127.116424386966));
#217614=CARTESIAN_POINT('Ctrl Pts',(197.381306929384,-4.52955239306734,
126.9943868238));
#217615=CARTESIAN_POINT('Ctrl Pts',(197.388704418721,-4.42497971392021,
126.876576879388));
#217616=CARTESIAN_POINT('Ctrl Pts',(197.396104501236,-4.32037037698219,
126.758725636883));
#217617=CARTESIAN_POINT('Ctrl Pts',(197.403504583751,-4.21109304215689,
126.645105242758));
#217618=CARTESIAN_POINT('Ctrl Pts',(197.410904666267,-4.09753619015153,
126.536090741738));
#217619=CARTESIAN_POINT('Ctrl Pts',(197.418312885934,-3.9838544707137,126.426956368068));
#217620=CARTESIAN_POINT('Ctrl Pts',(197.4257211056,-3.86588410582371,126.322438260625));
#217621=CARTESIAN_POINT('Ctrl Pts',(197.433129325267,-3.74404811053006,
126.222872397726));
#217622=CARTESIAN_POINT('Ctrl Pts',(197.440542104569,-3.62213712721409,
126.123245253698));
#217623=CARTESIAN_POINT('Ctrl Pts',(197.447954883872,-3.49635607014594,
126.028576651746));
#217624=CARTESIAN_POINT('Ctrl Pts',(197.455367663174,-3.36715745966806,
125.939159572974));
#217625=CARTESIAN_POINT('Ctrl Pts',(197.462791034203,-3.23777424415678,
125.849614730886));
#217626=CARTESIAN_POINT('Ctrl Pts',(197.470214405232,-3.10496403682583,
125.765336597878));
#217627=CARTESIAN_POINT('Ctrl Pts',(197.477637776261,-2.96920520601125,
125.686572911233));
#217628=CARTESIAN_POINT('Ctrl Pts',(197.481573825702,-2.89722261642787,
125.644810514667));
#217629=CARTESIAN_POINT('Ctrl Pts',(197.485509875143,-2.82441143032903,
125.604597636826));
#217630=CARTESIAN_POINT('Ctrl Pts',(197.489445924583,-2.75084517427645,
125.565965692624));
#217631=CARTESIAN_POINT('Ctrl Pts',(197.496869190989,-2.61210151128014,
125.493107051516));
#217632=CARTESIAN_POINT('Ctrl Pts',(197.504292457394,-2.47025146129094,
125.425654175521));
#217633=CARTESIAN_POINT('Ctrl Pts',(197.5117157238,-2.32575549227818,125.363883436965));
#217634=CARTESIAN_POINT('Ctrl Pts',(197.519130216521,-2.18143030550119,
125.302185706292));
#217635=CARTESIAN_POINT('Ctrl Pts',(197.526544709242,-2.03446576441921,
125.246156890495));
#217636=CARTESIAN_POINT('Ctrl Pts',(197.533959201963,-1.88534783816607,
125.19602805863));
#217637=CARTESIAN_POINT('Ctrl Pts',(197.541366548317,-1.73637363738422,
125.14594754282));
#217638=CARTESIAN_POINT('Ctrl Pts',(197.548773894671,-1.58525053483429,
125.101755808138));
#217639=CARTESIAN_POINT('Ctrl Pts',(197.556181241024,-1.432485332562,125.063636243892));
#217640=CARTESIAN_POINT('Ctrl Pts',(197.5635830627,-1.27983406834118,125.025545110655));
#217641=CARTESIAN_POINT('Ctrl Pts',(197.570984884375,-1.12554350365379,
124.993517220284));
#217642=CARTESIAN_POINT('Ctrl Pts',(197.57838670605,-0.970136385334234,
124.967686397057));
#217643=CARTESIAN_POINT('Ctrl Pts',(197.585784620362,-0.814811305222937,
124.941869209721));
#217644=CARTESIAN_POINT('Ctrl Pts',(197.593182534673,-0.658371212651233,
124.922242635465));
#217645=CARTESIAN_POINT('Ctrl Pts',(197.600580448984,-0.501349743220964,
124.908889559417));
#217646=CARTESIAN_POINT('Ctrl Pts',(197.607977133896,-0.3443543679101,124.895538702408));
#217647=CARTESIAN_POINT('Ctrl Pts',(197.615373818808,-0.186778179082625,
124.88845930607));
#217648=CARTESIAN_POINT('Ctrl Pts',(197.622770503721,-0.0291607638722707,
124.887682477566));
#217649=CARTESIAN_POINT('Ctrl Pts',(197.630166860656,0.128449662416806,
124.886905683508));
#217650=CARTESIAN_POINT('Ctrl Pts',(197.637563217591,0.286100938161007,
124.892430903457));
#217651=CARTESIAN_POINT('Ctrl Pts',(197.644959574526,0.443252910452061,
124.9042371087));
#217652=CARTESIAN_POINT('Ctrl Pts',(197.652357063863,0.600428943111264,
124.916045121502));
#217653=CARTESIAN_POINT('Ctrl Pts',(197.659754553199,0.757105147833064,
124.934136006373));
#217654=CARTESIAN_POINT('Ctrl Pts',(197.667152042536,0.912746078026357,
124.958436810369));
#217655=CARTESIAN_POINT('Ctrl Pts',(197.674552125051,1.06844156790636,124.982746132975));
#217656=CARTESIAN_POINT('Ctrl Pts',(197.681952207565,1.2231006920997,125.013269651301));
#217657=CARTESIAN_POINT('Ctrl Pts',(197.68935229008,1.37619793154745,125.049883246362));
#217658=CARTESIAN_POINT('Ctrl Pts',(197.696760509747,1.52946351714884,125.086537101834));
#217659=CARTESIAN_POINT('Ctrl Pts',(197.704168729413,1.68116342485591,125.12929432084));
#217660=CARTESIAN_POINT('Ctrl Pts',(197.711576949079,1.83078633663098,125.177980613327));
#217661=CARTESIAN_POINT('Ctrl Pts',(197.718989728381,1.98050133881175,125.226696871413));
#217662=CARTESIAN_POINT('Ctrl Pts',(197.726402507683,2.12813644850627,125.281349345265));
#217663=CARTESIAN_POINT('Ctrl Pts',(197.733815286985,2.27320057411559,125.341715680144));
#217664=CARTESIAN_POINT('Ctrl Pts',(197.741238658014,2.41847197415036,125.402168269274));
#217665=CARTESIAN_POINT('Ctrl Pts',(197.748662029042,2.56116471546263,125.468350868582));
#217666=CARTESIAN_POINT('Ctrl Pts',(197.756085400071,2.7008117998894,125.539994921295));
#217667=CARTESIAN_POINT('Ctrl Pts',(197.760021449512,2.77485603483877,125.577982317118));
#217668=CARTESIAN_POINT('Ctrl Pts',(197.763957498952,2.84804449245546,125.617504387378));
#217669=CARTESIAN_POINT('Ctrl Pts',(197.767893548393,2.92031099958208,125.658516252623));
#217670=CARTESIAN_POINT('Ctrl Pts',(197.775316814799,3.05660337666153,125.735863350536));
#217671=CARTESIAN_POINT('Ctrl Pts',(197.782740081204,3.19002680850025,125.818745887891));
#217672=CARTESIAN_POINT('Ctrl Pts',(197.790163347609,3.32009988104743,125.906925845936));
#217673=CARTESIAN_POINT('Ctrl Pts',(197.79757784033,3.4500192180248,125.995001582594));
#217674=CARTESIAN_POINT('Ctrl Pts',(197.804992333051,3.57659577183659,126.08836206974));
#217675=CARTESIAN_POINT('Ctrl Pts',(197.812406825772,3.69937245935516,126.186723346248));
#217676=CARTESIAN_POINT('Ctrl Pts',(197.819814172126,3.82203081007992,126.284989818454));
#217677=CARTESIAN_POINT('Ctrl Pts',(197.82722151848,3.94089629635784,126.38824725262));
#217678=CARTESIAN_POINT('Ctrl Pts',(197.834628864833,4.05554068868584,126.49616838823));
#217679=CARTESIAN_POINT('Ctrl Pts',(197.842030686509,4.17009957490073,126.604009032185));
#217680=CARTESIAN_POINT('Ctrl Pts',(197.849432508184,4.28044336511714,126.716506196922));
#217681=CARTESIAN_POINT('Ctrl Pts',(197.85683432986,4.38617691174633,126.833292416016));
#217682=CARTESIAN_POINT('Ctrl Pts',(197.864232244171,4.49185464245934,126.950016984573));
#217683=CARTESIAN_POINT('Ctrl Pts',(197.871630158482,4.59292672653128,127.071025822277));
#217684=CARTESIAN_POINT('Ctrl Pts',(197.879028072794,4.68903498727919,127.195914767817));
#217685=CARTESIAN_POINT('Ctrl Pts',(197.886424757706,4.78512727657764,127.32078295908));
#217686=CARTESIAN_POINT('Ctrl Pts',(197.893821442618,4.87625715228911,127.449529682885));
#217687=CARTESIAN_POINT('Ctrl Pts',(197.90121812753,4.96210678305087,127.581717783478));
#217688=CARTESIAN_POINT('Ctrl Pts',(197.908614484466,5.04795260715005,127.713900022711));
#217689=CARTESIAN_POINT('Ctrl Pts',(197.916010841401,5.12851844851035,127.849523022255));
#217690=CARTESIAN_POINT('Ctrl Pts',(197.923407198337,5.20353003334438,127.988120969634));
#217691=CARTESIAN_POINT('Ctrl Pts',(197.930804687674,5.27855310264355,128.126740136713));
#217692=CARTESIAN_POINT('Ctrl Pts',(197.93820217701,5.34802004452218,128.268334830214));
#217693=CARTESIAN_POINT('Ctrl Pts',(197.945599666347,5.41170281439631,128.412415130906));
#217694=CARTESIAN_POINT('Ctrl Pts',(197.952999748862,5.47540790816671,128.556545938723));
#217695=CARTESIAN_POINT('Ctrl Pts',(197.960399831377,5.5333246421133,128.703163747315));
#217696=CARTESIAN_POINT('Ctrl Pts',(197.967799913892,5.58527338516755,128.851759333269));
#217697=CARTESIAN_POINT('Ctrl Pts',(197.975208133559,5.63727925120526,129.000518315345));
#217698=CARTESIAN_POINT('Ctrl Pts',(197.982616353225,5.68330389749944,129.15125906534));
#217699=CARTESIAN_POINT('Ctrl Pts',(197.990024572892,5.72321757932056,129.303457188875));
#217700=CARTESIAN_POINT('Ctrl Pts',(197.997437352194,5.76315582734688,129.455748987816));
#217701=CARTESIAN_POINT('Ctrl Pts',(198.004850131496,5.79697553623499,129.609499583923));
#217702=CARTESIAN_POINT('Ctrl Pts',(198.012262910798,5.82459833231772,129.76417561976));
#217703=CARTESIAN_POINT('Ctrl Pts',(198.019686281827,5.85226059714686,129.91907266397));
#217704=CARTESIAN_POINT('Ctrl Pts',(198.027109652855,5.87370821410285,130.074897420031));
#217705=CARTESIAN_POINT('Ctrl Pts',(198.034533023884,5.88891470369336,130.231111827664));
#217706=CARTESIAN_POINT('Ctrl Pts',(198.038469073325,5.89697754934896,130.313940454904));
#217707=CARTESIAN_POINT('Ctrl Pts',(198.042405122766,5.90328666138535,130.396878621457));
#217708=CARTESIAN_POINT('Ctrl Pts',(198.046341172207,5.90784402994841,130.479846395531));
#217709=CARTESIAN_POINT('Ctrl Pts',(198.053764438612,5.91643908482775,130.636321028099));
#217710=CARTESIAN_POINT('Ctrl Pts',(198.061187705018,5.9188262827532,130.793373976012));
#217711=CARTESIAN_POINT('Ctrl Pts',(198.068610971423,5.91494565958679,130.950471557045));
#217712=CARTESIAN_POINT('Ctrl Pts',(198.076025464144,5.91106962299469,131.107383461784));
#217713=CARTESIAN_POINT('Ctrl Pts',(198.083439956865,5.90094052019157,131.264339525099));
#217714=CARTESIAN_POINT('Ctrl Pts',(198.090854449586,5.88455019112052,131.420801702085));
#217715=CARTESIAN_POINT('Ctrl Pts',(198.09826179594,5.86817565966571,131.577113074935));
#217716=CARTESIAN_POINT('Ctrl Pts',(198.105669142294,5.84555195468406,131.732931140355));
#217717=CARTESIAN_POINT('Ctrl Pts',(198.113076488647,5.81672294120831,131.887718724436));
#217718=CARTESIAN_POINT('Ctrl Pts',(198.120478310323,5.78791542949845,132.042390862097));
#217719=CARTESIAN_POINT('Ctrl Pts',(198.127880131998,5.75291189262878,132.196033683341));
#217720=CARTESIAN_POINT('Ctrl Pts',(198.135281953674,5.71180790358625,132.348116114732));
#217721=CARTESIAN_POINT('Ctrl Pts',(198.142679867985,5.67072561301959,132.500118262991));
#217722=CARTESIAN_POINT('Ctrl Pts',(198.150077782296,5.6235493809752,132.650561302415));
#217723=CARTESIAN_POINT('Ctrl Pts',(198.157475696608,5.57042563656271,132.798925429756));
#217724=CARTESIAN_POINT('Ctrl Pts',(198.16487238152,5.5173107203528,132.94726490167));
#217725=CARTESIAN_POINT('Ctrl Pts',(198.172269066432,5.45825037911139,133.093525796069));
#217726=CARTESIAN_POINT('Ctrl Pts',(198.179665751344,5.39344060874215,133.237204419061));
#217727=CARTESIAN_POINT('Ctrl Pts',(198.18706210828,5.32863371210605,133.380876671192));
#217728=CARTESIAN_POINT('Ctrl Pts',(198.194458465215,5.25807804673258,133.5219665393));
#217729=CARTESIAN_POINT('Ctrl Pts',(198.20185482215,5.18201726216687,133.659991486062));
#217730=CARTESIAN_POINT('Ctrl Pts',(198.209252311487,5.1059448325008,133.798037564794));
#217731=CARTESIAN_POINT('Ctrl Pts',(198.216649800824,5.02436578559861,133.933017460883));
#217732=CARTESIAN_POINT('Ctrl Pts',(198.22404729016,4.93756904071554,134.064474500649));
#217733=CARTESIAN_POINT('Ctrl Pts',(198.231447372675,4.85074186936809,134.195977622476));
#217734=CARTESIAN_POINT('Ctrl Pts',(198.23884745519,4.75869356396067,134.323955117915));
#217735=CARTESIAN_POINT('Ctrl Pts',(198.246247537705,4.66175545359166,134.447980610569));
#217736=CARTESIAN_POINT('Ctrl Pts',(198.253655757372,4.56471074980486,134.572142482001));
#217737=CARTESIAN_POINT('Ctrl Pts',(198.261063977038,4.4627657331708,134.692343377834));
#217738=CARTESIAN_POINT('Ctrl Pts',(198.268472196704,4.35629146133617,134.808190692181));
#217739=CARTESIAN_POINT('Ctrl Pts',(198.275884976006,4.24975165636372,134.924109308617));
#217740=CARTESIAN_POINT('Ctrl Pts',(198.283297755308,4.13867730416189,135.035668740291));
#217741=CARTESIAN_POINT('Ctrl Pts',(198.290710534611,4.0234747705666,135.142514756496));
#217742=CARTESIAN_POINT('Ctrl Pts',(198.298133905639,3.9081076301889,135.249513439299));
#217743=CARTESIAN_POINT('Ctrl Pts',(198.305557276668,3.7886008105804,135.351785013754));
#217744=CARTESIAN_POINT('Ctrl Pts',(198.312980647697,3.6653926842793,135.449016367192));
#217745=CARTESIAN_POINT('Ctrl Pts',(198.316916697138,3.60006477937584,135.500570763819));
#217746=CARTESIAN_POINT('Ctrl Pts',(198.320852746578,3.53369678008804,135.550708903358));
#217747=CARTESIAN_POINT('Ctrl Pts',(198.324788796019,3.4663570110182,135.599389255089));
#217748=CARTESIAN_POINT('Ctrl Pts',(198.332212062425,3.33935630815509,135.691198879192));
#217749=CARTESIAN_POINT('Ctrl Pts',(198.33963532883,3.2085135538949,135.778098250994));
#217750=CARTESIAN_POINT('Ctrl Pts',(198.347058595235,3.07424533812585,135.859748452689));
#217751=CARTESIAN_POINT('Ctrl Pts',(198.354473087956,2.94013581623739,135.941302150627));
#217752=CARTESIAN_POINT('Ctrl Pts',(198.361887580677,2.80260920746114,136.017618835655));
#217753=CARTESIAN_POINT('Ctrl Pts',(198.369302073398,2.66211377350456,136.088400816071));
#217754=CARTESIAN_POINT('Ctrl Pts',(198.376709419752,2.52175375433678,136.15911457415));
#217755=CARTESIAN_POINT('Ctrl Pts',(198.384116766106,2.37843093774423,136.22430408084));
#217756=CARTESIAN_POINT('Ctrl Pts',(198.39152411246,2.23262097347329,136.283715885415));
#217757=CARTESIAN_POINT('Ctrl Pts',(198.398925934135,2.08691975977482,136.343083378425));
#217758=CARTESIAN_POINT('Ctrl Pts',(198.406327755811,1.93873543618441,136.396681609322));
#217759=CARTESIAN_POINT('Ctrl Pts',(198.413729577486,1.7885664693587,136.444303928202));
#217760=CARTESIAN_POINT('Ctrl Pts',(198.421127491797,1.63847677556185,136.49190110763));
#217761=CARTESIAN_POINT('Ctrl Pts',(198.428525406109,1.48640487996303,136.533528545095));
#217762=CARTESIAN_POINT('Ctrl Pts',(198.43592332042,1.33286725626621,136.569028469201));
#217763=CARTESIAN_POINT('Ctrl Pts',(198.443320005332,1.17935514773689,136.604522493864));
#217764=CARTESIAN_POINT('Ctrl Pts',(198.450716690245,1.02437815788533,136.633890942145));
#217765=CARTESIAN_POINT('Ctrl Pts',(198.458113375157,0.868465999221073,
136.657026452098));
#217766=CARTESIAN_POINT('Ctrl Pts',(198.465509732092,0.712560753865369,
136.680160936198));
#217767=CARTESIAN_POINT('Ctrl Pts',(198.472906089028,0.555720791400502,
136.697062976703));
#217768=CARTESIAN_POINT('Ctrl Pts',(198.480302445963,0.398483782675044,
136.707676739666));
#217769=CARTESIAN_POINT('Ctrl Pts',(198.4876999353,0.241222700562017,136.718292127623));
#217770=CARTESIAN_POINT('Ctrl Pts',(198.495097424636,0.0835648236240816,
136.722617295928));
#217771=CARTESIAN_POINT('Ctrl Pts',(198.502494913973,-0.0739494677253907,
136.720648477257));
#217772=CARTESIAN_POINT('Ctrl Pts',(198.509894996488,-0.231518975465559,
136.718678968419));
#217773=CARTESIAN_POINT('Ctrl Pts',(198.517295079003,-0.388944424367331,
136.710411084445));
#217774=CARTESIAN_POINT('Ctrl Pts',(198.524695161518,-0.545688000420484,
136.695893115032));
#217775=CARTESIAN_POINT('Ctrl Pts',(198.532103381184,-0.702603932149111,
136.681359181619));
#217776=CARTESIAN_POINT('Ctrl Pts',(198.539511600851,-0.858836121715699,
136.660561472159));
#217777=CARTESIAN_POINT('Ctrl Pts',(198.546919820517,-1.01385369294746,
136.633599954889));
#217778=CARTESIAN_POINT('Ctrl Pts',(198.55433259982,-1.16896667490789,136.606621843255));
#217779=CARTESIAN_POINT('Ctrl Pts',(198.561745379122,-1.32286318481004,
136.573472442769));
#217780=CARTESIAN_POINT('Ctrl Pts',(198.569158158424,-1.47502554766598,
136.534302170168));
#217781=CARTESIAN_POINT('Ctrl Pts',(198.576581529452,-1.62740532724162,
136.495075929244));
#217782=CARTESIAN_POINT('Ctrl Pts',(198.584004900481,-1.77804565442718,
136.449811741413));
#217783=CARTESIAN_POINT('Ctrl Pts',(198.59142827151,-1.92644614760085,136.398709176862));
#217784=CARTESIAN_POINT('Ctrl Pts',(198.595364320951,-2.00513164990258,
136.371613370947));
#217785=CARTESIAN_POINT('Ctrl Pts',(198.599300370392,-2.083187811426,136.34287698262));
#217786=CARTESIAN_POINT('Ctrl Pts',(198.603236419832,-2.16054276008407,
136.312535046934));
#217787=CARTESIAN_POINT('Ctrl Pts',(198.610659686238,-2.30643177908773,
136.255311103171));
#217788=CARTESIAN_POINT('Ctrl Pts',(198.618082952643,-2.4502663863924,136.192200621447));
#217789=CARTESIAN_POINT('Ctrl Pts',(198.625506219049,-2.59153626383937,
136.12337089728));
#217790=CARTESIAN_POINT('Ctrl Pts',(198.63292071177,-2.73263917202303,136.054622524132));
#217791=CARTESIAN_POINT('Ctrl Pts',(198.640335204491,-2.87118305185535,
135.980168525608));
#217792=CARTESIAN_POINT('Ctrl Pts',(198.647749697212,-3.00667515047484,
135.900225127344));
#217793=CARTESIAN_POINT('Ctrl Pts',(198.655157043566,-3.14203665670858,
135.820358781537));
#217794=CARTESIAN_POINT('Ctrl Pts',(198.662564389919,-3.27435191817235,
135.735013757533));
#217795=CARTESIAN_POINT('Ctrl Pts',(198.669971736273,-3.40315059928627,
135.644453236626));
#217796=CARTESIAN_POINT('Ctrl Pts',(198.677373557949,-3.53185321748438,
135.553960259172));
#217797=CARTESIAN_POINT('Ctrl Pts',(198.684775379624,-3.65704417362253,
135.458259743947));
#217798=CARTESIAN_POINT('Ctrl Pts',(198.692177201299,-3.77828017388039,
135.357659365744));
#217799=CARTESIAN_POINT('Ctrl Pts',(198.699575115611,-3.89945217459736,
135.257112093699));
#217800=CARTESIAN_POINT('Ctrl Pts',(198.706973029922,-4.01667309082048,
135.151670347788));
#217801=CARTESIAN_POINT('Ctrl Pts',(198.714370944233,-4.12953101835425,
135.041683372673));
#217802=CARTESIAN_POINT('Ctrl Pts',(198.721767629146,-4.24237019094798,
134.931714675399));
#217803=CARTESIAN_POINT('Ctrl Pts',(198.729164314058,-4.35084754678297,
134.81720250832));
#217804=CARTESIAN_POINT('Ctrl Pts',(198.73656099897,-4.45458643666219,134.69853450182));
#217805=CARTESIAN_POINT('Ctrl Pts',(198.743957355906,-4.55832072665023,
134.579871757183));
#217806=CARTESIAN_POINT('Ctrl Pts',(198.751353712841,-4.65731672275938,
134.457053820572));
#217807=CARTESIAN_POINT('Ctrl Pts',(198.758750069776,-4.75123682608077,
134.330502870084));
#217808=CARTESIAN_POINT('Ctrl Pts',(198.766147559113,-4.84517130880985,
134.203932544323));
#217809=CARTESIAN_POINT('Ctrl Pts',(198.77354504845,-4.93402812889303,134.073628366469));
#217810=CARTESIAN_POINT('Ctrl Pts',(198.780942537786,-5.01751202795966,
133.940042937537));
#217811=CARTESIAN_POINT('Ctrl Pts',(198.788342620301,-5.10102519217775,
133.80641068044));
#217812=CARTESIAN_POINT('Ctrl Pts',(198.795742702816,-5.17916148769389,
133.669495198516));
#217813=CARTESIAN_POINT('Ctrl Pts',(198.803142785331,-5.25167084038773,
133.529775071685));
#217814=CARTESIAN_POINT('Ctrl Pts',(198.810551004998,-5.32425992456896,
133.389901308211));
#217815=CARTESIAN_POINT('Ctrl Pts',(198.817959224664,-5.39120953722308,
133.247217072428));
#217816=CARTESIAN_POINT('Ctrl Pts',(198.825367444331,-5.45231683291927,
133.102223040768));
#217817=CARTESIAN_POINT('Ctrl Pts',(198.832780223633,-5.51346173913636,
132.957139767702));
#217818=CARTESIAN_POINT('Ctrl Pts',(198.840193002935,-5.56875703240109,
132.809744214664));
#217819=CARTESIAN_POINT('Ctrl Pts',(198.847605782237,-5.61804944659764,
132.660553220203));
#217820=CARTESIAN_POINT('Ctrl Pts',(198.855029153265,-5.66741229210717,
132.511149054653));
#217821=CARTESIAN_POINT('Ctrl Pts',(198.862452524294,-5.71075502537524,
132.359944681874));
#217822=CARTESIAN_POINT('Ctrl Pts',(198.869875895323,-5.74797508196189,
132.207468959657));
#217823=CARTESIAN_POINT('Ctrl Pts',(198.873811944764,-5.76771004904698,
132.126622673133));
#217824=CARTESIAN_POINT('Ctrl Pts',(198.877747994205,-5.78572457362142,
132.045419093963));
#217825=CARTESIAN_POINT('Ctrl Pts',(198.881684043645,-5.80200928305024,
131.96393762747));
#217826=CARTESIAN_POINT('Ctrl Pts',(198.892415019576,-5.84640680080297,
131.741792131358));
#217827=CARTESIAN_POINT('Ctrl Pts',(198.903145995507,-5.87805736973165,
131.517021225439));
#217828=CARTESIAN_POINT('Ctrl Pts',(198.913876971438,-5.89671799543621,
131.290824845232));
#217829=CARTESIAN_POINT('Ctrl Pts',(198.921459583557,-5.90990377532492,
131.130992279687));
#217830=CARTESIAN_POINT('Ctrl Pts',(198.929042195676,-5.91660456247561,
130.970448251875));
#217831=CARTESIAN_POINT('Ctrl Pts',(198.936624807795,-5.91674765788855,
130.809625156515));
#217832=CARTESIAN_POINT('',(200.686624807795,-5.90698642445631,130.80494468951));
#217833=CARTESIAN_POINT('Ctrl Pts',(198.936625793059,-5.9188774747153,130.809606147102));
#217834=CARTESIAN_POINT('Ctrl Pts',(199.011127751193,-5.90425259497605,
129.228876773919));
#217835=CARTESIAN_POINT('Ctrl Pts',(199.178445583929,-4.43793552679426,
125.654919300417));
#217836=CARTESIAN_POINT('Ctrl Pts',(199.438579291272,1.60513008150291,123.992524011201));
#217837=CARTESIAN_POINT('Ctrl Pts',(199.717026915084,6.59860307470548,128.472837940681));
#217838=CARTESIAN_POINT('Ctrl Pts',(199.995474538897,5.52828220193623,135.095707309003));
#217839=CARTESIAN_POINT('Ctrl Pts',(200.27392216271,-0.622259942815148,
137.775038711833));
#217840=CARTESIAN_POINT('Ctrl Pts',(200.504305585676,-5.2380063121806,134.691886300211));
#217841=CARTESIAN_POINT('Ctrl Pts',(200.641873134038,-5.90782357734734,
131.759296891607));
#217842=CARTESIAN_POINT('Ctrl Pts',(200.686624807795,-5.90698642445631,
130.80494468951));
#217843=CARTESIAN_POINT('',(202.436624807795,-5.91672686803579,130.798894919773));
#217844=CARTESIAN_POINT('Ctrl Pts',(200.686624807795,-5.90698642445631,
130.80494468951));
#217845=CARTESIAN_POINT('Ctrl Pts',(200.734689008642,-5.90608730535493,
129.77995116259));
#217846=CARTESIAN_POINT('Ctrl Pts',(200.875569084094,-5.16390162333142,
126.774392662908));
#217847=CARTESIAN_POINT('Ctrl Pts',(201.109265034148,-0.373204209884669,
123.815921653964));
#217848=CARTESIAN_POINT('Ctrl Pts',(201.387712657962,5.67784563147399,126.712951384136));
#217849=CARTESIAN_POINT('Ctrl Pts',(201.666160281774,6.5112327157493,133.369786323417));
#217850=CARTESIAN_POINT('Ctrl Pts',(201.944607905587,1.36111502553663,137.669120366955));
#217851=CARTESIAN_POINT('Ctrl Pts',(202.201429414261,-4.54266270085758,
135.816111494225));
#217852=CARTESIAN_POINT('Ctrl Pts',(202.36543504833,-5.90274340491685,132.310756663458));
#217853=CARTESIAN_POINT('Ctrl Pts',(202.436624807795,-5.91672686803579,
130.798894919773));
#217854=CARTESIAN_POINT('',(204.186624807795,-5.92581928566479,130.806233519117));
#217855=CARTESIAN_POINT('Ctrl Pts',(202.436624807795,-5.91672686803579,
130.798894919773));
#217856=CARTESIAN_POINT('Ctrl Pts',(202.458250922934,-5.9209747821421,130.339619647749));
#217857=CARTESIAN_POINT('Ctrl Pts',(202.572692912681,-5.66197777958727,
127.913946320691));
#217858=CARTESIAN_POINT('Ctrl Pts',(202.779950777024,-2.32147802600033,
124.202217003606));
#217859=CARTESIAN_POINT('Ctrl Pts',(203.058398400839,4.2997548257633,125.28261551589));
#217860=CARTESIAN_POINT('Ctrl Pts',(203.336846024651,6.96972305013295,131.437228026285));
#217861=CARTESIAN_POINT('Ctrl Pts',(203.615293648464,3.23485627607878,137.010266301744));
#217862=CARTESIAN_POINT('Ctrl Pts',(203.893741272277,-3.4726853742618,136.880380435614));
#217863=CARTESIAN_POINT('Ctrl Pts',(204.084184992054,-5.87766124044895,
132.972676372107));
#217864=CARTESIAN_POINT('Ctrl Pts',(204.181812837227,-5.92623998325372,
130.908018473525));
#217865=CARTESIAN_POINT('Ctrl Pts',(204.186624807795,-5.92581928566479,
130.806233519117));
#217866=CARTESIAN_POINT('',(205.936623590202,-5.91340924895264,130.808944439334));
#217867=CARTESIAN_POINT('Ctrl Pts',(204.186624807795,-5.92581928566479,
130.806233519117));
#217868=CARTESIAN_POINT('Ctrl Pts',(204.274628711831,-5.91812534204668,
128.944735566654));
#217869=CARTESIAN_POINT('Ctrl Pts',(204.455448490471,-3.96770241261772,
125.106068119418));
#217870=CARTESIAN_POINT('Ctrl Pts',(204.729084143717,2.57533168687046,124.297039558175));
#217871=CARTESIAN_POINT('Ctrl Pts',(205.007531767529,6.86682325353852,129.453694210665));
#217872=CARTESIAN_POINT('Ctrl Pts',(205.285979391342,4.84803947518153,135.851545143624));
#217873=CARTESIAN_POINT('Ctrl Pts',(205.564427015155,-1.62585529160082,
137.611280375001));
#217874=CARTESIAN_POINT('Ctrl Pts',(205.781308123836,-5.50460122239126,
134.109769780245));
#217875=CARTESIAN_POINT('Ctrl Pts',(205.905373357914,-5.91576144076024,
131.474232650613));
#217876=CARTESIAN_POINT('Ctrl Pts',(205.936622717388,-5.911015738934,130.80896117583));
#217877=CARTESIAN_POINT('',(207.097234316256,3.07028764517384,135.860950196139));
#217878=CARTESIAN_POINT('Ctrl Pts',(205.936624807795,-5.91674824245351,
130.808921091594));
#217879=CARTESIAN_POINT('Ctrl Pts',(205.944320535086,-5.91687464410253,
130.644927890423));
#217880=CARTESIAN_POINT('Ctrl Pts',(205.952016262377,-5.91017796225583,
130.480857837863));
#217881=CARTESIAN_POINT('Ctrl Pts',(205.959711989668,-5.89667042808694,
130.31732014181));
#217882=CARTESIAN_POINT('Ctrl Pts',(205.967107144318,-5.8836904587688,130.160169750732));
#217883=CARTESIAN_POINT('Ctrl Pts',(205.974502298968,-5.86442165241146,
130.003511317041));
#217884=CARTESIAN_POINT('Ctrl Pts',(205.981897453618,-5.83892794642443,
129.847882181341));
#217885=CARTESIAN_POINT('Ctrl Pts',(205.989293079306,-5.81343261660182,
129.692243132757));
#217886=CARTESIAN_POINT('Ctrl Pts',(205.996688704995,-5.78171165733105,
129.53763388078));
#217887=CARTESIAN_POINT('Ctrl Pts',(206.004084330683,-5.74388042102671,
129.384583074623));
#217888=CARTESIAN_POINT('Ctrl Pts',(206.011481882822,-5.70603933025007,
129.231492401015));
#217889=CARTESIAN_POINT('Ctrl Pts',(206.01887943496,-5.66208488256809,129.079961343446));
#217890=CARTESIAN_POINT('Ctrl Pts',(206.026276987099,-5.61218269697228,
128.930504716408));
#217891=CARTESIAN_POINT('Ctrl Pts',(206.033677921977,-5.56225769219368,
128.780979746109));
#217892=CARTESIAN_POINT('Ctrl Pts',(206.041078856855,-5.50637965184727,
128.633531448377));
#217893=CARTESIAN_POINT('Ctrl Pts',(206.048479791733,-5.44476278582211,
128.488655807227));
#217894=CARTESIAN_POINT('Ctrl Pts',(206.055889603669,-5.38307201339005,
128.343606394855));
#217895=CARTESIAN_POINT('Ctrl Pts',(206.063299415605,-5.31562881696656,
128.201136143459));
#217896=CARTESIAN_POINT('Ctrl Pts',(206.070709227541,-5.24269425134762,
128.06171817835));
#217897=CARTESIAN_POINT('Ctrl Pts',(206.078124284764,-5.16970805651977,
127.922201521501));
#217898=CARTESIAN_POINT('Ctrl Pts',(206.085539341988,-5.09122293266157,
127.785741777807));
#217899=CARTESIAN_POINT('Ctrl Pts',(206.092954399211,-5.00754363174057,
127.652783656945));
#217900=CARTESIAN_POINT('Ctrl Pts',(206.100380033849,-4.92374496414771,
127.519635874265));
#217901=CARTESIAN_POINT('Ctrl Pts',(206.107805668488,-4.83473753693092,
127.389999992524));
#217902=CARTESIAN_POINT('Ctrl Pts',(206.115231303126,-4.74086717656672,
127.264288728938));
#217903=CARTESIAN_POINT('Ctrl Pts',(206.117261623011,-4.71520110645441,
127.229916706794));
#217904=CARTESIAN_POINT('Ctrl Pts',(206.119291942896,-4.68917170648531,
127.195837875561));
#217905=CARTESIAN_POINT('Ctrl Pts',(206.121322262781,-4.66278652276695,
127.162060189869));
#217906=CARTESIAN_POINT('Ctrl Pts',(206.128745542087,-4.56631670550191,
127.038561820438));
#217907=CARTESIAN_POINT('Ctrl Pts',(206.136168821393,-4.46479117026267,
126.918712002184));
#217908=CARTESIAN_POINT('Ctrl Pts',(206.1435921007,-4.35851586193957,126.802952110088));
#217909=CARTESIAN_POINT('Ctrl Pts',(206.151006606373,-4.25236616125308,
126.687329035533));
#217910=CARTESIAN_POINT('Ctrl Pts',(206.158421112046,-4.14147811176257,
126.575786537499));
#217911=CARTESIAN_POINT('Ctrl Pts',(206.165835617719,-4.02619954292322,
126.4687351952));
#217912=CARTESIAN_POINT('Ctrl Pts',(206.173242977064,-3.9110320831151,126.361787032278));
#217913=CARTESIAN_POINT('Ctrl Pts',(206.180650336408,-3.79148280018012,
126.259321659787));
#217914=CARTESIAN_POINT('Ctrl Pts',(206.188057695753,-3.66793813141363,
126.161714774232));
#217915=CARTESIAN_POINT('Ctrl Pts',(206.195459530445,-3.54448560632645,
126.064180687105));
#217916=CARTESIAN_POINT('Ctrl Pts',(206.202861365137,-3.41704392042245,
125.971498102217));
#217917=CARTESIAN_POINT('Ctrl Pts',(206.210263199829,-3.28603443959317,
125.884004103622));
#217918=CARTESIAN_POINT('Ctrl Pts',(206.217661127171,-3.15509411728722,
125.796556292186));
#217919=CARTESIAN_POINT('Ctrl Pts',(206.225059054513,-3.02059006058692,
125.714291818989));
#217920=CARTESIAN_POINT('Ctrl Pts',(206.232456981854,-2.88297452136991,
125.637505822661));
#217921=CARTESIAN_POINT('Ctrl Pts',(206.239853679775,-2.74538185171612,
125.560732586972));
#217922=CARTESIAN_POINT('Ctrl Pts',(206.247250377697,-2.60467905146201,
125.489436202917));
#217923=CARTESIAN_POINT('Ctrl Pts',(206.254647075618,-2.4613451038374,125.423867067499));
#217924=CARTESIAN_POINT('Ctrl Pts',(206.262043445548,-2.3180175120597,125.358300839608));
#217925=CARTESIAN_POINT('Ctrl Pts',(206.269439815478,-2.1720593443594,125.298461510681));
#217926=CARTESIAN_POINT('Ctrl Pts',(206.276836185407,-2.02397155401354,
125.244552193614));
#217927=CARTESIAN_POINT('Ctrl Pts',(206.284233687713,-1.87586109160203,
125.190634623095));
#217928=CARTESIAN_POINT('Ctrl Pts',(206.291631190018,-1.72562070814953,
125.142648999845));
#217929=CARTESIAN_POINT('Ctrl Pts',(206.299028692324,-1.57376843488975,
125.100749176045));
#217930=CARTESIAN_POINT('Ctrl Pts',(206.306428787771,-1.42186293089913,
125.058834664561));
#217931=CARTESIAN_POINT('Ctrl Pts',(206.313828883218,-1.26834477174244,
125.023010299208));
#217932=CARTESIAN_POINT('Ctrl Pts',(206.321228978665,-1.1137439959854,124.993379213887));
#217933=CARTESIAN_POINT('Ctrl Pts',(206.328637211142,-0.958973223613178,
124.963715546683));
#217934=CARTESIAN_POINT('Ctrl Pts',(206.336045443619,-0.803117824125187,
124.940258829909));
#217935=CARTESIAN_POINT('Ctrl Pts',(206.343453676096,-0.646715539100822,
124.923060627429));
#217936=CARTESIAN_POINT('Ctrl Pts',(206.35086646816,-0.490216992290331,
124.905851839875));
#217937=CARTESIAN_POINT('Ctrl Pts',(206.358279260223,-0.333171260766503,
124.894909268023));
#217938=CARTESIAN_POINT('Ctrl Pts',(206.365692052287,-0.176117430763197,
124.890232345954));
#217939=CARTESIAN_POINT('Ctrl Pts',(206.373115435889,-0.0188391992448544,
124.885548741409));
#217940=CARTESIAN_POINT('Ctrl Pts',(206.380538819491,0.13844678157505,124.887148662973));
#217941=CARTESIAN_POINT('Ctrl Pts',(206.387962203094,0.295204371712296,
124.894979521256));
#217942=CARTESIAN_POINT('Ctrl Pts',(206.391898097594,0.378317594721756,
124.899131459738));
#217943=CARTESIAN_POINT('Ctrl Pts',(206.395833992093,0.461282402246363,
124.905034131635));
#217944=CARTESIAN_POINT('Ctrl Pts',(206.399769886593,0.544020024813092,
124.912673866295));
#217945=CARTESIAN_POINT('Ctrl Pts',(206.407193124759,0.700066147897168,
124.927082679821));
#217946=CARTESIAN_POINT('Ctrl Pts',(206.414616362924,0.855775400938864,
124.947717077111));
#217947=CARTESIAN_POINT('Ctrl Pts',(206.42203960109,1.0106110768226,124.974558235503));
#217948=CARTESIAN_POINT('Ctrl Pts',(206.429454065568,1.1652637490334,125.001367669744));
#217949=CARTESIAN_POINT('Ctrl Pts',(206.436868530046,1.31904453505951,125.034369199787));
#217950=CARTESIAN_POINT('Ctrl Pts',(206.444282994524,1.47141999714576,125.07349211842));
#217951=CARTESIAN_POINT('Ctrl Pts',(206.451690312658,1.62364859393998,125.11257732889));
#217952=CARTESIAN_POINT('Ctrl Pts',(206.459097630792,1.77447420420068,125.157772089943));
#217953=CARTESIAN_POINT('Ctrl Pts',(206.466504948926,1.92337186920565,125.208954357494));
#217954=CARTESIAN_POINT('Ctrl Pts',(206.47390674243,2.07215848127999,125.260098451574));
#217955=CARTESIAN_POINT('Ctrl Pts',(206.481308535935,2.21901965969763,125.317221039542));
#217956=CARTESIAN_POINT('Ctrl Pts',(206.48871032944,2.36344405149433,125.380149819859));
#217957=CARTESIAN_POINT('Ctrl Pts',(206.496108215656,2.50779220395472,125.443045381076));
#217958=CARTESIAN_POINT('Ctrl Pts',(206.503506101871,2.64970579024399,125.511740881817));
#217959=CARTESIAN_POINT('Ctrl Pts',(206.510903988087,2.78869205246822,125.586015362698));
#217960=CARTESIAN_POINT('Ctrl Pts',(206.518300645105,2.92765522138042,125.660277502477));
#217961=CARTESIAN_POINT('Ctrl Pts',(206.525697302122,3.06369170265306,125.740116606851));
#217962=CARTESIAN_POINT('Ctrl Pts',(206.533093959139,3.19633193171053,125.825265042582));
#217963=CARTESIAN_POINT('Ctrl Pts',(206.540490288307,3.32896628161558,125.910409704189));
#217964=CARTESIAN_POINT('Ctrl Pts',(206.547886617474,3.45820436447894,126.000863027573));
#217965=CARTESIAN_POINT('Ctrl Pts',(206.555282946642,3.58360452178626,126.096313337224));
#217966=CARTESIAN_POINT('Ctrl Pts',(206.562680408361,3.70902388080001,126.191778262557));
#217967=CARTESIAN_POINT('Ctrl Pts',(206.57007787008,3.83060384705553,126.292241471571));
#217968=CARTESIAN_POINT('Ctrl Pts',(206.577475331799,3.94793497542389,126.397350293965));
#217969=CARTESIAN_POINT('Ctrl Pts',(206.584875386871,4.06530723695059,126.502495964703));
#217970=CARTESIAN_POINT('Ctrl Pts',(206.592275441942,4.17842741707443,126.612290242479));
#217971=CARTESIAN_POINT('Ctrl Pts',(206.599675497014,4.28692225118017,126.726342940454));
#217972=CARTESIAN_POINT('Ctrl Pts',(206.607083689639,4.39553639284793,126.840521057759));
#217973=CARTESIAN_POINT('Ctrl Pts',(206.614491882264,4.49951477334651,126.958966676524));
#217974=CARTESIAN_POINT('Ctrl Pts',(206.621900074889,4.59852335176967,127.081255254334));
#217975=CARTESIAN_POINT('Ctrl Pts',(206.629312827337,4.69759287104336,127.203619102085));
#217976=CARTESIAN_POINT('Ctrl Pts',(206.636725579785,4.79168627026316,127.329830323613));
#217977=CARTESIAN_POINT('Ctrl Pts',(206.644138332232,4.88051264007905,127.459435067942));
#217978=CARTESIAN_POINT('Ctrl Pts',(206.651561676931,4.96946593591552,127.589225007439));
#217979=CARTESIAN_POINT('Ctrl Pts',(206.658985021629,5.05313697283413,127.722417839174));
#217980=CARTESIAN_POINT('Ctrl Pts',(206.666408366327,5.13128020290801,127.85853407112));
#217981=CARTESIAN_POINT('Ctrl Pts',(206.670344747687,5.17271725948344,127.930712505499));
#217982=CARTESIAN_POINT('Ctrl Pts',(206.674281129047,5.21260076983565,128.003712593246));
#217983=CARTESIAN_POINT('Ctrl Pts',(206.678217510406,5.25089964747057,128.077460646043));
#217984=CARTESIAN_POINT('Ctrl Pts',(206.685640788461,5.32312415823055,128.21653566238));
#217985=CARTESIAN_POINT('Ctrl Pts',(206.693064066516,5.38992876580883,128.358692359875));
#217986=CARTESIAN_POINT('Ctrl Pts',(206.70048734457,5.45103920233567,128.503469012753));
#217987=CARTESIAN_POINT('Ctrl Pts',(206.707901848764,5.51207741006405,128.648074548482));
#217988=CARTESIAN_POINT('Ctrl Pts',(206.715316352958,5.56743469941679,128.795293535183));
#217989=CARTESIAN_POINT('Ctrl Pts',(206.722730857152,5.6168822217327,128.944638952993));
#217990=CARTESIAN_POINT('Ctrl Pts',(206.730138214794,5.66628208350716,129.093840422569));
#217991=CARTESIAN_POINT('Ctrl Pts',(206.737545572437,5.70978340170174,129.245163890935));
#217992=CARTESIAN_POINT('Ctrl Pts',(206.744952930079,5.7472051019998,129.398101723177));
#217993=CARTESIAN_POINT('Ctrl Pts',(206.752354762849,5.78459889084891,129.550925484801));
#217994=CARTESIAN_POINT('Ctrl Pts',(206.75975659562,5.81592200238151,129.705360851746));
#217995=CARTESIAN_POINT('Ctrl Pts',(206.767158428391,5.84104299956971,129.860884470715));
#217996=CARTESIAN_POINT('Ctrl Pts',(206.774556353595,5.86615073491423,130.016325985859));
#217997=CARTESIAN_POINT('Ctrl Pts',(206.7819542788,5.88506281728999,130.172854241276));
#217998=CARTESIAN_POINT('Ctrl Pts',(206.789352204005,5.89769879798622,130.329935227508));
#217999=CARTESIAN_POINT('Ctrl Pts',(206.796748899477,5.91033267824491,130.486990102683));
#218000=CARTESIAN_POINT('Ctrl Pts',(206.804145594949,5.9166924974782,130.644597154589));
#218001=CARTESIAN_POINT('Ctrl Pts',(206.811542290421,5.91674961156378,130.802216658633));
#218002=CARTESIAN_POINT('Ctrl Pts',(206.818938657709,5.91680672311526,130.959829169251));
#218003=CARTESIAN_POINT('Ctrl Pts',(206.826335024997,5.91056168541304,131.117453757611));
#218004=CARTESIAN_POINT('Ctrl Pts',(206.833731392284,5.89803799224837,131.274550371277));
#218005=CARTESIAN_POINT('Ctrl Pts',(206.841128891758,5.88551238204215,131.431671032222));
#218006=CARTESIAN_POINT('Ctrl Pts',(206.848526391231,5.86670623237485,131.588263185411));
#218007=CARTESIAN_POINT('Ctrl Pts',(206.855923890704,5.84169493924775,131.743791721622));
#218008=CARTESIAN_POINT('Ctrl Pts',(206.863323983132,5.81667487921999,131.899374773335));
#218009=CARTESIAN_POINT('Ctrl Pts',(206.870724075559,5.78544540453156,132.053893097464));
#218010=CARTESIAN_POINT('Ctrl Pts',(206.878124167987,5.74813303139562,132.206821745683));
#218011=CARTESIAN_POINT('Ctrl Pts',(206.885532397178,5.71077963148349,132.359918546418));
#218012=CARTESIAN_POINT('Ctrl Pts',(206.892940626368,5.66733006439983,132.511421817639));
#218013=CARTESIAN_POINT('Ctrl Pts',(206.900348855559,5.61796095209888,132.660821040843));
#218014=CARTESIAN_POINT('Ctrl Pts',(206.907761644179,5.56856145534191,132.810312212512));
#218015=CARTESIAN_POINT('Ctrl Pts',(206.9151744328,5.5132352846973,132.957696407148));
#218016=CARTESIAN_POINT('Ctrl Pts',(206.922587221421,5.45220703402161,133.102483551759));
#218017=CARTESIAN_POINT('Ctrl Pts',(206.930010601368,5.3910915867254,133.247477566952));
#218018=CARTESIAN_POINT('Ctrl Pts',(206.937433981315,5.32425794604157,133.389866784108));
#218019=CARTESIAN_POINT('Ctrl Pts',(206.944857361262,5.2519767974538,133.52918543423));
#218020=CARTESIAN_POINT('Ctrl Pts',(206.948793285581,5.21365286245629,133.60305308846));
#218021=CARTESIAN_POINT('Ctrl Pts',(206.9527292099,5.17379827248436,133.676058022512));
#218022=CARTESIAN_POINT('Ctrl Pts',(206.956665134219,5.13245820404137,133.748134275011));
#218023=CARTESIAN_POINT('Ctrl Pts',(206.964088434769,5.05448928799419,133.884072784351));
#218024=CARTESIAN_POINT('Ctrl Pts',(206.97151173532,4.9709980519811,134.01711704531));
#218025=CARTESIAN_POINT('Ctrl Pts',(206.97893503587,4.88222471713909,134.146786738493));
#218026=CARTESIAN_POINT('Ctrl Pts',(206.986349890745,4.79355238193565,134.27630890323));
#218027=CARTESIAN_POINT('Ctrl Pts',(206.993764745621,4.6996101168209,134.40246383611));
#218028=CARTESIAN_POINT('Ctrl Pts',(207.001179600497,4.60068401122566,134.524795698488));
#218029=CARTESIAN_POINT('Ctrl Pts',(207.008587484203,4.50185091226226,134.647012549015));
#218030=CARTESIAN_POINT('Ctrl Pts',(207.015995367909,4.39804353314303,134.76541319544));
#218031=CARTESIAN_POINT('Ctrl Pts',(207.023403251615,4.28959116052852,134.879570825398));
#218032=CARTESIAN_POINT('Ctrl Pts',(207.030804839437,4.18123096047179,134.993631433958));
#218033=CARTESIAN_POINT('Ctrl Pts',(207.038206427259,4.06823388760403,135.103455940601));
#218034=CARTESIAN_POINT('Ctrl Pts',(207.04560801508,3.95096917488711,135.208650928342));
#218035=CARTESIAN_POINT('Ctrl Pts',(207.053005982973,3.83376181337625,135.313794467873));
#218036=CARTESIAN_POINT('Ctrl Pts',(207.060403950865,3.71229124444,135.414312747539));
#218037=CARTESIAN_POINT('Ctrl Pts',(207.067801918757,3.58696326793364,135.509849442013));
#218038=CARTESIAN_POINT('Ctrl Pts',(207.075197872091,3.46166941979266,135.605360120658));
#218039=CARTESIAN_POINT('Ctrl Pts',(207.082593825425,3.33252055199012,135.695891689038));
#218040=CARTESIAN_POINT('Ctrl Pts',(207.089989778758,3.19995513205736,135.781128415577));
#218041=CARTESIAN_POINT('Ctrl Pts',(207.092357450587,3.15751686939226,135.808415309787));
#218042=CARTESIAN_POINT('Ctrl Pts',(207.094725122416,3.11472870081105,135.835159892579));
#218043=CARTESIAN_POINT('Ctrl Pts',(207.097092794244,3.07160564976242,135.861352736884));
#218044=CARTESIAN_POINT('',(207.496354727754,-4.58101859761927,134.548389190118));
#218045=CARTESIAN_POINT('Ctrl Pts',(207.491512994556,-4.5779532771514,134.556042095633));
#218046=CARTESIAN_POINT('Ctrl Pts',(207.421356448526,-4.23683712701248,
134.83229957677));
#218047=CARTESIAN_POINT('Ctrl Pts',(207.352125680575,-3.86351417701888,
135.072882748138));
#218048=CARTESIAN_POINT('Ctrl Pts',(207.181195423578,-2.80904512107275,
135.629548817307));
#218049=CARTESIAN_POINT('Ctrl Pts',(207.088686747424,-2.07976512179529,
135.888075083137));
#218050=CARTESIAN_POINT('Ctrl Pts',(207.01614411327,-1.16577810051545,136.0860323564));
#218051=CARTESIAN_POINT('Ctrl Pts',(207.004225116839,-0.992744253302746,
136.118115831311));
#218052=CARTESIAN_POINT('Ctrl Pts',(206.992042736604,-0.781551616182621,
136.150680383293));
#218053=CARTESIAN_POINT('Ctrl Pts',(206.989976350538,-0.744182570385334,
136.156193421598));
#218054=CARTESIAN_POINT('Ctrl Pts',(206.987814094324,-0.703290708056184,
136.161952974892));
#218055=CARTESIAN_POINT('Ctrl Pts',(206.987630613907,-0.699805954358256,
136.162441630612));
#218056=CARTESIAN_POINT('Ctrl Pts',(206.987412352986,-0.695642812310952,
136.163022825853));
#218057=CARTESIAN_POINT('Ctrl Pts',(206.987376833818,-0.694964747275408,
136.163117405068));
#218058=CARTESIAN_POINT('Ctrl Pts',(206.987297040828,-0.693440213561303,
136.163329868685));
#218059=CARTESIAN_POINT('Ctrl Pts',(206.987252783207,-0.692593737269296,
136.163447708353));
#218060=CARTESIAN_POINT('Ctrl Pts',(206.9871907909,-0.691406822344562,136.163612761929));
#218061=CARTESIAN_POINT('Ctrl Pts',(206.987173018248,-0.691066400707796,
136.163660080629));
#218062=CARTESIAN_POINT('Ctrl Pts',(206.987143756372,-0.690505675199503,
136.163737987573));
#218063=CARTESIAN_POINT('Ctrl Pts',(206.987132262873,-0.690285372904867,
136.163768587615));
#218064=CARTESIAN_POINT('Ctrl Pts',(206.987110033778,-0.689859179030206,
136.163827769298));
#218065=CARTESIAN_POINT('Ctrl Pts',(206.987099297795,-0.689653287658265,
136.163856352005));
#218066=CARTESIAN_POINT('Ctrl Pts',(206.987074311334,-0.689173982563819,
136.163922873553));
#218067=CARTESIAN_POINT('Ctrl Pts',(206.987060062896,-0.688900567806784,
136.163960806763));
#218068=CARTESIAN_POINT('Ctrl Pts',(206.987015178065,-0.688038975675799,
136.164080300919));
#218069=CARTESIAN_POINT('Ctrl Pts',(206.986984558832,-0.687450790881196,
136.164161814515));
#218070=CARTESIAN_POINT('Ctrl Pts',(206.986555882125,-0.6792100354052,136.165302995029));
#218071=CARTESIAN_POINT('Ctrl Pts',(206.986161508294,-0.671555860542454,
136.16635249923));
#218072=CARTESIAN_POINT('Ctrl Pts',(206.980492339162,-0.560455784136554,
136.181434286989));
#218073=CARTESIAN_POINT('Ctrl Pts',(206.975892611292,-0.456712139527467,
136.193609075703));
#218074=CARTESIAN_POINT('Ctrl Pts',(206.962946640849,-0.110636466825927,
136.227783756113));
#218075=CARTESIAN_POINT('Ctrl Pts',(206.957730504988,0.133311986351349,
136.241404694132));
#218076=CARTESIAN_POINT('Ctrl Pts',(206.955350122412,0.720758476191309,
136.247635367825));
#218077=CARTESIAN_POINT('Ctrl Pts',(206.962101132817,1.06313123841359,136.230086185341));
#218078=CARTESIAN_POINT('Ctrl Pts',(206.998981742942,1.96417607662476,136.132510665149));
#218079=CARTESIAN_POINT('Ctrl Pts',(207.041779761648,2.52223568288148,136.018742195627));
#218080=CARTESIAN_POINT('Ctrl Pts',(207.098250784982,3.06082119940109,135.858058984553));
#218081=CARTESIAN_POINT('',(207.686626030528,-5.91241378256136,130.800689035563));
#218082=CARTESIAN_POINT('Ctrl Pts',(207.495311715924,-4.57621626203826,
134.554850623626));
#218083=CARTESIAN_POINT('Ctrl Pts',(207.501394604565,-4.65780291324943,
134.455301455535));
#218084=CARTESIAN_POINT('Ctrl Pts',(207.507477493205,-4.73605204032821,
134.353195881539));
#218085=CARTESIAN_POINT('Ctrl Pts',(207.513560381845,-4.81080786236673,
134.248784847229));
#218086=CARTESIAN_POINT('Ctrl Pts',(207.521051269147,-4.90286732147391,
134.120205920782));
#218087=CARTESIAN_POINT('Ctrl Pts',(207.528542156449,-4.98990483109698,
133.987743324545));
#218088=CARTESIAN_POINT('Ctrl Pts',(207.53603304375,-5.07157846591905,133.851822254162));
#218089=CARTESIAN_POINT('Ctrl Pts',(207.54351476451,-5.15315215733168,133.716067509366));
#218090=CARTESIAN_POINT('Ctrl Pts',(207.55099648527,-5.22937485457296,133.57686302416));
#218091=CARTESIAN_POINT('Ctrl Pts',(207.558478206029,-5.29994590927886,
133.434665527879));
#218092=CARTESIAN_POINT('Ctrl Pts',(207.565952157474,-5.37044368021461,
133.292615695094));
#218093=CARTESIAN_POINT('Ctrl Pts',(207.57342610892,-5.43530133283305,133.14757936331));
#218094=CARTESIAN_POINT('Ctrl Pts',(207.580900060365,-5.49426246614912,
133.000040584129));
#218095=CARTESIAN_POINT('Ctrl Pts',(207.588367634612,-5.55317329048892,
132.852627693385));
#218096=CARTESIAN_POINT('Ctrl Pts',(207.595835208858,-5.6061974800907,132.702716943952));
#218097=CARTESIAN_POINT('Ctrl Pts',(207.603302783105,-5.6531254094204,132.550815216995));
#218098=CARTESIAN_POINT('Ctrl Pts',(207.610764849886,-5.70001872858451,
132.399025520208));
#218099=CARTESIAN_POINT('Ctrl Pts',(207.618226916667,-5.74082463923541,
132.24524811883));
#218100=CARTESIAN_POINT('Ctrl Pts',(207.625688983447,-5.77538238228886,
132.090007886784));
#218101=CARTESIAN_POINT('Ctrl Pts',(207.633147775048,-5.80992495758262,
131.934835791321));
#218102=CARTESIAN_POINT('Ctrl Pts',(207.640606566648,-5.83822474834345,
131.778202498953));
#218103=CARTESIAN_POINT('Ctrl Pts',(207.648065358249,-5.86017137152897,
131.620646142865));
#218104=CARTESIAN_POINT('Ctrl Pts',(207.655522975005,-5.88211453787224,
131.463114603691));
#218105=CARTESIAN_POINT('Ctrl Pts',(207.662980591761,-5.89770647524243,
131.304660650395));
#218106=CARTESIAN_POINT('Ctrl Pts',(207.670438208517,-5.90688824017458,
131.145830792819));
#218107=CARTESIAN_POINT('Ctrl Pts',(207.67583374161,-5.91353118230476,131.030918511769));
#218108=CARTESIAN_POINT('Ctrl Pts',(207.681229274702,-5.91681984302548,
130.915809664487));
#218109=CARTESIAN_POINT('Ctrl Pts',(207.686624807795,-5.91674887527788,
130.800712412811));
#218110=CARTESIAN_POINT('',(207.794693732013,-5.48556781411874,128.562630683018));
#218111=CARTESIAN_POINT('Ctrl Pts',(207.686626923708,-5.90924709096476,
130.800671958988));
#218112=CARTESIAN_POINT('Ctrl Pts',(207.721753951025,-5.91343857842015,
130.052291188706));
#218113=CARTESIAN_POINT('Ctrl Pts',(207.757773583639,-5.77836975406095,
129.286353104056));
#218114=CARTESIAN_POINT('Ctrl Pts',(207.793793216252,-5.49329697336549,
128.580043386892));
#218115=CARTESIAN_POINT('Ctrl Pts',(207.79468582155,-5.48614114834957,128.562577472722));
#218116=CARTESIAN_POINT('Ctrl Pts',(207.389091944887,-2.65474895531873,
126.670261218454));
#218117=CARTESIAN_POINT('Ctrl Pts',(207.41658252432,-2.94491541138629,126.767817078822));
#218118=CARTESIAN_POINT('Ctrl Pts',(207.448404209708,-3.22924395023264,
126.88438600989));
#218119=CARTESIAN_POINT('Ctrl Pts',(207.51505243423,-3.7596051150903,127.144324967448));
#218120=CARTESIAN_POINT('Ctrl Pts',(207.549736377932,-4.0084503222057,127.286186718169));
#218121=CARTESIAN_POINT('Ctrl Pts',(207.620038152494,-4.47672081944709,
127.597196151352));
#218122=CARTESIAN_POINT('Ctrl Pts',(207.655802877471,-4.69804475485952,
127.766387134892));
#218123=CARTESIAN_POINT('Ctrl Pts',(207.726681002879,-5.11470254565544,
128.138303711736));
#218124=CARTESIAN_POINT('Ctrl Pts',(207.761943960977,-5.31058055330982,
128.342384269375));
#218125=CARTESIAN_POINT('Ctrl Pts',(207.79468582155,-5.48614114834947,128.56257747272));
#218126=CARTESIAN_POINT('',(207.110140564062,-4.91824906508338,130.801328076312));
#218127=CARTESIAN_POINT('Ctrl Pts',(207.179891338435,-4.76405452823404,
129.582490119308));
#218128=CARTESIAN_POINT('Ctrl Pts',(207.171149836886,-4.80226849123941,
129.731485781088));
#218129=CARTESIAN_POINT('Ctrl Pts',(207.162408335336,-4.83353292882372,
129.882448181632));
#218130=CARTESIAN_POINT('Ctrl Pts',(207.153666833787,-4.85766325863286,
130.034756350278));
#218131=CARTESIAN_POINT('Ctrl Pts',(207.14497546476,-4.88165520097116,130.186191031391));
#218132=CARTESIAN_POINT('Ctrl Pts',(207.136284095732,-4.89859453685566,
130.338955897152));
#218133=CARTESIAN_POINT('Ctrl Pts',(207.127592726705,-4.90834771356455,
130.492421865171));
#218134=CARTESIAN_POINT('Ctrl Pts',(207.121775339157,-4.91487580005554,
130.595141127065));
#218135=CARTESIAN_POINT('Ctrl Pts',(207.11595795161,-4.91818546141412,130.698174100575));
#218136=CARTESIAN_POINT('Ctrl Pts',(207.110140564062,-4.91824906508338,
130.801328076312));
#218137=CARTESIAN_POINT('Ctrl Pts',(207.110140564008,-4.91824906508397,
130.801328077268));
#218138=CARTESIAN_POINT('Ctrl Pts',(207.10232974179,-4.91833446369157,130.939829657053));
#218139=CARTESIAN_POINT('Ctrl Pts',(207.094518919572,-4.91256506400957,
131.078351340995));
#218140=CARTESIAN_POINT('Ctrl Pts',(207.086708097354,-4.90096241100966,
131.216368515998));
#218141=CARTESIAN_POINT('Ctrl Pts',(207.078896410447,-4.88935847354873,
131.354400970065));
#218142=CARTESIAN_POINT('Ctrl Pts',(207.071084723539,-4.87192002824314,
131.491928423436));
#218143=CARTESIAN_POINT('Ctrl Pts',(207.063273036631,-4.84872054892325,
131.62843106416));
#218144=CARTESIAN_POINT('Ctrl Pts',(207.055458899586,-4.82551379308231,
131.764976518963));
#218145=CARTESIAN_POINT('Ctrl Pts',(207.047644762541,-4.79654246897585,
131.90049614474));
#218146=CARTESIAN_POINT('Ctrl Pts',(207.039830625497,-4.76193119291241,
132.034480276976));
#218147=CARTESIAN_POINT('Ctrl Pts',(207.032012451602,-4.72730203636823,
132.168533626559));
#218148=CARTESIAN_POINT('Ctrl Pts',(207.024194277707,-4.68702722138493,
132.301049533832));
#218149=CARTESIAN_POINT('Ctrl Pts',(207.016376103812,-4.64128115697165,
132.431533713595));
#218150=CARTESIAN_POINT('Ctrl Pts',(207.008547530707,-4.59547424421175,
132.562191454661));
#218151=CARTESIAN_POINT('Ctrl Pts',(207.000718957602,-4.54418167570927,
132.690811711221));
#218152=CARTESIAN_POINT('Ctrl Pts',(206.992890384497,-4.48762617673331,
132.816919774559));
#218153=CARTESIAN_POINT('Ctrl Pts',(206.985055811211,-4.43102733100928,
132.943124492946));
#218154=CARTESIAN_POINT('Ctrl Pts',(206.977221237926,-4.36915768710697,
133.066812840935));
#218155=CARTESIAN_POINT('Ctrl Pts',(206.96938666464,-4.30228542176686,133.187535645161));
#218156=CARTESIAN_POINT('Ctrl Pts',(206.961539696176,-4.23530735696238,
133.308449446476));
#218157=CARTESIAN_POINT('Ctrl Pts',(206.953692727712,-4.16331106348637,
133.426388009929));
#218158=CARTESIAN_POINT('Ctrl Pts',(206.945845759248,-4.08660777588555,
133.540931455051));
#218159=CARTESIAN_POINT('Ctrl Pts',(206.942922552185,-4.05803373571842,
133.583601972889));
#218160=CARTESIAN_POINT('Ctrl Pts',(206.939999345122,-4.02880687363292,
133.625801664281));
#218161=CARTESIAN_POINT('Ctrl Pts',(206.937076138059,-3.99894465188146,
133.667510060695));
#218162=CARTESIAN_POINT('Ctrl Pts',(206.929301998061,-3.91952739284056,
133.77843169773));
#218163=CARTESIAN_POINT('Ctrl Pts',(206.921527858062,-3.83536570986394,
133.886222330092));
#218164=CARTESIAN_POINT('Ctrl Pts',(206.913753718064,-3.74673486748187,
133.990449269078));
#218165=CARTESIAN_POINT('Ctrl Pts',(206.905989161858,-3.658213287293,134.09454771934));
#218166=CARTESIAN_POINT('Ctrl Pts',(206.898224605652,-3.56523376076694,
134.195090922469));
#218167=CARTESIAN_POINT('Ctrl Pts',(206.890460049446,-3.46811454805166,
134.291675421838));
#218168=CARTESIAN_POINT('Ctrl Pts',(206.882703207698,-3.37109182792838,
134.388163959878));
#218169=CARTESIAN_POINT('Ctrl Pts',(206.874946365951,-3.26993788205166,
134.480701347399));
#218170=CARTESIAN_POINT('Ctrl Pts',(206.867189524203,-3.16501068250007,
134.568917755153));
#218171=CARTESIAN_POINT('Ctrl Pts',(206.859438534277,-3.0601626408413,134.657067611766));
#218172=CARTESIAN_POINT('Ctrl Pts',(206.851687544352,-2.9515473094897,134.74090272641));
#218173=CARTESIAN_POINT('Ctrl Pts',(206.843936554426,-2.83955863515276,
134.820090914788));
#218174=CARTESIAN_POINT('Ctrl Pts',(206.836188861569,-2.72761759787636,
134.899245418577));
#218175=CARTESIAN_POINT('Ctrl Pts',(206.828441168712,-2.61230639015696,
134.973756702305));
#218176=CARTESIAN_POINT('Ctrl Pts',(206.820693475855,-2.49405090237109,
135.043333743086));
#218177=CARTESIAN_POINT('Ctrl Pts',(206.812947405249,-2.37582017552251,
135.112896215471));
#218178=CARTESIAN_POINT('Ctrl Pts',(206.805201334644,-2.25464673160865,
135.177526301768));
#218179=CARTESIAN_POINT('Ctrl Pts',(206.797455264038,-2.13098388076607,
135.236977312298));
#218180=CARTESIAN_POINT('Ctrl Pts',(206.789709137619,-2.00732013888212,
135.296428751197));
#218181=CARTESIAN_POINT('Ctrl Pts',(206.7819630112,-1.88116730665591,135.350700870453));
#218182=CARTESIAN_POINT('Ctrl Pts',(206.774216884781,-1.75300127162441,
135.399593974446));
#218183=CARTESIAN_POINT('Ctrl Pts',(206.766469024802,-1.62480655341618,
135.44849802057));
#218184=CARTESIAN_POINT('Ctrl Pts',(206.758721164823,-1.49459810110302,
135.492020516664));
#218185=CARTESIAN_POINT('Ctrl Pts',(206.750973304844,-1.36286927639058,
135.530010879485));
#218186=CARTESIAN_POINT('Ctrl Pts',(206.743217210822,-1.23100045680149,
135.568041616583));
#218187=CARTESIAN_POINT('Ctrl Pts',(206.735461116801,-1.09760841340135,
135.600528367403));
#218188=CARTESIAN_POINT('Ctrl Pts',(206.72770502278,-0.963199626022195,
135.627371040832));
#218189=CARTESIAN_POINT('Ctrl Pts',(206.719944789696,-0.828719111006118,
135.654228038931));
#218190=CARTESIAN_POINT('Ctrl Pts',(206.712184556613,-0.693221156955318,
135.675434897598));
#218191=CARTESIAN_POINT('Ctrl Pts',(206.70442432353,-0.557218799917317,
135.690943295831));
#218192=CARTESIAN_POINT('Ctrl Pts',(206.696651631796,-0.420998098163723,
135.706476591992));
#218193=CARTESIAN_POINT('Ctrl Pts',(206.688878940061,-0.284271765407574,
135.716293117923));
#218194=CARTESIAN_POINT('Ctrl Pts',(206.681106248327,-0.147555186392696,
135.720396676167));
#218195=CARTESIAN_POINT('Ctrl Pts',(206.6736136703,-0.015765624822631,135.724352349619));
#218196=CARTESIAN_POINT('Ctrl Pts',(206.666121092273,0.11601456527462,135.722999745079));
#218197=CARTESIAN_POINT('Ctrl Pts',(206.658628514246,0.247328944919121,
135.716387842196));
#218198=CARTESIAN_POINT('Ctrl Pts',(206.650854101252,0.383582743781857,
135.709527231134));
#218199=CARTESIAN_POINT('Ctrl Pts',(206.643079688257,0.519766647294013,
135.696982181141));
#218200=CARTESIAN_POINT('Ctrl Pts',(206.635305275263,0.655367801387527,
135.678750436549));
#218201=CARTESIAN_POINT('Ctrl Pts',(206.627540442734,0.790801853192383,
135.660541159068));
#218202=CARTESIAN_POINT('Ctrl Pts',(206.619775610205,0.925654200685813,
135.636659181934));
#218203=CARTESIAN_POINT('Ctrl Pts',(206.612010777677,1.05941334753652,135.607154223538));
#218204=CARTESIAN_POINT('Ctrl Pts',(206.604253656593,1.19303965490963,135.577678567237));
#218205=CARTESIAN_POINT('Ctrl Pts',(206.596496535509,1.32557454289324,135.542591126398));
#218206=CARTESIAN_POINT('Ctrl Pts',(206.588739414425,1.45651334525474,135.501993206179));
#218207=CARTESIAN_POINT('Ctrl Pts',(206.580988142457,1.5873534156012,135.461425898081));
#218208=CARTESIAN_POINT('Ctrl Pts',(206.573236870489,1.71659942391051,135.415356496345));
#218209=CARTESIAN_POINT('Ctrl Pts',(206.565485598521,1.84375893376221,135.363936919885));
#218210=CARTESIAN_POINT('Ctrl Pts',(206.557737620497,1.97086440649336,135.312539194452));
#218211=CARTESIAN_POINT('Ctrl Pts',(206.549989642474,2.09588478259786,135.255795962539));
#218212=CARTESIAN_POINT('Ctrl Pts',(206.542241664451,2.21834499216241,135.193908266043));
#218213=CARTESIAN_POINT('Ctrl Pts',(206.534495306817,2.34077959076295,135.132033512555));
#218214=CARTESIAN_POINT('Ctrl Pts',(206.526748949182,2.46065473910694,135.065016610731));
#218215=CARTESIAN_POINT('Ctrl Pts',(206.519002591548,2.57751784727511,134.993105633615));
#218216=CARTESIAN_POINT('Ctrl Pts',(206.511256176506,2.69438182151258,134.92119412357));
#218217=CARTESIAN_POINT('Ctrl Pts',(206.503509761464,2.80823337806547,134.844388670749));
#218218=CARTESIAN_POINT('Ctrl Pts',(206.495763346422,2.9186472625684,134.762981743565));
#218219=CARTESIAN_POINT('Ctrl Pts',(206.488015196492,3.0290858753689,134.681556584482));
#218220=CARTESIAN_POINT('Ctrl Pts',(206.480267046562,3.13608496949048,134.595528132329));
#218221=CARTESIAN_POINT('Ctrl Pts',(206.472518896633,3.23925116627507,134.505230102469));
#218222=CARTESIAN_POINT('Ctrl Pts',(206.464762512191,3.34252700513922,134.414836106449));
#218223=CARTESIAN_POINT('Ctrl Pts',(206.45700612775,3.44196151476943,134.320163726309));
#218224=CARTESIAN_POINT('Ctrl Pts',(206.449249743308,3.53719670723884,134.221585005399));
#218225=CARTESIAN_POINT('Ctrl Pts',(206.441489219088,3.63248272913906,134.122953670532));
#218226=CARTESIAN_POINT('Ctrl Pts',(206.433728694868,3.7235647084274,134.020412132682));
#218227=CARTESIAN_POINT('Ctrl Pts',(206.425968170648,3.81012466952417,133.914365933507));
#218228=CARTESIAN_POINT('Ctrl Pts',(206.418195189496,3.89682357375458,133.808149512546));
#218229=CARTESIAN_POINT('Ctrl Pts',(206.410422208344,3.9789857203556,133.698417501723));
#218230=CARTESIAN_POINT('Ctrl Pts',(206.402649227192,4.05633571762412,133.58560559211));
#218231=CARTESIAN_POINT('Ctrl Pts',(206.395159781606,4.13086421374525,133.47690873025));
#218232=CARTESIAN_POINT('Ctrl Pts',(206.387670336019,4.20092534590809,133.365353006456));
#218233=CARTESIAN_POINT('Ctrl Pts',(206.380180890433,4.266313865227,133.251348371085));
#218234=CARTESIAN_POINT('Ctrl Pts',(206.372406547022,4.33418975784089,133.133007009811));
#218235=CARTESIAN_POINT('Ctrl Pts',(206.36463220361,4.39724549814214,133.011651903751));
#218236=CARTESIAN_POINT('Ctrl Pts',(206.356857860199,4.45520197698344,132.887713301771));
#218237=CARTESIAN_POINT('Ctrl Pts',(206.349093097628,4.51308703219629,132.763927437583));
#218238=CARTESIAN_POINT('Ctrl Pts',(206.341328335058,4.56588516553323,132.637564763071));
#218239=CARTESIAN_POINT('Ctrl Pts',(206.333563572488,4.61336172857185,132.509082478706));
#218240=CARTESIAN_POINT('Ctrl Pts',(206.32580652166,4.66079113922843,132.380727799318));
#218241=CARTESIAN_POINT('Ctrl Pts',(206.318049470833,4.70290936280457,132.250258063749));
#218242=CARTESIAN_POINT('Ctrl Pts',(206.310292420006,4.73952884382674,132.118152610628));
#218243=CARTESIAN_POINT('Ctrl Pts',(206.302541218515,4.7761207113015,131.986146773889));
#218244=CARTESIAN_POINT('Ctrl Pts',(206.294790017025,4.80722198540851,131.852508049919));
#218245=CARTESIAN_POINT('Ctrl Pts',(206.287038815535,4.83269430378063,131.717732846565));
#218246=CARTESIAN_POINT('Ctrl Pts',(206.279290908073,4.85815579718011,131.583014918637));
#218247=CARTESIAN_POINT('Ctrl Pts',(206.271543000612,4.87799302016867,131.447161855274));
#218248=CARTESIAN_POINT('Ctrl Pts',(206.26379509315,4.89211832584772,131.310682006019));
#218249=CARTESIAN_POINT('Ctrl Pts',(206.256048806118,4.90624067730134,131.17423070073));
#218250=CARTESIAN_POINT('Ctrl Pts',(206.248302519086,4.9146534473754,131.037153258931));
#218251=CARTESIAN_POINT('Ctrl Pts',(206.240556232054,4.91732070875142,130.899964538952));
#218252=CARTESIAN_POINT('Ctrl Pts',(206.232809887587,4.91998798990394,130.762774801783));
#218253=CARTESIAN_POINT('Ctrl Pts',(206.22506354312,4.91690966975381,130.625474175676));
#218254=CARTESIAN_POINT('Ctrl Pts',(206.217317198653,4.90810194759419,130.488578517817));
#218255=CARTESIAN_POINT('Ctrl Pts',(206.209569119204,4.89929225273097,130.351652198845));
#218256=CARTESIAN_POINT('Ctrl Pts',(206.201821039754,4.88475062745858,130.21513141869));
#218257=CARTESIAN_POINT('Ctrl Pts',(206.194072960305,4.86454520291237,130.079527511726));
#218258=CARTESIAN_POINT('Ctrl Pts',(206.186316645792,4.84431830298384,129.943779477834));
#218259=CARTESIAN_POINT('Ctrl Pts',(206.178560331278,4.81841563632905,129.808950651116));
#218260=CARTESIAN_POINT('Ctrl Pts',(206.170804016765,4.78695671008173,129.675543308032));
#218261=CARTESIAN_POINT('Ctrl Pts',(206.163043562283,4.75548099249017,129.542064758175));
#218262=CARTESIAN_POINT('Ctrl Pts',(206.155283107802,4.71844321146889,129.410009580029));
#218263=CARTESIAN_POINT('Ctrl Pts',(206.14752265332,4.6760126848635,129.279864493105));
#218264=CARTESIAN_POINT('Ctrl Pts',(206.139749740871,4.63351404393066,129.149510482424));
#218265=CARTESIAN_POINT('Ctrl Pts',(206.131976828422,4.5856054945835,129.021073056925));
#218266=CARTESIAN_POINT('Ctrl Pts',(206.124203915972,4.53250473784456,128.895019405546));
#218267=CARTESIAN_POINT('Ctrl Pts',(206.116713699522,4.48133522265336,128.773550247191));
#218268=CARTESIAN_POINT('Ctrl Pts',(206.109223483071,4.42534474547032,128.654294760804));
#218269=CARTESIAN_POINT('Ctrl Pts',(206.101733266621,4.36476734543776,128.537647339999));
#218270=CARTESIAN_POINT('Ctrl Pts',(206.093958959944,4.30189235529015,128.416575695624));
#218271=CARTESIAN_POINT('Ctrl Pts',(206.086184653268,4.23387645089009,128.297930328045));
#218272=CARTESIAN_POINT('Ctrl Pts',(206.078410346591,4.16093074001882,128.18217861792));
#218273=CARTESIAN_POINT('Ctrl Pts',(206.070645621474,4.08807493217016,128.066569567707));
#218274=CARTESIAN_POINT('Ctrl Pts',(206.062880896357,4.01030161335004,127.953847406604));
#218275=CARTESIAN_POINT('Ctrl Pts',(206.05511617124,3.92786859889688,127.844456677858));
#218276=CARTESIAN_POINT('Ctrl Pts',(206.04735915854,3.84551746214591,127.735174602927));
#218277=CARTESIAN_POINT('Ctrl Pts',(206.039602145841,3.7585160740671,127.629217685533));
#218278=CARTESIAN_POINT('Ctrl Pts',(206.031845133142,3.66716633068647,127.52700281507));
#218279=CARTESIAN_POINT('Ctrl Pts',(206.024093970412,3.57588547893075,127.424865030194));
#218280=CARTESIAN_POINT('Ctrl Pts',(206.016342807682,3.48026305863852,127.326463965419));
#218281=CARTESIAN_POINT('Ctrl Pts',(206.008591644952,3.38064191709146,127.232184349392));
#218282=CARTESIAN_POINT('Ctrl Pts',(206.000843777079,3.28106312240745,127.137944809658));
#218283=CARTESIAN_POINT('Ctrl Pts',(205.993095909207,3.17748927055705,127.04782350237));
#218284=CARTESIAN_POINT('Ctrl Pts',(205.985348041334,3.070300668997,126.962168942954));
#218285=CARTESIAN_POINT('Ctrl Pts',(205.97760179439,2.96313449232946,126.876532303301));
#218286=CARTESIAN_POINT('Ctrl Pts',(205.969855547446,2.85235537539139,126.79536079669));
#218287=CARTESIAN_POINT('Ctrl Pts',(205.962109300503,2.73837705773569,126.718962943879));
#218288=CARTESIAN_POINT('Ctrl Pts',(205.954362996587,2.62439790178891,126.642564529175));
#218289=CARTESIAN_POINT('Ctrl Pts',(205.94661669267,2.5072198229346,126.570940056014));
#218290=CARTESIAN_POINT('Ctrl Pts',(205.938870388754,2.38728557715688,126.50435472971));
#218291=CARTESIAN_POINT('Ctrl Pts',(205.931122350283,2.26732447565317,126.437754493592));
#218292=CARTESIAN_POINT('Ctrl Pts',(205.923374311811,2.14460632090196,126.376195839389));
#218293=CARTESIAN_POINT('Ctrl Pts',(205.915626273339,2.01959813448211,126.319897836173));
#218294=CARTESIAN_POINT('Ctrl Pts',(205.907870000251,1.8944570893462,126.263539999433));
#218295=CARTESIAN_POINT('Ctrl Pts',(205.900113727163,1.76702150772587,126.212454143145));
#218296=CARTESIAN_POINT('Ctrl Pts',(205.892357454075,1.63777856078686,126.166811216392));
#218297=CARTESIAN_POINT('Ctrl Pts',(205.884597041329,1.5084666346276,126.121143929212));
#218298=CARTESIAN_POINT('Ctrl Pts',(205.876836628582,1.3773457946557,126.08092547459));
#218299=CARTESIAN_POINT('Ctrl Pts',(205.869076215836,1.24491704770284,126.046276485603));
#218300=CARTESIAN_POINT('Ctrl Pts',(205.861303345232,1.11227571174918,126.011571874297));
#218301=CARTESIAN_POINT('Ctrl Pts',(205.853530474629,0.97832265542302,125.982454678108));
#218302=CARTESIAN_POINT('Ctrl Pts',(205.845757604025,0.843568606457823,
125.958994267258));
#218303=CARTESIAN_POINT('Ctrl Pts',(205.838266950286,0.713707198462261,
125.93638565543));
#218304=CARTESIAN_POINT('Ctrl Pts',(205.830776296547,0.583102259513571,
125.919030219509));
#218305=CARTESIAN_POINT('Ctrl Pts',(205.823285642808,0.452212191984598,
125.90694423789));
#218306=CARTESIAN_POINT('Ctrl Pts',(205.815511295583,0.316364925691163,
125.894400523959));
#218307=CARTESIAN_POINT('Ctrl Pts',(205.807736948359,0.179780181164248,
125.887493536688));
#218308=CARTESIAN_POINT('Ctrl Pts',(205.799962601134,0.0429652936190226,
125.886298291198));
#218309=CARTESIAN_POINT('Ctrl Pts',(205.792197834953,-0.0936809843600888,
125.885104518719));
#218310=CARTESIAN_POINT('Ctrl Pts',(205.784433068771,-0.23055645382959,
125.889608485683));
#218311=CARTESIAN_POINT('Ctrl Pts',(205.77666830259,-0.367147747384615,
125.899833566556));
#218312=CARTESIAN_POINT('Ctrl Pts',(205.768911248356,-0.503603378781414,
125.910048491902));
#218313=CARTESIAN_POINT('Ctrl Pts',(205.761154194123,-0.639775008589745,
125.925973194331));
#218314=CARTESIAN_POINT('Ctrl Pts',(205.753397139889,-0.775148709250783,
125.94757901438));
#218315=CARTESIAN_POINT('Ctrl Pts',(205.745645935201,-0.910420325464687,
125.969168541617));
#218316=CARTESIAN_POINT('Ctrl Pts',(205.737894730512,-1.04489482568991,
125.996430597873));
#218317=CARTESIAN_POINT('Ctrl Pts',(205.730143525824,-1.17806320546229,
126.029284686606));
#218318=CARTESIAN_POINT('Ctrl Pts',(205.722395615495,-1.31117498700093,
126.062124811938));
#218319=CARTESIAN_POINT('Ctrl Pts',(205.714647705166,-1.44298137338557,
126.100552149252));
#218320=CARTESIAN_POINT('Ctrl Pts',(205.706899794837,-1.57298357962825,
126.144435111646));
#218321=CARTESIAN_POINT('Ctrl Pts',(205.699153505139,-1.70295859328728,
126.188308895034));
#218322=CARTESIAN_POINT('Ctrl Pts',(205.691407215442,-1.83112980724108,
126.237635908722));
#218323=CARTESIAN_POINT('Ctrl Pts',(205.683660925745,-1.9570140146508,126.292234820454));
#218324=CARTESIAN_POINT('Ctrl Pts',(205.675914578818,-2.08289915209403,
126.346834135564));
#218325=CARTESIAN_POINT('Ctrl Pts',(205.668168231891,-2.2064968905978,126.406705270871));
#218326=CARTESIAN_POINT('Ctrl Pts',(205.660421884964,-2.32734478203693,
126.471619068844));
#218327=CARTESIAN_POINT('Ctrl Pts',(205.652673803264,-2.44821973703175,
126.536547404084));
#218328=CARTESIAN_POINT('Ctrl Pts',(205.644925721563,-2.56634327519558,
126.606520464177));
#218329=CARTESIAN_POINT('Ctrl Pts',(205.637177639863,-2.6812786482065,126.68126373862));
#218330=CARTESIAN_POINT('Ctrl Pts',(205.629421323445,-2.79633617537112,
126.756086450761));
#218331=CARTESIAN_POINT('Ctrl Pts',(205.621665007027,-2.90819844040077,
126.835689291279));
#218332=CARTESIAN_POINT('Ctrl Pts',(205.613908690609,-3.01645828850523,
126.919754787342));
#218333=CARTESIAN_POINT('Ctrl Pts',(205.606148234409,-3.12477591819194,
127.003865151724));
#218334=CARTESIAN_POINT('Ctrl Pts',(205.598387778208,-3.22948700142695,
127.092442665323));
#218335=CARTESIAN_POINT('Ctrl Pts',(205.590627322007,-3.3302192372797,127.185131018031));
#218336=CARTESIAN_POINT('Ctrl Pts',(205.582854408177,-3.43111317560035,
127.277968160599));
#218337=CARTESIAN_POINT('Ctrl Pts',(205.575081494346,-3.52801522649826,
127.374929052501));
#218338=CARTESIAN_POINT('Ctrl Pts',(205.567308580516,-3.62059096362825,
127.475621496428));
#218339=CARTESIAN_POINT('Ctrl Pts',(205.559818393342,-3.70979941414655,
127.572651422196));
#218340=CARTESIAN_POINT('Ctrl Pts',(205.552328206168,-3.79499060911529,
127.673145922983));
#218341=CARTESIAN_POINT('Ctrl Pts',(205.544838018995,-3.87590312513928,
127.776728204766));
#218342=CARTESIAN_POINT('Ctrl Pts',(205.53706126549,-3.95991126511941,127.884273430835));
#218343=CARTESIAN_POINT('Ctrl Pts',(205.529284511985,-4.03957765797006,
127.995494127098));
#218344=CARTESIAN_POINT('Ctrl Pts',(205.521507758481,-4.11456321009359,
128.110004914871));
#218345=CARTESIAN_POINT('Ctrl Pts',(205.513743508267,-4.18942820212018,
128.224331594755));
#218346=CARTESIAN_POINT('Ctrl Pts',(205.505979258053,-4.25962712878069,
128.341937508539));
#218347=CARTESIAN_POINT('Ctrl Pts',(205.498215007839,-4.32486122114154,
128.462404494927));
#218348=CARTESIAN_POINT('Ctrl Pts',(205.490457952857,-4.39003486021618,
128.582759842984));
#218349=CARTESIAN_POINT('Ctrl Pts',(205.482700897876,-4.45025263063646,
128.705970650087));
#218350=CARTESIAN_POINT('Ctrl Pts',(205.474943842894,-4.50525896992651,
128.831589805638));
#218351=CARTESIAN_POINT('Ctrl Pts',(205.467193142368,-4.5602202488983,128.957106055974));
#218352=CARTESIAN_POINT('Ctrl Pts',(205.459442441842,-4.60997843839768,
129.085026371888));
#218353=CARTESIAN_POINT('Ctrl Pts',(205.451691741317,-4.65432411968393,
129.214879554002));
#218354=CARTESIAN_POINT('Ctrl Pts',(205.444469975199,-4.69564349946542,
129.335871109256));
#218355=CARTESIAN_POINT('Ctrl Pts',(205.437248209081,-4.73226423551571,
129.458540250484));
#218356=CARTESIAN_POINT('Ctrl Pts',(205.430026442963,-4.76405452823405,
129.582490119308));
#218357=CARTESIAN_POINT('Ctrl Pts',(210.578629502474,3.43871735229388,135.623751273273));
#218358=CARTESIAN_POINT('Ctrl Pts',(210.532211638871,4.24191310225744,135.050661598608));
#218359=CARTESIAN_POINT('Ctrl Pts',(210.439385837966,5.5417116830592,133.497735776206));
#218360=CARTESIAN_POINT('Ctrl Pts',(210.253744162458,6.40049231640402,129.500124813146));
#218361=CARTESIAN_POINT('Ctrl Pts',(210.021704475947,3.49988613106459,124.739836436729));
#218362=CARTESIAN_POINT('Ctrl Pts',(209.743256852134,-3.22132718841443,
124.582443963435));
#218363=CARTESIAN_POINT('Ctrl Pts',(209.464809228321,-6.97029916743427,
130.151104711613));
#218364=CARTESIAN_POINT('Ctrl Pts',(209.186361604508,-4.320155850937,136.315756482887));
#218365=CARTESIAN_POINT('Ctrl Pts',(208.907913980696,2.30329626696544,137.417975354914));
#218366=CARTESIAN_POINT('Ctrl Pts',(208.629466356883,6.80838731381026,132.441404887444));
#218367=CARTESIAN_POINT('Ctrl Pts',(208.35101873307,5.05782663488002,125.961106241921));
#218368=CARTESIAN_POINT('Ctrl Pts',(208.072571109257,-1.34111875541754,
123.931185212061));
#218369=CARTESIAN_POINT('Ctrl Pts',(207.794123485444,-6.50738248846785,
128.217554840719));
#218370=CARTESIAN_POINT('Ctrl Pts',(207.515675861631,-5.69381680528821,
134.880978212762));
#218371=CARTESIAN_POINT('Ctrl Pts',(207.237228237818,0.352161018465804,
137.798239159538));
#218372=CARTESIAN_POINT('Ctrl Pts',(206.958780614005,6.07448159193836,134.288440920842));
#218373=CARTESIAN_POINT('Ctrl Pts',(206.680332990192,6.21467071562046,127.576957111676));
#218374=CARTESIAN_POINT('Ctrl Pts',(206.40188536638,0.643870262773591,123.831292031177));
#218375=CARTESIAN_POINT('Ctrl Pts',(206.123437742567,-5.51860979104455,
126.493540260974));
#218376=CARTESIAN_POINT('Ctrl Pts',(205.844990118754,-6.60976007302988,
133.117219720399));
#218377=CARTESIAN_POINT('Ctrl Pts',(205.566542494941,-1.62686214948821,
137.615495756827));
#218378=CARTESIAN_POINT('Ctrl Pts',(205.288094871128,4.8510417637676,135.85467075854));
#218379=CARTESIAN_POINT('Ctrl Pts',(205.009647247315,6.87107573233629,129.452857771449));
#218380=CARTESIAN_POINT('Ctrl Pts',(204.731199623502,2.57692653546199,124.293009711503));
#218381=CARTESIAN_POINT('Ctrl Pts',(204.452751999689,-4.08529213152394,
125.116775123829));
#218382=CARTESIAN_POINT('Ctrl Pts',(204.174304375876,-6.9933269740478,131.167153704944));
#218383=CARTESIAN_POINT('Ctrl Pts',(203.895856752063,-3.47483593506387,
136.884143186524));
#218384=CARTESIAN_POINT('Ctrl Pts',(203.617409128251,3.23685955433703,137.014109488232));
#218385=CARTESIAN_POINT('Ctrl Pts',(203.338961504438,6.97403925260401,131.437619947721));
#218386=CARTESIAN_POINT('Ctrl Pts',(203.060513880625,4.30241757323156,125.27919601562));
#218387=CARTESIAN_POINT('Ctrl Pts',(202.782066256812,-2.32291566837452,
124.198128435325));
#218388=CARTESIAN_POINT('Ctrl Pts',(202.503618632999,-6.81360289295739,
129.18786549711));
#218389=CARTESIAN_POINT('Ctrl Pts',(202.225171009186,-5.0429219211382,135.663082604955));
#218390=CARTESIAN_POINT('Ctrl Pts',(201.946723385373,1.36195793536179,137.673371567868));
#218391=CARTESIAN_POINT('Ctrl Pts',(201.66827576156,6.51526498482727,133.371375037445));
#218392=CARTESIAN_POINT('Ctrl Pts',(201.389828137747,5.6813618015098,126.710417660699));
#218393=CARTESIAN_POINT('Ctrl Pts',(201.111380513935,-0.373435327379839,
123.811593861123));
#218394=CARTESIAN_POINT('Ctrl Pts',(200.832932890122,-6.08506363376988,
127.338781095048));
#218395=CARTESIAN_POINT('Ctrl Pts',(200.554485266309,-6.20481573259303,
134.050666607207));
#218396=CARTESIAN_POINT('Ctrl Pts',(200.276037642496,-0.622645295272457,
137.779355505743));
#218397=CARTESIAN_POINT('Ctrl Pts',(199.997590018683,5.53170575049466,135.098364849491));
#218398=CARTESIAN_POINT('Ctrl Pts',(199.71914239487,6.60268945040398,128.471394077867));
#218399=CARTESIAN_POINT('Ctrl Pts',(199.440694771057,1.60612410470526,123.988305584475));
#218400=CARTESIAN_POINT('Ctrl Pts',(199.162247147244,-4.86639082969376,
125.768838683693));
#218401=CARTESIAN_POINT('Ctrl Pts',(198.883799523432,-6.86693032801245,
132.176770441218));
#218402=CARTESIAN_POINT('Ctrl Pts',(198.605351899619,-2.5570963230842,137.323524616753));
#218403=CARTESIAN_POINT('Ctrl Pts',(198.326904275806,4.10258428165832,136.479485555902));
#218404=CARTESIAN_POINT('Ctrl Pts',(198.048456651993,6.99219035394115,130.420283921986));
#218405=CARTESIAN_POINT('Ctrl Pts',(197.77000902818,3.45631507844086,124.714030008118));
#218406=CARTESIAN_POINT('Ctrl Pts',(197.491561404367,-3.25574490376804,
124.604492395141));
#218407=CARTESIAN_POINT('Ctrl Pts',(197.213113780554,-6.97593437139489,
130.192330798173));
#218408=CARTESIAN_POINT('Ctrl Pts',(196.934666156741,-4.28558094504976,
136.342594705906));
#218409=CARTESIAN_POINT('Ctrl Pts',(196.656218532928,2.3430120075278,137.403492044232));
#218410=CARTESIAN_POINT('Ctrl Pts',(196.377770909115,6.81849138768721,132.400109986944));
#218411=CARTESIAN_POINT('Ctrl Pts',(196.099323285303,5.02811028438465,125.930312215887));
#218412=CARTESIAN_POINT('Ctrl Pts',(195.82087566149,-1.38285853342424,123.939526815472));
#218413=CARTESIAN_POINT('Ctrl Pts',(195.542428037677,-6.5230479154113,128.257188313404));
#218414=CARTESIAN_POINT('Ctrl Pts',(195.263980413864,-5.66887493174189,
134.915576722577));
#218415=CARTESIAN_POINT('Ctrl Pts',(194.985532790051,0.394717174261835,
137.795958375315));
#218416=CARTESIAN_POINT('Ctrl Pts',(194.707085166238,6.09558348012494,134.251403247221));
#218417=CARTESIAN_POINT('Ctrl Pts',(194.428637542425,6.19490635356113,127.539184339867));
#218418=CARTESIAN_POINT('Ctrl Pts',(194.150189918612,0.601412926074683,
123.827502918989));
#218419=CARTESIAN_POINT('Ctrl Pts',(193.871742294799,-5.54474959981957,
126.527212884656));
#218420=CARTESIAN_POINT('Ctrl Pts',(193.593294670987,-6.59555811955654,
133.157412666584));
#218421=CARTESIAN_POINT('Ctrl Pts',(193.314847047174,-1.58537093834796,
137.625272568447));
#218422=CARTESIAN_POINT('Ctrl Pts',(193.036399423361,4.88169468552635,135.825047607524));
#218423=CARTESIAN_POINT('Ctrl Pts',(192.757951799548,6.86272137744547,129.411056577024));
#218424=CARTESIAN_POINT('Ctrl Pts',(192.479504175735,2.53724238606986,124.277443893095));
#218425=CARTESIAN_POINT('Ctrl Pts',(192.201056551922,-4.11983840692253,
125.141748821346));
#218426=CARTESIAN_POINT('Ctrl Pts',(191.922608928109,-6.99098896924831,
131.209717356357));
#218427=CARTESIAN_POINT('Ctrl Pts',(191.644161304296,-3.43776219763276,
136.905182851196));
#218428=CARTESIAN_POINT('Ctrl Pts',(191.365713680483,3.27460008958736,136.994290755064));
#218429=CARTESIAN_POINT('Ctrl Pts',(191.08726605667,6.9777648675845,131.395155257469));
#218430=CARTESIAN_POINT('Ctrl Pts',(190.808818432858,4.26870461503614,125.253108347726));
#218431=CARTESIAN_POINT('Ctrl Pts',(190.530370809044,-2.36308664091672,
124.212391080215));
#218432=CARTESIAN_POINT('Ctrl Pts',(190.251923185232,-6.82331671706736,
129.229371781915));
#218433=CARTESIAN_POINT('Ctrl Pts',(189.973475561419,-5.01325206778612,
135.693690281095));
#218434=CARTESIAN_POINT('Ctrl Pts',(189.695027937606,1.40374632081163,137.664953676525));
#218435=CARTESIAN_POINT('Ctrl Pts',(189.416580313793,6.53077041740369,133.331667209374));
#218436=CARTESIAN_POINT('Ctrl Pts',(189.13813268998,5.65633554627347,126.675909450142));
#218437=CARTESIAN_POINT('Ctrl Pts',(188.859685066167,-0.41599536452862,
123.81399662772));
#218438=CARTESIAN_POINT('Ctrl Pts',(188.581237442354,-6.10604685783229,
127.375886813701));
#218439=CARTESIAN_POINT('Ctrl Pts',(188.302789818542,-6.18493958576042,
134.088376935175));
#218440=CARTESIAN_POINT('Ctrl Pts',(188.024342194729,-0.580174985471077,
137.783016493883));
#218441=CARTESIAN_POINT('Ctrl Pts',(187.745894570916,5.55774208334242,135.064612228548));
#218442=CARTESIAN_POINT('Ctrl Pts',(187.467446947103,6.58836568835925,128.431244857581));
#218443=CARTESIAN_POINT('Ctrl Pts',(187.18899932329,1.56460308533104,123.97865493689));
#218444=CARTESIAN_POINT('Ctrl Pts',(186.910551699478,-4.89695331800637,
125.798555082479));
#218445=CARTESIAN_POINT('Ctrl Pts',(186.632104075664,-6.85844885156509,
132.218545967617));
#218446=CARTESIAN_POINT('Ctrl Pts',(186.353656451852,-2.51736494438869,
137.338969602853));
#218447=CARTESIAN_POINT('Ctrl Pts',(186.075208828038,4.13705436656654,136.454406814005));
#218448=CARTESIAN_POINT('Ctrl Pts',(185.796761204226,6.98972282098866,130.377727590732));
#218449=CARTESIAN_POINT('Ctrl Pts',(185.518313580413,3.41917746986535,124.693103276936));
#218450=CARTESIAN_POINT('Ctrl Pts',(185.2398659566,-3.29342493995873,124.62442590766));
#218451=CARTESIAN_POINT('Ctrl Pts',(184.961418332787,-6.97953072271363,
130.234806630193));
#218452=CARTESIAN_POINT('Ctrl Pts',(184.682970708974,-4.25178874032612,
136.368579642862));
#218453=CARTESIAN_POINT('Ctrl Pts',(184.404523085161,2.38313938299372,137.389107198495));
#218454=CARTESIAN_POINT('Ctrl Pts',(184.126075461348,6.82807883617355,132.358574329007));
#218455=CARTESIAN_POINT('Ctrl Pts',(183.847627837535,4.99834740910532,125.899794986266));
#218456=CARTESIAN_POINT('Ctrl Pts',(183.569180213722,-1.42462110408482,
123.948071857337));
#218457=CARTESIAN_POINT('Ctrl Pts',(183.290732589909,-6.53843241923107,
128.296943150732));
#218458=CARTESIAN_POINT('Ctrl Pts',(183.012284966097,-5.64374376128527,
134.950008601993));
#218459=CARTESIAN_POINT('Ctrl Pts',(182.733837342284,0.437269701071178,
137.793426081729));
#218460=CARTESIAN_POINT('Ctrl Pts',(182.455389718471,6.11645366995566,134.214233834728));
#218461=CARTESIAN_POINT('Ctrl Pts',(182.176942094658,6.17491552152431,127.501534682722));
#218462=CARTESIAN_POINT('Ctrl Pts',(181.898494470845,0.558931670205695,
123.82397121282));
#218463=CARTESIAN_POINT('Ctrl Pts',(181.620046847032,-5.57068308070185,
126.561044594899));
#218464=CARTESIAN_POINT('Ctrl Pts',(181.341599223219,-6.58111222344223,
133.197518104296));
#218465=CARTESIAN_POINT('Ctrl Pts',(181.063151599407,-1.54382073804491,
137.634796795631));
#218466=CARTESIAN_POINT('Ctrl Pts',(180.784703975594,4.91216658577983,135.795238324681));
#218467=CARTESIAN_POINT('Ctrl Pts',(180.506256351781,6.85411278995147,129.369307058824));
#218468=CARTESIAN_POINT('Ctrl Pts',(180.227808727968,2.49746418218255,124.262119907186));
#218469=CARTESIAN_POINT('Ctrl Pts',(179.949361104155,-4.15423200110403,
125.16693236216));
#218470=CARTESIAN_POINT('Ctrl Pts',(179.670913480342,-6.98839192089168,
131.252265980172));
#218471=CARTESIAN_POINT('Ctrl Pts',(179.392465856529,-3.40056106730489,
136.925996451342));
#218472=CARTESIAN_POINT('Ctrl Pts',(179.114018232716,3.31221928049139,136.974242649806));
#218473=CARTESIAN_POINT('Ctrl Pts',(178.835570608904,6.98123192042358,131.352668676138));
#218474=CARTESIAN_POINT('Ctrl Pts',(178.55712298509,4.23483347762603,125.227226382977));
#218475=CARTESIAN_POINT('Ctrl Pts',(178.278675361277,-2.40317004799311,
124.22689799325));
#218476=CARTESIAN_POINT('Ctrl Pts',(178.000227737465,-6.83277770089014,
129.270936428355));
#218477=CARTESIAN_POINT('Ctrl Pts',(177.721780113652,-4.98339644641697,
135.724116781409));
#218478=CARTESIAN_POINT('Ctrl Pts',(177.443332489839,1.44548268986267,137.65628156334));
#218479=CARTESIAN_POINT('Ctrl Pts',(177.164884866026,6.54603384991367,133.291865731052));
#218480=CARTESIAN_POINT('Ctrl Pts',(176.886437242213,5.63109969342586,126.64155422085));
#218481=CARTESIAN_POINT('Ctrl Pts',(176.6079896184,-0.458539986806858,123.816658424832));
#218482=CARTESIAN_POINT('Ctrl Pts',(176.329541994587,-6.12680382008778,
127.413119575705));
#218483=CARTESIAN_POINT('Ctrl Pts',(176.051094370774,-6.16483425371434,
134.125965572714));
#218484=CARTESIAN_POINT('Ctrl Pts',(175.772646746962,-0.537683177073775,
137.786418885364));
#218485=CARTESIAN_POINT('Ctrl Pts',(175.494199123148,5.58357247201413,135.030701742416));
#218486=CARTESIAN_POINT('Ctrl Pts',(175.215751499336,6.57379779200069,128.391183573973));
#218487=CARTESIAN_POINT('Ctrl Pts',(174.937303875523,1.5230240890144,123.969257218339));
#218488=CARTESIAN_POINT('Ctrl Pts',(174.65885625171,-4.92733434791298,125.82845697323));
#218489=CARTESIAN_POINT('Ctrl Pts',(174.380408627897,-6.84971323277332,
132.260269090858));
#218490=CARTESIAN_POINT('Ctrl Pts',(174.101961004084,-2.4775402838095,137.354172446613));
#218491=CARTESIAN_POINT('Ctrl Pts',(173.823513380271,4.1713711514037,136.429118707571));
#218492=CARTESIAN_POINT('Ctrl Pts',(173.545065756458,6.98699628128659,130.335187068521));
#218493=CARTESIAN_POINT('Ctrl Pts',(173.266618132645,3.38191316241135,124.672403000642));
#218494=CARTESIAN_POINT('Ctrl Pts',(172.988170508833,-3.33098293707706,
124.644588419932));
#218495=CARTESIAN_POINT('Ctrl Pts',(172.709722885019,-6.98286844495469,
130.277303567246));
#218496=CARTESIAN_POINT('Ctrl Pts',(172.431275261207,-4.21783898400718,
136.394358395635));
#218497=CARTESIAN_POINT('Ctrl Pts',(172.152827637394,2.42317845035331,137.374478352552));
#218498=CARTESIAN_POINT('Ctrl Pts',(171.874380013581,6.83741326768756,132.316981079111));
#218499=CARTESIAN_POINT('Ctrl Pts',(171.595932389768,4.96839931822471,125.869459497128));
#218500=CARTESIAN_POINT('Ctrl Pts',(171.317484765955,-1.46633088488636,
123.956870961504));
#218501=CARTESIAN_POINT('Ctrl Pts',(171.039037142142,-6.55357463903296,
128.336790901335));
#218502=CARTESIAN_POINT('Ctrl Pts',(170.760589518329,-5.61840345982816,
134.984286862899));
#218503=CARTESIAN_POINT('Ctrl Pts',(170.482141894517,0.479806024690783,
137.79063480575));
#218504=CARTESIAN_POINT('Ctrl Pts',(170.203694270703,6.13709721234627,134.176938068128));
#218505=CARTESIAN_POINT('Ctrl Pts',(169.925246646891,6.15469587572206,127.464007413007));
#218506=CARTESIAN_POINT('Ctrl Pts',(169.646799023078,0.51642970291829,123.820698167548));
#218507=CARTESIAN_POINT('Ctrl Pts',(169.368351399265,-5.59641013787386,
126.595033542778));
#218508=CARTESIAN_POINT('Ctrl Pts',(169.089903775452,-6.56642246179436,
133.237534862678));
#218509=CARTESIAN_POINT('Ctrl Pts',(168.811456151639,-1.50221333089678,
137.644067918489));
#218510=CARTESIAN_POINT('Ctrl Pts',(168.533008527826,4.94245646389391,135.76524410303));
#218511=CARTESIAN_POINT('Ctrl Pts',(168.254560904013,6.84525022078748,129.32761071706));
#218512=CARTESIAN_POINT('Ctrl Pts',(167.976113280201,2.45759343384159,124.247038346411));
#218513=CARTESIAN_POINT('Ctrl Pts',(167.697665656387,-4.1884716586909,125.192324799951));
#218514=CARTESIAN_POINT('Ctrl Pts',(167.419218032575,-6.98553591510243,
131.294798006688));
#218515=CARTESIAN_POINT('Ctrl Pts',(167.140770408762,-3.36323392793624,
136.946583212019));
#218516=CARTESIAN_POINT('Ctrl Pts',(166.862322784949,3.34971573589186,136.953965917302));
#218517=CARTESIAN_POINT('Ctrl Pts',(166.583875161136,6.98444028114645,131.310161777048));
#218518=CARTESIAN_POINT('Ctrl Pts',(166.305427537323,4.20080541690416,125.20155108099));
#218519=CARTESIAN_POINT('Ctrl Pts',(166.02697991351,-2.44316440471955,124.241648636582));
#218520=CARTESIAN_POINT('Ctrl Pts',(165.748532289697,-6.84198549362249,
129.312557896394));
#218521=CARTESIAN_POINT('Ctrl Pts',(165.470084665885,-4.95335616345982,
135.754360978348));
#218522=CARTESIAN_POINT('Ctrl Pts',(165.191637042072,1.48716549602113,137.647355549705));
#218523=CARTESIAN_POINT('Ctrl Pts',(164.913189418259,6.56105471673207,133.251972077313));
#218524=CARTESIAN_POINT('Ctrl Pts',(164.634741794446,5.60565517810829,126.60735324588));
#218525=CARTESIAN_POINT('Ctrl Pts',(164.356294170633,-0.501067617717217,
123.819579153818));
#218526=CARTESIAN_POINT('Ctrl Pts',(164.07784654682,-6.1473337513746,127.450478001396));
#218527=CARTESIAN_POINT('Ctrl Pts',(163.799398923007,-6.14450048146789,
134.163431126959));
#218528=CARTESIAN_POINT('Ctrl Pts',(163.520951299194,-0.495171444628521,
137.789562554107));
#218529=CARTESIAN_POINT('Ctrl Pts',(163.242503675381,5.60919595935461,134.996634647659));
#218530=CARTESIAN_POINT('Ctrl Pts',(162.964056051569,6.55898630114736,128.351211711527));
#218531=CARTESIAN_POINT('Ctrl Pts',(162.685608427755,1.48138865648,123.960112777059));
#218532=CARTESIAN_POINT('Ctrl Pts',(162.407160803943,-4.95753279363329,
125.85854324792));
#218533=CARTESIAN_POINT('Ctrl Pts',(162.12871318013,-6.84072379533872,132.301938264875));
#218534=CARTESIAN_POINT('Ctrl Pts',(161.850265556317,-2.4376238170639,137.369132584688));
#218535=CARTESIAN_POINT('Ctrl Pts',(161.571817932504,4.20553336454888,136.403622173655));
#218536=CARTESIAN_POINT('Ctrl Pts',(161.293370308691,6.98401083586784,130.292663931709));
#218537=CARTESIAN_POINT('Ctrl Pts',(161.014922684878,3.34452353692138,124.651929946293));
#218538=CARTESIAN_POINT('Ctrl Pts',(160.736475061065,-3.36841750339773,
124.664979184829));
#218539=CARTESIAN_POINT('Ctrl Pts',(160.458027437253,-6.98594741443756,
130.319820034592));
#218540=CARTESIAN_POINT('Ctrl Pts',(160.179579813439,-4.18373293411359,
136.419930008985));
#218541=CARTESIAN_POINT('Ctrl Pts',(159.901132189627,2.46312772594441,137.35960604848));
#218542=CARTESIAN_POINT('Ctrl Pts',(159.622684565814,6.84649433633851,132.275331778507));
#218543=CARTESIAN_POINT('Ctrl Pts',(159.344236942001,4.93826712148011,125.839306872565));
#218544=CARTESIAN_POINT('Ctrl Pts',(159.065789318188,-1.50798633025781,
123.965923801919));
#218545=CARTESIAN_POINT('Ctrl Pts',(158.787341694375,-6.56847401371661,
128.376730088641));
#218546=CARTESIAN_POINT('Ctrl Pts',(158.508894070562,-5.59285496636459,
135.018410235101));
#218547=CARTESIAN_POINT('Ctrl Pts',(158.230446446749,0.522324568921774,
137.787584650814));
#218548=CARTESIAN_POINT('Ctrl Pts',(157.951998822937,6.15751334234277,134.139517329431));
#218549=CARTESIAN_POINT('Ctrl Pts',(157.673551199123,6.13424816540071,127.426603921307));
#218550=CARTESIAN_POINT('Ctrl Pts',(157.395103575311,0.473908599138188,
123.817683904457));
#218551=CARTESIAN_POINT('Ctrl Pts',(157.116655951498,-5.62192981801017,
126.62917846882));
#218552=CARTESIAN_POINT('Ctrl Pts',(156.838208327685,-6.55148937894732,
133.277461458893));
#218553=CARTESIAN_POINT('Ctrl Pts',(156.559760703872,-1.46055025868114,
137.653085593479));
#218554=CARTESIAN_POINT('Ctrl Pts',(156.281313080059,4.97256319746619,135.735066054016));
#218555=CARTESIAN_POINT('Ctrl Pts',(156.002865456246,6.83613399835919,129.285969096806));
#218556=CARTESIAN_POINT('Ctrl Pts',(155.724417832433,2.4176316184721,124.232199769625));
#218557=CARTESIAN_POINT('Ctrl Pts',(155.44597020862,-4.2225561109203,125.217925193794));
#218558=CARTESIAN_POINT('Ctrl Pts',(155.167522584808,-6.98242105771092,
131.337311859867));
#218559=CARTESIAN_POINT('Ctrl Pts',(154.889074960995,-3.3257821626974,136.96694237038));
#218560=CARTESIAN_POINT('Ctrl Pts',(154.610627337182,3.38708806634394,136.933461308912));
#218561=CARTESIAN_POINT('Ctrl Pts',(154.332179713369,6.98738983086623,131.267636135312));
#218562=CARTESIAN_POINT('Ctrl Pts',(154.053732089556,4.1666216937926,125.17608339317));
#218563=CARTESIAN_POINT('Ctrl Pts',(153.775284465743,-2.48306822909056,
124.256642463619));
#218564=CARTESIAN_POINT('Ctrl Pts',(153.49683684193,-6.85093975406627,129.354234643731));
#218565=CARTESIAN_POINT('Ctrl Pts',(153.218389218117,-4.92313233206838,
135.784421751204));
#218566=CARTESIAN_POINT('Ctrl Pts',(152.939941594304,1.52879319471521,137.638175966376));
#218567=CARTESIAN_POINT('Ctrl Pts',(152.661493970491,6.57583246125511,133.21198772643));
#218568=CARTESIAN_POINT('Ctrl Pts',(152.383046346679,5.58000294317656,126.573307792561));
#218569=CARTESIAN_POINT('Ctrl Pts',(152.104598722866,-0.543576681382813,
123.822758706449));
#218570=CARTESIAN_POINT('Ctrl Pts',(151.826151099053,-6.16763589094857,
127.487960706439));
#218571=CARTESIAN_POINT('Ctrl Pts',(151.54770347524,-6.12393902249645,134.200772209611));
#218572=CARTESIAN_POINT('Ctrl Pts',(151.269255851427,-0.452641363423277,
137.792447383624));
#218573=CARTESIAN_POINT('Ctrl Pts',(150.990808227614,5.63461159587598,134.962412206646));
#218574=CARTESIAN_POINT('Ctrl Pts',(150.712360603801,6.54393176464461,128.311330751416));
#218575=CARTESIAN_POINT('Ctrl Pts',(150.433912979988,1.4396983305442,123.951221951899));
#218576=CARTESIAN_POINT('Ctrl Pts',(150.155465356176,-4.98754753615285,
125.888812791691));
#218577=CARTESIAN_POINT('Ctrl Pts',(149.877017732362,-6.83148087236823,
132.343551945603));
#218578=CARTESIAN_POINT('Ctrl Pts',(149.59857010855,-2.39761702327129,137.383849462723));
#218579=CARTESIAN_POINT('Ctrl Pts',(149.320122484737,4.23953974010866,136.377918157044));
#218580=CARTESIAN_POINT('Ctrl Pts',(149.041674860924,6.98076659535922,130.250159756006));
#218581=CARTESIAN_POINT('Ctrl Pts',(148.763227237111,3.30700997888175,124.631684872525));
#218582=CARTESIAN_POINT('Ctrl Pts',(148.484779613298,-3.40572725176907,
124.685597446761));
#218583=CARTESIAN_POINT('Ctrl Pts',(148.206331989485,-6.98876751706998,
130.362354456768));
#218584=CARTESIAN_POINT('Ctrl Pts',(147.927884365672,-4.14947185445744,
136.445293535346));
#218585=CARTESIAN_POINT('Ctrl Pts',(147.649436741859,2.50298572943186,137.344490837378));
#218586=CARTESIAN_POINT('Ctrl Pts',(147.370989118047,6.85532170562399,132.233627970525));
#218587=CARTESIAN_POINT('Ctrl Pts',(147.092541494233,4.90795193543132,125.809338229895));
#218588=CARTESIAN_POINT('Ctrl Pts',(146.814093870421,-1.54958589664124,
123.975230043125));
#218589=CARTESIAN_POINT('Ctrl Pts',(146.535646246608,-6.58312999118006,
128.41675923269));
#218590=CARTESIAN_POINT('Ctrl Pts',(146.257198622795,-5.56709922760349,
135.052377454143));
#218591=CARTESIAN_POINT('Ctrl Pts',(145.978750998982,0.564823758223794,
137.784275729942));
#218592=CARTESIAN_POINT('Ctrl Pts',(145.700303375169,6.17770130341801,134.101973005276));
#218593=CARTESIAN_POINT('Ctrl Pts',(145.421855751356,6.11357314825767,127.389325593625));
#218594=CARTESIAN_POINT('Ctrl Pts',(145.143408127543,0.431369934500661,
123.81492853524));
#218595=CARTESIAN_POINT('Ctrl Pts',(144.864960503731,-5.64724117546963,
126.663478107772));
#218596=CARTESIAN_POINT('Ctrl Pts',(144.586512879918,-6.53631352825206,
133.317296413447));
#218597=CARTESIAN_POINT('Ctrl Pts',(144.308065256105,-1.41883306523854,
137.661849486446));
#218598=CARTESIAN_POINT('Ctrl Pts',(144.029617632292,5.00248567088053,135.704705295899));
#218599=CARTESIAN_POINT('Ctrl Pts',(143.751170008479,6.82676446047164,129.244383741109));
#218600=CARTESIAN_POINT('Ctrl Pts',(143.472722384666,2.37758021687388,124.217604726676));
#218601=CARTESIAN_POINT('Ctrl Pts',(143.194274760853,-4.25648409478009,
125.243732595056));
#218602=CARTESIAN_POINT('Ctrl Pts',(142.91582713704,-6.97904746413934,131.379805964341));
#218603=CARTESIAN_POINT('Ctrl Pts',(142.637379513228,-3.28820715937746,
136.987073172008));
#218604=CARTESIAN_POINT('Ctrl Pts',(142.358931889414,3.42433488700229,136.912729584442));
#218605=CARTESIAN_POINT('Ctrl Pts',(142.080484265602,6.99008046028611,131.225093326731));
#218606=CARTESIAN_POINT('Ctrl Pts',(141.802036641788,4.13228357498186,125.150824263232));
#218607=CARTESIAN_POINT('Ctrl Pts',(141.523589017976,-2.52288004245522,
124.271878918761));
#218608=CARTESIAN_POINT('Ctrl Pts',(141.245141394163,-6.859640150418,129.395965126019));
#218609=CARTESIAN_POINT('Ctrl Pts',(140.96669377035,-4.89272607219785,135.814297986063));
#218610=CARTESIAN_POINT('Ctrl Pts',(140.688246146537,1.57036424341533,137.628743153505));
#218611=CARTESIAN_POINT('Ctrl Pts',(140.409798522724,6.59036653588803,133.17191416004));
#218612=CARTESIAN_POINT('Ctrl Pts',(140.131350898911,5.55414393918375,126.539419122461));
#218613=CARTESIAN_POINT('Ctrl Pts',(139.852903275098,-0.586065602614643,
123.826196964908));
#218614=CARTESIAN_POINT('Ctrl Pts',(139.574455651286,-6.18770948650656,
127.525566301902));
#218615=CARTESIAN_POINT('Ctrl Pts',(139.296008027473,-6.10315063871238,
134.237987436982));
#218616=CARTESIAN_POINT('Ctrl Pts',(139.01756040366,-0.410094509425858,
137.795073267016));
#218617=CARTESIAN_POINT('Ctrl Pts',(138.739112779847,5.65981843979252,134.928035687503));
#218618=CARTESIAN_POINT('Ctrl Pts',(138.460665156034,6.52863474034383,128.271542171445));
#218619=CARTESIAN_POINT('Ctrl Pts',(138.182217532221,1.39795465605713,123.942585072312));
#218620=CARTESIAN_POINT('Ctrl Pts',(137.903769908408,-5.01737746326431,
125.919264482896));
#218621=CARTESIAN_POINT('Ctrl Pts',(137.625322284595,-6.82198480636163,
132.385108591028));
#218622=CARTESIAN_POINT('Ctrl Pts',(137.346874660782,-2.35752138489827,
137.39832253538));
#218623=CARTESIAN_POINT('Ctrl Pts',(137.06842703697,4.27338901796432,136.352007610208));
#218624=CARTESIAN_POINT('Ctrl Pts',(136.789979413157,6.9772636799772,130.20767611642));
#218625=CARTESIAN_POINT('Ctrl Pts',(136.511531789344,3.26937387837121,124.611668529527));
#218626=CARTESIAN_POINT('Ctrl Pts',(136.233084165531,-3.44291079966457,
124.706442441713));
#218627=CARTESIAN_POINT('Ctrl Pts',(135.954636541718,-6.99132864835187,
130.404905257644));
#218628=CARTESIAN_POINT('Ctrl Pts',(135.676188917905,-4.1150570145959,136.470448034864));
#218629=CARTESIAN_POINT('Ctrl Pts',(135.397741294092,2.54275098386259,137.329133279345));
#218630=CARTESIAN_POINT('Ctrl Pts',(135.11929367028,6.8638950484427,132.191871200516));
#218631=CARTESIAN_POINT('Ctrl Pts',(134.840846046466,4.87745488341857,125.779554679616));
#218632=CARTESIAN_POINT('Ctrl Pts',(134.562398422654,-1.59112804254939,
123.984789340275));
#218633=CARTESIAN_POINT('Ctrl Pts',(134.283950798841,-6.59754202834077,
128.456876850186));
#218634=CARTESIAN_POINT('Ctrl Pts',(134.005503175028,-5.54113719793324,
135.086187261361));
#218635=CARTESIAN_POINT('Ctrl Pts',(133.727055551215,0.607302017773813,
137.780708165749));
#218636=CARTESIAN_POINT('Ctrl Pts',(133.448607927402,6.19766034749954,134.064306486881));
#218637=CARTESIAN_POINT('Ctrl Pts',(133.170160303589,6.09267159041341,127.352173811322));
#218638=CARTESIAN_POINT('Ctrl Pts',(132.891712679776,0.388815285291658,
123.812432161999));
#218639=CARTESIAN_POINT('Ctrl Pts',(132.613265055963,-5.67234327233058,
126.697931188648));
#218640=CARTESIAN_POINT('Ctrl Pts',(132.334817432151,-6.52089547205522,
133.357038250242));
#218641=CARTESIAN_POINT('Ctrl Pts',(132.056369808337,-1.37706329641493,
137.670359272641));
#218642=CARTESIAN_POINT('Ctrl Pts',(131.777922184525,5.0322227753486,135.674162953708));
#218643=CARTESIAN_POINT('Ctrl Pts',(131.499474560712,6.81714195431646,129.20285619093));
#218644=CARTESIAN_POINT('Ctrl Pts',(131.221026936899,2.33744071316646,124.203253758389));
#218645=CARTESIAN_POINT('Ctrl Pts',(130.942579313086,-4.29025435305649,
125.269746047434));
#218646=CARTESIAN_POINT('Ctrl Pts',(130.664131689273,-6.97541525939744,
131.422278745477));
#218647=CARTESIAN_POINT('Ctrl Pts',(130.38568406546,-3.25051031033198,137.006974870947));
#218648=CARTESIAN_POINT('Ctrl Pts',(130.107236441647,3.46145481767177,136.891771512113));
#218649=CARTESIAN_POINT('Ctrl Pts',(129.828788817834,6.99251206970404,131.182534927744));
#218650=CARTESIAN_POINT('Ctrl Pts',(129.550341194022,4.09779233288376,125.125774627163));
#218651=CARTESIAN_POINT('Ctrl Pts',(129.271893570209,-2.5625983695722,124.287357437414));
#218652=CARTESIAN_POINT('Ctrl Pts',(128.993445946396,-6.86808636028122,
129.43774779692));
#218653=CARTESIAN_POINT('Ctrl Pts',(128.714998322583,-4.86213851056362,
135.84398857585));
#218654=CARTESIAN_POINT('Ctrl Pts',(128.43655069877,1.61187710169066,137.61905746063));
#218655=CARTESIAN_POINT('Ctrl Pts',(128.158103074957,6.60465640206541,133.131752863082));
#218656=CARTESIAN_POINT('Ctrl Pts',(127.879655451144,5.52807912434469,126.505688491336));
#218657=CARTESIAN_POINT('Ctrl Pts',(127.601207827331,-0.628532806970051,
123.829893801787));
#218658=CARTESIAN_POINT('Ctrl Pts',(127.322760203518,-6.20755379421381,
127.563293394292));
#218659=CARTESIAN_POINT('Ctrl Pts',(127.044312579706,-6.08213610043705,
134.275075430049));
#218660=CARTESIAN_POINT('Ctrl Pts',(126.765864955893,-0.367532459225645,
137.797440106979));
#218661=CARTESIAN_POINT('Ctrl Pts',(126.48741733208,5.68481555705546,134.893506364063));
#218662=CARTESIAN_POINT('Ctrl Pts',(126.208969708267,6.51309579508176,128.231847445991));
#218663=CARTESIAN_POINT('Ctrl Pts',(125.930522084454,1.35615917984635,123.934202458341));
#218664=CARTESIAN_POINT('Ctrl Pts',(125.652074460641,-5.04702146960864,
125.949897193134));
#218665=CARTESIAN_POINT('Ctrl Pts',(125.373626836828,-6.81223594919939,
132.426606661257));
#218666=CARTESIAN_POINT('Ctrl Pts',(125.095179213015,-2.3173383877032,137.412551266352));
#218667=CARTESIAN_POINT('Ctrl Pts',(124.816731589202,4.3070799438184,136.325891493273));
#218668=CARTESIAN_POINT('Ctrl Pts',(124.538283965389,6.97350221952356,130.165214587198));
#218669=CARTESIAN_POINT('Ctrl Pts',(124.259836341577,3.2316166300094,124.591881659011));
#218670=CARTESIAN_POINT('Ctrl Pts',(123.981388717764,-3.47996676923432,
124.727513397266));
#218671=CARTESIAN_POINT('Ctrl Pts',(123.702941093951,-6.99363071337966,
130.447470860486));
#218672=CARTESIAN_POINT('Ctrl Pts',(123.424493470138,-4.08048968978323,
136.495392575427));
#218673=CARTESIAN_POINT('Ctrl Pts',(123.146045846325,2.58242201572056,137.313533943462));
#218674=CARTESIAN_POINT('Ctrl Pts',(122.867598222512,6.87221404710605,132.150063015792));
#218675=CARTESIAN_POINT('Ctrl Pts',(122.589150598699,4.84677709552158,125.749957325369));
#218676=CARTESIAN_POINT('Ctrl Pts',(122.310702974886,-1.63261122862275,
123.994601339147));
#218677=CARTESIAN_POINT('Ctrl Pts',(122.032255351073,-6.6117095911554,128.497081454556));
#218678=CARTESIAN_POINT('Ctrl Pts',(121.753807727261,-5.51496983938628,
135.119838403918));
#218679=CARTESIAN_POINT('Ctrl Pts',(121.475360103447,0.649757773524084,
137.776882090432));
#218680=CARTESIAN_POINT('Ctrl Pts',(121.196912479635,6.21738973499768,134.026519169992));
#218681=CARTESIAN_POINT('Ctrl Pts',(120.918464855822,6.07154426638285,127.315149951069));
#218682=CARTESIAN_POINT('Ctrl Pts',(120.640017232009,0.346246228389124,
123.810194877238));
#218683=CARTESIAN_POINT('Ctrl Pts',(120.361569608196,-5.69723517842559,
126.732536434776));
#218684=CARTESIAN_POINT('Ctrl Pts',(120.083121984383,-6.50523578167861,
133.396685496627));
#218685=CARTESIAN_POINT('Ctrl Pts',(119.80467436057,-1.3352425000044,137.678614636731));
#218686=CARTESIAN_POINT('Ctrl Pts',(119.526226736757,5.06177340895125,135.6434401592));
#218687=CARTESIAN_POINT('Ctrl Pts',(119.247779112945,6.8072668364591,129.161387985085));
#218688=CARTESIAN_POINT('Ctrl Pts',(118.969331489131,2.29721459473369,124.189147396544));
#218689=CARTESIAN_POINT('Ctrl Pts',(118.690883865319,-4.32386563438011,
125.29596458699));
#218690=CARTESIAN_POINT('Ctrl Pts',(118.412436241506,-6.97152457807781,
131.464728629428));
#218691=CARTESIAN_POINT('Ctrl Pts',(118.133988617693,-3.21269301243169,
137.026646729736));
#218692=CARTESIAN_POINT('Ctrl Pts',(117.85554099388,3.49844648286018,136.870587868534));
#218693=CARTESIAN_POINT('Ctrl Pts',(117.577093370067,6.99468456901571,131.139962515369));
#218694=CARTESIAN_POINT('Ctrl Pts',(117.298645746254,4.06314924558364,125.100935413187));
#218695=CARTESIAN_POINT('Ctrl Pts',(117.020198122441,-2.60222173866402,
124.303077446017));
#218696=CARTESIAN_POINT('Ctrl Pts',(116.741750498628,-6.8762780706787,129.479581108162));
#218697=CARTESIAN_POINT('Ctrl Pts',(116.463302874816,-4.83137078059878,
135.873492420371));
#218698=CARTESIAN_POINT('Ctrl Pts',(116.184855251003,1.65333023126747,137.609119246659));
#218699=CARTESIAN_POINT('Ctrl Pts',(115.90640762719,6.61870153027093,133.09150532375));
#218700=CARTESIAN_POINT('Ctrl Pts',(115.627960003377,5.5018094645007,126.472117149089));
#218701=CARTESIAN_POINT('Ctrl Pts',(115.349512379564,-0.670976720811003,
123.833849080098));
#218702=CARTESIAN_POINT('Ctrl Pts',(115.071064755751,-6.22716807873245,
127.601140585621));
#218703=CARTESIAN_POINT('Ctrl Pts',(114.792617131938,-6.06089618637186,
134.312034814502));
#218704=CARTESIAN_POINT('Ctrl Pts',(114.514169508125,-0.324956789974863,
137.79954781581));
#218705=CARTESIAN_POINT('Ctrl Pts',(114.235721884312,5.70960202138734,134.858825515823));
#218706=CARTESIAN_POINT('Ctrl Pts',(113.957274260499,6.4973155046598,128.192248045959));
#218707=CARTESIAN_POINT('Ctrl Pts',(113.678826636687,1.31431345065849,123.926074420608));
#218708=CARTESIAN_POINT('Ctrl Pts',(113.400379012874,-5.07647845671644,
125.980709787299));
#218709=CARTESIAN_POINT('Ctrl Pts',(113.121931389061,-6.80223466212876,
132.468044618562));
#218710=CARTESIAN_POINT('Ctrl Pts',(112.843483765248,-2.27706952068197,
137.42653512839));
#218711=CARTESIAN_POINT('Ctrl Pts',(112.565036141435,4.34061126924124,136.299570773982));
#218712=CARTESIAN_POINT('Ctrl Pts',(112.286588517622,6.96948235338073,130.122776741767));
#218713=CARTESIAN_POINT('Ctrl Pts',(112.008140893809,3.1937396329048,124.572324994188));
#218714=CARTESIAN_POINT('Ctrl Pts',(111.729693269996,-3.51689378735575,
124.748809532627));
#218715=CARTESIAN_POINT('Ctrl Pts',(111.451245646184,-6.99567362684944,
130.490049688009));
#218716=CARTESIAN_POINT('Ctrl Pts',(111.172798022371,-4.0457711609245,136.52012623271));
#218717=CARTESIAN_POINT('Ctrl Pts',(110.894350398558,2.62199735498092,137.297693407768));
#218718=CARTESIAN_POINT('Ctrl Pts',(110.615902774745,6.88027839335069,132.108204965571));
#218719=CARTESIAN_POINT('Ctrl Pts',(110.337455150932,4.81591970851693,125.720547263895));
#218720=CARTESIAN_POINT('Ctrl Pts',(110.059007527119,-1.67403391768677,
124.004665676154));
#218721=CARTESIAN_POINT('Ctrl Pts',(109.780559903306,-6.62563215463966,
128.537371556004));
#218722=CARTESIAN_POINT('Ctrl Pts',(109.502112279493,-5.48859812160383,
135.153329634858));
#218723=CARTESIAN_POINT('Ctrl Pts',(109.22366465568,0.692189452261082,137.772797645767));
#218724=CARTESIAN_POINT('Ctrl Pts',(108.945217031867,6.23688873483282,133.988612454835));
#218725=CARTESIAN_POINT('Ctrl Pts',(108.666769408055,6.05019195904657,127.278255384801));
#218726=CARTESIAN_POINT('Ctrl Pts',(108.388321784241,0.303664341205276,
123.808216763862));
#218727=CARTESIAN_POINT('Ctrl Pts',(108.109874160429,-5.72191597137591,
126.767292563848));
#218728=CARTESIAN_POINT('Ctrl Pts',(107.831426536616,-6.48933503739778,
133.436236683461));
#218729=CARTESIAN_POINT('Ctrl Pts',(107.552978912803,-1.29337222569216,
137.68661527281));
#218730=CARTESIAN_POINT('Ctrl Pts',(107.27453128899,5.09113647667873,135.612538050821));
#218731=CARTESIAN_POINT('Ctrl Pts',(106.996083665177,6.79713947282576,129.119980660195));
#218732=CARTESIAN_POINT('Ctrl Pts',(106.717636041364,2.25690335216928,124.175286163858));
#218733=CARTESIAN_POINT('Ctrl Pts',(106.439188417551,-4.35731669327239,
125.322387242187));
#218734=CARTESIAN_POINT('Ctrl Pts',(106.160740793739,-6.96737556435125,
131.5071540432));
#218735=CARTESIAN_POINT('Ctrl Pts',(105.882293169926,-3.17475666701035,
137.046088019424));
#218736=CARTESIAN_POINT('Ctrl Pts',(105.603845546113,3.53530851182771,136.849179438675));
#218737=CARTESIAN_POINT('Ctrl Pts',(105.3253979223,6.99659787771835,131.097377667143));
#218738=CARTESIAN_POINT('Ctrl Pts',(105.046950298487,4.02835559679407,125.076307541727));
#218739=CARTESIAN_POINT('Ctrl Pts',(104.768502674674,-2.64174868147234,
124.319038362058));
#218740=CARTESIAN_POINT('Ctrl Pts',(104.490055050861,-6.88421497806359,
129.521463509594));
#218741=CARTESIAN_POINT('Ctrl Pts',(104.211607427049,-4.80042402241278,
135.902808426348));
#218742=CARTESIAN_POINT('Ctrl Pts',(103.933159803235,1.69472209608453,137.598928879852));
#218743=CARTESIAN_POINT('Ctrl Pts',(103.654712179423,6.63250140005722,133.051173033428));
#218744=CARTESIAN_POINT('Ctrl Pts',(103.37626455561,5.47533593308374,126.438706339714));
#218745=CARTESIAN_POINT('Ctrl Pts',(103.097816931797,-0.713395771362793,
123.838062653278));
#218746=CARTESIAN_POINT('Ctrl Pts',(102.819369307984,-6.24655161324796,
127.639106473447));
#218747=CARTESIAN_POINT('Ctrl Pts',(102.540921684171,-6.03943168356949,
134.348864220799));
#218748=CARTESIAN_POINT('Ctrl Pts',(102.262474060358,-0.282369079330704,
137.801396315408));
#218749=CARTESIAN_POINT('Ctrl Pts',(101.984026436545,5.73417691431645,134.823994427897));
#218750=CARTESIAN_POINT('Ctrl Pts',(101.705578812732,6.48129445382252,128.15274543872));
#218751=CARTESIAN_POINT('Ctrl Pts',(101.427131188919,1.27241901910234,123.9182012603));
#218752=CARTESIAN_POINT('Ctrl Pts',(101.148683565106,-5.1057473330482,126.01170112362));
#218753=CARTESIAN_POINT('Ctrl Pts',(100.870235941294,-6.7919813157512,132.509420927444));
#218754=CARTESIAN_POINT('Ctrl Pts',(100.591788317481,-2.23671627601227,
137.440273603317));
#218755=CARTESIAN_POINT('Ctrl Pts',(100.313340693668,4.37398175171709,136.273046427655));
#218756=CARTESIAN_POINT('Ctrl Pts',(100.034893069855,6.96520423050629,130.080364152676));
#218757=CARTESIAN_POINT('Ctrl Pts',(99.7564454460421,3.15574429060373,124.552999259737));
#218758=CARTESIAN_POINT('Ctrl Pts',(99.4779978222292,-3.55369048568456,
124.770330058661));
#218759=CARTESIAN_POINT('Ctrl Pts',(99.1995501984162,-6.99745731306031,
130.532640162439));
#218760=CARTESIAN_POINT('Ctrl Pts',(98.9211025746034,-4.01090271452764,
136.544648090195));
#218761=CARTESIAN_POINT('Ctrl Pts',(98.6426549507905,2.66147553516503,137.281612259238));
#218762=CARTESIAN_POINT('Ctrl Pts',(98.3642073269776,6.88808778834931,132.066298600918));
#218763=CARTESIAN_POINT('Ctrl Pts',(98.0857597031646,4.78488386583629,125.691325584995));
#218764=CARTESIAN_POINT('Ctrl Pts',(97.8073120793519,-1.71539457480834,
124.014981978356));
#218765=CARTESIAN_POINT('Ctrl Pts',(97.5288644555388,-6.63930920288774,
128.577745661565));
#218766=CARTESIAN_POINT('Ctrl Pts',(97.2504168317261,-5.46202302179963,
135.186659713151));
#218767=CARTESIAN_POINT('Ctrl Pts',(96.9719692079131,0.734595481663425,
137.768454983106));
#218768=CARTESIAN_POINT('Ctrl Pts',(96.6935215841003,6.25615662446226,133.950587746053));
#218769=CARTESIAN_POINT('Ctrl Pts',(96.4150739602873,6.0286154596223,127.24149147966));
#218770=CARTESIAN_POINT('Ctrl Pts',(96.1366263364746,0.26107120162757,123.806497895168));
#218771=CARTESIAN_POINT('Ctrl Pts',(95.8581787126614,-5.74638473662552,
126.80219828796));
#218772=CARTESIAN_POINT('Ctrl Pts',(95.5797310888487,-6.47319382842077,
133.47569034516));
#218773=CARTESIAN_POINT('Ctrl Pts',(95.3012834650358,-1.25145402499642,
137.694360884412));
#218774=CARTESIAN_POINT('Ctrl Pts',(95.0228358412229,5.12031089047184,135.581457773658));
#218775=CARTESIAN_POINT('Ctrl Pts',(94.7443882174101,6.78676023868958,129.078635750625));
#218776=CARTESIAN_POINT('Ctrl Pts',(94.465940593597,2.21650847922131,124.161670573963));
#218777=CARTESIAN_POINT('Ctrl Pts',(94.1874929697842,-4.39060629019222,
125.349013033923));
#218778=CARTESIAN_POINT('Ctrl Pts',(93.9090453459715,-6.96296837196094,
131.549553414704));
#218779=CARTESIAN_POINT('Ctrl Pts',(93.6305977221583,-3.13670267981308,
137.065298019608));
#218780=CARTESIAN_POINT('Ctrl Pts',(93.3521500983456,3.5720395386382,136.82754701583));
#218781=CARTESIAN_POINT('Ctrl Pts',(93.0737024745325,6.99825192491364,131.054781961061));
#218782=CARTESIAN_POINT('Ctrl Pts',(92.7952548507199,3.99341267580637,125.051891925383));
#218783=CARTESIAN_POINT('Ctrl Pts',(92.5168072269068,-2.68117773331193,
124.335239594101));
#218784=CARTESIAN_POINT('Ctrl Pts',(92.238359603094,-6.89189678833074,129.563393449252));
#218785=CARTESIAN_POINT('Ctrl Pts',(91.959911979281,-4.7692993827493,135.931935507467));
#218786=CARTESIAN_POINT('Ctrl Pts',(91.6814643554683,1.73605116235111,137.588486737821));
#218787=CARTESIAN_POINT('Ctrl Pts',(91.4030167316553,6.6460555000649,133.010757486647));
#218788=CARTESIAN_POINT('Ctrl Pts',(91.1245691078424,5.44865951108031,126.405457301267));
#218789=CARTESIAN_POINT('Ctrl Pts',(90.8461214840295,-0.755788386771977,
123.84253436519));
#218790=CARTESIAN_POINT('Ctrl Pts',(90.5676738602166,-6.26570367949625,
127.677189650927));
#218791=CARTESIAN_POINT('Ctrl Pts',(90.2892262364038,-6.01774338740505,
134.38556228421));
#218792=CARTESIAN_POINT('Ctrl Pts',(90.0107786125907,-0.239770905396614,
137.802985537273));
#218793=CARTESIAN_POINT('Ctrl Pts',(89.7323309887781,5.75853932521132,134.78901439096));
#218794=CARTESIAN_POINT('Ctrl Pts',(89.453883364965,6.46503323623579,128.113341088056));
#218795=CARTESIAN_POINT('Ctrl Pts',(89.1754357411521,1.23047743759138,123.910583269158));
#218796=CARTESIAN_POINT('Ctrl Pts',(88.8969881173393,-5.13482701403487,
126.042870053701));
#218797=CARTESIAN_POINT('Ctrl Pts',(88.6185404935264,-6.78147629000823,
132.550734054689));
#218798=CARTESIAN_POINT('Ctrl Pts',(88.3400928697134,-2.19628014899849,
137.453766182047));
#218799=CARTESIAN_POINT('Ctrl Pts',(88.0616452459006,4.4071901546906,136.246319437167));
#218800=CARTESIAN_POINT('Ctrl Pts',(87.7831976220877,6.96066800942769,130.037978391542));
#218801=CARTESIAN_POINT('Ctrl Pts',(87.5047499982748,3.1176320110373,124.533905171779));
#218802=CARTESIAN_POINT('Ctrl Pts',(87.2263023744621,-3.59035550070555,
124.792074177916));
#218803=CARTESIAN_POINT('Ctrl Pts',(86.9478547506488,-6.99898170591706,
130.57524070557));
#218804=CARTESIAN_POINT('Ctrl Pts',(86.6694071268362,-3.97588564265574,
136.568957239218));
#218805=CARTESIAN_POINT('Ctrl Pts',(86.3909595030232,2.70085509339449,137.265291093768));
#218806=CARTESIAN_POINT('Ctrl Pts',(86.1125118792103,6.89564194272181,132.024345474689));
#218807=CARTESIAN_POINT('Ctrl Pts',(85.8340642553976,4.75367071752436,125.662293371487));
#218808=CARTESIAN_POINT('Ctrl Pts',(85.5556166315845,-1.75669166735309,
124.025549863481));
#218809=CARTESIAN_POINT('Ctrl Pts',(85.2771690077717,-6.65274022909182,
128.618202275162));
#218810=CARTESIAN_POINT('Ctrl Pts',(84.9987213839588,-5.4352455247236,135.21982740374));
#218811=CARTESIAN_POINT('Ctrl Pts',(84.7202737601459,0.776974290360158,
137.763854263368));
#218812=CARTESIAN_POINT('Ctrl Pts',(84.4418261363329,6.27519268990729,133.912446452669));
#218813=CARTESIAN_POINT('Ctrl Pts',(84.1633785125202,6.00681556763514,127.204859597945));
#218814=CARTESIAN_POINT('Ctrl Pts',(83.8849308887072,0.218468387960617,
123.805038334852));
#218815=CARTESIAN_POINT('Ctrl Pts',(83.6064832648944,-5.77064056747553,
126.837252313669));
#218816=CARTESIAN_POINT('Ctrl Pts',(83.3280356410814,-6.45681275286598,
133.515045019753));
#218817=CARTESIAN_POINT('Ctrl Pts',(83.0495880172686,-1.20948945121144,
137.701851184522));
#218818=CARTESIAN_POINT('Ctrl Pts',(82.7711403934555,5.14929556926191,135.550200479404));
#218819=CARTESIAN_POINT('Ctrl Pts',(82.4926927696429,6.77612951865689,129.037354788424));
#218820=CARTESIAN_POINT('Ctrl Pts',(82.2142451458298,2.17603147273656,124.148301131391));
#218821=CARTESIAN_POINT('Ctrl Pts',(81.9357975220171,-4.42373319158141,
125.375840975569));
#218822=CARTESIAN_POINT('Ctrl Pts',(81.6573498982041,-6.95830316421689,
131.591925172815));
#218823=CARTESIAN_POINT('Ctrl Pts',(81.3789022743912,-3.09853246094448,
137.084276018453));
#218824=CARTESIAN_POINT('Ctrl Pts',(81.1004546505783,3.60863820220999,136.805691401599));
#218825=CARTESIAN_POINT('Ctrl Pts',(80.8220070267654,6.99964664931016,131.012176975526));
#218826=CARTESIAN_POINT('Ctrl Pts',(80.5435594029525,3.95832177744353,125.02768946888));
#218827=CARTESIAN_POINT('Ctrl Pts',(80.2651117791397,-2.72050743312451,
124.351680541802));
#218828=CARTESIAN_POINT('Ctrl Pts',(79.9866641553267,-6.89932321682792,
129.605369373404));
#218829=CARTESIAN_POINT('Ctrl Pts',(79.7082165315139,-4.73799801494326,
135.960872584412));
#218830=CARTESIAN_POINT('Ctrl Pts',(79.4297689077009,1.77731589860328,137.577793207502));
#218831=CARTESIAN_POINT('Ctrl Pts',(79.1513212838881,6.65936332804202,132.970260181018));
#218832=CARTESIAN_POINT('Ctrl Pts',(78.8728736600752,5.42178118699497,126.372371265798));
#218833=CARTESIAN_POINT('Ctrl Pts',(78.5944260362623,-0.798152996164653,
123.847264050135));
#218834=CARTESIAN_POINT('Ctrl Pts',(78.3159784124494,-6.28462356779051,
127.715388706879));
#218835=CARTESIAN_POINT('Ctrl Pts',(78.0375307886365,-5.99583210154638,
134.422127644877));
#218836=CARTESIAN_POINT('Ctrl Pts',(77.7590831648237,-0.197163846663491,
137.804315422519));
#218837=CARTESIAN_POINT('Ctrl Pts',(77.4806355410107,5.78268835131386,134.753886701214));
#218838=CARTESIAN_POINT('Ctrl Pts',(77.2021879171979,6.44853245446487,128.07403645411));
#218839=CARTESIAN_POINT('Ctrl Pts',(76.9237402933849,1.18849026028645,123.903220729472));
#218840=CARTESIAN_POINT('Ctrl Pts',(76.6452926695721,-5.16371642211823,
126.074215422566));
#218841=CARTESIAN_POINT('Ctrl Pts',(76.3668450457591,-6.77071997416741,
132.591982469425));
#218842=CARTESIAN_POINT('Ctrl Pts',(76.0883974219463,-2.15576263801617,
137.467012364608));
#218843=CARTESIAN_POINT('Ctrl Pts',(75.8099497981334,4.44023524761227,136.219390792892));
#218844=CARTESIAN_POINT('Ctrl Pts',(75.5315021743204,6.95587385823614,129.995621028982));
#218845=CARTESIAN_POINT('Ctrl Pts',(75.2530545505077,3.0794042064702,124.515043437855));
#218846=CARTESIAN_POINT('Ctrl Pts',(74.9746069266946,-3.62688747378295,
124.814041084656));
#218847=CARTESIAN_POINT('Ctrl Pts',(74.6961593028819,-7.0002467489329,130.617849738824));
#218848=CARTESIAN_POINT('Ctrl Pts',(74.4177116790688,-3.94072124287924,
136.593052778991));
#218849=CARTESIAN_POINT('Ctrl Pts',(74.1392640552561,2.74013457044532,137.248730516143));
#218850=CARTESIAN_POINT('Ctrl Pts',(73.860816431443,6.90294057654623,131.982347141473));
#218851=CARTESIAN_POINT('Ctrl Pts',(73.5823688076304,4.72228142019582,125.633451699173));
#218852=CARTESIAN_POINT('Ctrl Pts',(73.3039211838172,-1.79792366504193,
124.036368939932));
#218853=CARTESIAN_POINT('Ctrl Pts',(73.0254735600045,-6.66592473556012,
128.658739897661));
#218854=CARTESIAN_POINT('Ctrl Pts',(72.7470259361915,-5.40826662262595,
135.252831477583));
#218855=CARTESIAN_POINT('Ctrl Pts',(72.4685783123786,0.819324307988826,
137.758995657032));
#218856=CARTESIAN_POINT('Ctrl Pts',(72.1901306885658,6.2939962257795,133.87418998802));
#218857=CARTESIAN_POINT('Ctrl Pts',(71.9116830647529,5.98479309088811,127.168361097063));
#218858=CARTESIAN_POINT('Ctrl Pts',(71.63323544094,0.17585747886725,123.803838136996));
#218859=CARTESIAN_POINT('Ctrl Pts',(71.3547878171271,-5.79468256511725,
126.872453342036));
#218860=CARTESIAN_POINT('Ctrl Pts',(71.0763401933142,-6.44019241774003,
133.554299248939));
#218861=CARTESIAN_POINT('Ctrl Pts',(70.7978925695013,-1.16748005934989,
137.709085895581));
#218862=CARTESIAN_POINT('Ctrl Pts',(70.5194449456884,5.17808943901089,135.518767326308));
#218863=CARTESIAN_POINT('Ctrl Pts',(70.2409973218756,6.76524770665308,128.996139303274));
#218864=CARTESIAN_POINT('Ctrl Pts',(69.9625496980626,2.1354738326052,124.135178331551));
#218865=CARTESIAN_POINT('Ctrl Pts',(69.6841020742497,-4.45669616991057,
125.402870073008));
#218866=CARTESIAN_POINT('Ctrl Pts',(69.4056544504369,-6.95338011399016,
131.634267747431));
#218867=CARTESIAN_POINT('Ctrl Pts',(69.1272068266238,-3.06024742481583,
137.103021312725));
#218868=CARTESIAN_POINT('Ctrl Pts',(68.8487592028112,3.64510314636624,136.783613405848));
#218869=CARTESIAN_POINT('Ctrl Pts',(68.5703115789981,7.00078199922599,130.969564289278));
#218870=CARTESIAN_POINT('Ctrl Pts',(68.2918639551854,3.92308420201135,125.003701069051));
#218871=CARTESIAN_POINT('Ctrl Pts',(68.0134163313723,-2.75973632353393,
124.368360595937));
#218872=CARTESIAN_POINT('Ctrl Pts',(67.7349687075595,-6.90649398836592,
129.647389726619));
#218873=CARTESIAN_POINT('Ctrl Pts',(67.4565210837467,-4.70652107887851,
135.98961858491));
#218874=CARTESIAN_POINT('Ctrl Pts',(67.1780734599337,1.81851477576126,137.566848685147));
#218875=CARTESIAN_POINT('Ctrl Pts',(66.8996258361208,6.67242439086218,132.929682617185));
#218876=CARTESIAN_POINT('Ctrl Pts',(66.6211782123079,5.39470195681365,126.339449459324));
#218877=CARTESIAN_POINT('Ctrl Pts',(66.3427305884951,-0.840488029704522,
123.852251532852));
#218878=CARTESIAN_POINT('Ctrl Pts',(66.0642829646821,-6.30331057704718,
127.753702225821));
#218879=CARTESIAN_POINT('Ctrl Pts',(65.7858353408693,-5.97369863792435,
134.458558947856));
#218880=CARTESIAN_POINT('Ctrl Pts',(65.5073877170563,-0.154549481951222,
137.805385921867));
#218881=CARTESIAN_POINT('Ctrl Pts',(65.2289400932435,5.80662309777304,134.718612660325));
#218882=CARTESIAN_POINT('Ctrl Pts',(64.9504924694306,6.43179271995227,128.03483299333));
#218883=CARTESIAN_POINT('Ctrl Pts',(64.6720448456177,1.14645904303803,123.896113914062));
#218884=CARTESIAN_POINT('Ctrl Pts',(64.3935972218049,-5.19241448679041,
126.1057360687));
#218885=CARTESIAN_POINT('Ctrl Pts',(64.1151495979918,-6.75971276680813,
132.633164643176));
#218886=CARTESIAN_POINT('Ctrl Pts',(63.8367019741791,-2.11516524445634,
137.480011660159));
#218887=CARTESIAN_POINT('Ctrl Pts',(63.5582543503661,4.47311580598391,136.192261492683));
#218888=CARTESIAN_POINT('Ctrl Pts',(63.2798067265533,6.95082195458075,129.953293634565));
#218889=CARTESIAN_POINT('Ctrl Pts',(63.0013591027403,3.041062293448,124.496414756892));
#218890=CARTESIAN_POINT('Ctrl Pts',(62.7229114789275,-3.66328505121137,
124.836229964889));
#218891=CARTESIAN_POINT('Ctrl Pts',(62.4444638551145,-7.00125239523119,
130.660465683307));
#218892=CARTESIAN_POINT('Ctrl Pts',(62.1660162313017,-3.90541081822766,
136.616933816649));
#218893=CARTESIAN_POINT('Ctrl Pts',(61.8875686074887,2.77931251080179,137.231931140021));
#218894=CARTESIAN_POINT('Ctrl Pts',(61.609120983676,6.909983419369,131.940305157533));
#218895=CARTESIAN_POINT('Ctrl Pts',(61.3306733598629,4.69071713699276,125.604801636791));
#218896=CARTESIAN_POINT('Ctrl Pts',(61.0522257360502,-1.83908904000824,
124.047438806804));
#218897=CARTESIAN_POINT('Ctrl Pts',(60.7737781122372,-6.67886223373588,
128.699357026925));
#218898=CARTESIAN_POINT('Ctrl Pts',(60.4953304884244,-5.38108731521968,
135.285670711703));
#218899=CARTESIAN_POINT('Ctrl Pts',(60.2168828646114,0.861643965253713,
137.753879344138));
#218900=CARTESIAN_POINT('Ctrl Pts',(59.9384352407986,6.31256653530686,133.835819769716));
#218901=CARTESIAN_POINT('Ctrl Pts',(59.6599876169856,5.96254884543232,127.131997329482));
#218902=CARTESIAN_POINT('Ctrl Pts',(59.3815399931728,0.133240053310041,
123.802897346075));
#218903=CARTESIAN_POINT('Ctrl Pts',(59.1030923693598,-5.81850983866561,
126.907800068673));
#218904=CARTESIAN_POINT('Ctrl Pts',(58.824644745547,-6.42333343891552,133.593451578138));
#218905=CARTESIAN_POINT('Ctrl Pts',(58.5461971217341,-1.12542740608588,
137.716064749505));
#218906=CARTESIAN_POINT('Ctrl Pts',(58.2677494979212,5.20669143275151,135.487159479138));
#218907=CARTESIAN_POINT('Ctrl Pts',(57.9893018741083,6.75411520590753,128.954990822428));
#218908=CARTESIAN_POINT('Ctrl Pts',(57.7108542502954,2.09483706170563,124.122302660713));
#218909=CARTESIAN_POINT('Ctrl Pts',(57.4324066264825,-4.48949400372376,
125.430099324666));
#218910=CARTESIAN_POINT('Ctrl Pts',(57.1539590026696,-6.94819940370625,
131.676579569534));
#218911=CARTESIAN_POINT('Ctrl Pts',(56.8755113788568,-3.02184899009409,
137.121533207807));
#218912=CARTESIAN_POINT('Ctrl Pts',(56.5970637550437,3.68143301988451,136.761313846687));
#218913=CARTESIAN_POINT('Ctrl Pts',(56.318616131231,7.00165793259049,130.926945481348));
#218914=CARTESIAN_POINT('Ctrl Pts',(56.040168507418,3.88770125525153,124.979927614796));
#218915=CARTESIAN_POINT('Ctrl Pts',(55.7617208836052,-2.79886295089852,
124.385279138419));
#218916=CARTESIAN_POINT('Ctrl Pts',(55.4832732597923,-6.91340883722955,
129.689452951814));
#218917=CARTESIAN_POINT('Ctrl Pts',(55.2048256359794,-4.67486974094423,
136.018172443767));
#218918=CARTESIAN_POINT('Ctrl Pts',(54.9263780121665,1.85964626718557,137.555653576309));
#218919=CARTESIAN_POINT('Ctrl Pts',(54.6479303883536,6.68523820454244,132.889026298762));
#218920=CARTESIAN_POINT('Ctrl Pts',(54.3694827645407,5.36742282396772,126.306693101776));
#218921=CARTESIAN_POINT('Ctrl Pts',(54.0910351407278,-0.882791918651148,
123.857496628527));
#218922=CARTESIAN_POINT('Ctrl Pts',(53.8125875169149,-6.32176401481248,
127.792128788032));
#218923=CARTESIAN_POINT('Ctrl Pts',(53.534139893102,-5.95134381670231,134.494854843172));
#218924=CARTESIAN_POINT('Ctrl Pts',(53.2556922692892,-0.111929390351441,
137.806196995646));
#218925=CARTESIAN_POINT('Ctrl Pts',(52.9772446454762,5.83034267767769,134.683193575387));
#218926=CARTESIAN_POINT('Ctrl Pts',(52.6987970216634,6.41481465299549,127.995732158415));
#218927=CARTESIAN_POINT('Ctrl Pts',(52.4203493978505,1.10438534332797,123.889263086274));
#218928=CARTESIAN_POINT('Ctrl Pts',(52.1419017740376,-5.22092014463445,
126.137430824095));
#218929=CARTESIAN_POINT('Ctrl Pts',(51.8634541502246,-6.74845507580631,
132.674279049921));
#218930=CARTESIAN_POINT('Ctrl Pts',(51.5850065264118,-2.07448947267055,
137.492763587005));
#218931=CARTESIAN_POINT('Ctrl Pts',(51.3065589025989,4.50583061140446,136.164932541826));
#218932=CARTESIAN_POINT('Ctrl Pts',(51.028111278786,6.94551248566166,129.910997776748));
#218933=CARTESIAN_POINT('Ctrl Pts',(50.7496636549731,3.00260769274395,124.478019819181));
#218934=CARTESIAN_POINT('Ctrl Pts',(50.4712160311602,-3.69954688426507,
124.858639996399));
#218935=CARTESIAN_POINT('Ctrl Pts',(50.1927684073473,-7.00199860754717,
130.70308695987));
#218936=CARTESIAN_POINT('Ctrl Pts',(49.9143207835345,-3.86995567714208,
136.640599467269));
#218937=CARTESIAN_POINT('Ctrl Pts',(49.6358731597215,2.81838746271124,137.214893587909));
#218938=CARTESIAN_POINT('Ctrl Pts',(49.3574255359087,6.91677021021505,131.89822108075));
#218939=CARTESIAN_POINT('Ctrl Pts',(49.0789779120958,4.65897903754105,125.576344245977));
#218940=CARTESIAN_POINT('Ctrl Pts',(48.8005302882828,-1.88018626685394,
124.058759053897));
#218941=CARTESIAN_POINT('Ctrl Pts',(48.5220826644701,-6.69155224421552,
128.740052157871));
#218942=CARTESIAN_POINT('Ctrl Pts',(48.243635040657,-5.35370860964396,135.318343889229));
#218943=CARTESIAN_POINT('Ctrl Pts',(47.9651874168443,0.903931693984841,
137.748505514272));
#218944=CARTESIAN_POINT('Ctrl Pts',(47.6867397930313,6.33090293035988,133.797337219578));
#218945=CARTESIAN_POINT('Ctrl Pts',(47.4082921692184,5.94008365553619,127.095769642671));
#218946=CARTESIAN_POINT('Ctrl Pts',(47.1298445454056,0.0906176904940206,
123.80221599695));
#218947=CARTESIAN_POINT('Ctrl Pts',(46.8513969215926,-5.84212150519187,
126.943291183793));
#218948=CARTESIAN_POINT('Ctrl Pts',(46.5729492977799,-6.40623644110861,
133.632500556544));
#218949=CARTESIAN_POINT('Ctrl Pts',(46.2945016739667,-1.08333304969514,
137.722787487691));
#218950=CARTESIAN_POINT('Ctrl Pts',(46.016054050154,5.23510049062639,135.455378109134));
#218951=CARTESIAN_POINT('Ctrl Pts',(45.737606426341,6.7427324289391,128.913910870662));
#218952=CARTESIAN_POINT('Ctrl Pts',(45.4591588025282,2.0541226658487,124.10967459599));
#218953=CARTESIAN_POINT('Ctrl Pts',(45.1807111787153,-4.5221254776858,125.457527721552));
#218954=CARTESIAN_POINT('Ctrl Pts',(44.9022635549024,-6.94276122533821,
131.718859071242));
#218955=CARTESIAN_POINT('Ctrl Pts',(44.6238159310895,-2.98333857964632,
137.139811017737));
#218956=CARTESIAN_POINT('Ctrl Pts',(44.3453683072766,3.71762647654865,136.738793550433));
#218957=CARTESIAN_POINT('Ctrl Pts',(44.0669206834637,7.00227441694529,130.88432213099));
#218958=CARTESIAN_POINT('Ctrl Pts',(43.7884730596509,3.85217424829189,124.956369987047));
#218959=CARTESIAN_POINT('Ctrl Pts',(43.5100254358379,-2.8378858653675,124.402435542326));
#218960=CARTESIAN_POINT('Ctrl Pts',(43.2315778120251,-6.92006750718621,
129.731557490323));
#218961=CARTESIAN_POINT('Ctrl Pts',(42.9531301882121,-4.64304517399252,
136.04653310291));
#218962=CARTESIAN_POINT('Ctrl Pts',(42.6746825643993,1.90070884873357,137.544208295828));
#218963=CARTESIAN_POINT('Ctrl Pts',(42.3962349405864,6.69780429426274,132.848292732287));
#218964=CARTESIAN_POINT('Ctrl Pts',(42.1177873167735,5.33994479929498,126.274103406951));
#218965=CARTESIAN_POINT('Ctrl Pts',(41.8393396929606,-0.925063095418803,
123.862999142802));
#218966=CARTESIAN_POINT('Ctrl Pts',(41.5608920691476,-6.33998319728738,
127.8306669696));
#218967=CARTESIAN_POINT('Ctrl Pts',(41.2824444453348,-5.92876846624656,
134.531013985867));
#218968=CARTESIAN_POINT('Ctrl Pts',(41.0039968215219,-0.069305151166692,
137.806748613804));
#218969=CARTESIAN_POINT('Ctrl Pts',(40.725549197709,5.85384621209049,134.647630758868));
#218970=CARTESIAN_POINT('Ctrl Pts',(40.4471015738961,6.39759888272248,127.956735398261));
#218971=CARTESIAN_POINT('Ctrl Pts',(40.1686539500832,1.06227072021291,123.882668499967));
#218972=CARTESIAN_POINT('Ctrl Pts',(39.8902063262704,-5.24923233936253,
126.169298514289));
#218973=CARTESIAN_POINT('Ctrl Pts',(39.6117587024575,-6.73694731831984,
132.715324166149));
#218974=CARTESIAN_POINT('Ctrl Pts',(39.3333110786445,-2.03373682991476,
137.505267672621));
#218975=CARTESIAN_POINT('Ctrl Pts',(39.0548634548317,4.53837845161457,136.137404953004));
#218976=CARTESIAN_POINT('Ctrl Pts',(38.7764158310188,6.9399456482232,129.86873502282));
#218977=CARTESIAN_POINT('Ctrl Pts',(38.4979682072059,2.96404182930761,124.459859306355));
#218978=CARTESIAN_POINT('Ctrl Pts',(38.219520583393,-3.73567162924815,124.881270348773));
#218979=CARTESIAN_POINT('Ctrl Pts',(37.9410729595801,-7.00248535822977,
130.745711989165));
#218980=CARTESIAN_POINT('Ctrl Pts',(37.6626253357672,-3.83435713342598,
136.664048853912));
#218981=CARTESIAN_POINT('Ctrl Pts',(37.3841777119543,2.8573579782368,137.197618491141));
#218982=CARTESIAN_POINT('Ctrl Pts',(37.1057300881414,6.92330069759731,131.856096470565));
#218983=CARTESIAN_POINT('Ctrl Pts',(36.8272824643285,4.62706829790778,125.548080581235));
#218984=CARTESIAN_POINT('Ctrl Pts',(36.5488348405156,-1.92121382270608,
124.070329261737));
#218985=CARTESIAN_POINT('Ctrl Pts',(36.2703872167028,-6.70399429676593,
128.780823782526));
#218986=CARTESIAN_POINT('Ctrl Pts',(35.9919395928899,-5.32613152042688,
135.350849799446));
#218987=CARTESIAN_POINT('Ctrl Pts',(35.7134919690769,0.946185927194629,
137.742874366562));
#218988=CARTESIAN_POINT('Ctrl Pts',(35.4350443452641,6.34900473147662,133.758743763591));
#218989=CARTESIAN_POINT('Ctrl Pts',(35.1565967214512,5.91739835365575,127.059679379064));
#218990=CARTESIAN_POINT('Ctrl Pts',(34.8781490976383,0.0479919698059151,
123.80179411487));
#218991=CARTESIAN_POINT('Ctrl Pts',(34.5997014738253,-5.8655166897575,126.978925372262));
#218992=CARTESIAN_POINT('Ctrl Pts',(34.3212538500126,-6.38890205785425,
133.671444737187));
#218993=CARTESIAN_POINT('Ctrl Pts',(34.0428062261996,-1.04119854999986,
137.729253861025));
#218994=CARTESIAN_POINT('Ctrl Pts',(33.7643586023867,5.26331555992738,135.423424393967));
#218995=CARTESIAN_POINT('Ctrl Pts',(33.4859109785738,6.73109979754094,128.872900970206));
#218996=CARTESIAN_POINT('Ctrl Pts',(33.207463354761,2.01333215372067,124.097294605319));
#218997=CARTESIAN_POINT('Ctrl Pts',(32.9290157309481,-4.55458938262534,
125.485154247296));
#218998=CARTESIAN_POINT('Ctrl Pts',(32.6505681071352,-6.93706578039975,
131.761104685873));
#218999=CARTESIAN_POINT('Ctrl Pts',(32.3721204833222,-2.94471762049033,
137.157854065221));
#219000=CARTESIAN_POINT('Ctrl Pts',(32.0936728595094,3.75368217519627,136.716053351584));
#219001=CARTESIAN_POINT('Ctrl Pts',(31.8152252356965,7.00263142944649,130.84169581763));
#219002=CARTESIAN_POINT('Ctrl Pts',(31.5367776118836,3.8165044975991,124.933029058741));
#219003=CARTESIAN_POINT('Ctrl Pts',(31.2583299880707,-2.87680362093211,
124.41982917192));
#219004=CARTESIAN_POINT('Ctrl Pts',(30.9798823642578,-6.92646975149653,
129.773701781947));
#219005=CARTESIAN_POINT('Ctrl Pts',(30.7014347404449,-4.6110485572945,136.074699511423));
#219006=CARTESIAN_POINT('Ctrl Pts',(30.422987116632,1.94170099881587,137.532513267813));
#219007=CARTESIAN_POINT('Ctrl Pts',(30.1445394928192,6.71012219438185,132.807483427156));
#219008=CARTESIAN_POINT('Ctrl Pts',(29.8660918690062,5.31226890100394,126.241681582474));
#219009=CARTESIAN_POINT('Ctrl Pts',(29.5876442451933,-0.967299993633269,
123.868758871779));
#219010=CARTESIAN_POINT('Ctrl Pts',(29.3091966213805,-6.35796744935336,
127.869315342481));
#219011=CARTESIAN_POINT('Ctrl Pts',(29.0307489975676,-5.90597342309497,
134.567035036052));
#219012=CARTESIAN_POINT('Ctrl Pts',(28.7523013737546,-0.026678343854083,
137.807040755898));
#219013=CARTESIAN_POINT('Ctrl Pts',(28.4738537499418,5.87713283007914,134.611925528561));
#219014=CARTESIAN_POINT('Ctrl Pts',(28.1954061261289,6.38014604707014,127.917844157905));
#219015=CARTESIAN_POINT('Ctrl Pts',(27.916958502316,1.02011673426565,123.876330399509));
#219016=CARTESIAN_POINT('Ctrl Pts',(27.6385108785031,-5.27735002185588,
126.201337958415));
#219017=CARTESIAN_POINT('Ctrl Pts',(27.3600632546902,-6.72518992077305,
132.756298470923));
#219018=CARTESIAN_POINT('Ctrl Pts',(27.0816156308773,-1.99290882629253,
137.51752345366));
#219019=CARTESIAN_POINT('Ctrl Pts',(26.8031680070644,4.57075812054227,136.109679746264));
#219020=CARTESIAN_POINT('Ctrl Pts',(26.5247203832516,6.93412164854658,129.826506938842));
#219021=CARTESIAN_POINT('Ctrl Pts',(26.2462727594386,2.92536613221128,124.441933891359));
#219022=CARTESIAN_POINT('Ctrl Pts',(25.9678251356258,-3.7716579475455,124.904120183435));
#219023=CARTESIAN_POINT('Ctrl Pts',(25.6893775118128,-7.00271262924226,
130.788339191706));
#219024=CARTESIAN_POINT('Ctrl Pts',(25.410929888,-3.79861650619593,136.687281107654));
#219025=CARTESIAN_POINT('Ctrl Pts',(25.1324822641871,2.89622261331168,137.180106489852));
#219026=CARTESIAN_POINT('Ctrl Pts',(24.8540346403742,6.92957463952618,131.813932887921));
#219027=CARTESIAN_POINT('Ctrl Pts',(24.5755870165613,4.59498610055721,125.520011689881));
#219028=CARTESIAN_POINT('Ctrl Pts',(24.2971393927484,-1.96217018727317,
124.082149001586));
#219029=CARTESIAN_POINT('Ctrl Pts',(24.0186917689355,-6.71618793034234,
128.821670390082));
#219030=CARTESIAN_POINT('Ctrl Pts',(23.7402441451226,-5.29835706944761,
135.383187237832));
#219031=CARTESIAN_POINT('Ctrl Pts',(23.4617965213097,0.988405099136929,
137.736986109674));
#219032=CARTESIAN_POINT('Ctrl Pts',(23.1833488974968,6.36687126788796,133.720040831851));
#219033=CARTESIAN_POINT('Ctrl Pts',(22.9049012736839,5.89449378040337,127.023727875996));
#219034=CARTESIAN_POINT('Ctrl Pts',(22.6264536498711,0.00536447075796404,
123.801631715467));
#219035=CARTESIAN_POINT('Ctrl Pts',(22.3480060260581,-5.88869452544514,
127.01470131364));
#219036=CARTESIAN_POINT('Ctrl Pts',(22.0695584022453,-6.3713309314846,133.710282676972));
#219037=CARTESIAN_POINT('Ctrl Pts',(21.7911107784324,-0.999025468309402,
137.735463629893));
#219038=CARTESIAN_POINT('Ctrl Pts',(21.5126631546195,5.29133559513472,135.391299517692));
#219039=CARTESIAN_POINT('Ctrl Pts',(21.2342155308066,6.71921774276442,128.831962640697));
#219040=CARTESIAN_POINT('Ctrl Pts',(20.9557679069937,1.97246703682929,124.085163147446));
#219041=CARTESIAN_POINT('Ctrl Pts',(20.6773202831809,-4.58688451558038,
125.51297787819));
#219042=CARTESIAN_POINT('Ctrl Pts',(20.3988726593679,-6.93111327993769,
131.803314848003));
#219043=CARTESIAN_POINT('Ctrl Pts',(20.120425035555,-2.90598754374001,137.175661681671));
#219044=CARTESIAN_POINT('Ctrl Pts',(19.8419774117421,3.78959877977074,136.693094092787));
#219045=CARTESIAN_POINT('Ctrl Pts',(19.5635297879293,7.00272895686486,130.799068120799));
#219046=CARTESIAN_POINT('Ctrl Pts',(19.2850821641163,3.78069332492835,124.909905694786));
#219047=CARTESIAN_POINT('Ctrl Pts',(19.0066345403035,-2.91561477548059,
124.437459382677));
#219048=CARTESIAN_POINT('Ctrl Pts',(18.7281869164906,-6.932615332923,129.815884265012));
#219049=CARTESIAN_POINT('Ctrl Pts',(18.4497392926777,-4.57888107649638,
136.102670625591));
#219050=CARTESIAN_POINT('Ctrl Pts',(18.1712916688647,1.98262119845391,137.520568925627));
#219051=CARTESIAN_POINT('Ctrl Pts',(17.892844045052,6.72219144845534,132.766599895572));
#219052=CARTESIAN_POINT('Ctrl Pts',(17.614396421239,5.28439615463518,126.209428829746));
#219053=CARTESIAN_POINT('Ctrl Pts',(17.3359487974261,-1.00950104819076,
123.87477560203));
#219054=CARTESIAN_POINT('Ctrl Pts',(17.0575011736132,-6.37571610459714,
127.908072474542));
#219055=CARTESIAN_POINT('Ctrl Pts',(16.7790535498004,-5.88295953192644,
134.602916658952));
#219056=CARTESIAN_POINT('Ctrl Pts',(16.5006059259874,0.0159494520341194,
137.807073411106));
#219057=CARTESIAN_POINT('Ctrl Pts',(16.2221583021745,5.90020166874948,134.576079207535));
#219058=CARTESIAN_POINT('Ctrl Pts',(15.9437106783617,6.3624567927597,127.879059878479));
#219059=CARTESIAN_POINT('Ctrl Pts',(15.6652630545488,0.977924947517885,
123.870249019757));
#219060=CARTESIAN_POINT('Ctrl Pts',(15.3868154307359,-5.3052721502032,126.233547969238));
#219061=CARTESIAN_POINT('Ctrl Pts',(15.108367806923,-6.71318331884074,132.797200445919));
#219062=CARTESIAN_POINT('Ctrl Pts',(14.8299201831101,-1.95200697470083,
137.529530475982));
#219063=CARTESIAN_POINT('Ctrl Pts',(14.5514725592972,4.6029684183469,136.081757948972));
#219064=CARTESIAN_POINT('Ctrl Pts',(14.2730249354843,6.92804070244224,129.784315089592));
#219065=CARTESIAN_POINT('Ctrl Pts',(13.9945773116714,2.88658203459712,124.424244238425));
#219066=CARTESIAN_POINT('Ctrl Pts',(13.7161296878585,-3.80750450567058,
124.927188653676));
#219067=CARTESIAN_POINT('Ctrl Pts',(13.4376820640456,-7.00268041216303,
130.830966987928));
#219068=CARTESIAN_POINT('Ctrl Pts',(13.1592344402328,-3.7627351198343,136.710295367612));
#219069=CARTESIAN_POINT('Ctrl Pts',(12.8807868164199,2.93497992779253,137.162358232954));
#219070=CARTESIAN_POINT('Ctrl Pts',(12.602339192607,6.93559180351842,131.771731895206));
#219071=CARTESIAN_POINT('Ctrl Pts',(12.323891568794,4.56273363430679,125.49213861202));
#219072=CARTESIAN_POINT('Ctrl Pts',(12.0454439449812,-2.00305384290271,
124.094217835458));
#219073=CARTESIAN_POINT('Ctrl Pts',(11.7669963211683,-6.72813269310505,
128.862590466954));
#219074=CARTESIAN_POINT('Ctrl Pts',(11.4885486973554,-5.27038628589867,
135.415355006116));
#219075=CARTESIAN_POINT('Ctrl Pts',(11.2101010735425,1.03058764536478,137.730840961799));
#219076=CARTESIAN_POINT('Ctrl Pts',(10.9316534497296,6.38450187754329,133.681229858508));
#219077=CARTESIAN_POINT('Ctrl Pts',(10.6532058259167,5.87137078451608,126.987916465666));
#219078=CARTESIAN_POINT('Ctrl Pts',(10.3747582021038,-0.0372632270726686,
123.801728804758));
#219079=CARTESIAN_POINT('Ctrl Pts',(10.0963105782909,-5.91165415339157,
127.050617682238));
#219080=CARTESIAN_POINT('Ctrl Pts',(9.81786295447806,-6.35352371310424,
133.749012936746));
#219081=CARTESIAN_POINT('Ctrl Pts',(9.53941533066515,-0.956815367363035,
137.741416564191));
#219082=CARTESIAN_POINT('Ctrl Pts',(9.26096770685226,5.31915955795546,135.35900467071));
#219083=CARTESIAN_POINT('Ctrl Pts',(8.98252008303941,6.70708670490366,128.791097399121));
#219084=CARTESIAN_POINT('Ctrl Pts',(8.70407245922646,1.93152882944647,124.073280671906));
#219085=CARTESIAN_POINT('Ctrl Pts',(8.42562483541358,-4.61900967984285,
125.540997583217));
#219086=CARTESIAN_POINT('Ctrl Pts',(8.14717721160073,-6.92490394452403,
131.845487993513));
#219087=CARTESIAN_POINT('Ctrl Pts',(7.86872958778781,-2.86714978455288,
137.193233207215));
#219088=CARTESIAN_POINT('Ctrl Pts',(7.59028196397491,3.82537495936868,136.669916624805));
#219089=CARTESIAN_POINT('Ctrl Pts',(7.31183434016203,7.00256699558648,130.756440620084));
#219090=CARTESIAN_POINT('Ctrl Pts',(7.03338671634916,3.7447420572761,124.887000752025));
#219091=CARTESIAN_POINT('Ctrl Pts',(6.75493909253623,-2.95431789085107,
124.455325521299));
#219092=CARTESIAN_POINT('Ctrl Pts',(6.47649146872337,-6.9385040237388,129.858103376433));
#219093=CARTESIAN_POINT('Ctrl Pts',(6.19804384491048,-4.54654392357636,
136.130445408932));
#219094=CARTESIAN_POINT('Ctrl Pts',(5.91959622109758,2.02346793133434,137.508375711873));
#219095=CARTESIAN_POINT('Ctrl Pts',(5.64114859728465,6.73401160925262,132.725643652489));
#219096=CARTESIAN_POINT('Ctrl Pts',(5.36270097347181,5.25632759302358,126.177346343905));
#219097=CARTESIAN_POINT('Ctrl Pts',(5.08425334965889,-1.05166469531565,
123.881049110601));
#219098=CARTESIAN_POINT('Ctrl Pts',(4.80580572584599,-6.39322850533622,
127.946936929627));
#219099=CARTESIAN_POINT('Ctrl Pts',(4.5273581020331,-5.85972764552883,134.638657524961));
#219100=CARTESIAN_POINT('Ctrl Pts',(4.24891047822024,0.0585766569097649,
137.806846578216));
#219101=CARTESIAN_POINT('Ctrl Pts',(3.97046285440732,5.92305187327717,134.54009312409));
#219102=CARTESIAN_POINT('Ctrl Pts',(3.69201523059441,6.34453177527304,127.840383997147));
#219103=CARTESIAN_POINT('Ctrl Pts',(3.41356760678156,0.935696923401329,
123.864424586062));
#219104=CARTESIAN_POINT('Ctrl Pts',(3.13511998296867,-5.33299768974021,
126.265927353204));
#219105=CARTESIAN_POINT('Ctrl Pts',(2.85667235915575,-6.70092795743158,
132.838028575505));
#219106=CARTESIAN_POINT('Ctrl Pts',(2.57822473534285,-1.91103279077285,
137.541288294661));
#219107=CARTESIAN_POINT('Ctrl Pts',(2.29977711153,4.63500815146407,136.053640595781));
#219108=CARTESIAN_POINT('Ctrl Pts',(2.02132948771708,6.92170303524179,129.742161038504));
#219109=CARTESIAN_POINT('Ctrl Pts',(1.74288186390418,2.84769097362441,124.40679100305));
#219110=CARTESIAN_POINT('Ctrl Pts',(1.46443424009131,-3.84320997531586,
124.950474904685));
#219111=CARTESIAN_POINT('Ctrl Pts',(1.18598661627842,-7.00238870818588,
130.873593798241));
#219112=CARTESIAN_POINT('Ctrl Pts',(0.907538992465495,-3.72671430393905,
136.733090780986));
#219113=CARTESIAN_POINT('Ctrl Pts',(0.629091368652655,2.97362848551254,
137.144374378117));
#219114=CARTESIAN_POINT('Ctrl Pts',(0.350643744839755,6.94135196660579,
131.729495056193));
#219115=CARTESIAN_POINT('Ctrl Pts',(0.0721961210268491,4.53031209428387,
125.4644623805));
#219116=CARTESIAN_POINT('Ctrl Pts',(-0.206251502786054,-2.04386327463549,
124.106535316138));
#219117=CARTESIAN_POINT('Ctrl Pts',(-0.484699126598912,-6.73982814243653,
128.903582496833));
#219118=CARTESIAN_POINT('Ctrl Pts',(-0.763146750411823,-5.24222020624778,
135.447351912307));
#219119=CARTESIAN_POINT('Ctrl Pts',(-1.04159437422473,1.07273200278813,
137.724439150648));
#219120=CARTESIAN_POINT('Ctrl Pts',(-1.32004199803759,6.40189590713365,
133.642312281717));
#219121=CARTESIAN_POINT('Ctrl Pts',(-1.59848962185049,5.84803022282516,
126.952246475077));
#219122=CARTESIAN_POINT('Ctrl Pts',(-1.87693724566341,-0.0798895441007186,
123.802085379146));
#219123=CARTESIAN_POINT('Ctrl Pts',(-2.1553848694763,-5.93439472281934,
127.08667314716));
#219124=CARTESIAN_POINT('Ctrl Pts',(-2.43383249328916,-6.33548106256618,
133.787634081347));
#219125=CARTESIAN_POINT('Ctrl Pts',(-2.71228011710207,-0.914569811271147,
137.747112443329));
#219126=CARTESIAN_POINT('Ctrl Pts',(-2.99072774091498,5.34678641736288,
135.326541049718));
#219127=CARTESIAN_POINT('Ctrl Pts',(-3.26917536472784,6.6947071334783,128.750306759754));
#219128=CARTESIAN_POINT('Ctrl Pts',(-3.54762298854074,1.89051904855254,
124.061647619009));
#219129=CARTESIAN_POINT('Ctrl Pts',(-3.82607061235365,-4.65096368500298,
125.569212324096));
#219130=CARTESIAN_POINT('Ctrl Pts',(-4.10451823616654,-6.91843800424817,
131.887622559669));
#219131=CARTESIAN_POINT('Ctrl Pts',(-4.38296585997939,-2.82820578207579,
137.210567990736));
#219132=CARTESIAN_POINT('Ctrl Pts',(-4.66141348379231,3.86100938829084,
136.646521806489));
#219133=CARTESIAN_POINT('Ctrl Pts',(-4.93986110760522,7.00214555161287,
130.713814895061));
#219134=CARTESIAN_POINT('Ctrl Pts',(-5.21830873141809,3.70865202682979,
124.864315079211));
#219135=CARTESIAN_POINT('Ctrl Pts',(-5.49675635523098,-2.99291153288594,
124.473426925751));
#219136=CARTESIAN_POINT('Ctrl Pts',(-5.77520397904388,-6.9441356057364,
129.900357551763));
#219137=CARTESIAN_POINT('Ctrl Pts',(-6.05365160285679,-4.51403829679898,
136.158022832244));
#219138=CARTESIAN_POINT('Ctrl Pts',(-6.33209922666964,2.06423968386644,
137.495934078373));
#219139=CARTESIAN_POINT('Ctrl Pts',(-6.61054685048256,6.74558223877327,
132.684616215558));
#219140=CARTESIAN_POINT('Ctrl Pts',(-6.88899447429547,5.22806425626005,
126.145435313781));
#219141=CARTESIAN_POINT('Ctrl Pts',(-7.16744209810832,-1.09378937261818,
123.887579165027));
#219142=CARTESIAN_POINT('Ctrl Pts',(-7.44588972192122,-6.41050400264194,
127.985907267597));
#219143=CARTESIAN_POINT('Ctrl Pts',(-7.72433734573414,-5.8362786247684,
134.674256309687));
#219144=CARTESIAN_POINT('Ctrl Pts',(-8.002784969547,0.101201691205851,137.806360265633));
#219145=CARTESIAN_POINT('Ctrl Pts',(-8.28123259335988,5.94568259693924,
134.503968611703));
#219146=CARTESIAN_POINT('Ctrl Pts',(-8.55968021717279,6.32637165882838,
127.80181794706));
#219147=CARTESIAN_POINT('Ctrl Pts',(-8.8381278409857,0.893434226691435,
123.858857314246));
#219148=CARTESIAN_POINT('Ctrl Pts',(-9.11657546479855,-5.3605256130866,
126.298474910485));
#219149=CARTESIAN_POINT('Ctrl Pts',(-9.39502308861147,-6.68842429067269,
132.878781346775));
#219150=CARTESIAN_POINT('Ctrl Pts',(-9.67347071242438,-1.86998779282204,
137.552796474009));
#219151=CARTESIAN_POINT('Ctrl Pts',(-9.95191833623725,4.66687613264966,
136.025328728591));
#219152=CARTESIAN_POINT('Ctrl Pts',(-10.2303659600501,6.91510888178999,
129.700046347612));
#219153=CARTESIAN_POINT('Ctrl Pts',(-10.508813583863,2.80869439041515,124.389574831969));
#219154=CARTESIAN_POINT('Ctrl Pts',(-10.787261207676,-3.87877303340228,
124.973978073582));
#219155=CARTESIAN_POINT('Ctrl Pts',(-11.0657088314888,-7.00183752812002,
130.916218043094));
#219156=CARTESIAN_POINT('Ctrl Pts',(-11.3441564553017,-3.69055539327479,
136.755666503084));
#219157=CARTESIAN_POINT('Ctrl Pts',(-11.6226040791146,3.01216685433575,
137.126155591738));
#219158=CARTESIAN_POINT('Ctrl Pts',(-11.9010517029275,6.94685491534338,
131.687223935982));
#219159=CARTESIAN_POINT('Ctrl Pts',(-12.1794993267404,4.49772268187999,
125.436984020872));
#219160=CARTESIAN_POINT('Ctrl Pts',(-12.4579469505533,-2.08459697026297,
124.119100987199));
#219161=CARTESIAN_POINT('Ctrl Pts',(-12.7363945743662,-6.75127384495765,
128.944644960744));
#219162=CARTESIAN_POINT('Ctrl Pts',(-13.0148421981791,-5.21385987419926,
135.479176770748));
#219163=CARTESIAN_POINT('Ctrl Pts',(-13.2932898219919,1.11483660973293,
137.717780913442));
#219164=CARTESIAN_POINT('Ctrl Pts',(-13.5717374458049,6.41905271211686,
133.603289543584));
#219165=CARTESIAN_POINT('Ctrl Pts',(-13.8501850696177,5.82447296022373,
126.916719225995));
#219166=CARTESIAN_POINT('Ctrl Pts',(-14.1286326934306,-0.122512900792341,
123.802701425419));
#219167=CARTESIAN_POINT('Ctrl Pts',(-14.4070803172435,-5.95691539106803,
127.122866372359));
#219168=CARTESIAN_POINT('Ctrl Pts',(-14.6855279410564,-6.31720364844761,
133.826144679651));
#219169=CARTESIAN_POINT('Ctrl Pts',(-14.9639755648693,-0.872290365458834,
137.752551056246));
#219170=CARTESIAN_POINT('Ctrl Pts',(-15.2424231886822,5.37421514963333,
135.293909857666));
#219171=CARTESIAN_POINT('Ctrl Pts',(-15.5208708124951,6.68207948721813,
128.709592234107));
#219172=CARTESIAN_POINT('Ctrl Pts',(-15.799318436308,1.84943921378025,124.050264419823));
#219173=CARTESIAN_POINT('Ctrl Pts',(-16.0777660601209,-4.68274534699314,
125.59762105532));
#219174=CARTESIAN_POINT('Ctrl Pts',(-16.3562136839338,-6.91171569870797,
131.929716985153));
#219175=CARTESIAN_POINT('Ctrl Pts',(-16.6346613077467,-2.78915697939336,
137.227665389888));
#219176=CARTESIAN_POINT('Ctrl Pts',(-16.9131089315595,3.89650074609022,
136.622910504741));
#219177=CARTESIAN_POINT('Ctrl Pts',(-17.1915565553724,7.00146464056082,
130.671192525245));
#219178=CARTESIAN_POINT('Ctrl Pts',(-17.4700041791854,3.67242457091876,
124.841849516969));
#219179=CARTESIAN_POINT('Ctrl Pts',(-17.7484518029982,-3.0313942714833,
124.491762925279));
#219180=CARTESIAN_POINT('Ctrl Pts',(-18.0268994268111,-6.94950987023543,
129.942645225261));
#219181=CARTESIAN_POINT('Ctrl Pts',(-18.305347050624,-4.48136540067248,
136.185401873632));
#219182=CARTESIAN_POINT('Ctrl Pts',(-18.5837946744369,2.10493494523792,
137.483244486159));
#219183=CARTESIAN_POINT('Ctrl Pts',(-18.8622422982498,6.75690290826339,
132.643519105064));
#219184=CARTESIAN_POINT('Ctrl Pts',(-19.1406899220627,5.19960719165284,
126.113696921846));
#219185=CARTESIAN_POINT('Ctrl Pts',(-19.4191375458756,-1.1358735191536,
123.894365523333));
#219186=CARTESIAN_POINT('Ctrl Pts',(-19.6975851696885,-6.42754195636435,
128.024982044393));
#219187=CARTESIAN_POINT('Ctrl Pts',(-19.9760327935014,-5.81261333855723,
134.709711694007));
#219188=CARTESIAN_POINT('Ctrl Pts',(-20.2544804173143,0.143822975436045,
137.805614491377));
#219189=CARTESIAN_POINT('Ctrl Pts',(-20.5329280411272,5.96809300114641,
134.467707008981));
#219190=CARTESIAN_POINT('Ctrl Pts',(-20.81137566494,6.30797711635522,127.763363157294));
#219191=CARTESIAN_POINT('Ctrl Pts',(-21.089823288753,0.851138423447451,
123.853547410611));
#219192=CARTESIAN_POINT('Ctrl Pts',(-21.3682709125658,-5.38785490018508,
126.331189435016));
#219193=CARTESIAN_POINT('Ctrl Pts',(-21.6467185363787,-6.67567278189203,
132.919457249623));
#219194=CARTESIAN_POINT('Ctrl Pts',(-21.9251661601916,-1.82887350178604,
137.564054587584));
#219195=CARTESIAN_POINT('Ctrl Pts',(-22.2036137840045,4.69857118102365,
135.996823396506));
#219196=CARTESIAN_POINT('Ctrl Pts',(-22.4820614078173,6.90825848643574,
129.657972577492));
#219197=CARTESIAN_POINT('Ctrl Pts',(-22.7605090316303,2.76959373000234,
124.372596363135));
#219198=CARTESIAN_POINT('Ctrl Pts',(-23.0389566554432,-3.91419236212754,
124.997697289448));
#219199=CARTESIAN_POINT('Ctrl Pts',(-23.3174042792561,-7.0010268923895,
130.958838143028));
#219200=CARTESIAN_POINT('Ctrl Pts',(-23.5958519030689,-3.65425972772349,
136.778021697354));
#219201=CARTESIAN_POINT('Ctrl Pts',(-23.8742995268818,3.05059360620828,
137.107702548922));
#219202=CARTESIAN_POINT('Ctrl Pts',(-24.1527471506948,6.95210044581739,
131.644920100946));
#219203=CARTESIAN_POINT('Ctrl Pts',(-24.4311947745076,4.4649666047081,125.409704551357));
#219204=CARTESIAN_POINT('Ctrl Pts',(-24.7096423983205,-2.12525342038311,
124.131914383013));
#219205=CARTESIAN_POINT('Ctrl Pts',(-24.9880900221334,-6.76246937654364,
128.985776337104));
#219206=CARTESIAN_POINT('Ctrl Pts',(-25.2665376459463,-5.18530634065569,
135.510828402156));
#219207=CARTESIAN_POINT('Ctrl Pts',(-25.5449852697592,1.15689990599717,
137.710866496904));
#219208=CARTESIAN_POINT('Ctrl Pts',(-25.8234328935721,6.43597165674122,
133.564163090109));
#219209=CARTESIAN_POINT('Ctrl Pts',(-26.101880517385,5.8006998696348,126.881336034893));
#219210=CARTESIAN_POINT('Ctrl Pts',(-26.3803281411979,-0.165131717723356,
123.803576920747));
#219211=CARTESIAN_POINT('Ctrl Pts',(-26.6587757650107,-5.9792153236265,
127.15919601668));
#219212=CARTESIAN_POINT('Ctrl Pts',(-26.9372233888237,-6.29869214802456,
133.864543304637));
#219213=CARTESIAN_POINT('Ctrl Pts',(-27.2156710126366,-0.829978596605981,
137.75773220141));
#219214=CARTESIAN_POINT('Ctrl Pts',(-27.4941186364494,5.40144473838504,
135.261112303716));
#219215=CARTESIAN_POINT('Ctrl Pts',(-27.7725662602623,6.66920423404522,
128.668955330874));
#219216=CARTESIAN_POINT('Ctrl Pts',(-28.0510138840753,1.80829084735756,
124.039131496154));
#219217=CARTESIAN_POINT('Ctrl Pts',(-28.3294615078881,-4.71435348813263,
125.626222724194));
#219218=CARTESIAN_POINT('Ctrl Pts',(-28.607909131701,-6.9047372770006,131.971769710144));
#219219=CARTESIAN_POINT('Ctrl Pts',(-28.8863567555139,-2.75000482347336,
137.244524771118));
#219220=CARTESIAN_POINT('Ctrl Pts',(-29.1648043793268,3.93184771762154,
136.599083594488));
#219221=CARTESIAN_POINT('Ctrl Pts',(-29.4432520031397,7.00052428766157,
130.628575090021));
#219222=CARTESIAN_POINT('Ctrl Pts',(-29.7216996269525,3.63606103196502,
124.819604897767));
#219223=CARTESIAN_POINT('Ctrl Pts',(-30.0001472507655,-3.06976468065099,
124.510332840438));
#219224=CARTESIAN_POINT('Ctrl Pts',(-30.2785948745783,-6.95462661809053,
129.984964829937));
#219225=CARTESIAN_POINT('Ctrl Pts',(-30.5570424983912,-4.44852644590303,
136.212581518559));
#219226=CARTESIAN_POINT('Ctrl Pts',(-30.8354901222041,2.14555220747066,
137.470307405446));
#219227=CARTESIAN_POINT('Ctrl Pts',(-31.113937746017,6.7679731982313,132.602353843876));
#219228=CARTESIAN_POINT('Ctrl Pts',(-31.3923853698299,5.17095745368924,
126.082132344179));
#219229=CARTESIAN_POINT('Ctrl Pts',(-31.6708329936428,-1.17791557547805,
123.901407934047));
#219230=CARTESIAN_POINT('Ctrl Pts',(-31.9492806174558,-6.44434173515584,
128.064159812084));
#219231=CARTESIAN_POINT('Ctrl Pts',(-32.2277282412685,-5.78873266382121,
134.745022364106));
#219232=CARTESIAN_POINT('Ctrl Pts',(-32.5061758650815,0.186438930252996,
137.804609283086));
#219233=CARTESIAN_POINT('Ctrl Pts',(-32.7846234888944,5.99028225547263,
134.431309659613));
#219234=CARTESIAN_POINT('Ctrl Pts',(-33.0630711127073,6.28934882947028,
127.725021052809));
#219235=CARTESIAN_POINT('Ctrl Pts',(-33.3415187365202,0.808811080956172,
123.848495071916));
#219236=CARTESIAN_POINT('Ctrl Pts',(-33.619966360333,-5.41498453833882,
126.364069714552));
#219237=CARTESIAN_POINT('Ctrl Pts',(-33.898413984146,-6.66267390360147,
132.960054776787));
#219238=CARTESIAN_POINT('Ctrl Pts',(-34.1768616079588,-1.78769144116968,
137.575062218212));
#219239=CARTESIAN_POINT('Ctrl Pts',(-34.4553092317717,4.73009212211488,
135.968125655805));
#219240=CARTESIAN_POINT('Ctrl Pts',(-34.7337568555846,6.90115210302259,
129.615941287202));
#219241=CARTESIAN_POINT('Ctrl Pts',(-35.0122044793975,2.73039044127535,
124.355856225691));
#219242=CARTESIAN_POINT('Ctrl Pts',(-35.2906521032104,-3.94946664901538,
125.02163167336));
#219243=CARTESIAN_POINT('Ctrl Pts',(-35.5690997270233,-6.99995683103299,
131.00145251874));
#219244=CARTESIAN_POINT('Ctrl Pts',(-35.8475473508362,-3.61782865223385,
136.800155535415));
#219245=CARTESIAN_POINT('Ctrl Pts',(-36.125994974649,3.08890731721304,137.089015933453));
#219246=CARTESIAN_POINT('Ctrl Pts',(-36.404442598462,6.95708836365274,131.60258511867));
#219247=CARTESIAN_POINT('Ctrl Pts',(-36.6828902222748,4.43204507655667,
125.382624982808));
#219248=CARTESIAN_POINT('Ctrl Pts',(-36.9613378460878,-2.16583111845593,
124.144975028777));
#219249=CARTESIAN_POINT('Ctrl Pts',(-37.2397854699006,-6.7734143223399,
129.026975101771));
#219250=CARTESIAN_POINT('Ctrl Pts',(-37.5182330937135,-5.15656066367905,
135.54230563367));
#219251=CARTESIAN_POINT('Ctrl Pts',(-37.7966807175264,1.19892033290996,
137.703696157251));
#219252=CARTESIAN_POINT('Ctrl Pts',(-38.0751283413393,6.45265211406898,
133.524934371139));
#219253=CARTESIAN_POINT('Ctrl Pts',(-38.3535759651522,5.77671183197903,
126.846098212911));
#219254=CARTESIAN_POINT('Ctrl Pts',(-38.6320235889651,-0.207744415637528,
123.80471183269));
#219255=CARTESIAN_POINT('Ctrl Pts',(-38.910471212778,-6.00129369416227,
127.195660733917));
#219256=CARTESIAN_POINT('Ctrl Pts',(-39.1889188365908,-6.27994724724761,
133.902828533427));
#219257=CARTESIAN_POINT('Ctrl Pts',(-39.4673664604039,-0.787636072591,137.762655686833));
#219258=CARTESIAN_POINT('Ctrl Pts',(-39.7458140842166,5.42847417461558,
135.228149603194));
#219259=CARTESIAN_POINT('Ctrl Pts',(-40.0242617080296,6.65608185105682,
128.628397555869));
#219260=CARTESIAN_POINT('Ctrl Pts',(-40.3027093318424,1.76707547405252,
124.028249260538));
#219261=CARTESIAN_POINT('Ctrl Pts',(-40.5811569556554,-4.7457869371699,
125.655016270872));
#219262=CARTESIAN_POINT('Ctrl Pts',(-40.8596045794682,-6.89750299771422,
132.013779176361));
#219263=CARTESIAN_POINT('Ctrl Pts',(-41.1380522032811,-2.7107507651133,
137.261145509698));
#219264=CARTESIAN_POINT('Ctrl Pts',(-41.416499827094,3.96704899308973,136.575041958643));
#219265=CARTESIAN_POINT('Ctrl Pts',(-41.694947450907,6.99932452776054,130.585964168594));
#219266=CARTESIAN_POINT('Ctrl Pts',(-41.9733950747197,3.59956275743227,
124.79758204589));
#219267=CARTESIAN_POINT('Ctrl Pts',(-42.2518426985328,-3.10802133855968,
124.529135983109));
#219268=CARTESIAN_POINT('Ctrl Pts',(-42.5302903223456,-6.95948565969872,
130.027314797628));
#219269=CARTESIAN_POINT('Ctrl Pts',(-42.8087379461585,-4.41552264935019,
136.23956075987));
#219270=CARTESIAN_POINT('Ctrl Pts',(-43.0871855699714,2.18608996547759,
137.457123315624));
#219271=CARTESIAN_POINT('Ctrl Pts',(-43.3656331937842,6.77879269846351,
132.561121957388));
#219272=CARTESIAN_POINT('Ctrl Pts',(-43.6440808175972,5.14211610399531,
126.050742750417));
#219273=CARTESIAN_POINT('Ctrl Pts',(-43.92252844141,-1.21991398370768,123.908706136214));
#219274=CARTESIAN_POINT('Ctrl Pts',(-44.200976065223,-6.46090271649442,
128.103439118922));
#219275=CARTESIAN_POINT('Ctrl Pts',(-44.4794236890358,-5.76463748546755,
134.780187011534));
#219276=CARTESIAN_POINT('Ctrl Pts',(-44.7578713128487,0.229047976506494,
137.803344678006));
#219277=CARTESIAN_POINT('Ctrl Pts',(-45.0363189366615,6.01224953768695,
134.394777912313));
#219278=CARTESIAN_POINT('Ctrl Pts',(-45.3147665604746,6.27048748845154,
127.686793054383));
#219279=CARTESIAN_POINT('Ctrl Pts',(-45.5932141842873,0.766453767672844,
123.843700485376));
#219280=CARTESIAN_POINT('Ctrl Pts',(-45.8716618081003,-5.44191352224889,
126.397114530699));
#219281=CARTESIAN_POINT('Ctrl Pts',(-46.1501094319132,-6.6494281374793,
133.000572423912));
#219282=CARTESIAN_POINT('Ctrl Pts',(-46.4285570557261,-1.74644313698983,
137.585818958004));
#219283=CARTESIAN_POINT('Ctrl Pts',(-46.7070046795389,4.76143778790304,
135.93923656989));
#219284=CARTESIAN_POINT('Ctrl Pts',(-46.9854523033519,6.89378999488032,
129.573954034227));
#219285=CARTESIAN_POINT('Ctrl Pts',(-47.2638999271647,2.69108597692664,
124.339355039948));
#219286=CARTESIAN_POINT('Ctrl Pts',(-47.5423475509777,-3.98459458696386,
125.045780338419));
#219287=CARTESIAN_POINT('Ctrl Pts',(-47.8207951747905,-6.998627383702,131.044059591139));
#219288=CARTESIAN_POINT('Ctrl Pts',(-48.0992427986034,-3.58126351677304,
136.822067197091));
#219289=CARTESIAN_POINT('Ctrl Pts',(-48.3776904224163,3.1271065676212,137.070096437769));
#219290=CARTESIAN_POINT('Ctrl Pts',(-48.6561380462292,6.9618184840203,131.560220557891));
#219291=CARTESIAN_POINT('Ctrl Pts',(-48.9345856700421,4.39895931734504,
125.355746318666));
#219292=CARTESIAN_POINT('Ctrl Pts',(-49.213033293855,-2.20632856086043,
124.158282440523));
#219293=CARTESIAN_POINT('Ctrl Pts',(-49.4914809176678,-6.78410827677761,
129.068239728113));
#219294=CARTESIAN_POINT('Ctrl Pts',(-49.7699285414808,-5.12762390845042,
135.573607298891));
#219295=CARTESIAN_POINT('Ctrl Pts',(-50.0483761652936,1.2408963333889,137.696270160183));
#219296=CARTESIAN_POINT('Ctrl Pts',(-50.3268237891066,6.46909346599971,
133.485604840309));
#219297=CARTESIAN_POINT('Ctrl Pts',(-50.6052714129194,5.7525097361419,126.811007065796));
#219298=CARTESIAN_POINT('Ctrl Pts',(-50.8837190367324,-0.250349415506305,
123.806106119193));
#219299=CARTESIAN_POINT('Ctrl Pts',(-51.1621666605453,-6.02314968455324,
127.232259172855));
#219300=CARTESIAN_POINT('Ctrl Pts',(-51.4406142843581,-6.26096964071598,
133.94099894735));
#219301=CARTESIAN_POINT('Ctrl Pts',(-51.719061908171,-0.745264362431691,
137.767321330073));
#219302=CARTESIAN_POINT('Ctrl Pts',(-51.997509531984,5.45530245673899,135.195022977544));
#219303=CARTESIAN_POINT('Ctrl Pts',(-52.2759571557968,6.64271282450778,
128.587920411975));
#219304=CARTESIAN_POINT('Ctrl Pts',(-52.5544047796097,1.72579462111621,
124.01761811622));
#219305=CARTESIAN_POINT('Ctrl Pts',(-52.8328524034226,-4.77704452932697,
125.684000628399));
#219306=CARTESIAN_POINT('Ctrl Pts',(-53.1113000272355,-6.89001312891767,
132.05574382713));
#219307=CARTESIAN_POINT('Ctrl Pts',(-53.3897476510484,-2.67139625888694,
137.277526989739));
#219308=CARTESIAN_POINT('Ctrl Pts',(-53.6681952748612,4.00210326809833,
136.550786488079));
#219309=CARTESIAN_POINT('Ctrl Pts',(-53.9466428986742,6.99786540531528,
130.543361339928));
#219310=CARTESIAN_POINT('Ctrl Pts',(-54.225090522487,3.56293109977782,124.775781777402));
#219311=CARTESIAN_POINT('Ctrl Pts',(-54.5035381462999,-3.14616282759469,
124.548171656537));
#219312=CARTESIAN_POINT('Ctrl Pts',(-54.7819857701128,-6.9640868150063,
130.069693559035));
#219313=CARTESIAN_POINT('Ctrl Pts',(-55.0604333939257,-4.382355233982,136.266338597842));
#219314=CARTESIAN_POINT('Ctrl Pts',(-55.3388810177386,2.22654671711671,
137.443692705233));
#219315=CARTESIAN_POINT('Ctrl Pts',(-55.6173286415515,6.78936100803939,
132.519824973462));
#219316=CARTESIAN_POINT('Ctrl Pts',(-55.8957762653644,5.11308421129812,
126.019529303714));
#219317=CARTESIAN_POINT('Ctrl Pts',(-56.1742238891773,-1.26186718757599,
123.916259859391));
#219318=CARTESIAN_POINT('Ctrl Pts',(-56.4526715129901,-6.47722428670686,
128.142818509401));
#219319=CARTESIAN_POINT('Ctrl Pts',(-56.7311191368031,-5.74032869635189,
134.815204333253));
#219320=CARTESIAN_POINT('Ctrl Pts',(-57.0095667606159,0.271648535303317,
137.801820722997));
#219321=CARTESIAN_POINT('Ctrl Pts',(-57.2880143844289,6.03399403378365,
134.358113120779));
#219322=CARTESIAN_POINT('Ctrl Pts',(-57.5664620082417,6.25139379221294,
127.64868057857));
#219323=CARTESIAN_POINT('Ctrl Pts',(-57.8449096320546,0.724068053163303,
123.839163828657));
#219324=CARTESIAN_POINT('Ctrl Pts',(-58.1233572558676,-5.46864085405239,
126.430322658971));
#219325=CARTESIAN_POINT('Ctrl Pts',(-58.4018048796803,-6.63593597435208,
133.0410086896));
#219326=CARTESIAN_POINT('Ctrl Pts',(-58.6802525034934,-1.705130117717,137.596324408362));
#219327=CARTESIAN_POINT('Ctrl Pts',(-58.9587001273061,4.79260701686295,
135.910157209259));
#219328=CARTESIAN_POINT('Ctrl Pts',(-59.2371477511191,6.88617243481463,
129.532012374421));
#219329=CARTESIAN_POINT('Ctrl Pts',(-59.515595374932,2.65168179339722,124.323093417365));
#219330=CARTESIAN_POINT('Ctrl Pts',(-59.7940429987449,-4.01957487429483,
125.070142389788));
#219331=CARTESIAN_POINT('Ctrl Pts',(-60.0724906225578,-6.99703859965941,
131.086657781405));
#219332=CARTESIAN_POINT('Ctrl Pts',(-60.3509382463707,-3.5445656762756,
136.843755870437));
#219333=CARTESIAN_POINT('Ctrl Pts',(-60.6293858701835,3.16518994194552,
137.050944762941));
#219334=CARTESIAN_POINT('Ctrl Pts',(-60.9078334939965,6.96629063164357,
131.517827988445));
#219335=CARTESIAN_POINT('Ctrl Pts',(-61.1862811178092,4.36571055307847,
125.32906955493));
#219336=CARTESIAN_POINT('Ctrl Pts',(-61.4647287416223,-2.24674424694855,
124.171836125139));
#219337=CARTESIAN_POINT('Ctrl Pts',(-61.743176365435,-6.79455084358828,
129.109568687053));
#219338=CARTESIAN_POINT('Ctrl Pts',(-62.0216239892481,-5.09849714723216,
135.60473223792));
#219339=CARTESIAN_POINT('Ctrl Pts',(-62.3000716130609,1.2828263519976,137.688588780872));
#219340=CARTESIAN_POINT('Ctrl Pts',(-62.5785192368738,6.48529510329292,
133.446175954988));
#219341=CARTESIAN_POINT('Ctrl Pts',(-62.8569668606868,5.72809447894126,
126.776063893867));
#219342=CARTESIAN_POINT('Ctrl Pts',(-63.1354144844995,-0.292945138585431,
123.80775972859));
#219343=CARTESIAN_POINT('Ctrl Pts',(-63.4138621083125,-6.04478248491762,
127.268989977326));
#219344=CARTESIAN_POINT('Ctrl Pts',(-63.6923097321254,-6.24176003165182,
133.979053131985));
#219345=CARTESIAN_POINT('Ctrl Pts',(-63.9707573559382,-0.702865036227365,
137.771728958244));
#219346=CARTESIAN_POINT('Ctrl Pts',(-64.2492049797512,5.48192859062395,
135.161733654286));
#219347=CARTESIAN_POINT('Ctrl Pts',(-64.527652603564,6.62909764979204,128.547525399088));
#219348=CARTESIAN_POINT('Ctrl Pts',(-64.806100227377,1.68444981822529,124.007238457143));
#219349=CARTESIAN_POINT('Ctrl Pts',(-65.0845478511898,-4.80812510634223,
125.713174722747));
#219350=CARTESIAN_POINT('Ctrl Pts',(-65.3629954750027,-6.88226794815085,
132.097662107432));
#219351=CARTESIAN_POINT('Ctrl Pts',(-65.6414430988157,-2.63194276308962,
137.29366860422));
#219352=CARTESIAN_POINT('Ctrl Pts',(-65.9198907226284,4.03700924369883,
136.526318081592));
#219353=CARTESIAN_POINT('Ctrl Pts',(-66.1983383464414,6.99614697439381,
130.500768182686));
#219354=CARTESIAN_POINT('Ctrl Pts',(-66.4767859702543,3.5261674164012,124.75420490012));
#219355=CARTESIAN_POINT('Ctrl Pts',(-66.7552335940671,-3.18418773440913,
124.567439155348));
#219356=CARTESIAN_POINT('Ctrl Pts',(-67.0336812178801,-6.96842991351606,
130.112099543802));
#219357=CARTESIAN_POINT('Ctrl Pts',(-67.3121288416929,-4.34902542882876,
136.292914040211));
#219358=CARTESIAN_POINT('Ctrl Pts',(-67.5905764655059,2.26692096324861,
137.43001607195));
#219359=CARTESIAN_POINT('Ctrl Pts',(-67.8690240893187,6.79967773534632,
132.478464422373));
#219360=CARTESIAN_POINT('Ctrl Pts',(-68.1474717131316,5.08386285138514,
125.988493160695));
#219361=CARTESIAN_POINT('Ctrl Pts',(-68.4259193369445,-1.30377363249137,
123.924068823677));
#219362=CARTESIAN_POINT('Ctrl Pts',(-68.7043669607574,-6.49330584099122,
128.182296524302));
#219363=CARTESIAN_POINT('Ctrl Pts',(-68.9828145845703,-5.71580719724563,
134.850073031684));
#219364=CARTESIAN_POINT('Ctrl Pts',(-69.2612622083832,0.314239028063776,
137.800037474531));
#219365=CARTESIAN_POINT('Ctrl Pts',(-69.5397098321961,6.05551493801243,
134.32131664364));
#219366=CARTESIAN_POINT('Ctrl Pts',(-69.818157456009,6.23206844827842,127.610685037641));
#219367=CARTESIAN_POINT('Ctrl Pts',(-70.0966050798218,0.681655508046095,
123.834885269867));
#219368=CARTESIAN_POINT('Ctrl Pts',(-70.3750527036349,-5.49516554335789,
126.463692868828));
#219369=CARTESIAN_POINT('Ctrl Pts',(-70.6535003274475,-6.62219791417695,
133.081362075471));
#219370=CARTESIAN_POINT('Ctrl Pts',(-70.9319479512606,-1.66375391422059,
137.606578180005));
#219371=CARTESIAN_POINT('Ctrl Pts',(-71.2103955750734,4.82359865400735,
135.880888651457));
#219372=CARTESIAN_POINT('Ctrl Pts',(-71.4888431988863,6.87829970509706,
129.490117861946));
#219373=CARTESIAN_POINT('Ctrl Pts',(-71.7672908226993,2.6121793508235,124.307071960521));
#219374=CARTESIAN_POINT('Ctrl Pts',(-72.045738446512,-4.05440621480077,
125.094716924722));
#219375=CARTESIAN_POINT('Ctrl Pts',(-72.3241860703251,-6.99519053777849,
131.129245511046));
#219376=CARTESIAN_POINT('Ctrl Pts',(-72.6026336941378,-3.5077364905931,
136.865220751771));
#219377=CARTESIAN_POINT('Ctrl Pts',(-72.8810813179508,3.20315602899298,
137.031561618638));
#219378=CARTESIAN_POINT('Ctrl Pts',(-73.1595289417638,6.97050464080582,
131.475408981201));
#219379=CARTESIAN_POINT('Ctrl Pts',(-73.4379765655765,4.33230001580124,
125.302595680118));
#219380=CARTESIAN_POINT('Ctrl Pts',(-73.7164241893894,-2.28707667910305,
124.18563558039));
#219381=CARTESIAN_POINT('Ctrl Pts',(-73.9948718132024,-6.80474163581863,
129.150960447132));
#219382=CARTESIAN_POINT('Ctrl Pts',(-74.2733194370152,-5.0691814593271,
135.635679297414));
#219383=CARTESIAN_POINT('Ctrl Pts',(-74.5517670608282,1.32470883500465,
137.680652303954));
#219384=CARTESIAN_POINT('Ctrl Pts',(-74.830214684641,6.5012564255912,133.406649176227));
#219385=CARTESIAN_POINT('Ctrl Pts',(-75.108662308454,5.70346696509291,126.741269991954));
#219386=CARTESIAN_POINT('Ctrl Pts',(-75.3871099322667,-0.335530006474783,
123.809672599606));
#219387=CARTESIAN_POINT('Ctrl Pts',(-75.6655575560798,-6.06619129364391,
127.305851786256));
#219388=CARTESIAN_POINT('Ctrl Pts',(-75.9440051798925,-6.22231913187452,
134.016989677222));
#219389=CARTESIAN_POINT('Ctrl Pts',(-76.2224528037055,-0.66043966510086,
137.775878408018));
#219390=CARTESIAN_POINT('Ctrl Pts',(-76.5009004275184,5.50835158962877,
135.128282866967));
#219391=CARTESIAN_POINT('Ctrl Pts',(-76.7793480513312,6.61523683142527,
128.507214014061));
#219392=CARTESIAN_POINT('Ctrl Pts',(-77.0577956751442,1.64304259742666,
123.997110667925));
#219393=CARTESIAN_POINT('Ctrl Pts',(-77.336243298957,-4.83902751651344,
125.742537472861));
#219394=CARTESIAN_POINT('Ctrl Pts',(-77.6146909227699,-6.87426774241415,
132.139532463972));
#219395=CARTESIAN_POINT('Ctrl Pts',(-77.8931385465828,-2.59239173968542,
137.309569755007));
#219396=CARTESIAN_POINT('Ctrl Pts',(-78.1715861703958,4.07176562643718,
136.501637645866));
#219397=CARTESIAN_POINT('Ctrl Pts',(-78.4500337942086,6.99416929867323,
130.458186275174));
#219398=CARTESIAN_POINT('Ctrl Pts',(-78.7284814180215,3.48927306959449,
124.732852213582));
#219399=CARTESIAN_POINT('Ctrl Pts',(-79.0069290418344,-3.22209464997582,
124.586937765577));
#219400=CARTESIAN_POINT('Ctrl Pts',(-79.2853766656473,-6.97251479429268,
130.154531180556));
#219401=CARTESIAN_POINT('Ctrl Pts',(-79.5638242894601,-4.3155344689392,
136.319286102215));
#219402=CARTESIAN_POINT('Ctrl Pts',(-79.8422719132732,2.30721120779087,
137.416093922569));
#219403=CARTESIAN_POINT('Ctrl Pts',(-80.1207195370859,6.80974249809405,
132.437041836753));
#219404=CARTESIAN_POINT('Ctrl Pts',(-80.3991671608989,5.0544531070646,125.957635471416));
#219405=CARTESIAN_POINT('Ctrl Pts',(-80.6776147847117,-1.34563176559565,
123.932132739704));
#219406=CARTESIAN_POINT('Ctrl Pts',(-80.9560624085247,-6.50914678343976,
128.221871700751));
#219407=CARTESIAN_POINT('Ctrl Pts',(-81.2345100323374,-5.69107389680138,
134.884791814753));
#219408=CARTESIAN_POINT('Ctrl Pts',(-81.5129576561506,0.356817876581242,
137.797994998686));
#219409=CARTESIAN_POINT('Ctrl Pts',(-81.7914052799631,6.07681145290804,
134.284389844403));
#219410=CARTESIAN_POINT('Ctrl Pts',(-82.0698529037763,6.21251217275584,
127.572807839535));
#219411=CARTESIAN_POINT('Ctrl Pts',(-82.348300527589,0.639217703933302,
123.830864967548));
#219412=CARTESIAN_POINT('Ctrl Pts',(-82.626748151402,-5.52148660728364,
126.497223923725));
#219413=CARTESIAN_POINT('Ctrl Pts',(-82.9051957752149,-6.60821446602265,
133.121631086217));
#219414=CARTESIAN_POINT('Ctrl Pts',(-83.1836433990278,-1.62231605971109,
137.616579892973));
#219415=CARTESIAN_POINT('Ctrl Pts',(-83.4620910228406,4.85441155092967,
135.851431981043));
#219416=CARTESIAN_POINT('Ctrl Pts',(-83.7405386466535,6.87017209745416,
129.448272049221));
#219417=CARTESIAN_POINT('Ctrl Pts',(-84.0189862704665,2.57258011298421,
124.291291263097));
#219418=CARTESIAN_POINT('Ctrl Pts',(-84.2974338942792,-4.08908731779306,
125.119503032603));
#219419=CARTESIAN_POINT('Ctrl Pts',(-84.5758815180923,-6.99308326653956,
131.171821201958));
#219420=CARTESIAN_POINT('Ctrl Pts',(-84.8543291419051,-3.47077732444568,
136.886461045702));
#219421=CARTESIAN_POINT('Ctrl Pts',(-85.132776765718,3.2410034219148,137.011947723114));
#219422=CARTESIAN_POINT('Ctrl Pts',(-85.4112243895309,6.97446035535538,
131.432965108015));
#219423=CARTESIAN_POINT('Ctrl Pts',(-85.6896720133437,4.29872894355427,
125.27632567523));
#219424=CARTESIAN_POINT('Ctrl Pts',(-85.9681196371569,-2.327324362789,124.19968029493));
#219425=CARTESIAN_POINT('Ctrl Pts',(-86.2465672609694,-6.81468027584547,
129.192413474561));
#219426=CARTESIAN_POINT('Ctrl Pts',(-86.5250148847825,-5.03967793103904,
135.666447330617));
#219427=CARTESIAN_POINT('Ctrl Pts',(-86.8034625085954,1.36654223043768,
137.672461023519));
#219428=CARTESIAN_POINT('Ctrl Pts',(-87.0819101324082,6.51697684144191,
133.367025968708));
#219429=CARTESIAN_POINT('Ctrl Pts',(-87.3603577562212,5.67862810717874,
126.706626649358));
#219430=CARTESIAN_POINT('Ctrl Pts',(-87.638805380034,-0.378102441176264,
123.811844661359));
#219431=CARTESIAN_POINT('Ctrl Pts',(-87.917253003847,-6.08737531742114,
127.342843233717));
#219432=CARTESIAN_POINT('Ctrl Pts',(-88.1957006276599,-6.20264766177327,
134.054807177307));
#219433=CARTESIAN_POINT('Ctrl Pts',(-88.4741482514726,-0.617989821139493,
137.779769525637));
#219434=CARTESIAN_POINT('Ctrl Pts',(-88.7525958752857,5.53457047463998,
135.094671855119));
#219435=CARTESIAN_POINT('Ctrl Pts',(-89.0310434990984,6.6011308830247,128.466987750645));
#219436=CARTESIAN_POINT('Ctrl Pts',(-89.3094911229114,1.60157449308101,
123.987235123859));
#219437=CARTESIAN_POINT('Ctrl Pts',(-89.5879387467241,-4.86975061474005,
125.772087790693));
#219438=CARTESIAN_POINT('Ctrl Pts',(-89.8663863705374,-6.8660128081587,
132.181353345229));
#219439=CARTESIAN_POINT('Ctrl Pts',(-90.1448339943499,-2.55274465425183,
137.325229852876));
#219440=CARTESIAN_POINT('Ctrl Pts',(-90.4232816181632,4.10637112840284,
136.476746095445));
#219441=CARTESIAN_POINT('Ctrl Pts',(-90.7017292419757,6.99193245143733,
130.415617195278));
#219442=CARTESIAN_POINT('Ctrl Pts',(-90.9801768657889,3.45224942649073,
124.711724509022));
#219443=CARTESIAN_POINT('Ctrl Pts',(-91.2586244896016,-3.2598821696406,
124.606666764696));
#219444=CARTESIAN_POINT('Ctrl Pts',(-91.5370721134145,-6.97634130596949,
130.196986896981));
#219445=CARTESIAN_POINT('Ctrl Pts',(-91.8155197372274,-4.28188359533257,
136.345453806627));
#219446=CARTESIAN_POINT('Ctrl Pts',(-92.0939673610402,2.34741595777304,
137.401926772977));
#219447=CARTESIAN_POINT('Ctrl Pts',(-92.3724149848533,6.81955492332935,
132.395558751529));
#219448=CARTESIAN_POINT('Ctrl Pts',(-92.650862608666,5.02485606812542,125.926957379319));
#219449=CARTESIAN_POINT('Ctrl Pts',(-92.929310232479,-1.38744003581995,
123.940451308663));
#219450=CARTESIAN_POINT('Ctrl Pts',(-93.2077578562919,-6.52474652706058,
128.261542572277));
#219451=CARTESIAN_POINT('Ctrl Pts',(-93.4862054801047,-5.66612971152105,
134.919359395943));
#219452=CARTESIAN_POINT('Ctrl Pts',(-93.7646531039176,0.39938350308132,
137.795693371147));
#219453=CARTESIAN_POINT('Ctrl Pts',(-94.0431007277306,6.09788278932073,
134.247334091402));
#219454=CARTESIAN_POINT('Ctrl Pts',(-94.3215483515434,6.19272569030992,
127.535050387806));
#219455=CARTESIAN_POINT('Ctrl Pts',(-94.5999959753563,0.596756213373149,
123.827103070676));
#219456=CARTESIAN_POINT('Ctrl Pts',(-94.8784435991693,-5.54760307049237,
126.530914581157));
#219457=CARTESIAN_POINT('Ctrl Pts',(-95.1568912229821,-6.59398614805128,
133.161814229653));
#219458=CARTESIAN_POINT('Ctrl Pts',(-95.4353388467949,-1.58081808968337,
137.626329176652));
#219459=CARTESIAN_POINT('Ctrl Pts',(-95.7137864706081,4.88504456584684,
135.821788289543));
#219460=CARTESIAN_POINT('Ctrl Pts',(-95.9922340944205,6.86178991305786,
129.406476486855));
#219461=CARTESIAN_POINT('Ctrl Pts',(-96.2706817182339,2.53288554724217,
124.275751909854));
#219462=CARTESIAN_POINT('Ctrl Pts',(-96.5491293420464,-4.12361689815126,
125.144499794972));
#219463=CARTESIAN_POINT('Ctrl Pts',(-96.8275769658595,-6.99071686402826,
131.214383276482));
#219464=CARTESIAN_POINT('Ctrl Pts',(-97.1060245896722,-3.4336895473684,
136.907475965166));
#219465=CARTESIAN_POINT('Ctrl Pts',(-97.3844722134854,3.27873071826322,
136.992103803166));
#219466=CARTESIAN_POINT('Ctrl Pts',(-97.6629198372979,6.9781576287114,131.390497941658));
#219467=CARTESIAN_POINT('Ctrl Pts',(-97.9413674611112,4.26499858032525,
125.250260513709));
#219468=CARTESIAN_POINT('Ctrl Pts',(-98.2198150849237,-2.36748580661544,
124.21396974833));
#219469=CARTESIAN_POINT('Ctrl Pts',(-98.498262708737,-6.82436639538843,
129.233926233285));
#219470=CARTESIAN_POINT('Ctrl Pts',(-98.7767103325495,-5.00998765563179,
135.69703519741));
#219471=CARTESIAN_POINT('Ctrl Pts',(-99.0551579563628,1.40832498814648,
137.664015243098));
#219472=CARTESIAN_POINT('Ctrl Pts',(-99.3336055801754,6.53245576831905,
133.327307800681));
#219473=CARTESIAN_POINT('Ctrl Pts',(-99.6120532039884,5.65357882561176,
126.672135149802));
#219474=CARTESIAN_POINT('Ctrl Pts',(-99.8905008278013,-0.420660865152761,
123.814275833361));
#219475=CARTESIAN_POINT('Ctrl Pts',(-100.168948451614,-6.10833377126732,
127.379962948978));
#219476=CARTESIAN_POINT('Ctrl Pts',(-100.447396075427,-6.18274635028192,
134.092504230901));
#219477=CARTESIAN_POINT('Ctrl Pts',(-100.72584369924,-0.575517077338011,
137.783402166914));
#219478=CARTESIAN_POINT('Ctrl Pts',(-101.004291323053,5.56058427410689,
135.060901864211));
#219479=CARTESIAN_POINT('Ctrl Pts',(-101.282738946866,6.58678032729173,
128.426848099441));
#219480=CARTESIAN_POINT('Ctrl Pts',(-101.561186570679,1.56004704180311,
123.977612190885));
#219481=CARTESIAN_POINT('Ctrl Pts',(-101.839634194492,-4.90029326256724,
125.801824581246));
#219482=CARTESIAN_POINT('Ctrl Pts',(-102.118081818304,-6.85750345127332,
132.223123201514));
#219483=CARTESIAN_POINT('Ctrl Pts',(-102.396529442117,-2.51300297592632,
137.340648317539));
#219484=CARTESIAN_POINT('Ctrl Pts',(-102.67497706593,4.14082446727623,136.451644352694));
#219485=CARTESIAN_POINT('Ctrl Pts',(-102.953424689743,6.98943651557314,
130.373062520413));
#219486=CARTESIAN_POINT('Ctrl Pts',(-103.231872313556,3.41509785901489,
124.690822569333));
#219487=CARTESIAN_POINT('Ctrl Pts',(-103.510319937369,-3.29754889317273,
124.626625421641));
#219488=CARTESIAN_POINT('Ctrl Pts',(-103.788767561182,-6.97990930675369,
130.239465119861));
#219489=CARTESIAN_POINT('Ctrl Pts',(-104.067215184995,-4.24807405495459,
136.371416183792));
#219490=CARTESIAN_POINT('Ctrl Pts',(-104.345662808808,2.38753372339306,
137.387515148146));
#219491=CARTESIAN_POINT('Ctrl Pts',(-104.62411043262,6.82911464744894,132.354016703874));
#219492=CARTESIAN_POINT('Ctrl Pts',(-104.902558056433,4.99507283129728,
125.896460021193));
#219493=CARTESIAN_POINT('Ctrl Pts',(-105.181005680246,-1.42919689394351,
123.949024222305));
#219494=CARTESIAN_POINT('Ctrl Pts',(-105.459453304059,-6.54010449379936,
128.301307668861));
#219495=CARTESIAN_POINT('Ctrl Pts',(-105.737900927872,-5.64097556572054,
134.953774494342));
#219496=CARTESIAN_POINT('Ctrl Pts',(-106.016348551685,0.441934330278796,
137.793132677202));
#219497=CARTESIAN_POINT('Ctrl Pts',(-106.294796175498,6.11872816644418,
134.210150757753));
#219498=CARTESIAN_POINT('Ctrl Pts',(-106.573243799311,6.17270973413615,
127.49741408157));
#219499=CARTESIAN_POINT('Ctrl Pts',(-106.851691423124,0.554272609792058,
123.823599718647));
#219500=CARTESIAN_POINT('Ctrl Pts',(-107.130139046936,-5.57351396522919,
126.564763592701));
#219501=CARTESIAN_POINT('Ctrl Pts',(-107.40858667075,-6.57951348749827,
133.201910016778));
#219502=CARTESIAN_POINT('Ctrl Pts',(-107.687034294562,-1.53926154185996,
137.635825669776));
#219503=CARTESIAN_POINT('Ctrl Pts',(-107.965481918375,4.91549656364115,
135.791958675416));
#219504=CARTESIAN_POINT('Ctrl Pts',(-108.243929542188,6.85315346251289,
129.364732723601));
#219505=CARTESIAN_POINT('Ctrl Pts',(-108.522377166001,2.49309712449469,
124.260454476607));
#219506=CARTESIAN_POINT('Ctrl Pts',(-108.800824789814,-4.15799367636883,
125.169706285567));
#219507=CARTESIAN_POINT('Ctrl Pts',(-109.079272413627,-6.98809141793296,
131.256930157466));
#219508=CARTESIAN_POINT('Ctrl Pts',(-109.35772003744,-3.39647453366164,
136.928264731447));
#219509=CARTESIAN_POINT('Ctrl Pts',(-109.636167661252,3.31633652003941,
136.97203059412));
#219510=CARTESIAN_POINT('Ctrl Pts',(-109.914615285065,6.98159632387027,
131.348009055767));
#219511=CARTESIAN_POINT('Ctrl Pts',(-110.193062908878,4.23111017600536,
125.22440116141));
#219512=CARTESIAN_POINT('Ctrl Pts',(-110.471510532691,-2.40755952238467,
124.228503411086));
#219513=CARTESIAN_POINT('Ctrl Pts',(-110.749958156504,-6.83379963552497,
129.275497185033));
#219514=CARTESIAN_POINT('Ctrl Pts',(-111.028405780317,-4.98011173328953,
135.727441764346));
#219515=CARTESIAN_POINT('Ctrl Pts',(-111.30685340413,1.45005555985492,137.655315275653));
#219516=CARTESIAN_POINT('Ctrl Pts',(-111.585301027943,6.54769263264538,
133.287496143919));
#219517=CARTESIAN_POINT('Ctrl Pts',(-111.863748651756,5.62832004860235,
126.63779677138));
#219518=CARTESIAN_POINT('Ctrl Pts',(-112.142196275568,-0.463203701385527,
123.816966025527));
#219519=CARTESIAN_POINT('Ctrl Pts',(-112.420643899382,-6.12906587855929,
127.417209556553));
#219520=CARTESIAN_POINT('Ctrl Pts',(-112.699091523194,-6.16261593485082,
134.130079441122));
#219521=CARTESIAN_POINT('Ctrl Pts',(-112.977539147007,-0.533023007539609,
137.786776197239));
#219522=CARTESIAN_POINT('Ctrl Pts',(-113.25598677082,5.58639202407863,135.026974145601));
#219523=CARTESIAN_POINT('Ctrl Pts',(-113.534434394633,6.57218569599142,
128.386796547837));
#219524=CARTESIAN_POINT('Ctrl Pts',(-113.812882018446,1.5184617824084,123.968242225583));
#219525=CARTESIAN_POINT('Ctrl Pts',(-114.091329642259,-4.93065432822552,
125.831746742611));
#219526=CARTESIAN_POINT('Ctrl Pts',(-114.369777266072,-6.84873998707567,
132.26484048503));
#219527=CARTESIAN_POINT('Ctrl Pts',(-114.648224889884,-2.4731681773514,
137.355824577657));
#219528=CARTESIAN_POINT('Ctrl Pts',(-114.926672513697,4.17512436637621,
136.426333347767));
#219529=CARTESIAN_POINT('Ctrl Pts',(-115.20512013751,6.98668158356849,130.330523827459));
#219530=CARTESIAN_POINT('Ctrl Pts',(-115.483567761323,3.377819743832,124.670147169045));
#219531=CARTESIAN_POINT('Ctrl Pts',(-115.762015385136,-3.33509342481799,
124.646812996834));
#219532=CARTESIAN_POINT('Ctrl Pts',(-116.040463008949,-6.98321866443162,
130.281964275151));
#219533=CARTESIAN_POINT('Ctrl Pts',(-116.318910632762,-4.21410710063033,
136.397172271667));
#219534=CARTESIAN_POINT('Ctrl Pts',(-116.597358256575,2.42756301807353,
137.372859582102));
#219535=CARTESIAN_POINT('Ctrl Pts',(-116.875805880388,6.83842131621399,
132.312417233142));
#219536=CARTESIAN_POINT('Ctrl Pts',(-117.154253504201,4.96510450020791,
125.866144527128));
#219537=CARTESIAN_POINT('Ctrl Pts',(-117.432701128013,-1.47090079265054,
123.957851162959));
#219538=CARTESIAN_POINT('Ctrl Pts',(-117.711148751826,-6.55522011456102,
128.341165516992));
#219539=CARTESIAN_POINT('Ctrl Pts',(-117.989596375639,-5.61561239149597,
134.988035834682));
#219540=CARTESIAN_POINT('Ctrl Pts',(-118.268043999452,0.484468781437156,
137.790313011739));
#219541=CARTESIAN_POINT('Ctrl Pts',(-118.546491623265,6.13934681184524,
134.172841221298));
#219542=CARTESIAN_POINT('Ctrl Pts',(-118.824939247078,6.15246504593319,
127.459900315453));
#219543=CARTESIAN_POINT('Ctrl Pts',(-119.103386870891,0.511768467435545,
123.820355041281));
#219544=CARTESIAN_POINT('Ctrl Pts',(-119.381834494704,-5.59921833135585,
126.598769704074));
#219545=CARTESIAN_POINT('Ctrl Pts',(-119.660282118516,-6.56479702065358,
133.241916961827));
#219546=CARTESIAN_POINT('Ctrl Pts',(-119.93872974233,-1.49764795613459,
137.645069020452));
#219547=CARTESIAN_POINT('Ctrl Pts',(-120.217177366142,4.94576641590264,
135.761944244007));
#219548=CARTESIAN_POINT('Ctrl Pts',(-120.495624989955,6.84426306584611,
129.323042306287));
#219549=CARTESIAN_POINT('Ctrl Pts',(-120.774072613768,2.45321631911644,
124.245399530209));
#219550=CARTESIAN_POINT('Ctrl Pts',(-121.052520237581,-4.19221637860163,
125.195121570349));
#219551=CARTESIAN_POINT('Ctrl Pts',(-121.330967861394,-6.98520702554029,
131.299460268319));
#219552=CARTESIAN_POINT('Ctrl Pts',(-121.609415485207,-3.35913366234199,
136.948826574209));
#219553=CARTESIAN_POINT('Ctrl Pts',(-121.88786310902,3.3538194337463,136.951728839794));
#219554=CARTESIAN_POINT('Ctrl Pts',(-122.166310732833,6.98477631340985,
131.305500024783));
#219555=CARTESIAN_POINT('Ctrl Pts',(-122.444758356646,4.19706498634193,
125.198748576561));
#219556=CARTESIAN_POINT('Ctrl Pts',(-122.723205980458,-2.44754402515043,
124.24328074465));
#219557=CARTESIAN_POINT('Ctrl Pts',(-123.001653604271,-6.84297964670285,
129.317124789377));
#219558=CARTESIAN_POINT('Ctrl Pts',(-123.280101228084,-4.95005127107555,
135.7576659047));
#219559=CARTESIAN_POINT('Ctrl Pts',(-123.558548851897,1.49173239922134,
137.646361443563));
#219560=CARTESIAN_POINT('Ctrl Pts',(-123.83699647571,6.5626868698133,133.247592473656));
#219561=CARTESIAN_POINT('Ctrl Pts',(-124.115444099523,5.60285271212367,
126.603612786514));
#219562=CARTESIAN_POINT('Ctrl Pts',(-124.393891723336,-0.505729373435472,
123.819915138168));
#219563=CARTESIAN_POINT('Ctrl Pts',(-124.672339347149,-6.14957087106115,
127.454581676257));
#219564=CARTESIAN_POINT('Ctrl Pts',(-124.950786970961,-6.14225716141998,
134.167531415611));
#219565=CARTESIAN_POINT('Ctrl Pts',(-125.229234594775,-0.490509186377616,
137.789891491587));
#219566=CARTESIAN_POINT('Ctrl Pts',(-125.507682218587,5.6119927682395,134.992889956494));
#219567=CARTESIAN_POINT('Ctrl Pts',(-125.786129842401,6.55734752993325,
128.346834579959));
#219568=CARTESIAN_POINT('Ctrl Pts',(-126.064577466213,1.47682025585389,
123.959125575163));
#219569=CARTESIAN_POINT('Ctrl Pts',(-126.343025090026,-4.9608326866744,
125.861853166013));
#219570=CARTESIAN_POINT('Ctrl Pts',(-126.621472713839,-6.8397227402992,
132.306503649927));
#219571=CARTESIAN_POINT('Ctrl Pts',(-126.899920337652,-2.43324173462049,
137.370758070868));
#219572=CARTESIAN_POINT('Ctrl Pts',(-127.178367961465,4.20926955470684,
136.400814018573));
#219573=CARTESIAN_POINT('Ctrl Pts',(-127.456815585278,6.98366775750873,
130.288002692701));
#219574=CARTESIAN_POINT('Ctrl Pts',(-127.73526320909,3.34041646229627,124.649699074291));
#219575=CARTESIAN_POINT('Ctrl Pts',(-128.013710832904,-3.37251437334987,
124.66722874222));
#219576=CARTESIAN_POINT('Ctrl Pts',(-128.292158456716,-6.9862692563739,
130.324482788031));
#219577=CARTESIAN_POINT('Ctrl Pts',(-128.570606080529,-4.17998399101771,
136.422721115849));
#219578=CARTESIAN_POINT('Ctrl Pts',(-128.849053704342,2.46750235851359,
137.357960617914));
#219579=CARTESIAN_POINT('Ctrl Pts',(-129.127501328155,6.84747458476236,
132.270761880817));
#219580=CARTESIAN_POINT('Ctrl Pts',(-129.405948951968,4.93495218534535,
125.836012020477));
#219581=CARTESIAN_POINT('Ctrl Pts',(-129.684396575781,-1.51255018658779,
123.966931803538));
#219582=CARTESIAN_POINT('Ctrl Pts',(-129.962844199593,-6.57009282923063,
128.381114639724));
#219583=CARTESIAN_POINT('Ctrl Pts',(-130.241291823406,-5.59004112868908,
135.022142147398));
#219584=CARTESIAN_POINT('Ctrl Pts',(-130.519739447219,0.52698528042665,
137.78723447924));
#219585=CARTESIAN_POINT('Ctrl Pts',(-130.798187071032,6.15973796149245,
134.135406864555));
#219586=CARTESIAN_POINT('Ctrl Pts',(-131.076634694845,6.13199237587537,
127.422510479544));
#219587=CARTESIAN_POINT('Ctrl Pts',(-131.355082318658,0.4692453613103,123.81736915881));
#219588=CARTESIAN_POINT('Ctrl Pts',(-131.633529942471,-5.62471521638866,
126.632931655165));
#219589=CARTESIAN_POINT('Ctrl Pts',(-131.911977566284,-6.54983729284086,
133.281833582332));
#219590=CARTESIAN_POINT('Ctrl Pts',(-132.190425190097,-1.45597887451291,
137.654058886162));
#219591=CARTESIAN_POINT('Ctrl Pts',(-132.46887281391,4.97585300097076,135.731746107516));
#219592=CARTESIAN_POINT('Ctrl Pts',(-132.747320437723,6.83511905249447,
129.281406779768));
#219593=CARTESIAN_POINT('Ctrl Pts',(-133.025768061535,2.4132446089053,124.230587628526));
#219594=CARTESIAN_POINT('Ctrl Pts',(-133.304215685348,-4.22628373671482,
125.220744707546));
#219595=CARTESIAN_POINT('Ctrl Pts',(-133.582663309161,-6.98206379373247,
131.341972033073));
#219596=CARTESIAN_POINT('Ctrl Pts',(-133.861110932974,-3.32166831708915,
136.969160731525));
#219597=CARTESIAN_POINT('Ctrl Pts',(-134.139558556787,3.39117807044069,
136.931199292478));
#219598=CARTESIAN_POINT('Ctrl Pts',(-134.4180061806,6.98769747949419,131.262972423894));
#219599=CARTESIAN_POINT('Ctrl Pts',(-134.696453804413,4.16286427289247,
125.173303709728));
#219600=CARTESIAN_POINT('Ctrl Pts',(-134.974901428226,-2.48743783327188,
124.25830120144));
#219601=CARTESIAN_POINT('Ctrl Pts',(-135.253349052039,-6.85190608875344,
129.358807503792));
#219602=CARTESIAN_POINT('Ctrl Pts',(-135.531796675851,-4.91980738289134,
135.787706498505));
#219603=CARTESIAN_POINT('Ctrl Pts',(-135.810244299665,1.53335396189511,
137.637154078616));
#219604=CARTESIAN_POINT('Ctrl Pts',(-136.088691923477,6.57743792420584,
133.207598268539));
#219605=CARTESIAN_POINT('Ctrl Pts',(-136.36713954729,5.57717775987727,126.569584461903));
#219606=CARTESIAN_POINT('Ctrl Pts',(-136.645587171103,-0.548236305497475,
123.823123062006));
#219607=CARTESIAN_POINT('Ctrl Pts',(-136.924034794916,-6.1698479889529,
127.492077923251));
#219608=CARTESIAN_POINT('Ctrl Pts',(-137.202482418729,-6.12167078439119,
134.204858766568));
#219609=CARTESIAN_POINT('Ctrl Pts',(-137.480930042542,-0.447977189217358,
137.792747934521));
#219610=CARTESIAN_POINT('Ctrl Pts',(-137.759377666354,5.63738555794455,
134.958650559891));
#219611=CARTESIAN_POINT('Ctrl Pts',(-138.037825290167,6.54226637895086,
128.306963676612));
#219612=CARTESIAN_POINT('Ctrl Pts',(-138.31627291398,1.43512400518173,123.950262577445));
#219613=CARTESIAN_POINT('Ctrl Pts',(-138.594720537793,-4.99082721964375,
125.892142735845));
#219614=CARTESIAN_POINT('Ctrl Pts',(-138.873168161606,-6.83045204508126,
132.348111152362));
#219615=CARTESIAN_POINT('Ctrl Pts',(-139.151615785419,-2.39322512722196,
137.385448243807));
#219616=CARTESIAN_POINT('Ctrl Pts',(-139.430063409232,4.24325876700673,
136.375087310741));
#219617=CARTESIAN_POINT('Ctrl Pts',(-139.708511033045,6.98039514907165,
130.245500691775));
#219618=CARTESIAN_POINT('Ctrl Pts',(-139.986958656858,3.30288940040013,
124.629479042785));
#219619=CARTESIAN_POINT('Ctrl Pts',(-140.26540628067,-3.40981035212143,
124.687871901284));
#219620=CARTESIAN_POINT('Ctrl Pts',(-140.543853904484,-6.98906096953965,
130.36701908296));
#219621=CARTESIAN_POINT('Ctrl Pts',(-140.822301528296,-4.1457059905611,
136.448061769617));
#219622=CARTESIAN_POINT('Ctrl Pts',(-141.100749152109,2.50735026474636,
137.342818807668));
#219623=CARTESIAN_POINT('Ctrl Pts',(-141.379196775922,6.85627411762182,
132.229052190456));
#219624=CARTESIAN_POINT('Ctrl Pts',(-141.657644399735,4.90461700401472,
125.80606361781));
#219625=CARTESIAN_POINT('Ctrl Pts',(-141.936092023548,-1.5541435324211,
123.976265807557));
#219626=CARTESIAN_POINT('Ctrl Pts',(-142.214539647361,-6.58472208669408,
128.421153556726));
#219627=CARTESIAN_POINT('Ctrl Pts',(-142.492987271174,-5.56426272485295,
135.056092168669));
#219628=CARTESIAN_POINT('Ctrl Pts',(-142.771434894987,0.569482251782813,
137.783897193782));
#219629=CARTESIAN_POINT('Ctrl Pts',(-143.0498825188,6.17990085978423,134.097849074668));
#219630=CARTESIAN_POINT('Ctrl Pts',(-143.328330142612,6.11129248258502,
127.385245959334));
#219631=CARTESIAN_POINT('Ctrl Pts',(-143.606777766425,0.426704867125613,
123.814642181877));
#219632=CARTESIAN_POINT('Ctrl Pts',(-143.885225390238,-5.65000367553061,
126.667248180088));
#219633=CARTESIAN_POINT('Ctrl Pts',(-144.163673014051,-6.53463485839856,
133.321658399163));
#219634=CARTESIAN_POINT('Ctrl Pts',(-144.442120637864,-1.4142558410586,
137.662794933783));
#219635=CARTESIAN_POINT('Ctrl Pts',(-144.720568261677,5.00575520397605,
135.701365384942));
#219636=CARTESIAN_POINT('Ctrl Pts',(-144.99901588549,6.82572176129271,129.239827686864));
#219637=CARTESIAN_POINT('Ctrl Pts',(-145.277463509303,2.37318347502772,
124.216019320419));
#219638=CARTESIAN_POINT('Ctrl Pts',(-145.555911133116,-4.26019448832994,
125.246574747685));
#219639=CARTESIAN_POINT('Ctrl Pts',(-145.834358756928,-6.97866183898313,
131.384463876438));
#219640=CARTESIAN_POINT('Ctrl Pts',(-146.112806380741,-3.28407988619528,
136.989266449907));
#219641=CARTESIAN_POINT('Ctrl Pts',(-146.391254004554,3.42841104578457,
136.910442712901));
#219642=CARTESIAN_POINT('Ctrl Pts',(-146.669701628367,6.99035971387901,
131.220427828976));
#219643=CARTESIAN_POINT('Ctrl Pts',(-146.94814925218,4.12850930297597,125.148067503779));
#219644=CARTESIAN_POINT('Ctrl Pts',(-147.226596875993,-2.52723946847004,
124.27356422487));
#219645=CARTESIAN_POINT('Ctrl Pts',(-147.505044499806,-6.86057863090408,
129.400543783708));
#219646=CARTESIAN_POINT('Ctrl Pts',(-147.783492123619,-4.88938118943532,
135.817562432597));
#219647=CARTESIAN_POINT('Ctrl Pts',(-148.061939747432,1.57491870557395,
137.627693521995));
#219648=CARTESIAN_POINT('Ctrl Pts',(-148.340387371245,6.5919452492172,133.167515010566));
#219649=CARTESIAN_POINT('Ctrl Pts',(-148.618834995057,5.55129614325799,
126.535713058481));
#219650=CARTESIAN_POINT('Ctrl Pts',(-148.89728261887,-0.590722922461593,
123.826589678167));
#219651=CARTESIAN_POINT('Ctrl Pts',(-149.175730242683,-6.18989648085842,
127.529696908099));
#219652=CARTESIAN_POINT('Ctrl Pts',(-149.454177866496,-6.10085756660025,
134.242060110815));
#219653=CARTESIAN_POINT('Ctrl Pts',(-149.732625490309,-0.405428592098244,
137.795345420191));
#219654=CARTESIAN_POINT('Ctrl Pts',(-150.011073114122,5.66256945225453,
134.924257224548));
#219655=CARTESIAN_POINT('Ctrl Pts',(-150.289520737935,6.52694280188189,
128.267185315226));
#219656=CARTESIAN_POINT('Ctrl Pts',(-150.567968361748,1.39337457546175,
123.94165356085));
#219657=CARTESIAN_POINT('Ctrl Pts',(-150.84641598556,-5.02063681567507,
125.922614329717));
#219658=CARTESIAN_POINT('Ctrl Pts',(-151.124863609373,-6.8209282449509,
132.389661450552));
#219659=CARTESIAN_POINT('Ctrl Pts',(-151.403311233186,-2.35311983798619,
137.399894552124));
#219660=CARTESIAN_POINT('Ctrl Pts',(-151.681758856999,4.2770907437925,136.349154177582));
#219661=CARTESIAN_POINT('Ctrl Pts',(-151.960206480812,6.97686387952531,
130.20301939961));
#219662=CARTESIAN_POINT('Ctrl Pts',(-152.238654104625,3.26523994872261,
124.609487823786));
#219663=CARTESIAN_POINT('Ctrl Pts',(-152.517101728438,-3.44697997911642,
124.708741709087));
#219664=CARTESIAN_POINT('Ctrl Pts',(-152.795549352251,-6.99159370048095,
130.40957158374));
#219665=CARTESIAN_POINT('Ctrl Pts',(-153.073996976064,-4.11127436944443,
136.473193293963));
#219666=CARTESIAN_POINT('Ctrl Pts',(-153.352444599876,2.54710526019297,
137.327434712448));
#219667=CARTESIAN_POINT('Ctrl Pts',(-153.63089222369,6.86481958872245,132.187289707623));
#219668=CARTESIAN_POINT('Ctrl Pts',(-153.909339847502,4.87410008029735,
125.776300428876));
#219669=CARTESIAN_POINT('Ctrl Pts',(-154.187787471315,-1.5956792888948,
123.98585282914));
#219670=CARTESIAN_POINT('Ctrl Pts',(-154.466235095128,-6.5991073448593,
128.461280784342));
#219671=CARTESIAN_POINT('Ctrl Pts',(-154.744682718941,-5.53827813521478,
135.089884640464));
#219672=CARTESIAN_POINT('Ctrl Pts',(-155.023130342754,0.611958120764675,
137.78030127903));
#219673=CARTESIAN_POINT('Ctrl Pts',(-155.301577966567,6.19983475957701,
134.060169243357));
#219674=CARTESIAN_POINT('Ctrl Pts',(-155.58002559038,6.0903661331043,127.348108135675));
#219675=CARTESIAN_POINT('Ctrl Pts',(-155.858473214192,0.38414856123516,
123.812174211531));
#219676=CARTESIAN_POINT('Ctrl Pts',(-156.136920838005,-5.67508277170857,
126.701718007236));
#219677=CARTESIAN_POINT('Ctrl Pts',(-156.415368461818,-6.51919028065846,
133.3613899366));
#219678=CARTESIAN_POINT('Ctrl Pts',(-156.693816085631,-1.37248040183399,
137.671276839599));
#219679=CARTESIAN_POINT('Ctrl Pts',(-156.972263709444,5.03547191688086,
135.670803202055));
#219680=CARTESIAN_POINT('Ctrl Pts',(-157.250711333257,6.81607154046107,
129.198306568304));
#219681=CARTESIAN_POINT('Ctrl Pts',(-157.52915895707,2.33303440196427,124.201695145721));
#219682=CARTESIAN_POINT('Ctrl Pts',(-157.807606580883,-4.29394737687161,
125.272610733624));
#219683=CARTESIAN_POINT('Ctrl Pts',(-158.086054204696,-6.97500128735293,
131.426934223863));
#219684=CARTESIAN_POINT('Ctrl Pts',(-158.364501828508,-3.2463697625135,
137.009142984327));
#219685=CARTESIAN_POINT('Ctrl Pts',(-158.642949452322,3.46551698009634,
136.889459870208));
#219686=CARTESIAN_POINT('Ctrl Pts',(-158.921397076134,6.99276291791392,
131.177867816534));
#219687=CARTESIAN_POINT('Ctrl Pts',(-159.199844699947,4.09400134962899,
125.123040893851));
#219688=CARTESIAN_POINT('Ctrl Pts',(-159.47829232376,-2.56694745588028,
124.289069249361));
#219689=CARTESIAN_POINT('Ctrl Pts',(-159.756739947573,-6.86899695179061,
129.442332082575));
#219690=CARTESIAN_POINT('Ctrl Pts',(-160.035187571386,-4.85877381816122,
135.84723260065));
#219691=CARTESIAN_POINT('Ctrl Pts',(-160.313635195198,1.61642509006095,
137.617980124263));
#219692=CARTESIAN_POINT('Ctrl Pts',(-160.592082819012,6.60620830727321,
133.12734418504));
#219693=CARTESIAN_POINT('Ctrl Pts',(-160.870530442824,5.52520882131862,
126.501999831362));
#219694=CARTESIAN_POINT('Ctrl Pts',(-161.148978066638,-0.633187649970563,
123.830314858198));
#219695=CARTESIAN_POINT('Ctrl Pts',(-161.42742569045,-6.20971560387352,
127.567437236815));
#219696=CARTESIAN_POINT('Ctrl Pts',(-161.705873314263,-6.07981827928859,
134.279134069845));
#219697=CARTESIAN_POINT('Ctrl Pts',(-161.984320938076,-0.362864971672915,
137.79768385235));
#219698=CARTESIAN_POINT('Ctrl Pts',(-162.262768561889,5.68754351797111,
134.889711224922));
#219699=CARTESIAN_POINT('Ctrl Pts',(-162.541216185702,6.5113773665471,128.227500969805));
#219700=CARTESIAN_POINT('Ctrl Pts',(-162.819663809515,1.35157351373451,
123.93329884439));
#219701=CARTESIAN_POINT('Ctrl Pts',(-163.098111433328,-5.05026037016286,
125.953266818493));
#219702=CARTESIAN_POINT('Ctrl Pts',(-163.376559057141,-6.81115169281603,
132.431153004838));
#219703=CARTESIAN_POINT('Ctrl Pts',(-163.655006680953,-2.31292735302948,
137.414096460505));
#219704=CARTESIAN_POINT('Ctrl Pts',(-163.933454304766,4.31076423140788,
136.323015580059));
#219705=CARTESIAN_POINT('Ctrl Pts',(-164.211901928579,6.97307407972212,
130.160560390364));
#219706=CARTESIAN_POINT('Ctrl Pts',(-164.490349552392,3.2274695023783,124.589726158078));
#219707=CARTESIAN_POINT('Ctrl Pts',(-164.768797176205,-3.4840218770001,
124.729837392289));
#219708=CARTESIAN_POINT('Ctrl Pts',(-165.047244800018,-6.99386735534677,
130.452138713572));
#219709=CARTESIAN_POINT('Ctrl Pts',(-165.325692423831,-4.07669040354407,
136.498114757629));
#219710=CARTESIAN_POINT('Ctrl Pts',(-165.604140047644,2.58676587171747,
137.31180890232));
#219711=CARTESIAN_POINT('Ctrl Pts',(-165.882587671457,6.87311068140868,
132.145475979844));
#219712=CARTESIAN_POINT('Ctrl Pts',(-166.161035295269,4.84340254500906,
125.746723556562));
#219713=CARTESIAN_POINT('Ctrl Pts',(-166.439482919082,-1.63715591688565,
123.995692513036));
#219714=CARTESIAN_POINT('Ctrl Pts',(-166.717930542895,-6.61324807067504,
128.501494835643));
#219715=CARTESIAN_POINT('Ctrl Pts',(-166.996378166708,-5.5120883226436,
135.12351831059));
#219716=CARTESIAN_POINT('Ctrl Pts',(-167.274825790521,0.654411313413328,
137.776446868231));
#219717=CARTESIAN_POINT('Ctrl Pts',(-167.553273414334,6.21953892221278,
134.022368766858));
#219718=CARTESIAN_POINT('Ctrl Pts',(-167.831721038147,6.06921410286677,
127.311098384725));
#219719=CARTESIAN_POINT('Ctrl Pts',(-168.11016866196,0.3415780205785,123.809965339223));
#219720=CARTESIAN_POINT('Ctrl Pts',(-168.388616285773,-5.69995157560742,
126.736339859314));
#219721=CARTESIAN_POINT('Ctrl Pts',(-168.667063909585,-6.50350413192509,
133.401026722375));
#219722=CARTESIAN_POINT('Ctrl Pts',(-168.945511533399,-1.33065410484337,
137.679504289309));
#219723=CARTESIAN_POINT('Ctrl Pts',(-169.223959157211,5.06500203852252,
135.640060691349));
#219724=CARTESIAN_POINT('Ctrl Pts',(-169.502406781024,6.80616874759175,
129.156844962666));
#219725=CARTESIAN_POINT('Ctrl Pts',(-169.780854404837,2.29279887745254,
124.18761563522));
#219726=CARTESIAN_POINT('Ctrl Pts',(-170.05930202865,-4.32754115161411,
125.298851700587));
#219727=CARTESIAN_POINT('Ctrl Pts',(-170.337749652463,-6.97108227448498,
131.469381501595));
#219728=CARTESIAN_POINT('Ctrl Pts',(-170.616197276276,-3.20853934340632,
137.028789598255));
#219729=CARTESIAN_POINT('Ctrl Pts',(-170.894644900089,3.50249449840198,
136.868251541923));
#219730=CARTESIAN_POINT('Ctrl Pts',(-171.173092523901,6.99490700254731,
131.135293963646));
#219731=CARTESIAN_POINT('Ctrl Pts',(-171.451540147715,4.05934169155642,
125.098224807315));
#219732=CARTESIAN_POINT('Ctrl Pts',(-171.729987771527,-2.60656032410858,
124.304815700371));
#219733=CARTESIAN_POINT('Ctrl Pts',(-172.00843539534,-6.87716073946864,
129.484170851909));
#219734=CARTESIAN_POINT('Ctrl Pts',(-172.286883019153,-4.82798640323697,
135.876715903229));
#219735=CARTESIAN_POINT('Ctrl Pts',(-172.565330642966,1.65787157732142,
137.608014245356));
#219736=CARTESIAN_POINT('Ctrl Pts',(-172.843778266779,6.62022656985093,
133.087087280501));
#219737=CARTESIAN_POINT('Ctrl Pts',(-173.122225890592,5.49891676073447,
126.468446029806));
#219738=CARTESIAN_POINT('Ctrl Pts',(-173.400673514405,-0.675628914478315,
123.834298464058));
#219739=CARTESIAN_POINT('Ctrl Pts',(-173.679121138218,-6.22930462359329,
127.605297510917));
#219740=CARTESIAN_POINT('Ctrl Pts',(-173.95756876203,-6.05855370207473,
134.316079269865));
#219741=CARTESIAN_POINT('Ctrl Pts',(-174.236016385844,-0.320287905152608,
137.799763144343));
#219742=CARTESIAN_POINT('Ctrl Pts',(-174.514464009656,5.71230682967103,
134.855013841124));
#219743=CARTESIAN_POINT('Ctrl Pts',(-174.792911633469,6.49557064972945,
128.187912110866));
#219744=CARTESIAN_POINT('Ctrl Pts',(-175.071359257282,1.30972236895365,
123.925198737649));
#219745=CARTESIAN_POINT('Ctrl Pts',(-175.349806881095,-5.07969678539539,
125.984099066334));
#219746=CARTESIAN_POINT('Ctrl Pts',(-175.628254504908,-6.80112275095037,
132.472584277733));
#219747=CARTESIAN_POINT('Ctrl Pts',(-175.906702128721,-2.27264916169912,
137.428053442694));
#219748=CARTESIAN_POINT('Ctrl Pts',(-176.185149752534,4.34427798206938,
136.296672486746));
#219749=CARTESIAN_POINT('Ctrl Pts',(-176.463597376347,6.96902589009458,
130.118125237372));
#219750=CARTESIAN_POINT('Ctrl Pts',(-176.742045000159,3.18957946096438,
124.570194777934));
#219751=CARTESIAN_POINT('Ctrl Pts',(-177.020492623972,-3.52093467317244,
124.751158169184));
#219752=CARTESIAN_POINT('Ctrl Pts',(-177.298940247785,-6.99588184988549,
130.494718895118));
#219753=CARTESIAN_POINT('Ctrl Pts',(-177.577387871598,-4.04195537438161,
136.522825237142));
#219754=CARTESIAN_POINT('Ctrl Pts',(-177.855835495411,2.62633062968132,
137.295941956302));
#219755=CARTESIAN_POINT('Ctrl Pts',(-178.134283119224,6.88114708845103,
132.103612556543));
#219756=CARTESIAN_POINT('Ctrl Pts',(-178.412730743037,4.81252553565828,
125.717334096849));
#219757=CARTESIAN_POINT('Ctrl Pts',(-178.69117836685,-1.67857187946192,
124.005784494632));
#219758=CARTESIAN_POINT('Ctrl Pts',(-178.969625990663,-6.62714374015151,
128.541794220484));
#219759=CARTESIAN_POINT('Ctrl Pts',(-179.248073614475,-5.48569425761253,
135.15699193274));
#219760=CARTESIAN_POINT('Ctrl Pts',(-179.526521238288,0.696840256609583,
137.772334104211));
#219761=CARTESIAN_POINT('Ctrl Pts',(-179.804968862101,6.23901261754625,
133.984449045885));
#219762=CARTESIAN_POINT('Ctrl Pts',(-180.083416485914,6.0478371756692,127.27421807789));
#219763=CARTESIAN_POINT('Ctrl Pts',(-180.361864109727,0.298994822622653,
123.808015646805));
#219764=CARTESIAN_POINT('Ctrl Pts',(-180.64031173354,-5.72460916570447,
126.771112453397));
#219765=CARTESIAN_POINT('Ctrl Pts',(-180.918759357353,-6.48757699345442,
133.440567287733));
#219766=CARTESIAN_POINT('Ctrl Pts',(-181.197206981166,-1.28877849997557,
137.687476978041));
#219767=CARTESIAN_POINT('Ctrl Pts',(-181.475654604978,5.094344474651,135.609138992));
#219768=CARTESIAN_POINT('Ctrl Pts',(-181.754102228792,6.79601374963652,
129.115444406326));
#219769=CARTESIAN_POINT('Ctrl Pts',(-182.032549852604,2.25247839243521,
124.173781310638));
#219770=CARTESIAN_POINT('Ctrl Pts',(-182.310997476417,-4.36097456772779,
125.32529667621));
#219771=CARTESIAN_POINT('Ctrl Pts',(-182.58944510023,-6.96690494559973,
131.511804136733));
#219772=CARTESIAN_POINT('Ctrl Pts',(-182.867892724043,-3.17059003069381,
137.048205563678));
#219773=CARTESIAN_POINT('Ctrl Pts',(-183.146340347856,3.53934223048593,
136.84681851393));
#219774=CARTESIAN_POINT('Ctrl Pts',(-183.424787971669,6.99679188832936,
131.092707847901));
#219775=CARTESIAN_POINT('Ctrl Pts',(-183.703235595482,4.02453161308464,
125.07362016374));
#219776=CARTESIAN_POINT('Ctrl Pts',(-183.981683219295,-2.64607660528548,
124.320802994409));
#219777=CARTESIAN_POINT('Ctrl Pts',(-184.260130843107,-6.88506969142675,
129.52605854136));
#219778=CARTESIAN_POINT('Ctrl Pts',(-184.53857846692,-4.79702008550057,
135.906011247817));
#219779=CARTESIAN_POINT('Ctrl Pts',(-184.817026090733,1.6992566315413,137.597796254561));
#219780=CARTESIAN_POINT('Ctrl Pts',(-185.095473714546,6.63399951749853,
133.046745788687));
#219781=CARTESIAN_POINT('Ctrl Pts',(-185.373921338359,5.47242093576752,
126.435052897159));
#219782=CARTESIAN_POINT('Ctrl Pts',(-185.652368962172,-0.718045143308166,
123.838540348135));
#219783=CARTESIAN_POINT('Ctrl Pts',(-185.930816585985,-6.24866281413942,
127.64327632748));
#219784=CARTESIAN_POINT('Ctrl Pts',(-186.209264209798,-6.03706462292539,
134.35289434186));
#219785=CARTESIAN_POINT('Ctrl Pts',(-186.487711833611,-0.277698970246197,
137.801583219124));
#219786=CARTESIAN_POINT('Ctrl Pts',(-186.766159457423,5.73685846974069,
134.820166358884));
#219787=CARTESIAN_POINT('Ctrl Pts',(-187.044607081237,6.47952323715255,
128.148420205389));
#219788=CARTESIAN_POINT('Ctrl Pts',(-187.323054705049,1.2678226919294,123.917353540782));
#219789=CARTESIAN_POINT('Ctrl Pts',(-187.601502328862,-5.10894497059535,
126.01510993074));
#219790=CARTESIAN_POINT('Ctrl Pts',(-187.879949952675,-6.79084179098006,
132.513953733987));
#219791=CARTESIAN_POINT('Ctrl Pts',(-188.158397576488,-2.23228675651833,
137.44176498151));
#219792=CARTESIAN_POINT('Ctrl Pts',(-188.436845200301,4.37763075391265,
136.270125873797));
#219793=CARTESIAN_POINT('Ctrl Pts',(-188.715292824114,6.96471946064982,
130.075715513085));
#219794=CARTESIAN_POINT('Ctrl Pts',(-188.993740447926,3.15157122851057,
124.550894407098));
#219795=CARTESIAN_POINT('Ctrl Pts',(-189.27218807174,-3.55771699981564,
124.772703249722));
#219796=CARTESIAN_POINT('Ctrl Pts',(-189.550635695553,-6.99763710944952,
130.53731055055));
#219797=CARTESIAN_POINT('Ctrl Pts',(-189.829083319365,-4.00707056907658,
136.547323816845));
#219798=CARTESIAN_POINT('Ctrl Pts',(-190.107530943179,2.66579806799723,
137.279834462351));
#219799=CARTESIAN_POINT('Ctrl Pts',(-190.385978566991,6.88892851205765,
132.061700988983));
#219800=CARTESIAN_POINT('Ctrl Pts',(-190.664426190804,4.78147019640398,
125.688133138775));
#219801=CARTESIAN_POINT('Ctrl Pts',(-190.942873814617,-1.71992564193992,
124.016128399968));
#219802=CARTESIAN_POINT('Ctrl Pts',(-191.22132143843,-6.64079383837953,
128.582177445553));
#219803=CARTESIAN_POINT('Ctrl Pts',(-191.499769062243,-5.45909691816341,
135.190304266535));
#219804=CARTESIAN_POINT('Ctrl Pts',(-191.778216686055,0.739243378134395,
137.767963139373));
#219805=CARTESIAN_POINT('Ctrl Pts',(-192.056664309869,6.25825512397307,
133.946411485565));
#219806=CARTESIAN_POINT('Ctrl Pts',(-192.335111933681,6.0262361436405,127.237468581785));
#219807=CARTESIAN_POINT('Ctrl Pts',(-192.613559557494,0.256400545303713,
123.806325206523));
#219808=CARTESIAN_POINT('Ctrl Pts',(-192.892007181307,-5.74905462830365,
126.806034500975));
#219809=CARTESIAN_POINT('Ctrl Pts',(-193.17045480512,-6.47140945543246,
133.480010167483));
#219810=CARTESIAN_POINT('Ctrl Pts',(-193.448902428933,-1.24685513894648,
137.695194610365));
#219811=CARTESIAN_POINT('Ctrl Pts',(-193.727350052746,5.12349813797151,
135.578039249819));
#219812=CARTESIAN_POINT('Ctrl Pts',(-194.005797676559,6.78560692289256,
129.074106433399));
#219813=CARTESIAN_POINT('Ctrl Pts',(-194.284245300372,2.2120744410027,124.160192684611));
#219814=CARTESIAN_POINT('Ctrl Pts',(-194.562692924184,-4.39424638632456,
125.35194468056));
#219815=CARTESIAN_POINT('Ctrl Pts',(-194.841140547997,-6.9624694554897,
131.554200557291));
#219816=CARTESIAN_POINT('Ctrl Pts',(-195.11958817181,-3.13252323060231,
137.067390161131));
#219817=CARTESIAN_POINT('Ctrl Pts',(-195.398035795623,3.57605881094196,
136.825161580438));
#219818=CARTESIAN_POINT('Ctrl Pts',(-195.676483419436,6.99841750541489,
131.050111047343));
#219819=CARTESIAN_POINT('Ctrl Pts',(-195.954931043249,3.98957240411393,
125.04922787486));
#219820=CARTESIAN_POINT('Ctrl Pts',(-196.233378667062,-2.68549483512068,
124.337030539057));
#219821=CARTESIAN_POINT('Ctrl Pts',(-196.511826290875,-6.89272351459547,
129.567993598765));
#219822=CARTESIAN_POINT('Ctrl Pts',(-196.790273914688,-4.76587601242081,
135.935117548864));
#219823=CARTESIAN_POINT('Ctrl Pts',(-197.0687215385,1.74057871918182,137.58732653051));
#219824=CARTESIAN_POINT('Ctrl Pts',(-197.347169162313,6.64752663985393,
133.006321204467));
#219825=CARTESIAN_POINT('Ctrl Pts',(-197.625616786126,5.44572232823074,
126.401821670817));
#219826=CARTESIAN_POINT('Ctrl Pts',(-197.904064409939,-0.760434764710735,
123.843040353244));
#219827=CARTESIAN_POINT('Ctrl Pts',(-198.182512033752,-6.26778945818702,
127.681372279183));
#219828=CARTESIAN_POINT('Ctrl Pts',(-198.460959657565,-6.01535183812634,
134.389577921633));
#219829=CARTESIAN_POINT('Ctrl Pts',(-198.739407281378,-0.235099745102313,
137.803144009248));
#219830=CARTESIAN_POINT('Ctrl Pts',(-199.017854905191,5.76119752841001,
134.785170069484));
#219831=CARTESIAN_POINT('Ctrl Pts',(-199.296302529004,6.46323572345932,
128.10902671676));
#219832=CARTESIAN_POINT('Ctrl Pts',(-199.574750152817,1.22587603526843,
123.909763544495));
#219833=CARTESIAN_POINT('Ctrl Pts',(-199.853197776629,-5.13800384196074,
126.04629826259));
#219834=CARTESIAN_POINT('Ctrl Pts',(-200.131645400443,-6.78030919386985,
132.555259840639));
#219835=CARTESIAN_POINT('Ctrl Pts',(-200.410093024255,-2.19184163313082,
137.455230568865));
#219836=CARTESIAN_POINT('Ctrl Pts',(-200.688540648069,4.41082131103843,
136.243376724908));
#219837=CARTESIAN_POINT('Ctrl Pts',(-200.96698827188,6.96015495096418,130.03333278901));
#219838=CARTESIAN_POINT('Ctrl Pts',(-201.245435895694,3.11344621342587,
124.531825760752));
#219839=CARTESIAN_POINT('Ctrl Pts',(-201.523883519507,-3.59436749394705,
124.794471835542));
#219840=CARTESIAN_POINT('Ctrl Pts',(-201.80233114332,-6.99913306899709,
130.579912101622));
#219841=CARTESIAN_POINT('Ctrl Pts',(-202.080778767133,-3.97203728029775,
136.571609588935));
#219842=CARTESIAN_POINT('Ctrl Pts',(-202.359226390945,2.705166724186,137.263487017335));
#219843=CARTESIAN_POINT('Ctrl Pts',(-202.637674014758,6.89645466388467,
132.019742830214));
#219844=CARTESIAN_POINT('Ctrl Pts',(-202.916121638571,4.75023767801316,
125.659121764391));
#219845=CARTESIAN_POINT('Ctrl Pts',(-203.194569262384,-1.76121567194074,
124.026723845744));
#219846=CARTESIAN_POINT('Ctrl Pts',(-203.473016886197,-6.65419785954973,
128.622643014438));
#219847=CARTESIAN_POINT('Ctrl Pts',(-203.75146451001,-5.43229728987039,
135.223454077576));
#219848=CARTESIAN_POINT('Ctrl Pts',(-204.029912133822,0.781619106723946,
137.763334135682));
#219849=CARTESIAN_POINT('Ctrl Pts',(-204.308359757636,6.27726572845484,
133.908257495395));
#219850=CARTESIAN_POINT('Ctrl Pts',(-204.586807381448,6.00441180721532,
127.200851258176));
#219851=CARTESIAN_POINT('Ctrl Pts',(-204.865255005262,0.213796766968775,
123.804894081017));
#219852=CARTESIAN_POINT('Ctrl Pts',(-205.143702629074,-5.77328705756903,
126.841104707996));
#219853=CARTESIAN_POINT('Ctrl Pts',(-205.422150252887,-6.4550021169537,
133.519353900054));
#219854=CARTESIAN_POINT('Ctrl Pts',(-205.7005978767,-1.20488557524167,137.702656900301));
#219855=CARTESIAN_POINT('Ctrl Pts',(-205.979045500513,5.15246194818434,
135.546762617222));
#219856=CARTESIAN_POINT('Ctrl Pts',(-206.257493124326,6.77494865298866,
129.032832575676));
#219857=CARTESIAN_POINT('Ctrl Pts',(-206.535940748139,2.17158852033829,
124.14685026067));
#219858=CARTESIAN_POINT('Ctrl Pts',(-206.814388371952,-4.42735537450605,
125.378794726189));
#219859=CARTESIAN_POINT('Ctrl Pts',(-207.092835995765,-6.9577759685135,
131.596569192254));
#219860=CARTESIAN_POINT('Ctrl Pts',(-207.371283619578,-3.09434035370993,
137.086342679721));
#219861=CARTESIAN_POINT('Ctrl Pts',(-207.64973124339,3.61264287922363,136.803281543952));
#219862=CARTESIAN_POINT('Ctrl Pts',(-207.928178867203,6.99978379356611,
131.007505140413));
#219863=CARTESIAN_POINT('Ctrl Pts',(-208.206626491016,3.95446536007061,
125.025048844539));
#219864=CARTESIAN_POINT('Ctrl Pts',(-208.485074114829,-2.72481355295718,
124.353497733001));
#219865=CARTESIAN_POINT('Ctrl Pts',(-208.763521738642,-6.90012192535954,
129.609974470206));
#219866=CARTESIAN_POINT('Ctrl Pts',(-209.041969362455,-4.73455533805275,
135.964033727826));
#219867=CARTESIAN_POINT('Ctrl Pts',(-209.320416986268,1.78183630903778,
137.576605461163));
#219868=CARTESIAN_POINT('Ctrl Pts',(-209.598864610081,6.66080743566547,
132.965815025787));
#219869=CARTESIAN_POINT('Ctrl Pts',(-209.877312233893,5.41882192745001,
126.368753582173));
#219870=CARTESIAN_POINT('Ctrl Pts',(-210.155759857706,-0.802796207923886,
123.847798312635));
#219871=CARTESIAN_POINT('Ctrl Pts',(-210.434207481519,-6.28668384699127,
127.719583954367));
#219872=CARTESIAN_POINT('Ctrl Pts',(-210.712655105332,-5.99341615225276,
134.42612864986));
#219873=CARTESIAN_POINT('Ctrl Pts',(-210.991102729145,-0.19249180825093,
137.804445456879));
#219874=CARTESIAN_POINT('Ctrl Pts',(-211.269550352958,5.78532310378624,
134.750026269725));
#219875=CARTESIAN_POINT('Ctrl Pts',(-211.547997976771,6.44670871218949,
128.069733104719));
#219876=CARTESIAN_POINT('Ctrl Pts',(-211.826445600584,1.18388395332015,
123.902429030038));
#219877=CARTESIAN_POINT('Ctrl Pts',(-212.104893224396,-5.16687232270428,
126.077662906191));
#219878=CARTESIAN_POINT('Ctrl Pts',(-212.38334084821,-6.76952534990887,
132.596501067076));
#219879=CARTESIAN_POINT('Ctrl Pts',(-212.661788472022,-2.15131529024619,
137.468449705789));
#219880=CARTESIAN_POINT('Ctrl Pts',(-212.940236095835,4.44384842355829,
136.216426031276));
#219881=CARTESIAN_POINT('Ctrl Pts',(-213.218683719648,6.95533253017721,
129.990978635656));
#219882=CARTESIAN_POINT('Ctrl Pts',(-213.497131343461,3.0752058284468,124.512989545492));
#219883=CARTESIAN_POINT('Ctrl Pts',(-213.775578967274,-3.63088479746918,
124.81646312));
#219884=CARTESIAN_POINT('Ctrl Pts',(-214.054026591087,-7.00036967309483,
130.622521969716));
#219885=CARTESIAN_POINT('Ctrl Pts',(-214.3324742149,-3.93685680621679,136.595681653493));
#219886=CARTESIAN_POINT('Ctrl Pts',(-214.610921838713,2.74443513942699,
137.246900227015));
#219887=CARTESIAN_POINT('Ctrl Pts',(-214.889369462525,6.90372526504794,
131.977739635008));
#219888=CARTESIAN_POINT('Ctrl Pts',(-215.167817086339,4.71882913781829,
125.630301048724));
#219889=CARTESIAN_POINT('Ctrl Pts',(-215.446264710151,-1.80244043944716,
124.037570439344));
#219890=CARTESIAN_POINT('Ctrl Pts',(-215.724712333964,-6.66735530697114,
128.66318942767));
#219891=CARTESIAN_POINT('Ctrl Pts',(-216.003159957777,-5.40529636580357,
135.256440137483));
#219892=CARTESIAN_POINT('Ctrl Pts',(-216.28160758159,0.823965872130078,
137.758447264668));
#219893=CARTESIAN_POINT('Ctrl Pts',(-216.560055205403,6.29604372654653,
133.869988489185));
#219894=CARTESIAN_POINT('Ctrl Pts',(-216.838502829216,5.98236497510254,
127.164367463932));
#219895=CARTESIAN_POINT('Ctrl Pts',(-217.116950453029,0.171185066315507,
123.803722323317));
#219896=CARTESIAN_POINT('Ctrl Pts',(-217.395398076842,-5.79730555555969,
126.876321774922));
#219897=CARTESIAN_POINT('Ctrl Pts',(-217.673845700654,-6.43835558599724,
133.558597027552));
#219898=CARTESIAN_POINT('Ctrl Pts',(-217.952293324468,-1.16287136405879,
137.709863571333));
#219899=CARTESIAN_POINT('Ctrl Pts',(-218.23074094828,5.18123483202488,135.515310253174));
#219900=CARTESIAN_POINT('Ctrl Pts',(-218.509188572093,6.76403933487094,
128.991624362576));
#219901=CARTESIAN_POINT('Ctrl Pts',(-218.787636195906,2.13102213066266,
124.133754533223));
#219902=CARTESIAN_POINT('Ctrl Pts',(-219.066083819719,-4.46030030540597,
125.405845818157));
#219903=CARTESIAN_POINT('Ctrl Pts',(-219.344531443532,-6.95282465859006,
131.638908471637));
#219904=CARTESIAN_POINT('Ctrl Pts',(-219.622979067345,-3.0560428148978,
137.105062417155));
#219905=CARTESIAN_POINT('Ctrl Pts',(-219.901426691158,3.6490930796943,136.781179215245));
#219906=CARTESIAN_POINT('Ctrl Pts',(-220.179874314971,7.00089070215466,
130.964891705888));
#219907=CARTESIAN_POINT('Ctrl Pts',(-220.458321938783,3.91921178185968,
125.001083968743));
#219908=CARTESIAN_POINT('Ctrl Pts',(-220.736769562596,-2.76403130182543,
124.370203966041));
#219909=CARTESIAN_POINT('Ctrl Pts',(-221.015217186409,-6.90726464956813,
129.651999600063));
#219910=CARTESIAN_POINT('Ctrl Pts',(-221.293664810222,-4.7030592229955,
135.992758713204));
#219911=CARTESIAN_POINT('Ctrl Pts',(-221.572112434035,1.82302787229404,
137.565633443793));
#219912=CARTESIAN_POINT('Ctrl Pts',(-221.850560057848,6.67384141280798,
132.925228753618));
#219913=CARTESIAN_POINT('Ctrl Pts',(-222.129007681661,5.39172073022998,
126.33584985658));
#219914=CARTESIAN_POINT('Ctrl Pts',(-222.407455305474,-0.845127903228338,
123.85281405));
#219915=CARTESIAN_POINT('Ctrl Pts',(-222.685902929286,-6.30534528041361,
127.757909937084));
#219916=CARTESIAN_POINT('Ctrl Pts',(-222.964350553099,-5.9712583781396,
134.462545172141));
#219917=CARTESIAN_POINT('Ctrl Pts',(-223.242798176912,-0.14987673854478,
137.805487513793));
#219918=CARTESIAN_POINT('Ctrl Pts',(-223.521245800725,5.80923430188729,
134.714736261875));
#219919=CARTESIAN_POINT('Ctrl Pts',(-223.799693424538,6.42994281575757,
128.030540825308));
#219920=CARTESIAN_POINT('Ctrl Pts',(-224.078141048351,1.1418480021166,123.895350269195));
#219921=CARTESIAN_POINT('Ctrl Pts',(-224.356588672164,-5.19554934309376,
126.109202699315));
#219922=CARTESIAN_POINT('Ctrl Pts',(-224.635036295977,-6.75849065869668,
132.637675885092));
#219923=CARTESIAN_POINT('Ctrl Pts',(-224.913483919789,-2.11070922958169,
137.481421902441));
#219924=CARTESIAN_POINT('Ctrl Pts',(-225.191931543603,4.47671086764076,
136.189274791569));
#219925=CARTESIAN_POINT('Ctrl Pts',(-225.470379167415,6.95025237698553,
129.948654622468));
#219926=CARTESIAN_POINT('Ctrl Pts',(-225.748826791228,3.03685149058481,
124.494386459301));
#219927=CARTESIAN_POINT('Ctrl Pts',(-226.027274415041,-3.66726755721984,
124.838676288203));
#219928=CARTESIAN_POINT('Ctrl Pts',(-226.305722038854,-7.00134687591997,
130.665138575908));
#219929=CARTESIAN_POINT('Ctrl Pts',(-226.584169662667,-3.9015304504591,
136.619539118521));
#219930=CARTESIAN_POINT('Ctrl Pts',(-226.86261728648,2.78360185861461,137.230074706019));
#219931=CARTESIAN_POINT('Ctrl Pts',(-227.141064910293,6.91074004613266,
131.935692959814));
#219932=CARTESIAN_POINT('Ctrl Pts',(-227.419512534106,4.68724573967455,
125.601672059739));
#219933=CARTESIAN_POINT('Ctrl Pts',(-227.697960157918,-1.8435984168596,
124.048667778841));
#219934=CARTESIAN_POINT('Ctrl Pts',(-227.976407781732,-6.68026569308986,
128.703815182788));
#219935=CARTESIAN_POINT('Ctrl Pts',(-228.254855405544,-5.37809514649209,
135.289261223946));
#219936=CARTESIAN_POINT('Ctrl Pts',(-228.533303029357,0.86628210517778,
137.753302707416));
#219937=CARTESIAN_POINT('Ctrl Pts',(-228.81175065317,6.31458842242258,133.831605885006));
#219938=CARTESIAN_POINT('Ctrl Pts',(-229.090198276983,5.96009646425557,
127.128018550972));
#219939=CARTESIAN_POINT('Ctrl Pts',(-229.368645900796,0.128567022336676,
123.802809976843));
#219940=CARTESIAN_POINT('Ctrl Pts',(-229.647093524609,-5.82110923226107,
126.911684396774));
#219941=CARTESIAN_POINT('Ctrl Pts',(-229.925541148421,-6.42147047940683,
133.597738095807));
#219942=CARTESIAN_POINT('Ctrl Pts',(-230.203988772235,-1.12081406224988,
137.716814356412));
#219943=CARTESIAN_POINT('Ctrl Pts',(-230.482436396047,5.20981572330331,
135.483683323156));
#219944=CARTESIAN_POINT('Ctrl Pts',(-230.76088401986,6.75287937278817,128.950483321085));
#219945=CARTESIAN_POINT('Ctrl Pts',(-231.039331643673,2.0903767751783,124.120905987538));
#219946=CARTESIAN_POINT('Ctrl Pts',(-231.317779267486,-4.49307995823781,
125.433096954076));
#219947=CARTESIAN_POINT('Ctrl Pts',(-231.596226891299,-6.94761570919197,
131.681216826544));
#219948=CARTESIAN_POINT('Ctrl Pts',(-231.874674515112,-3.01763203329532,
137.123548679767));
#219949=CARTESIAN_POINT('Ctrl Pts',(-232.153122138925,3.68540806167951,
136.758855413326));
#219950=CARTESIAN_POINT('Ctrl Pts',(-232.431569762738,7.00173819016367,
130.922272322824));
#219951=CARTESIAN_POINT('Ctrl Pts',(-232.71001738655,3.88381297581431,124.977334135496));
#219952=CARTESIAN_POINT('Ctrl Pts',(-232.988465010364,-2.80314662849731,
124.38714861912));
#219953=CARTESIAN_POINT('Ctrl Pts',(-233.266912634176,-6.914151422545,129.694067431082));
#219954=CARTESIAN_POINT('Ctrl Pts',(-233.545360257989,-4.67138883434919,
136.021291440583));
#219955=CARTESIAN_POINT('Ctrl Pts',(-233.823807881803,1.86415188258208,
137.554410884971));
#219956=CARTESIAN_POINT('Ctrl Pts',(-234.102255505615,6.68662808830262,
132.884563891901));
#219957=CARTESIAN_POINT('Ctrl Pts',(-234.380703129428,5.36441974081549,
126.303111713297));
#219958=CARTESIAN_POINT('Ctrl Pts',(-234.659150753241,-0.887428282007554,
123.858087379481));
#219959=CARTESIAN_POINT('Ctrl Pts',(-234.937598377053,-6.32377306694735,
127.796348807152));
#219960=CARTESIAN_POINT('Ctrl Pts',(-235.216046000867,-5.94887933685163,
134.498826139047));
#219961=CARTESIAN_POINT('Ctrl Pts',(-235.494493624679,-0.107256115101469,
137.806270141374));
#219962=CARTESIAN_POINT('Ctrl Pts',(-235.772941248493,5.83293023667497,
134.679301353618));
#219963=CARTESIAN_POINT('Ctrl Pts',(-236.051388872305,6.41293865542997,
127.991451330808));
#219964=CARTESIAN_POINT('Ctrl Pts',(-236.329836496118,1.09976973931543,
123.88852752427));
#219965=CARTESIAN_POINT('Ctrl Pts',(-236.608284119931,-5.22403384049169,
126.140916473241));
#219966=CARTESIAN_POINT('Ctrl Pts',(-236.886731743744,-6.7472055291277,
132.678782768935));
#219967=CARTESIAN_POINT('Ctrl Pts',(-237.165179367557,-2.07002495581049,
137.494146678133));
#219968=CARTESIAN_POINT('Ctrl Pts',(-237.44362699137,4.50940742555574,136.161924011888));
#219969=CARTESIAN_POINT('Ctrl Pts',(-237.722074615182,6.94491467963605,
129.906362317783));
#219970=CARTESIAN_POINT('Ctrl Pts',(-238.000522238996,2.99838462107406,
124.476017191522));
#219971=CARTESIAN_POINT('Ctrl Pts',(-238.278969862808,-3.70351442502255,
124.861110517033));
#219972=CARTESIAN_POINT('Ctrl Pts',(-238.557417486622,-7.00206464126185,
130.707760341024));
#219973=CARTESIAN_POINT('Ctrl Pts',(-238.835865110434,-3.86605952205578,
136.64318109997));
#219974=CARTESIAN_POINT('Ctrl Pts',(-239.114312734247,2.82266543041169,
137.213011077826));
#219975=CARTESIAN_POINT('Ctrl Pts',(-239.39276035806,6.91749874720356,131.893604362681));
#219976=CARTESIAN_POINT('Ctrl Pts',(-239.671207981873,4.655488653916,125.573235858291));
#219977=CARTESIAN_POINT('Ctrl Pts',(-239.949655605686,-1.88468807905538,
124.060015453022));
#219978=CARTESIAN_POINT('Ctrl Pts',(-240.228103229498,-6.69292853950653,
128.74451877439));
#219979=CARTESIAN_POINT('Ctrl Pts',(-240.506550853312,-5.35069463988719,
135.321916120768));
#219980=CARTESIAN_POINT('Ctrl Pts',(-240.784998477124,0.908566237823527,
137.747900654559));
#219981=CARTESIAN_POINT('Ctrl Pts',(-241.063446100938,6.33289912890243,
133.79311110514));
#219982=CARTESIAN_POINT('Ctrl Pts',(-241.34189372475,5.9376070998423,127.091805866219));
#219983=CARTESIAN_POINT('Ctrl Pts',(-241.620341348563,0.0859442142595387,
123.802157075403));
#219984=CARTESIAN_POINT('Ctrl Pts',(-241.898788972376,-5.84469720561911,
126.947191263173));
#219985=CARTESIAN_POINT('Ctrl Pts',(-242.177236596189,-6.40434742286629,
133.636775654432));
#219986=CARTESIAN_POINT('Ctrl Pts',(-242.455684220002,-1.07871522826414,
137.723508997977));
#219987=CARTESIAN_POINT('Ctrl Pts',(-242.734131843815,5.23820356294377,
135.451882999115));
#219988=CARTESIAN_POINT('Ctrl Pts',(-243.012579467628,6.74146918027728,
128.909410975699));
#219989=CARTESIAN_POINT('Ctrl Pts',(-243.29102709144,2.04965396001378,124.108305099723));
#219990=CARTESIAN_POINT('Ctrl Pts',(-243.569474715254,-4.52569311833944,
125.460547124147));
#219991=CARTESIAN_POINT('Ctrl Pts',(-243.847922339066,-6.94214931333881,
131.72349268922));
#219992=CARTESIAN_POINT('Ctrl Pts',(-244.12636996288,-2.9791094322281,137.141800782542));
#219993=CARTESIAN_POINT('Ctrl Pts',(-244.404817586691,3.72158647951367,
136.736310965414));
#219994=CARTESIAN_POINT('Ctrl Pts',(-244.683265210505,7.00232622618917,
130.879648570499));
#219995=CARTESIAN_POINT('Ctrl Pts',(-244.961712834317,3.84827025365086,
124.953800224859));
#219996=CARTESIAN_POINT('Ctrl Pts',(-245.240160458131,-2.84215808354001,
124.404331064352));
#219997=CARTESIAN_POINT('Ctrl Pts',(-245.518608081943,-6.92078198909823,
129.736176404423));
#219998=CARTESIAN_POINT('Ctrl Pts',(-245.797055705757,-4.63954534567172,
136.049630852671));
#219999=CARTESIAN_POINT('Ctrl Pts',(-246.075503329569,1.90520681603656,
137.542938200555));
#220000=CARTESIAN_POINT('Ctrl Pts',(-246.353950953382,6.69916698833444,
132.843821947487));
#220001=CARTESIAN_POINT('Ctrl Pts',(-246.632398577195,5.33691997085474,
126.270540365447));
#220002=CARTESIAN_POINT('Ctrl Pts',(-246.910846201008,-0.929695776805409,
123.86361810567));
#220003=CARTESIAN_POINT('Ctrl Pts',(-247.189293824821,-6.34196652374499,
127.834899140205));
#220004=CARTESIAN_POINT('Ctrl Pts',(-247.467741448634,-5.9262798576518,
134.534970206175));
#220005=CARTESIAN_POINT('Ctrl Pts',(-247.746189072447,-0.0646315172428821,
137.806793310625));
#220006=CARTESIAN_POINT('Ctrl Pts',(-248.024636696259,5.85641003008765,
134.643722858007));
#220007=CARTESIAN_POINT('Ctrl Pts',(-248.303084320073,6.39569686130214,
127.952466069697));
#220008=CARTESIAN_POINT('Ctrl Pts',(-248.581531943885,1.05765072414216,
123.881961048084));
#220009=CARTESIAN_POINT('Ctrl Pts',(-248.859979567699,-5.25232475939459,
126.172803052805));
#220010=CARTESIAN_POINT('Ctrl Pts',(-249.138427191511,-6.73567037937639,
132.719820195375));
#220011=CARTESIAN_POINT('Ctrl Pts',(-249.416874815324,-2.02926397650361,
137.506623561341));
#220012=CARTESIAN_POINT('Ctrl Pts',(-249.695322439137,4.54193688572079,
136.134374705723));
#220013=CARTESIAN_POINT('Ctrl Pts',(-249.97377006295,6.93931963591783,129.864103288757));
#220014=CARTESIAN_POINT('Ctrl Pts',(-250.252217686763,2.95980664532115,
124.457882422832));
#220015=CARTESIAN_POINT('Ctrl Pts',(-250.530665310576,-3.73962405773988,
124.883764975191));
#220016=CARTESIAN_POINT('Ctrl Pts',(-250.809112934388,-7.00252294251614,
130.750385685678));
#220017=CARTESIAN_POINT('Ctrl Pts',(-251.087560558202,-3.83044533540895,
136.666606721818));
#220018=CARTESIAN_POINT('Ctrl Pts',(-251.366008182014,2.86162440732935,
137.195709974661));
#220019=CARTESIAN_POINT('Ctrl Pts',(-251.644455805827,6.9240011177651,131.851475403357));
#220020=CARTESIAN_POINT('Ctrl Pts',(-251.92290342964,4.62355905740654,125.54499349784));
#220021=CARTESIAN_POINT('Ctrl Pts',(-252.201351053453,-1.92570790361727,
124.071613041873));
#220022=CARTESIAN_POINT('Ctrl Pts',(-252.479798677266,-6.70534337666252,
128.785298693283));
#220023=CARTESIAN_POINT('Ctrl Pts',(-252.758246301079,-5.3230958619522,
135.354403619622));
#220024=CARTESIAN_POINT('Ctrl Pts',(-253.036693924892,0.950816704398073,
137.74224130304));
#220025=CARTESIAN_POINT('Ctrl Pts',(-253.315141548704,6.35097516523885,
133.754505582129));
#220026=CARTESIAN_POINT('Ctrl Pts',(-253.593589172518,5.91489771943887,
127.055730740027));
#220027=CARTESIAN_POINT('Ctrl Pts',(-253.87203679633,0.0433182135112656,
123.801763664947));
#220028=CARTESIAN_POINT('Ctrl Pts',(-254.150484420143,-5.86806858651122,
126.982841017323));
#220029=CARTESIAN_POINT('Ctrl Pts',(-254.428932043956,-6.38698707931617,
133.675708334441));
#220030=CARTESIAN_POINT('Ctrl Pts',(-254.707379667769,-1.03657636838919,
137.729947101491));
#220031=CARTESIAN_POINT('Ctrl Pts',(-254.985827291582,5.26639719763008,
135.41991073597));
#220032=CARTESIAN_POINT('Ctrl Pts',(-255.264274915395,6.72980937160111,
128.868408326187));
#220033=CARTESIAN_POINT('Ctrl Pts',(-255.542722539208,2.00885483266244,
124.095953322692));
#220034=CARTESIAN_POINT('Ctrl Pts',(-255.821170163021,-4.5581378946222,
125.488193449449));
#220035=CARTESIAN_POINT('Ctrl Pts',(-256.099617786833,-6.93642696247006,
131.765738008466));
#220036=CARTESIAN_POINT('Ctrl Pts',(-256.378065410647,-2.94047400549736,
137.159811411449));
#220037=CARTESIAN_POINT('Ctrl Pts',(-256.656513034459,3.7576223973322,136.713559240208));
#220038=CARTESIAN_POINT('Ctrl Pts',(-256.934960658272,7.0026634652268,130.836998362911));
#220039=CARTESIAN_POINT('Ctrl Pts',(-257.213408282085,3.81256854888166,
124.930527794066));
#220040=CARTESIAN_POINT('Ctrl Pts',(-257.491855905898,-2.88103328591622,
124.421666290213));
#220041=CARTESIAN_POINT('Ctrl Pts',(-257.770303529711,-6.92721451599304,
129.778484277494));
#220042=CARTESIAN_POINT('Ctrl Pts',(-258.048751153524,-4.60741964202412,
136.077475067175));
#220043=CARTESIAN_POINT('Ctrl Pts',(-258.327198777336,1.94598288966397,
137.53178391186));
#220044=CARTESIAN_POINT('Ctrl Pts',(-258.60564640115,6.71185090883407,132.801931226644));
#220045=CARTESIAN_POINT('Ctrl Pts',(-258.884094024962,5.30847971878909,
126.240167716581));
#220046=CARTESIAN_POINT('Ctrl Pts',(-259.162541648776,-0.970525071554103,
123.86553674091));
#220047=CARTESIAN_POINT('Ctrl Pts',(-259.440989272588,-6.36258613651914,
127.881151058581));
#220048=CARTESIAN_POINT('Ctrl Pts',(-259.673028959099,-5.97575359986218,
133.442106215535));
#220049=CARTESIAN_POINT('Ctrl Pts',(-259.858689921174,-2.9628379271774,
136.206922793942));
#220050=CARTESIAN_POINT('Ctrl Pts',(-259.951535008647,-1.00384119663989,
136.721969923993));
#220051=CARTESIAN_POINT('Ctrl Pts',(-259.997972158816,-0.016740685831905,
136.724751058381));
#220052=CARTESIAN_POINT('Ctrl Pts',(210.384788400103,3.2437100417032,135.350446923363));
#220053=CARTESIAN_POINT('Ctrl Pts',(210.338370536501,4.00135710969089,134.809856772425));
#220054=CARTESIAN_POINT('Ctrl Pts',(210.245544735596,5.2274450014198,133.344996311945));
#220055=CARTESIAN_POINT('Ctrl Pts',(210.059903060087,6.03752477204218,129.574087134129));
#220056=CARTESIAN_POINT('Ctrl Pts',(209.827863373576,3.30140998082846,125.08375145776));
#220057=CARTESIAN_POINT('Ctrl Pts',(209.549415749763,-3.03864792542705,
124.935284604053));
#220058=CARTESIAN_POINT('Ctrl Pts',(209.27096812595,-6.57501826603042,130.18815040753));
#220059=CARTESIAN_POINT('Ctrl Pts',(208.992520502138,-4.0751627655632,136.003208990552));
#220060=CARTESIAN_POINT('Ctrl Pts',(208.714072878324,2.17267791003586,137.042921783734));
#220061=CARTESIAN_POINT('Ctrl Pts',(208.435625254512,6.42228832295553,132.348569225854));
#220062=CARTESIAN_POINT('Ctrl Pts',(208.157177630698,4.77100074356668,126.235763887068));
#220063=CARTESIAN_POINT('Ctrl Pts',(207.878730006886,-1.26506482749479,
124.320958291314));
#220064=CARTESIAN_POINT('Ctrl Pts',(207.600282383073,-6.13835327551471,
128.364250828182));
#220065=CARTESIAN_POINT('Ctrl Pts',(207.32183475926,-5.37092434612766,134.649796015418));
#220066=CARTESIAN_POINT('Ctrl Pts',(207.043387135447,0.332190207827403,
137.40162108792));
#220067=CARTESIAN_POINT('Ctrl Pts',(206.764939511634,5.73000189292936,134.090861108297));
#220068=CARTESIAN_POINT('Ctrl Pts',(206.486491887821,5.86224098722307,127.759980958474));
#220069=CARTESIAN_POINT('Ctrl Pts',(206.208044264008,0.607356820266201,
124.226729984437));
#220070=CARTESIAN_POINT('Ctrl Pts',(205.929596640195,-5.20565320191231,
126.738003936844));
#220071=CARTESIAN_POINT('Ctrl Pts',(205.651149016382,-6.23492509722864,
132.986059061584));
#220072=CARTESIAN_POINT('Ctrl Pts',(205.37270139257,-1.53460390898592,137.229240938669));
#220073=CARTESIAN_POINT('Ctrl Pts',(205.094253768756,4.57594250116295,135.568271122458));
#220074=CARTESIAN_POINT('Ctrl Pts',(204.815806144944,6.48142172411287,129.529500574057));
#220075=CARTESIAN_POINT('Ctrl Pts',(204.537358521131,2.43079079302514,124.662263970705));
#220076=CARTESIAN_POINT('Ctrl Pts',(204.258910897318,-3.85361800715474,
125.439314209572));
#220077=CARTESIAN_POINT('Ctrl Pts',(203.980463273505,-6.5967401814699,131.146579956944));
#220078=CARTESIAN_POINT('Ctrl Pts',(203.702015649692,-3.27778036432047,
136.539362872731));
#220079=CARTESIAN_POINT('Ctrl Pts',(203.42356802588,3.05329946149495,136.661958874297));
#220080=CARTESIAN_POINT('Ctrl Pts',(203.145120402066,6.5785462535266,131.40170824395));
#220081=CARTESIAN_POINT('Ctrl Pts',(202.866672778254,4.05843041346184,125.592524323598));
#220082=CARTESIAN_POINT('Ctrl Pts',(202.58822515444,-2.19118470860141,124.572763346851));
#220083=CARTESIAN_POINT('Ctrl Pts',(202.309777530628,-6.42720813017419,
129.279535830482));
#220084=CARTESIAN_POINT('Ctrl Pts',(202.031329906815,-4.75694126595338,
135.387547802118));
#220085=CARTESIAN_POINT('Ctrl Pts',(201.752882283002,1.28472223178851,137.283834652022));
#220086=CARTESIAN_POINT('Ctrl Pts',(201.474434659189,6.14578876089344,133.225801404307));
#220087=CARTESIAN_POINT('Ctrl Pts',(201.195987035376,5.35917565710019,126.94258236746));
#220088=CARTESIAN_POINT('Ctrl Pts',(200.917539411563,-0.352258065224466,
124.208148884143));
#220089=CARTESIAN_POINT('Ctrl Pts',(200.63909178775,-5.73998383440169,127.535311740963));
#220090=CARTESIAN_POINT('Ctrl Pts',(200.360644163938,-5.85294487354697,
133.866570813476));
#220091=CARTESIAN_POINT('Ctrl Pts',(200.082196540124,-0.587335506164227,
137.383808313225));
#220092=CARTESIAN_POINT('Ctrl Pts',(199.803748916312,5.2180064984534,134.854854804556));
#220093=CARTESIAN_POINT('Ctrl Pts',(199.525301292498,6.22825544477889,128.603695015683));
#220094=CARTESIAN_POINT('Ctrl Pts',(199.246853668687,1.51504190454761,124.374839406449));
#220095=CARTESIAN_POINT('Ctrl Pts',(198.968406044873,-4.5904211320519,126.054399690658));
#220096=CARTESIAN_POINT('Ctrl Pts',(198.689958421061,-6.47751140283473,
132.098942018204));
#220097=CARTESIAN_POINT('Ctrl Pts',(198.411510797247,-2.41208513843682,
136.95382728238));
#220098=CARTESIAN_POINT('Ctrl Pts',(198.133063173434,3.86992953127461,136.15765309974));
#220099=CARTESIAN_POINT('Ctrl Pts',(197.854615549622,6.59566801831256,130.442064648858));
#220100=CARTESIAN_POINT('Ctrl Pts',(197.576167925809,3.26030981281707,125.059408494076));
#220101=CARTESIAN_POINT('Ctrl Pts',(197.297720301996,-3.07111383566833,
124.956082684267));
#220102=CARTESIAN_POINT('Ctrl Pts',(197.019272678183,-6.58033390142619,
130.227038590899));
#220103=CARTESIAN_POINT('Ctrl Pts',(196.74082505437,-4.04254857895594,136.028525236289));
#220104=CARTESIAN_POINT('Ctrl Pts',(196.462377430557,2.21014139809766,137.029259811701));
#220105=CARTESIAN_POINT('Ctrl Pts',(196.183929806745,6.43181940170927,132.309616130935));
#220106=CARTESIAN_POINT('Ctrl Pts',(195.905482182931,4.74296958699597,126.206716169203));
#220107=CARTESIAN_POINT('Ctrl Pts',(195.627034559119,-1.30443757122094,
124.328826848098));
#220108=CARTESIAN_POINT('Ctrl Pts',(195.348586935305,-6.15313032680387,
128.401636713722));
#220109=CARTESIAN_POINT('Ctrl Pts',(195.070139311493,-5.34739690918169,
134.682432467391));
#220110=CARTESIAN_POINT('Ctrl Pts',(194.791691687679,0.372333033116476,
137.399469645412));
#220111=CARTESIAN_POINT('Ctrl Pts',(194.513244063867,5.74990710746052,134.055923815831));
#220112=CARTESIAN_POINT('Ctrl Pts',(194.234796440054,5.84359744862664,127.724350254736));
#220113=CARTESIAN_POINT('Ctrl Pts',(193.956348816241,0.567307210110782,
124.223155750211));
#220114=CARTESIAN_POINT('Ctrl Pts',(193.677901192428,-5.23031063999889,
126.769767009054));
#220115=CARTESIAN_POINT('Ctrl Pts',(193.399453568615,-6.22152852682933,
133.023972693263));
#220116=CARTESIAN_POINT('Ctrl Pts',(193.121005944802,-1.49546563606909,
137.238463313985));
#220117=CARTESIAN_POINT('Ctrl Pts',(192.84255832099,4.60485711668079,135.540327880088));
#220118=CARTESIAN_POINT('Ctrl Pts',(192.564110697177,6.47354113897745,129.490069896797));
#220119=CARTESIAN_POINT('Ctrl Pts',(192.285663073364,2.39335710461987,124.64758087922));
#220120=CARTESIAN_POINT('Ctrl Pts',(192.007215449551,-3.88620518688872,
125.462871665772));
#220121=CARTESIAN_POINT('Ctrl Pts',(191.728767825738,-6.59453476332446,
131.18672985278));
#220122=CARTESIAN_POINT('Ctrl Pts',(191.450320201925,-3.24280905319821,
136.559209392401));
#220123=CARTESIAN_POINT('Ctrl Pts',(191.171872578112,3.08889975678785,136.643264047941));
#220124=CARTESIAN_POINT('Ctrl Pts',(190.893424954299,6.58206059142805,131.361651697256));
#220125=CARTESIAN_POINT('Ctrl Pts',(190.614977330486,4.02662929408197,125.567916069518));
#220126=CARTESIAN_POINT('Ctrl Pts',(190.336529706674,-2.22907761274862,
124.586217166899));
#220127=CARTESIAN_POINT('Ctrl Pts',(190.05808208286,-6.43637108995848,129.318688322246));
#220128=CARTESIAN_POINT('Ctrl Pts',(189.779634459048,-4.72895396970476,
135.416419737866));
#220129=CARTESIAN_POINT('Ctrl Pts',(189.501186835235,1.32414082646293,137.275894133543));
#220130=CARTESIAN_POINT('Ctrl Pts',(189.222739211422,6.16041489098677,133.188345380025));
#220131=CARTESIAN_POINT('Ctrl Pts',(188.944291587609,5.33556862369218,126.910031093937));
#220132=CARTESIAN_POINT('Ctrl Pts',(188.665843963796,-0.392404551757433,
124.210415391489));
#220133=CARTESIAN_POINT('Ctrl Pts',(188.387396339983,-5.75977711417006,
127.570313219673));
#220134=CARTESIAN_POINT('Ctrl Pts',(188.10894871617,-5.83419588941534,133.902142614521));
#220135=CARTESIAN_POINT('Ctrl Pts',(187.830501092358,-0.547273658602122,
137.387261689231));
#220136=CARTESIAN_POINT('Ctrl Pts',(187.552053468544,5.24256632866185,134.823016271676));
#220137=CARTESIAN_POINT('Ctrl Pts',(187.273605844732,6.214743973489,128.565822630237));
#220138=CARTESIAN_POINT('Ctrl Pts',(186.995158220918,1.47587551380139,124.365736040492));
#220139=CARTESIAN_POINT('Ctrl Pts',(186.716710597106,-4.61925044254253,
126.082430892781));
#220140=CARTESIAN_POINT('Ctrl Pts',(186.438262973293,-6.46951090511933,
132.138348483055));
#220141=CARTESIAN_POINT('Ctrl Pts',(186.15981534948,-2.37460689906969,136.968396393875));
#220142=CARTESIAN_POINT('Ctrl Pts',(185.881367725667,3.90244484122886,136.133996556155));
#220143=CARTESIAN_POINT('Ctrl Pts',(185.602920101854,6.59334041746713,130.401921658061));
#220144=CARTESIAN_POINT('Ctrl Pts',(185.324472478041,3.22527825263932,125.039668503516));
#220145=CARTESIAN_POINT('Ctrl Pts',(185.046024854228,-3.10665706276191,
124.974885780916));
#220146=CARTESIAN_POINT('Ctrl Pts',(184.767577230416,-6.5837263061198,130.26710564752));
#220147=CARTESIAN_POINT('Ctrl Pts',(184.489129606603,-4.01067270706429,
136.05303658523));
#220148=CARTESIAN_POINT('Ctrl Pts',(184.21068198279,2.247993177529,137.015690720733));
#220149=CARTESIAN_POINT('Ctrl Pts',(183.932234358977,6.44086315254518,132.270435931769));
#220150=CARTESIAN_POINT('Ctrl Pts',(183.653786735164,4.71489454403,126.177929550814));
#220151=CARTESIAN_POINT('Ctrl Pts',(183.375339111351,-1.34383181504516,
124.33688730648));
#220152=CARTESIAN_POINT('Ctrl Pts',(183.096891487538,-6.16764238592767,
128.439137081397));
#220153=CARTESIAN_POINT('Ctrl Pts',(182.818443863726,-5.32369091022383,
134.71491173846));
#220154=CARTESIAN_POINT('Ctrl Pts',(182.539996239912,0.412472435216218,
137.397080956463));
#220155=CARTESIAN_POINT('Ctrl Pts',(182.2615486161,5.76959376309122,134.020862255314));
#220156=CARTESIAN_POINT('Ctrl Pts',(181.983100992287,5.82474028301032,127.688835683913));
#220157=CARTESIAN_POINT('Ctrl Pts',(181.704653368474,0.527235037225083,
124.219824324685));
#220158=CARTESIAN_POINT('Ctrl Pts',(181.426205744661,-5.25477345090652,
126.801680146133));
#220159=CARTESIAN_POINT('Ctrl Pts',(181.147758120848,-6.20790184760947,
133.061803779016));
#220160=CARTESIAN_POINT('Ctrl Pts',(180.869310497035,-1.45627171922457,
137.247447428754));
#220161=CARTESIAN_POINT('Ctrl Pts',(180.590862873222,4.63360097629919,135.5122090613));
#220162=CARTESIAN_POINT('Ctrl Pts',(180.31241524941,6.46542073859599,129.450687965235));
#220163=CARTESIAN_POINT('Ctrl Pts',(180.033967625596,2.35583469548556,124.633125906077));
#220164=CARTESIAN_POINT('Ctrl Pts',(179.755520001784,-3.91864834385308,
125.4866270652));
#220165=CARTESIAN_POINT('Ctrl Pts',(179.477072377971,-6.59208499180493,
131.226865573221));
#220166=CARTESIAN_POINT('Ctrl Pts',(179.198624754158,-3.20771757354326,
136.578842667508));
#220167=CARTESIAN_POINT('Ctrl Pts',(178.920177130345,3.12438558908937,136.62435285703));
#220168=CARTESIAN_POINT('Ctrl Pts',(178.641729506532,6.58533103007041,131.32157450091));
#220169=CARTESIAN_POINT('Ctrl Pts',(178.363281882719,3.99467896572256,125.5435018533));
#220170=CARTESIAN_POINT('Ctrl Pts',(178.084834258906,-2.26688791720775,
124.599901402811));
#220171=CARTESIAN_POINT('Ctrl Pts',(177.806386635093,-6.44529554785546,
129.357895865998));
#220172=CARTESIAN_POINT('Ctrl Pts',(177.527939011281,-4.70079144021631,
135.445120772143));
#220173=CARTESIAN_POINT('Ctrl Pts',(177.249491387467,1.36351035455298,137.26771380997));
#220174=CARTESIAN_POINT('Ctrl Pts',(176.971043763655,6.17481274467203,133.150801016333));
#220175=CARTESIAN_POINT('Ctrl Pts',(176.692596139842,5.31176387881016,126.877624126216));
#220176=CARTESIAN_POINT('Ctrl Pts',(176.414148516029,-0.432536497586617,
124.212926239906));
#220177=CARTESIAN_POINT('Ctrl Pts',(176.135700892216,-5.77935696328393,
127.605434537195));
#220178=CARTESIAN_POINT('Ctrl Pts',(175.857253268403,-5.81523071700703,
133.937599626117));
#220179=CARTESIAN_POINT('Ctrl Pts',(175.57880564459,-0.50719153161477,137.390471133416));
#220180=CARTESIAN_POINT('Ctrl Pts',(175.300358020777,5.2669318936477,134.791028826034));
#220181=CARTESIAN_POINT('Ctrl Pts',(175.021910396965,6.20100221257536,128.528033194638));
#220182=CARTESIAN_POINT('Ctrl Pts',(174.743462773151,1.43665443394553,124.356871260137));
#220183=CARTESIAN_POINT('Ctrl Pts',(174.465015149339,-4.64790858500931,
126.110637067746));
#220184=CARTESIAN_POINT('Ctrl Pts',(174.186567525525,-6.46127067729819,
132.177705516496));
#220185=CARTESIAN_POINT('Ctrl Pts',(173.908119901713,-2.33704066777073,
136.982737094758));
#220186=CARTESIAN_POINT('Ctrl Pts',(173.6296722779,3.93481554465429,136.11014252095));
#220187=CARTESIAN_POINT('Ctrl Pts',(173.351224654087,6.59076849796787,130.361793579788));
#220188=CARTESIAN_POINT('Ctrl Pts',(173.072777030274,3.1901271785899,125.020142125741));
#220189=CARTESIAN_POINT('Ctrl Pts',(172.794329406461,-3.14208517153551,
124.993904890899));
#220190=CARTESIAN_POINT('Ctrl Pts',(172.515881782648,-6.58687474841394,
130.30719261232));
#220191=CARTESIAN_POINT('Ctrl Pts',(172.237434158836,-3.97864821822065,
136.077353442554));
#220192=CARTESIAN_POINT('Ctrl Pts',(171.958986535022,2.28576165674636,137.001891466644));
#220193=CARTESIAN_POINT('Ctrl Pts',(171.68053891121,6.44966823482829,132.231201406644));
#220194=CARTESIAN_POINT('Ctrl Pts',(171.402091287397,4.68664478891289,126.149314366529));
#220195=CARTESIAN_POINT('Ctrl Pts',(171.123643663584,-1.38317626268716,
124.345187419464));
#220196=CARTESIAN_POINT('Ctrl Pts',(170.845196039771,-6.18192590079466,
128.476725093301));
#220197=CARTESIAN_POINT('Ctrl Pts',(170.566748415958,-5.29978763994156,
134.747246102621));
#220198=CARTESIAN_POINT('Ctrl Pts',(170.288300792145,0.452596552998033,
137.394447971839));
#220199=CARTESIAN_POINT('Ctrl Pts',(170.009853168332,5.78906662430322,133.985681506144));
#220200=CARTESIAN_POINT('Ctrl Pts',(169.73140554452,5.80566727950083,127.653436560012));
#220201=CARTESIAN_POINT('Ctrl Pts',(169.452957920706,0.487143327451347,
124.216736891574));
#220202=CARTESIAN_POINT('Ctrl Pts',(169.174510296894,-5.27904154425138,
126.833741604011));
#220203=CARTESIAN_POINT('Ctrl Pts',(168.896062673081,-6.19404513230377,
133.099551214382));
#220204=CARTESIAN_POINT('Ctrl Pts',(168.617615049268,-1.41702383969606,
137.256192792574));
#220205=CARTESIAN_POINT('Ctrl Pts',(168.339167425455,4.66217313612931,135.483915791456));
#220206=CARTESIAN_POINT('Ctrl Pts',(168.060719801642,6.45706075967145,129.411356194513));
#220207=CARTESIAN_POINT('Ctrl Pts',(167.782272177829,2.3182249900303,124.618899610305));
#220208=CARTESIAN_POINT('Ctrl Pts',(167.503824554016,-3.95094629386185,
125.510579515201));
#220209=CARTESIAN_POINT('Ctrl Pts',(167.225376930203,-6.58939094815179,
131.266985637585));
#220210=CARTESIAN_POINT('Ctrl Pts',(166.946929306391,-3.1725072307341,136.59826196706));
#220211=CARTESIAN_POINT('Ctrl Pts',(166.668481682578,3.15975564613386,136.605226004165));
#220212=CARTESIAN_POINT('Ctrl Pts',(166.390034058765,6.58835744684964,131.281478139015));
#220213=CARTESIAN_POINT('Ctrl Pts',(166.111586434952,3.96258061306513,125.519282580138));
#220214=CARTESIAN_POINT('Ctrl Pts',(165.833138811139,-2.30461422130139,
124.613815547242));
#220215=CARTESIAN_POINT('Ctrl Pts',(165.554691187326,-6.45398117295568,
129.397157009033));
#220216=CARTESIAN_POINT('Ctrl Pts',(165.276243563513,-4.67245472117232,
135.473649841348));
#220217=CARTESIAN_POINT('Ctrl Pts',(164.9977959397,1.40282935726546,137.259293984466));
#220218=CARTESIAN_POINT('Ctrl Pts',(164.719348315888,6.18898178840028,133.11316970443));
#220219=CARTESIAN_POINT('Ctrl Pts',(164.440900692075,5.2877623045642,126.845362665158));
#220220=CARTESIAN_POINT('Ctrl Pts',(164.162453068262,-0.472652415616787,
124.215681336348));
#220221=CARTESIAN_POINT('Ctrl Pts',(163.884005444449,-5.79872265620017,
127.640674392099));
#220222=CARTESIAN_POINT('Ctrl Pts',(163.605557820636,-5.79605005908598,
133.97294053439));
#220223=CARTESIAN_POINT('Ctrl Pts',(163.327110196823,-0.467090610458611,
137.393436526853));
#220224=CARTESIAN_POINT('Ctrl Pts',(163.04866257301,5.29110229053537,134.758893652935));
#220225=CARTESIAN_POINT('Ctrl Pts',(162.770214949197,6.18703067124424,128.49032810919));
#220226=CARTESIAN_POINT('Ctrl Pts',(162.491767325384,1.39738011833125,124.34824539387));
#220227=CARTESIAN_POINT('Ctrl Pts',(162.213319701571,-4.67639449751423,
126.139017170363));
#220228=CARTESIAN_POINT('Ctrl Pts',(161.934872077759,-6.45279102471594,
132.217011660137));
#220229=CARTESIAN_POINT('Ctrl Pts',(161.656424453946,-2.29938783657033,
136.996848853628));
#220230=CARTESIAN_POINT('Ctrl Pts',(161.377976830133,3.96704044204275,136.086091878046));
#220231=CARTESIAN_POINT('Ctrl Pts',(161.09952920632,6.58795235511813,130.321681900999));
#220232=CARTESIAN_POINT('Ctrl Pts',(160.821081582507,3.15485789320466,125.000830084311));
#220233=CARTESIAN_POINT('Ctrl Pts',(160.542633958694,-3.17739684918762,
125.013139309456));
#220234=CARTESIAN_POINT('Ctrl Pts',(160.264186334881,-6.58977911164196,
130.347297999864));
#220235=CARTESIAN_POINT('Ctrl Pts',(159.985738711068,-3.94647629910411,
136.10147490719));
#220236=CARTESIAN_POINT('Ctrl Pts',(159.707291087255,2.32344543622502,136.98786256077));
#220237=CARTESIAN_POINT('Ctrl Pts',(159.428843463442,6.45823432228318,132.191914009409));
#220238=CARTESIAN_POINT('Ctrl Pts',(159.15039583963,4.65822136844951,126.120871676696));
#220239=CARTESIAN_POINT('Ctrl Pts',(158.871948215817,-1.42246945622416,
124.353726879487));
#220240=CARTESIAN_POINT('Ctrl Pts',(158.593500592004,-6.19598034212407,
128.514399356595));
#220241=CARTESIAN_POINT('Ctrl Pts',(158.315052968191,-5.2756879840792,134.779434361708));
#220242=CARTESIAN_POINT('Ctrl Pts',(158.036605344378,0.49270389964821,137.391570789103));
#220243=CARTESIAN_POINT('Ctrl Pts',(157.758157720565,5.80832496952254,133.950382871961));
#220244=CARTESIAN_POINT('Ctrl Pts',(157.479710096752,5.78637914485521,127.618154194761));
#220245=CARTESIAN_POINT('Ctrl Pts',(157.201262472939,0.447033566402335,
124.213893565282));
#220246=CARTESIAN_POINT('Ctrl Pts',(156.922814849126,-5.3031140207705,126.865950194636));
#220247=CARTESIAN_POINT('Ctrl Pts',(156.644367225313,-6.17995889437779,
133.137213600617));
#220248=CARTESIAN_POINT('Ctrl Pts',(156.365919601501,-1.37772345182797,
137.264699081378));
#220249=CARTESIAN_POINT('Ctrl Pts',(156.087471977688,4.69057253741941,135.455449118975));
#220250=CARTESIAN_POINT('Ctrl Pts',(155.809024353875,6.44846151198586,129.372076042081));
#220251=CARTESIAN_POINT('Ctrl Pts',(155.530576730062,2.28052938189546,124.604902519066));
#220252=CARTESIAN_POINT('Ctrl Pts',(155.252129106249,-3.98309784010292,
125.534728128207));
#220253=CARTESIAN_POINT('Ctrl Pts',(154.973681482436,-6.58645273219382,
131.307088559209));
#220254=CARTESIAN_POINT('Ctrl Pts',(154.695233858623,-3.13717932950269,
136.617466571466));
#220255=CARTESIAN_POINT('Ctrl Pts',(154.41678623481,3.19500861727094,136.585884198101));
#220256=CARTESIAN_POINT('Ctrl Pts',(154.138338610998,6.59113972962085,131.241364097354));
#220257=CARTESIAN_POINT('Ctrl Pts',(153.859890987185,3.93033542552574,125.495259147487));
#220258=CARTESIAN_POINT('Ctrl Pts',(153.581443363372,-2.3422551270676,124.627959084596));
#220259=CARTESIAN_POINT('Ctrl Pts',(153.302995739559,-6.46242764341012,
129.436470296516));
#220260=CARTESIAN_POINT('Ctrl Pts',(153.024548115746,-4.64394486260028,
135.502005888322));
#220261=CARTESIAN_POINT('Ctrl Pts',(152.746100491933,1.44209637762021,137.250634969033));
#220262=CARTESIAN_POINT('Ctrl Pts',(152.46765286812,6.20292149713234,133.075452838754));
#220263=CARTESIAN_POINT('Ctrl Pts',(152.189205244307,5.26356479034146,126.813247906226));
#220264=CARTESIAN_POINT('Ctrl Pts',(151.910757620494,-0.512750819337957,
124.218680578724));
#220265=CARTESIAN_POINT('Ctrl Pts',(151.632309996682,-5.8178734753159,127.676031478561));
#220266=CARTESIAN_POINT('Ctrl Pts',(151.353862372869,-5.77665462639848,
134.008164029768));
#220267=CARTESIAN_POINT('Ctrl Pts',(151.075414749056,-0.4269723810881,137.39615775966));
#220268=CARTESIAN_POINT('Ctrl Pts',(150.796967125243,5.31507662368183,134.72661194316));
#220269=CARTESIAN_POINT('Ctrl Pts',(150.51851950143,6.17282986721635,128.452708771068));
#220270=CARTESIAN_POINT('Ctrl Pts',(150.240071877617,1.35805402228283,124.339858761329));
#220271=CARTESIAN_POINT('Ctrl Pts',(149.961624253804,-4.70470712450132,
126.167570148998));
#220272=CARTESIAN_POINT('Ctrl Pts',(149.683176629991,-6.44407226158927,
132.256265457474));
#220273=CARTESIAN_POINT('Ctrl Pts',(149.404729006178,-2.26164980070799,
137.010731147569));
#220274=CARTESIAN_POINT('Ctrl Pts',(149.126281382365,3.99911833928874,136.061845518646));
#220275=CARTESIAN_POINT('Ctrl Pts',(148.847833758553,6.58489209327119,130.281588108047));
#220276=CARTESIAN_POINT('Ctrl Pts',(148.56938613474,3.11947170339994,124.981733094838));
#220277=CARTESIAN_POINT('Ctrl Pts',(148.290938510927,-3.21259078723097,
125.032588323847));
#220278=CARTESIAN_POINT('Ctrl Pts',(148.012490887114,-6.59243928818165,
130.387420324031));
#220279=CARTESIAN_POINT('Ctrl Pts',(147.734043263301,-3.91415814185689,
136.125400085308));
#220280=CARTESIAN_POINT('Ctrl Pts',(147.455595639488,2.36104311957866,136.973604522958));
#220281=CARTESIAN_POINT('Ctrl Pts',(147.177148015675,6.46656109749016,132.152575195872));
#220282=CARTESIAN_POINT('Ctrl Pts',(146.898700391862,4.6296253358803,126.092602535266));
#220283=CARTESIAN_POINT('Ctrl Pts',(146.62025276805,-1.46170993963237,124.362505370115));
#220284=CARTESIAN_POINT('Ctrl Pts',(146.341805144237,-6.20980518912327,
128.552158475246));
#220285=CARTESIAN_POINT('Ctrl Pts',(146.063357520424,-5.2513928356585,134.811475322978));
#220286=CARTESIAN_POINT('Ctrl Pts',(145.784909896611,0.532792988974217,
137.388449514872));
#220287=CARTESIAN_POINT('Ctrl Pts',(145.506462272798,5.82736808512415,133.914967660766));
#220288=CARTESIAN_POINT('Ctrl Pts',(145.228014648985,5.76687659380242,127.582989895561));
#220289=CARTESIAN_POINT('Ctrl Pts',(144.949567025172,0.406907240360106,
124.211294451169));
#220290=CARTESIAN_POINT('Ctrl Pts',(144.671119401359,-5.32698998844935,
126.898304724507));
#220291=CARTESIAN_POINT('Ctrl Pts',(144.392671777546,-6.16564365580234,
133.174789542127));
#220292=CARTESIAN_POINT('Ctrl Pts',(144.114224153734,-1.33837201191069,
137.272965979966));
#220293=CARTESIAN_POINT('Ctrl Pts',(143.83577652992,4.71879812781917,135.426810098699));
#220294=CARTESIAN_POINT('Ctrl Pts',(143.557328906108,6.43962331418753,129.332848963481));
#220295=CARTESIAN_POINT('Ctrl Pts',(143.278881282295,2.24274926790569,124.591135151027));
#220296=CARTESIAN_POINT('Ctrl Pts',(143.000433658482,-4.01510179118866,
125.559072009383));
#220297=CARTESIAN_POINT('Ctrl Pts',(142.721986034669,-6.58327045280769,
131.347172852065));
#220298=CARTESIAN_POINT('Ctrl Pts',(142.443538410856,-3.10173517893752,
136.636455769093));
#220299=CARTESIAN_POINT('Ctrl Pts',(142.165090787043,3.23014319618891,136.566328155556));
#220300=CARTESIAN_POINT('Ctrl Pts',(141.886643163231,6.5936777752854,131.201233862367));
#220301=CARTESIAN_POINT('Ctrl Pts',(141.608195539417,3.89794459796173,125.471432445543));
#220302=CARTESIAN_POINT('Ctrl Pts',(141.329747915605,-2.37980923970876,
124.642331490782));
#220303=CARTESIAN_POINT('Ctrl Pts',(141.051300291792,-6.47063464623165,
129.475834271677));
#220304=CARTESIAN_POINT('Ctrl Pts',(140.772852667979,-4.61526292094352,
135.530187862324));
#220305=CARTESIAN_POINT('Ctrl Pts',(140.494405044166,1.48130996056343,137.241737084533));
#220306=CARTESIAN_POINT('Ctrl Pts',(140.215957420353,6.21663135432719,133.037651816923));
#220307=CARTESIAN_POINT('Ctrl Pts',(139.93750979654,5.23917223278974,126.781281039444));
#220308=CARTESIAN_POINT('Ctrl Pts',(139.659062172727,-0.552830222889001,
124.221923855894));
#220309=CARTESIAN_POINT('Ctrl Pts',(139.380614548914,-5.83680871099059,
127.711504486408));
#220310=CARTESIAN_POINT('Ctrl Pts',(139.102166925101,-5.75704513764935,
134.043268807033));
#220311=CARTESIAN_POINT('Ctrl Pts',(138.823719301288,-0.386838330098996,
137.398634730999));
#220312=CARTESIAN_POINT('Ctrl Pts',(138.545271677476,5.33885400470937,134.694184892919));
#220313=CARTESIAN_POINT('Ctrl Pts',(138.266824053663,6.15840032670771,128.41517657427));
#220314=CARTESIAN_POINT('Ctrl Pts',(137.98837642985,1.31867760304303,124.331711673279));
#220315=CARTESIAN_POINT('Ctrl Pts',(137.709928806037,-4.7328454168358,126.196294945608));
#220316=CARTESIAN_POINT('Ctrl Pts',(137.431481182224,-6.43511471099507,
132.295465453942));
#220317=CARTESIAN_POINT('Ctrl Pts',(137.153033558411,-2.22382795858067,
137.024383462168));
#220318=CARTESIAN_POINT('Ctrl Pts',(136.874585934598,4.03104804773404,136.037404341212));
#220319=CARTESIAN_POINT('Ctrl Pts',(136.596138310785,6.5815878258261,130.241513686623));
#220320=CARTESIAN_POINT('Ctrl Pts',(136.317690686972,3.08396992042408,124.96285186497));
#220321=CARTESIAN_POINT('Ctrl Pts',(136.03924306316,-3.24766568154122,125.052251213384));
#220322=CARTESIAN_POINT('Ctrl Pts',(135.760795439346,-6.5948551794591,130.427558098075));
#220323=CARTESIAN_POINT('Ctrl Pts',(135.482347815534,-3.88169494404043,
136.149128090351));
#220324=CARTESIAN_POINT('Ctrl Pts',(135.203900191721,2.3985533136112,136.959117881544));
#220325=CARTESIAN_POINT('Ctrl Pts',(134.925452567908,6.47464825189767,132.113186423748));
#220326=CARTESIAN_POINT('Ctrl Pts',(134.647004944095,4.60085775084163,126.064507989766));
#220327=CARTESIAN_POINT('Ctrl Pts',(134.368557320282,-1.50089625884118,
124.371522566057));
#220328=CARTESIAN_POINT('Ctrl Pts',(134.090109696469,-6.22339992950755,
128.590001050074));
#220329=CARTESIAN_POINT('Ctrl Pts',(133.811662072656,-5.22690309494509,
134.843367799137));
#220330=CARTESIAN_POINT('Ctrl Pts',(133.533214448844,0.572862335460145,
137.385084264805));
#220331=CARTESIAN_POINT('Ctrl Pts',(133.25476682503,5.84619526545829,133.879437184883));
#220332=CARTESIAN_POINT('Ctrl Pts',(132.976319201218,5.7471603490167,127.547944965438));
#220333=CARTESIAN_POINT('Ctrl Pts',(132.697871577405,0.366765836220533,
124.208939645549));
#220334=CARTESIAN_POINT('Ctrl Pts',(132.419423953592,-5.35066856255522,
126.930803994717));
#220335=CARTESIAN_POINT('Ctrl Pts',(132.140976329779,-6.15109994703373,
133.212277646521));
#220336=CARTESIAN_POINT('Ctrl Pts',(131.862528705966,-1.29897097812634,
137.280993182001));
#220337=CARTESIAN_POINT('Ctrl Pts',(131.584081082153,4.74684886141891,135.397999791857));
#220338=CARTESIAN_POINT('Ctrl Pts',(131.30563345834,6.43054649377913,129.293676412286));
#220339=CARTESIAN_POINT('Ctrl Pts',(131.027185834528,2.20488604801711,124.577598016342));
#220340=CARTESIAN_POINT('Ctrl Pts',(130.748738210715,-4.04695696120101,
125.583610256657));
#220341=CARTESIAN_POINT('Ctrl Pts',(130.470290586902,-6.57984422791396,
131.387237030814));
#220342=CARTESIAN_POINT('Ctrl Pts',(130.191842963089,-3.06617609243459,
136.65522885629));
#220343=CARTESIAN_POINT('Ctrl Pts',(129.913395339276,3.26515808096253,136.546558601182));
#220344=CARTESIAN_POINT('Ctrl Pts',(129.634947715463,6.59597148979528,131.161088921098));
#220345=CARTESIAN_POINT('Ctrl Pts',(129.35650009165,3.86540933062731,125.447803357213));
#220346=CARTESIAN_POINT('Ctrl Pts',(129.078052467837,-2.41727516764341,
124.656932233223));
#220347=CARTESIAN_POINT('Ctrl Pts',(128.799604844024,-6.47860187730669,
129.515247475871));
#220348=CARTESIAN_POINT('Ctrl Pts',(128.521157220212,-4.58640995902212,
135.558194719059));
#220349=CARTESIAN_POINT('Ctrl Pts',(128.242709596398,1.52046865302106,137.232600660681));
#220350=CARTESIAN_POINT('Ctrl Pts',(127.964261972586,6.23011085196111,132.999768039666));
#220351=CARTESIAN_POINT('Ctrl Pts',(127.685814348773,5.2145855357842,126.749463249355));
#220352=CARTESIAN_POINT('Ctrl Pts',(127.40736672496,-0.592889141112855,
124.225411047681));
#220353=CARTESIAN_POINT('Ctrl Pts',(127.128919101147,-5.85552766157182,
127.747092101177));
#220354=CARTESIAN_POINT('Ctrl Pts',(126.850471477334,-5.7372223194756,134.078253565364));
#220355=CARTESIAN_POINT('Ctrl Pts',(126.572023853521,-0.346689944673359,
137.400867349086));
#220356=CARTESIAN_POINT('Ctrl Pts',(126.293576229708,5.36243355253846,134.66161370381));
#220357=CARTESIAN_POINT('Ctrl Pts',(126.015128605896,6.14374258441013,128.377732909565));
#220358=CARTESIAN_POINT('Ctrl Pts',(125.736680982083,1.27925231971985,124.323804431618));
#220359=CARTESIAN_POINT('Ctrl Pts',(125.45823335827,-4.76080833184274,126.225190495787));
#220360=CARTESIAN_POINT('Ctrl Pts',(125.179785734457,-6.42591870485886,
132.334610196974));
#220361=CARTESIAN_POINT('Ctrl Pts',(124.901338110644,-2.1859237116904,137.037805291532));
#220362=CARTESIAN_POINT('Ctrl Pts',(124.622890486831,4.06282838421153,136.012769251418));
#220363=CARTESIAN_POINT('Ctrl Pts',(124.344442863018,6.5780396752237,130.201460121699));
#220364=CARTESIAN_POINT('Ctrl Pts',(124.065995239205,3.04835385980878,124.944187094356));
#220365=CARTESIAN_POINT('Ctrl Pts',(123.787547615392,-3.28262023240536,
125.07212724945));
#220366=CARTESIAN_POINT('Ctrl Pts',(123.509099991579,-6.59702669595264,
130.467709834674));
#220367=CARTESIAN_POINT('Ctrl Pts',(123.230652367767,-3.84908790859021,
136.17265804307));
#220368=CARTESIAN_POINT('Ctrl Pts',(122.952204743954,2.43597462836867,136.944403173336));
#220369=CARTESIAN_POINT('Ctrl Pts',(122.673757120141,6.48249548583303,132.073749152604));
#220370=CARTESIAN_POINT('Ctrl Pts',(122.395309496328,4.57191967932717,126.036589081248));
#220371=CARTESIAN_POINT('Ctrl Pts',(122.116861872515,-1.54002696178715,
124.380778133181));
#220372=CARTESIAN_POINT('Ctrl Pts',(121.838414248702,-6.23676405951882,
128.627925678811));
#220373=CARTESIAN_POINT('Ctrl Pts',(121.559966624889,-5.20221966941523,
134.8751106084));
#220374=CARTESIAN_POINT('Ctrl Pts',(121.281519001076,0.612910454321425,
137.381475163605));
#220375=CARTESIAN_POINT('Ctrl Pts',(121.003071377263,5.86480581287692,133.843792760907));
#220376=CARTESIAN_POINT('Ctrl Pts',(120.724623753451,5.72723114109079,127.513020702994));
#220377=CARTESIAN_POINT('Ctrl Pts',(120.446176129638,0.326610841437887,
124.206829235678));
#220378=CARTESIAN_POINT('Ctrl Pts',(120.167728505825,-5.3741488656698,126.963446800991));
#220379=CARTESIAN_POINT('Ctrl Pts',(119.889280882012,-6.13632830699453,
133.249676524665));
#220380=CARTESIAN_POINT('Ctrl Pts',(119.610833258199,-1.25952181049465,
137.288780390037));
#220381=CARTESIAN_POINT('Ctrl Pts',(119.332385634386,4.77472369878856,135.369019266025));
#220382=CARTESIAN_POINT('Ctrl Pts',(119.053938010573,6.42123138710552,129.254559840052));
#220383=CARTESIAN_POINT('Ctrl Pts',(118.77549038676,2.16694112526505,124.564291616636));
#220384=CARTESIAN_POINT('Ctrl Pts',(118.497042762948,-4.07866216973492,
125.608341960757));
#220385=CARTESIAN_POINT('Ctrl Pts',(118.218595139134,-6.57617418447253,
131.427279610862));
#220386=CARTESIAN_POINT('Ctrl Pts',(117.940147515322,-3.03050338764912,
136.673785137412));
#220387=CARTESIAN_POINT('Ctrl Pts',(117.661699891509,3.30005197410286,136.526576267552));
#220388=CARTESIAN_POINT('Ctrl Pts',(117.383252267696,6.59802078815589,131.120930761129));
#220389=CARTESIAN_POINT('Ctrl Pts',(117.104804643883,3.83273082912851,125.424372758082));
#220390=CARTESIAN_POINT('Ctrl Pts',(116.82635702007,-2.45465152255762,124.671760770883));
#220391=CARTESIAN_POINT('Ctrl Pts',(116.547909396257,-6.48632904140672,
129.554708448625));
#220392=CARTESIAN_POINT('Ctrl Pts',(116.269461772444,-4.55738704599302,
135.586025420722));
#220393=CARTESIAN_POINT('Ctrl Pts',(115.991014148631,1.55957100395386,137.223226036031));
#220394=CARTESIAN_POINT('Ctrl Pts',(115.712566524818,6.24335949054626,132.961802910777));
#220395=CARTESIAN_POINT('Ctrl Pts',(115.434118901006,5.18980561039392,126.717795714978));
#220396=CARTESIAN_POINT('Ctrl Pts',(115.155671277193,-0.632926089611396,
124.229142024863));
#220397=CARTESIAN_POINT('Ctrl Pts',(114.87722365338,-5.87402963342224,127.782793004156));
#220398=CARTESIAN_POINT('Ctrl Pts',(114.598776029567,-5.71718690641897,
134.113117008387));
#220399=CARTESIAN_POINT('Ctrl Pts',(114.320328405754,-0.306528712524212,
137.40285553119));
#220400=CARTESIAN_POINT('Ctrl Pts',(114.041880781941,5.38581439342023,134.628899582769));
#220401=CARTESIAN_POINT('Ctrl Pts',(113.763433158128,6.12885718347172,128.340379164441));
#220402=CARTESIAN_POINT('Ctrl Pts',(113.484985534315,1.23977963323159,124.316137329349));
#220403=CARTESIAN_POINT('Ctrl Pts',(113.206537910502,-4.78859483334625,
126.254255728798));
#220404=CARTESIAN_POINT('Ctrl Pts',(112.92809028669,-6.41648458394181,132.373698236044));
#220405=CARTESIAN_POINT('Ctrl Pts',(112.649642662877,-2.14793846459313,
137.050996138312));
#220406=CARTESIAN_POINT('Ctrl Pts',(112.371195039064,4.09445817108915,135.987941162125));
#220407=CARTESIAN_POINT('Ctrl Pts',(112.092747415251,6.57424777294209,130.161428897475));
#220408=CARTESIAN_POINT('Ctrl Pts',(111.814299791438,3.01262484132005,124.925739474628));
#220409=CARTESIAN_POINT('Ctrl Pts',(111.535852167625,-3.31745314456969,
125.092215695531));
#220410=CARTESIAN_POINT('Ctrl Pts',(111.257404543812,-6.59895375719588,
130.507874045991));
#220411=CARTESIAN_POINT('Ctrl Pts',(110.978956919999,-3.816338243772,136.195989071554));
#220412=CARTESIAN_POINT('Ctrl Pts',(110.700509296186,2.47330567719032,136.929460943594));
#220413=CARTESIAN_POINT('Ctrl Pts',(110.422061672374,6.49010250851429,132.0342648438));
#220414=CARTESIAN_POINT('Ctrl Pts',(110.143614048561,4.54281219364771,126.008846844259));
#220415=CARTESIAN_POINT('Ctrl Pts',(109.865166424748,-1.57910059846782,
124.390271728514));
#220416=CARTESIAN_POINT('Ctrl Pts',(109.586718800935,-6.24989708394428,
128.665930956147));
#220417=CARTESIAN_POINT('Ctrl Pts',(109.308271177122,-5.17734347372243,
134.906702574525));
#220418=CARTESIAN_POINT('Ctrl Pts',(109.029823553309,0.652935861560398,
137.377622345005));
#220419=CARTESIAN_POINT('Ctrl Pts',(108.751375929496,5.88319903775945,133.808035709655));
#220420=CARTESIAN_POINT('Ctrl Pts',(108.472928305683,5.70708970850866,127.478218402361));
#220421=CARTESIAN_POINT('Ctrl Pts',(108.19448068187,0.286443743970404,124.204963299759));
#220422=CARTESIAN_POINT('Ctrl Pts',(107.916033058058,-5.39743002772183,
126.996231933739));
#220423=CARTESIAN_POINT('Ctrl Pts',(107.637585434244,-6.12132928305326,
133.286984790727));
#220424=CARTESIAN_POINT('Ctrl Pts',(107.359137810432,-1.22002597081922,
137.296327315513));
#220425=CARTESIAN_POINT('Ctrl Pts',(107.080690186619,4.80242160701559,135.339869595089));
#220426=CARTESIAN_POINT('Ctrl Pts',(106.802242562806,6.41167833934146,129.215500696253));
#220427=CARTESIAN_POINT('Ctrl Pts',(106.523794938993,2.12891590571267,124.551216444981));
#220428=CARTESIAN_POINT('Ctrl Pts',(106.24534731518,-4.11021624194206,125.633266205238));
#220429=CARTESIAN_POINT('Ctrl Pts',(105.966899691367,-6.57226045847839,
131.467299108419));
#220430=CARTESIAN_POINT('Ctrl Pts',(105.688452067554,-2.99471838644612,
136.692123924851));
#220431=CARTESIAN_POINT('Ctrl Pts',(105.410004443742,3.33482358260376,136.506381895117));
#220432=CARTESIAN_POINT('Ctrl Pts',(105.131556819929,6.59982559442975,131.080760870538));
#220433=CARTESIAN_POINT('Ctrl Pts',(104.853109196116,3.79991030437941,125.401141516381));
#220434=CARTESIAN_POINT('Ctrl Pts',(104.574661572303,-2.49193691945696,
124.686816554284));
#220435=CARTESIAN_POINT('Ctrl Pts',(104.29621394849,-6.49381585219884,129.594215727701));
#220436=CARTESIAN_POINT('Ctrl Pts',(104.017766324677,-4.52819525731082,
135.613678936038));
#220437=CARTESIAN_POINT('Ctrl Pts',(103.739318700864,1.59861556440955,137.213613557961));
#220438=CARTESIAN_POINT('Ctrl Pts',(103.460871077051,6.25637677914949,132.923757837073));
#220439=CARTESIAN_POINT('Ctrl Pts',(103.182423453238,5.16483337484823,126.686279609768));
#220440=CARTESIAN_POINT('Ctrl Pts',(102.903975829425,-0.672939584800916,
124.233116649188));
#220441=CARTESIAN_POINT('Ctrl Pts',(102.625528205613,-5.89231394094447,
127.818605872432));
#220442=CARTESIAN_POINT('Ctrl Pts',(102.347080581799,-5.69693964089892,
134.147857844226));
#220443=CARTESIAN_POINT('Ctrl Pts',(102.068632957987,-0.266356121840884,
137.40459920364));
#220444=CARTESIAN_POINT('Ctrl Pts',(101.790185334174,5.40899566096888,134.59604374203));
#220445=CARTESIAN_POINT('Ctrl Pts',(101.511737710361,6.11374467547657,128.303116723058));
#220446=CARTESIAN_POINT('Ctrl Pts',(101.233290086548,1.20026100625305,124.308710650579));
#220447=CARTESIAN_POINT('Ctrl Pts',(100.954842462735,-4.81620389170723,
126.28348956762));
#220448=CARTESIAN_POINT('Ctrl Pts',(100.676394838922,-6.40681269782886,
132.412728122731));
#220449=CARTESIAN_POINT('Ctrl Pts',(100.397947215109,-2.10987362484612,
137.063955513716));
#220450=CARTESIAN_POINT('Ctrl Pts',(100.119499591297,4.12593623631335,135.962920993349));
#220451=CARTESIAN_POINT('Ctrl Pts',(99.8410519674839,6.5702122594916,130.121421497322));
#220452=CARTESIAN_POINT('Ctrl Pts',(99.5626043436712,2.97678418891005,124.907509689368));
#220453=CARTESIAN_POINT('Ctrl Pts',(99.2841567198582,-3.35216312728773,
125.112515807244));
#220454=CARTESIAN_POINT('Ctrl Pts',(99.0057090960455,-6.6006362917809,130.548049243728));
#220455=CARTESIAN_POINT('Ctrl Pts',(98.7272614722323,-3.78344716313679,
136.219120311263));
#220456=CARTESIAN_POINT('Ctrl Pts',(98.4488138484198,2.51054507676055,136.914291746006));
#220457=CARTESIAN_POINT('Ctrl Pts',(98.1703662246066,6.49746903806041,131.994734960442));
#220458=CARTESIAN_POINT('Ctrl Pts',(97.8919186007939,4.51353637239165,125.981282306795));
#220459=CARTESIAN_POINT('Ctrl Pts',(97.6134709769809,-1.61811572099509,
124.400003000271));
#220460=CARTESIAN_POINT('Ctrl Pts',(97.335023353168,-6.26279851613479,128.704015473778));
#220461=CARTESIAN_POINT('Ctrl Pts',(97.0565757293552,-5.15227542966332,
134.938142526861));
#220462=CARTESIAN_POINT('Ctrl Pts',(96.7781281055422,0.692937074020952,
137.373525951775));
#220463=CARTESIAN_POINT('Ctrl Pts',(96.4996804817294,5.90137425853808,133.772167356118));
#220464=CARTESIAN_POINT('Ctrl Pts',(96.2212328579164,5.6867367976186,127.443539353151));
#220465=CARTESIAN_POINT('Ctrl Pts',(95.9427852341037,0.246266032224636,
124.203341906934));
#220466=CARTESIAN_POINT('Ctrl Pts',(95.6643376102905,-5.42051118601915,
127.029158178097));
#220467=CARTESIAN_POINT('Ctrl Pts',(95.3858899864779,-6.10610343100435,
133.324201062238));
#220468=CARTESIAN_POINT('Ctrl Pts',(95.1074423626648,-1.18048492263276,
137.303633678775));
#220469=CARTESIAN_POINT('Ctrl Pts',(94.828994738852,4.82994155974394,135.3105518592));
#220470=CARTESIAN_POINT('Ctrl Pts',(94.5505471150391,6.40188770447863,129.176500428244));
#220471=CARTESIAN_POINT('Ctrl Pts',(94.2720994912261,2.09081179839861,124.538372985881));
#220472=CARTESIAN_POINT('Ctrl Pts',(93.9936518674133,-4.14161800857485,
125.658382066524));
#220473=CARTESIAN_POINT('Ctrl Pts',(93.7152042436005,-6.56810319495607,
131.507294040545));
#220474=CARTESIAN_POINT('Ctrl Pts',(93.4367566197874,-2.95882241485189,
136.710244539055));
#220475=CARTESIAN_POINT('Ctrl Pts',(93.1583089959747,3.36947161799043,136.485976232185));
#220476=CARTESIAN_POINT('Ctrl Pts',(92.8798613721617,6.60138584173913,131.040580737834));
#220477=CARTESIAN_POINT('Ctrl Pts',(92.6014137483489,3.76694897255651,125.37811049295));
#220478=CARTESIAN_POINT('Ctrl Pts',(92.3229661245359,-2.5291299767175,124.702099025532));
#220479=CARTESIAN_POINT('Ctrl Pts',(92.044518500723,-6.50106203225643,129.633767849141));
#220480=CARTESIAN_POINT('Ctrl Pts',(91.7660708769102,-4.49883567468812,
135.641154240296));
#220481=CARTESIAN_POINT('Ctrl Pts',(91.4876232530973,1.63760088757763,137.203763582666));
#220482=CARTESIAN_POINT('Ctrl Pts',(91.2091756292845,6.26916223541028,132.885634228324));
#220483=CARTESIAN_POINT('Ctrl Pts',(90.9307280054714,5.13966975450256,126.654916101563));
#220484=CARTESIAN_POINT('Ctrl Pts',(90.6522803816587,-0.71292814396669,
124.237334773374));
#220485=CARTESIAN_POINT('Ctrl Pts',(90.3738327578456,-5.91037990660673,
127.85452937895));
#220486=CARTESIAN_POINT('Ctrl Pts',(90.0953851340328,-5.67648127318543,
134.182474785545));
#220487=CARTESIAN_POINT('Ctrl Pts',(89.8169375102199,-0.226173661233629,
137.406098301819));
#220488=CARTESIAN_POINT('Ctrl Pts',(89.5384898864071,5.43197649619419,134.563047399079));
#220489=CARTESIAN_POINT('Ctrl Pts',(89.260042262594,6.09840562042418,128.265946966186));
#220490=CARTESIAN_POINT('Ctrl Pts',(88.9815946387814,1.1606979031614,124.301524670509));
#220491=CARTESIAN_POINT('Ctrl Pts',(88.7031470149683,-4.84363448386183,
126.312890928981));
#220492=CARTESIAN_POINT('Ctrl Pts',(88.4246993911556,-6.39690340491527,
132.45169841077));
#220493=CARTESIAN_POINT('Ctrl Pts',(88.1462517673426,-2.07173060295614,
137.076682937528));
#220494=CARTESIAN_POINT('Ctrl Pts',(87.8678041435297,4.15726141345302,135.937709672222));
#220495=CARTESIAN_POINT('Ctrl Pts',(87.5893565197169,6.5659332844097,130.081439403729));
#220496=CARTESIAN_POINT('Ctrl Pts',(87.3109088959039,2.94083323066708,124.889498414087));
#220497=CARTESIAN_POINT('Ctrl Pts',(87.032461272091,-3.38674889436835,125.133026832359));
#220498=CARTESIAN_POINT('Ctrl Pts',(86.7540136482781,-6.60207423736065,
130.588233939178));
#220499=CARTESIAN_POINT('Ctrl Pts',(86.4755660244652,-3.75041588547566,
136.242050905059));
#220500=CARTESIAN_POINT('Ctrl Pts',(86.1971184006524,2.54769144715974,136.898896142674));
#220501=CARTESIAN_POINT('Ctrl Pts',(85.9186707768394,6.50459480150186,131.955160967326));
#220502=CARTESIAN_POINT('Ctrl Pts',(85.6402231530266,4.48409330038545,125.953896490271));
#220503=CARTESIAN_POINT('Ctrl Pts',(85.3617755292137,-1.65707088364924,
124.409971587854));
#220504=CARTESIAN_POINT('Ctrl Pts',(85.0833279054008,-6.27546787802325,
128.742177820471));
#220505=CARTESIAN_POINT('Ctrl Pts',(84.8048802815879,-5.12701646614329,
134.969429300388));
#220506=CARTESIAN_POINT('Ctrl Pts',(84.526432657775,0.732912609443495,137.369186135708));
#220507=CARTESIAN_POINT('Ctrl Pts',(84.2479850339622,5.91933080172332,133.73618902941));
#220508=CARTESIAN_POINT('Ctrl Pts',(83.9695374101491,5.6661731626052,127.408984840408));
#220509=CARTESIAN_POINT('Ctrl Pts',(83.6910897863363,0.206079195000604,
124.201965117285));
#220510=CARTESIAN_POINT('Ctrl Pts',(83.4126421625234,-5.44339148528112,
127.062224313968));
#220511=CARTESIAN_POINT('Ctrl Pts',(83.1341945387106,-6.09065131504733,
133.361323960135));
#220512=CARTESIAN_POINT('Ctrl Pts',(82.8557469148977,-1.14090013114324,
137.310699209084));
#220513=CARTESIAN_POINT('Ctrl Pts',(82.5772992910847,4.85728253721157,135.281067144739));
#220514=CARTESIAN_POINT('Ctrl Pts',(82.2988516672719,6.39185984531258,129.137560481192));
#220515=CARTESIAN_POINT('Ctrl Pts',(82.0204040434589,2.05263021528453,124.52576171526));
#220516=CARTESIAN_POINT('Ctrl Pts',(81.7419564196462,-4.17286630602932,
125.683688613938));
#220517=CARTESIAN_POINT('Ctrl Pts',(81.4635087958331,-6.56370254795435,
131.547262925216));
#220518=CARTESIAN_POINT('Ctrl Pts',(81.1850611720204,-2.92281680300497,
136.728146308557));
#220519=CARTESIAN_POINT('Ctrl Pts',(80.9066135482074,3.40399479636718,136.465360034899));
#220520=CARTESIAN_POINT('Ctrl Pts',(80.6281659243945,6.60270147226842,131.000391851905));
#220521=CARTESIAN_POINT('Ctrl Pts',(80.3497183005816,3.73384805505426,125.355280541214));
#220522=CARTESIAN_POINT('Ctrl Pts',(80.0712706767688,-2.56622931613655,
124.717607618327));
#220523=CARTESIAN_POINT('Ctrl Pts',(79.7928230529558,-6.50806731306963,
129.673363347327));
#220524=CARTESIAN_POINT('Ctrl Pts',(79.514375429143,-4.46930938605503,135.668450315387));
#220525=CARTESIAN_POINT('Ctrl Pts',(79.23592780533,1.67652552884245,137.193676475141));
#220526=CARTESIAN_POINT('Ctrl Pts',(78.9574801815173,6.28171538555901,132.847433497217));
#220527=CARTESIAN_POINT('Ctrl Pts',(78.6790325577042,5.11431568180404,126.62370635255));
#220528=CARTESIAN_POINT('Ctrl Pts',(78.4005849338915,-0.752890285318027,
124.241796241119));
#220529=CARTESIAN_POINT('Ctrl Pts',(78.1221373100785,-5.92822686096799,
127.890562192549));
#220530=CARTESIAN_POINT('Ctrl Pts',(77.8436896862655,-5.65581256137084,
134.216966549603));
#220531=CARTESIAN_POINT('Ctrl Pts',(77.5652420624528,-0.185982819678218,
137.407352770183));
#220532=CARTESIAN_POINT('Ctrl Pts',(77.2867944386398,5.45475604753291,134.529911776607));
#220533=CARTESIAN_POINT('Ctrl Pts',(77.008346814827,6.08284058670873,128.228871271165));
#220534=CARTESIAN_POINT('Ctrl Pts',(76.729899191014,1.12109178998211,124.294579655415));
#220535=CARTESIAN_POINT('Ctrl Pts',(76.4514515672013,-4.8708855933594,126.342458723402));
#220536=CARTESIAN_POINT('Ctrl Pts',(76.1730039433881,-6.38675707239351,
132.4906076561));
#220537=CARTESIAN_POINT('Ctrl Pts',(75.8945563195755,-2.03351081232684,
137.089177938131));
#220538=CARTESIAN_POINT('Ctrl Pts',(75.6161086957625,4.18843254174224,135.912308132958));
#220539=CARTESIAN_POINT('Ctrl Pts',(75.3376610719495,6.56141100625526,130.041484098248));
#220540=CARTESIAN_POINT('Ctrl Pts',(75.0592134481368,2.90477329876725,124.871706316201));
#220541=CARTESIAN_POINT('Ctrl Pts',(74.7807658243238,-3.42120916422307,
125.153748010832));
#220542=CARTESIAN_POINT('Ctrl Pts',(74.5023182005109,-6.60326754065171,
130.628426643279));
#220543=CARTESIAN_POINT('Ctrl Pts',(74.223870576698,-3.71724563477466,136.264780003243));
#220544=CARTESIAN_POINT('Ctrl Pts',(73.9454229528852,2.58474341191554,136.883274704086));
#220545=CARTESIAN_POINT('Ctrl Pts',(73.6669753290721,6.51147953479087,131.915544330879));
#220546=CARTESIAN_POINT('Ctrl Pts',(73.3885277052595,4.45448406865298,125.926690409479));
#220547=CARTESIAN_POINT('Ctrl Pts',(73.1100800814464,-1.6959646429323,124.420177121874));
#220548=CARTESIAN_POINT('Ctrl Pts',(72.8316324576336,-6.28790470014163,
128.780416582107));
#220549=CARTESIAN_POINT('Ctrl Pts',(72.5531848338207,-5.1015675191428,135.000561735763));
#220550=CARTESIAN_POINT('Ctrl Pts',(72.2747372100078,0.772860986519783,
137.364603057617));
#220551=CARTESIAN_POINT('Ctrl Pts',(71.996289586195,5.93706800192887,133.700102062723));
#220552=CARTESIAN_POINT('Ctrl Pts',(71.7178419623819,5.64539956546153,127.374556144564));
#220553=CARTESIAN_POINT('Ctrl Pts',(71.4393943385692,0.165884721436248,
124.20083298183));
#220554=CARTESIAN_POINT('Ctrl Pts',(71.1609467147562,-5.46607007766984,
127.095429116077));
#220555=CARTESIAN_POINT('Ctrl Pts',(70.8824990909434,-6.07497350776591,
133.398352108815));
#220556=CARTESIAN_POINT('Ctrl Pts',(70.6040514671303,-1.10127306317963,
137.317523644624));
#220557=CARTESIAN_POINT('Ctrl Pts',(70.3256038433176,4.88444352628841,135.251416544269));
#220558=CARTESIAN_POINT('Ctrl Pts',(70.0471562195047,6.38159513342946,129.098682298033));
#220559=CARTESIAN_POINT('Ctrl Pts',(69.7687085956917,2.01437257120279,124.513383100429));
#220560=CARTESIAN_POINT('Ctrl Pts',(69.4902609718789,-4.20395997638847,
125.709184909736));
#220561=CARTESIAN_POINT('Ctrl Pts',(69.211813348066,-6.5590586805409,131.587204281367));
#220562=CARTESIAN_POINT('Ctrl Pts',(68.9333657242531,-2.88670288510633,
136.745828570004));
#220563=CARTESIAN_POINT('Ctrl Pts',(68.6549181004402,3.43839183846502,136.444534067195));
#220564=CARTESIAN_POINT('Ctrl Pts',(68.3764704766273,6.60377243726651,130.960195701968));
#220565=CARTESIAN_POINT('Ctrl Pts',(68.0980228528144,3.70060877843901,125.332652507142));
#220566=CARTESIAN_POINT('Ctrl Pts',(67.8195752290015,-2.6032335629848,124.733341757993));
#220567=CARTESIAN_POINT('Ctrl Pts',(67.5411276051886,-6.51483143505509,
129.713000755032));
#220568=CARTESIAN_POINT('Ctrl Pts',(67.2626799813758,-4.43961748551916,
135.695566149845));
#220569=CARTESIAN_POINT('Ctrl Pts',(66.9842323575627,1.71538804583728,137.183352609169));
#220570=CARTESIAN_POINT('Ctrl Pts',(66.7057847337499,6.29403576443417,132.809157059292));
#220571=CARTESIAN_POINT('Ctrl Pts',(66.4273371099371,5.08877209625689,126.592651519219));
#220572=CARTESIAN_POINT('Ctrl Pts',(66.1488894861241,-0.792824528042931,
124.246500887099));
#220573=CARTESIAN_POINT('Ctrl Pts',(65.8704418623113,-5.94585414270274,
127.92670297802));
#220574=CARTESIAN_POINT('Ctrl Pts',(65.5919942384984,-5.63493427134196,
134.251331858291));
#220575=CARTESIAN_POINT('Ctrl Pts',(65.3135466146855,-0.145785086460763,
137.408362562243));
#220576=CARTESIAN_POINT('Ctrl Pts',(65.0350989908726,5.47733347088038,134.496638102466));
#220577=CARTESIAN_POINT('Ctrl Pts',(64.7566513670597,6.06705015109826,128.191891011849));
#220578=CARTESIAN_POINT('Ctrl Pts',(64.4782037432468,1.0814441343344,124.28787586265));
#220579=CARTESIAN_POINT('Ctrl Pts',(64.199756119434,-4.89795621039988,126.37219185524));
#220580=CARTESIAN_POINT('Ctrl Pts',(63.921308495621,-6.37637407623982,132.529454416925));
#220581=CARTESIAN_POINT('Ctrl Pts',(63.6428608718081,-1.99521566920641,
137.101440052517));
#220582=CARTESIAN_POINT('Ctrl Pts',(63.3644132479953,4.21944846612332,135.886717316821));
#220583=CARTESIAN_POINT('Ctrl Pts',(63.0859656241823,6.556645592603,130.001557061437));
#220584=CARTESIAN_POINT('Ctrl Pts',(62.8075180003696,2.86860572942485,124.854134055001));
#220585=CARTESIAN_POINT('Ctrl Pts',(62.5290703765565,-3.4555426599142,125.174678574835));
#220586=CARTESIAN_POINT('Ctrl Pts',(62.2506227527437,-6.60421615743575,
130.66862586668));
#220587=CARTESIAN_POINT('Ctrl Pts',(61.9721751289308,-3.68393764016947,
136.287306763578));
#220588=CARTESIAN_POINT('Ctrl Pts',(61.6937275051179,2.62169959805353,136.867428009101));
#220589=CARTESIAN_POINT('Ctrl Pts',(61.415279881305,6.51812298281107,131.875886519111));
#220590=CARTESIAN_POINT('Ctrl Pts',(61.1368322574921,4.42470977437533,125.899665072552));
#220591=CARTESIAN_POINT('Ctrl Pts',(60.8583846336791,-1.73479555762186,
124.430619224162));
#220592=CARTESIAN_POINT('Ctrl Pts',(60.5799370098664,-6.30010852163892,
128.818730341733));
#220593=CARTESIAN_POINT('Ctrl Pts',(60.3014893860534,-5.07592953168175,
135.031538679362));
#220594=CARTESIAN_POINT('Ctrl Pts',(60.0230417622406,0.81278072494776,137.35977688733));
#220595=CARTESIAN_POINT('Ctrl Pts',(59.7445941384276,5.95458520189618,133.663907793273));
#220596=CARTESIAN_POINT('Ctrl Pts',(59.4661465146148,5.62441677596096,127.340254541386));
#220597=CARTESIAN_POINT('Ctrl Pts',(59.1876988908018,0.125684100952275,
124.199945542519));
#220598=CARTESIAN_POINT('Ctrl Pts',(58.909251266989,-5.48854612282181,127.128771354006));
#220599=CARTESIAN_POINT('Ctrl Pts',(58.6308036431761,-6.05907059010694,
133.435284136186));
#220600=CARTESIAN_POINT('Ctrl Pts',(58.3523560193632,-1.06160518713815,
137.324106732513));
#220601=CARTESIAN_POINT('Ctrl Pts',(58.0739083955504,4.91142352051418,135.221601156507));
#220602=CARTESIAN_POINT('Ctrl Pts',(57.7954607717374,6.37109394919177,129.059867319411));
#220603=CARTESIAN_POINT('Ctrl Pts',(57.5170131479246,1.97604028380464,124.501237600083));
#220604=CARTESIAN_POINT('Ctrl Pts',(57.2385655241116,-4.23489786746425,
125.734870009144));
#220605=CARTESIAN_POINT('Ctrl Pts',(56.9601179002987,-6.554171764796,131.627116628959));
#220606=CARTESIAN_POINT('Ctrl Pts',(56.6816702764859,-2.85048199937133,
136.76329066817));
#220607=CARTESIAN_POINT('Ctrl Pts',(56.4032226526729,3.47266146968847,136.423499100792));
#220608=CARTESIAN_POINT('Ctrl Pts',(56.1247750288601,6.60459869704857,130.919993777505));
#220609=CARTESIAN_POINT('Ctrl Pts',(55.8463274050471,3.66723237440476,125.310227229228));
#220610=CARTESIAN_POINT('Ctrl Pts',(55.5678797812343,-2.6401413460556,124.749300861495));
#220611=CARTESIAN_POINT('Ctrl Pts',(55.2894321574214,-6.5213541475661,129.752678603477));
#220612=CARTESIAN_POINT('Ctrl Pts',(55.0109845336085,-4.40976107332459,
135.722500738884));
#220613=CARTESIAN_POINT('Ctrl Pts',(54.7325369097956,1.75418699849736,137.172792367301));
#220614=CARTESIAN_POINT('Ctrl Pts',(54.4540892859827,6.30612291549916,132.770806332897));
#220615=CARTESIAN_POINT('Ctrl Pts',(54.1756416621698,5.06303994438864,126.561752752318));
#220616=CARTESIAN_POINT('Ctrl Pts',(53.897194038357,-0.832729392363195,
124.251448536985));
#220617=CARTESIAN_POINT('Ctrl Pts',(53.618746414544,-5.96326109862574,127.962950396153));
#220618=CARTESIAN_POINT('Ctrl Pts',(53.3402987907312,-5.61384717675129,
134.285569438194));
#220619=CARTESIAN_POINT('Ctrl Pts',(53.0618511669183,-0.105581951123662,
137.409127640582));
#220620=CARTESIAN_POINT('Ctrl Pts',(52.7834035431054,5.49970792962155,134.463227609627));
#220621=CARTESIAN_POINT('Ctrl Pts',(52.5049559192925,6.05103489871361,128.155007558556));
#220622=CARTESIAN_POINT('Ctrl Pts',(52.2265082954796,1.04175640537643,124.281413540623));
#220623=CARTESIAN_POINT('Ctrl Pts',(51.9480606716666,-4.9248453318719,126.402089222721));
#220624=CARTESIAN_POINT('Ctrl Pts',(51.6696130478539,-6.36575480119974,
132.568237253767));
#220625=CARTESIAN_POINT('Ctrl Pts',(51.3911654240409,-1.95684659263562,
137.113468826308));
#220626=CARTESIAN_POINT('Ctrl Pts',(51.112717800228,4.25030803728985,135.860938172086));
#220627=CARTESIAN_POINT('Ctrl Pts',(50.8342701764151,6.55163722003711,129.961659772806));
#220628=CARTESIAN_POINT('Ctrl Pts',(50.5558225526023,2.83233186284197,124.836782281636));
#220629=CARTESIAN_POINT('Ctrl Pts',(50.2773749287893,-3.48974810920128,
125.195817748775));
#220630=CARTESIAN_POINT('Ctrl Pts',(49.9989273049765,-6.60492005256131,
130.708830119782));
#220631=CARTESIAN_POINT('Ctrl Pts',(49.7204796811635,-3.65049313590031,
136.309630351328));
#220632=CARTESIAN_POINT('Ctrl Pts',(49.4420320573507,2.65855863614892,136.851356644924));
#220633=CARTESIAN_POINT('Ctrl Pts',(49.1635844335378,6.52452489938715,131.836189001557));
#220634=CARTESIAN_POINT('Ctrl Pts',(48.8851368097249,4.39477152084969,125.87282148092));
#220635=CARTESIAN_POINT('Ctrl Pts',(48.606689185912,-1.77356218882415,124.441297507781));
#220636=CARTESIAN_POINT('Ctrl Pts',(48.3282415620992,-6.31207889029818,
128.857117679619));
#220637=CARTESIAN_POINT('Ctrl Pts',(48.0497939382862,-5.05010345378512,
135.062358983324));
#220638=CARTESIAN_POINT('Ctrl Pts',(47.7713463144734,0.852670345487299,
137.354707803682));
#220639=CARTESIAN_POINT('Ctrl Pts',(47.4928986906604,5.97188175251911,133.627607562248));
#220640=CARTESIAN_POINT('Ctrl Pts',(47.2144510668476,5.60322557162828,127.306081301933));
#220641=CARTESIAN_POINT('Ctrl Pts',(46.9360034430346,0.0854788231980546,
124.199302832238));
#220642=CARTESIAN_POINT('Ctrl Pts',(46.6575558192218,-5.5108187878785,127.162249792247));
#220643=CARTESIAN_POINT('Ctrl Pts',(46.3791081954089,-6.04294315135938,
133.47211867372));
#220644=CARTESIAN_POINT('Ctrl Pts',(46.100660571596,-1.02189797292572,137.330448228811));
#220645=CARTESIAN_POINT('Ctrl Pts',(45.822212947783,4.93822152013526,135.191622086273));
#220646=CARTESIAN_POINT('Ctrl Pts',(45.5437653239702,6.36035668172477,129.02111698363));
#220647=CARTESIAN_POINT('Ctrl Pts',(45.2653177001572,1.9376347735074,124.489325664279));
#220648=CARTESIAN_POINT('Ctrl Pts',(44.9868700763445,-4.26567883284234,
125.76074296039));
#220649=CARTESIAN_POINT('Ctrl Pts',(44.7084224525315,-6.54904198180601,
131.666998489025));
#220650=CARTESIAN_POINT('Ctrl Pts',(44.4299748287186,-2.81415548797717,
136.780531955991));
#220651=CARTESIAN_POINT('Ctrl Pts',(44.1515272049057,3.50680242016433,136.402255915145));
#220652=CARTESIAN_POINT('Ctrl Pts',(43.8730795810928,6.60518022099696,130.879787568212));
#220653=CARTESIAN_POINT('Ctrl Pts',(43.59463195728,3.63372007972613,125.288005538446));
#220654=CARTESIAN_POINT('Ctrl Pts',(43.316184333467,-2.6769512977182,124.765484337463));
#220655=CARTESIAN_POINT('Ctrl Pts',(43.0377367096542,-6.52763520890084,
129.792395422388));
#220656=CARTESIAN_POINT('Ctrl Pts',(42.7592890858413,-4.37974125581177,
135.749253084432));
#220657=CARTESIAN_POINT('Ctrl Pts',(42.4808414620283,1.79292094911309,137.161996140853));
#220658=CARTESIAN_POINT('Ctrl Pts',(42.2023938382155,6.31797639086063,132.732382739134));
#220659=CARTESIAN_POINT('Ctrl Pts',(41.9239462144025,5.0371201797131,126.531011196811));
#220660=CARTESIAN_POINT('Ctrl Pts',(41.6454985905898,-0.872603399589798,
124.256639007436));
#220661=CARTESIAN_POINT('Ctrl Pts',(41.3670509667768,-5.98044708371573,
127.999303103786));
#220662=CARTESIAN_POINT('Ctrl Pts',(41.0886033429639,-5.592552058989,134.319678020622));
#220663=CARTESIAN_POINT('Ctrl Pts',(40.810155719151,-0.0653749034083074,
137.409647976851));
#220664=CARTESIAN_POINT('Ctrl Pts',(40.5317080953382,5.52187859466303,134.429681536124));
#220665=CARTESIAN_POINT('Ctrl Pts',(40.2532604715252,6.03479542300531,128.118222278014));
#220666=CARTESIAN_POINT('Ctrl Pts',(39.9748128477124,1.00203007375177,124.275192928799));
#220667=CARTESIAN_POINT('Ctrl Pts',(39.6963652238994,-4.95155196138904,
126.432149717987));
#220668=CARTESIAN_POINT('Ctrl Pts',(39.4179176000866,-6.35489964077443,
132.60695472951));
#220669=CARTESIAN_POINT('Ctrl Pts',(39.1394699762736,-1.91840500439501,
137.125263813774));
#220670=CARTESIAN_POINT('Ctrl Pts',(38.8610223524608,4.28101011172891,135.834971654011));
#220671=CARTESIAN_POINT('Ctrl Pts',(38.5825747286478,6.54638607414467,129.921793710766));
#220672=CARTESIAN_POINT('Ctrl Pts',(38.304127104835,2.79595304316033,124.819651639079));
#220673=CARTESIAN_POINT('Ctrl Pts',(38.0256794810221,-3.52382424458856,
125.217164749334));
#220674=CARTESIAN_POINT('Ctrl Pts',(37.7472318572093,-6.60537919994535,
130.749037912801));
#220675=CARTESIAN_POINT('Ctrl Pts',(37.4687842333963,-3.61691336126579,
136.331749939282));
#220676=CARTESIAN_POINT('Ctrl Pts',(37.1903366095834,2.69531916037638,136.835061207086));
#220677=CARTESIAN_POINT('Ctrl Pts',(36.9118889857706,6.53068504729366,131.796453249222));
#220678=CARTESIAN_POINT('Ctrl Pts',(36.6334413619576,4.36467041744916,125.846160629286));
#220679=CARTESIAN_POINT('Ctrl Pts',(36.3549937381448,-1.8122631000273,124.452211577043));
#220680=CARTESIAN_POINT('Ctrl Pts',(36.0765461143319,-6.32381536255287,
128.895577173308));
#220681=CARTESIAN_POINT('Ctrl Pts',(35.798098490519,-5.02409024244786,135.093021505591));
#220682=CARTESIAN_POINT('Ctrl Pts',(35.5196508667061,0.892528370013623,
137.34939599451));
#220683=CARTESIAN_POINT('Ctrl Pts',(35.2412032428932,5.98895701286753,133.591202714771));
#220684=CARTESIAN_POINT('Ctrl Pts',(34.9627556190803,5.58182673771145,127.272037692505));
#220685=CARTESIAN_POINT('Ctrl Pts',(34.6843079952674,0.0452703779943793,
124.198904874802));
#220686=CARTESIAN_POINT('Ctrl Pts',(34.4058603714545,-5.53288724751859,
127.195863190245));
#220687=CARTESIAN_POINT('Ctrl Pts',(34.1274127476417,-6.02659178913083,
133.508854356496));
#220688=CARTESIAN_POINT('Ctrl Pts',(33.8489651238287,-0.982152891908117,
137.336547898535));
#220689=CARTESIAN_POINT('Ctrl Pts',(33.5705175000158,4.96483653214189,135.161480444452));
#220690=CARTESIAN_POINT('Ctrl Pts',(33.292069876203,6.34938372890195,128.982432726597));
#220691=CARTESIAN_POINT('Ctrl Pts',(33.0136222523901,1.89915746344075,124.477647734417));
#220692=CARTESIAN_POINT('Ctrl Pts',(32.7351746285772,-4.29630173192265,
125.786802804744));
#220693=CARTESIAN_POINT('Ctrl Pts',(32.4567270047643,-6.543669521657,131.706848383727));
#220694=CARTESIAN_POINT('Ctrl Pts',(32.1782793809514,-2.77772469701646,
136.797551794587));
#220695=CARTESIAN_POINT('Ctrl Pts',(31.8998317571386,3.54081342478663,136.380805297429));
#220696=CARTESIAN_POINT('Ctrl Pts',(31.6213841333256,6.60551698756319,130.839578563946));
#220697=CARTESIAN_POINT('Ctrl Pts',(31.3429365095127,3.6000731362139,125.26598825823));
#220698=CARTESIAN_POINT('Ctrl Pts',(31.0644888856998,-2.71366205396602,
124.781891586214));
#220699=CARTESIAN_POINT('Ctrl Pts',(30.7860412618869,-6.53367438631237,
129.83214974004));
#220700=CARTESIAN_POINT('Ctrl Pts',(30.507593638074,-4.34955914537615,135.775822195171));
#220701=CARTESIAN_POINT('Ctrl Pts',(30.2291460142612,1.83158846238341,137.150964329883));
#220702=CARTESIAN_POINT('Ctrl Pts',(29.9506983904483,6.32959575128355,132.693887701803));
#220703=CARTESIAN_POINT('Ctrl Pts',(29.6722507666353,5.01101376269691,126.500427991838));
#220704=CARTESIAN_POINT('Ctrl Pts',(29.3938031428225,-0.912445072176531,
124.26207210612));
#220705=CARTESIAN_POINT('Ctrl Pts',(29.1153555190096,-5.99741146113971,
128.035759753857));
#220706=CARTESIAN_POINT('Ctrl Pts',(28.8369078951967,-5.57104970715349,
134.353656341672));
#220707=CARTESIAN_POINT('Ctrl Pts',(28.5584602713837,-0.0251654332018655,
137.409923551768));
#220708=CARTESIAN_POINT('Ctrl Pts',(28.280012647571,5.54384464446253,134.396001125022));
#220709=CARTESIAN_POINT('Ctrl Pts',(28.001565023758,6.0183323257333,128.081536533317));
#220710=CARTESIAN_POINT('Ctrl Pts',(27.7231173999451,0.962266611534229,
124.269214257685));
#220711=CARTESIAN_POINT('Ctrl Pts',(27.4446697761322,-4.97807510932732,
126.462372227135));
#220712=CARTESIAN_POINT('Ctrl Pts',(27.1662221523194,-6.34380899720599,
132.645605409466));
#220713=CARTESIAN_POINT('Ctrl Pts',(26.8877745285064,-1.87989232895117,
137.136824577849));
#220714=CARTESIAN_POINT('Ctrl Pts',(26.6093269046936,4.31155355176403,135.808818724794));
#220715=CARTESIAN_POINT('Ctrl Pts',(26.3308792808807,6.5408923495088,129.881960352566));
#220716=CARTESIAN_POINT('Ctrl Pts',(26.0524316570678,2.75947061841045,124.802742762115));
#220717=CARTESIAN_POINT('Ctrl Pts',(25.7739840332549,-3.55776980337282,
125.238718785491));
#220718=CARTESIAN_POINT('Ctrl Pts',(25.4955364094419,-6.60559358257403,
130.789247755823));
#220719=CARTESIAN_POINT('Ctrl Pts',(25.2170887856292,-3.58319956057628,
136.353664707793));
#220720=CARTESIAN_POINT('Ctrl Pts',(24.9386411618162,2.73197980856112,136.81854229942));
#220721=CARTESIAN_POINT('Ctrl Pts',(24.6601935380033,6.5366031982641,131.756680734531));
#220722=CARTESIAN_POINT('Ctrl Pts',(24.3817459141905,4.3344075795813,125.819683505575));
#220723=CARTESIAN_POINT('Ctrl Pts',(24.1032982903775,-1.85089685715453,
124.463361027524));
#220724=CARTESIAN_POINT('Ctrl Pts',(23.8248506665647,-6.33531750350378,
128.934107397669));
#220725=CARTESIAN_POINT('Ctrl Pts',(23.5464030427517,-4.99789086159903,
135.123525109951));
#220726=CARTESIAN_POINT('Ctrl Pts',(23.2679554189389,0.932353321572971,
137.343841656646));
#220727=CARTESIAN_POINT('Ctrl Pts',(22.9895077951259,6.00581035021119,133.554694599836));
#220728=CARTESIAN_POINT('Ctrl Pts',(22.7110601713131,5.56022106715229,127.238124974604));
#220729=CARTESIAN_POINT('Ctrl Pts',(22.4326125475002,0.00506025528043594,
124.198751684957));
#220730=CARTESIAN_POINT('Ctrl Pts',(22.1541649236873,-5.554750683987,127.229610302442));
#220731=CARTESIAN_POINT('Ctrl Pts',(21.8757172998744,-6.01001710932725,
133.545489823263));
#220732=CARTESIAN_POINT('Ctrl Pts',(21.5972696760615,-0.942371416853923,
137.342405515655));
#220733=CARTESIAN_POINT('Ctrl Pts',(21.3188220522486,4.99126757030501,135.131177347952));
#220734=CARTESIAN_POINT('Ctrl Pts',(21.0403744284357,6.33817549733007,128.943815981773));
#220735=CARTESIAN_POINT('Ctrl Pts',(20.7619268046228,1.86060977939589,124.466204243228));
#220736=CARTESIAN_POINT('Ctrl Pts',(20.48347918081,-4.32676542996233,125.813048576547));
#220737=CARTESIAN_POINT('Ctrl Pts',(20.205031556997,-6.5380545834274,131.746664836412));
#220738=CARTESIAN_POINT('Ctrl Pts',(19.9265839331841,-2.74119097644563,
136.814349553278));
#220739=CARTESIAN_POINT('Ctrl Pts',(19.6481363093713,3.57469322326559,136.359148042506));
#220740=CARTESIAN_POINT('Ctrl Pts',(19.3696886855584,6.60560898426828,130.799368254665));
#220741=CARTESIAN_POINT('Ctrl Pts',(19.0912410617455,3.56629279066743,125.244176204439));
#220742=CARTESIAN_POINT('Ctrl Pts',(18.8127934379326,-2.75027225446848,
124.798521999768));
#220743=CARTESIAN_POINT('Ctrl Pts',(18.5343458141197,-6.53947145601676,
129.871940083324));
#220744=CARTESIAN_POINT('Ctrl Pts',(18.2558981903068,-4.31921586042675,
135.802207086573));
#220745=CARTESIAN_POINT('Ctrl Pts',(17.9774505664939,1.87018810546999,137.139697343177));
#220746=CARTESIAN_POINT('Ctrl Pts',(17.6990029426811,6.34098056620813,132.65532264735));
#220747=CARTESIAN_POINT('Ctrl Pts',(17.4205553188681,4.98472166072295,126.470004270672));
#220748=CARTESIAN_POINT('Ctrl Pts',(17.1421076950552,-0.95225293377558,
124.26774763171));
#220749=CARTESIAN_POINT('Ctrl Pts',(16.8636600712423,-6.01415360227624,
128.072318995452));
#220750=CARTESIAN_POINT('Ctrl Pts',(16.5852124474295,-5.54934091802252,
134.387503142263));
#220751=CARTESIAN_POINT('Ctrl Pts',(16.3067648236166,0.0150449695187284,
137.409954355121));
#220752=CARTESIAN_POINT('Ctrl Pts',(16.0283171998036,5.56560526505998,134.362187624359));
#220753=CARTESIAN_POINT('Ctrl Pts',(15.7498695759908,6.00164621694371,128.044951683866));
#220754=CARTESIAN_POINT('Ctrl Pts',(15.4714219521779,0.922467492173741,
124.263477748823));
#220755=CARTESIAN_POINT('Ctrl Pts',(15.192974328365,-5.00441379286154,126.492755630261));
#220756=CARTESIAN_POINT('Ctrl Pts',(14.9145267045521,-6.33248328146239,
132.684187861418));
#220757=CARTESIAN_POINT('Ctrl Pts',(14.6360790807393,-1.84130999340576,
137.148150690142));
#220758=CARTESIAN_POINT('Ctrl Pts',(14.3576314569263,4.34193722559672,135.782480353541));
#220759=CARTESIAN_POINT('Ctrl Pts',(14.0791838331134,6.53515624970152,129.842161174248));
#220760=CARTESIAN_POINT('Ctrl Pts',(13.8007362093005,2.72288594046203,124.786056277307));
#220761=CARTESIAN_POINT('Ctrl Pts',(13.5222885854877,-3.59158352768866,
125.260479058552));
#220762=CARTESIAN_POINT('Ctrl Pts',(13.2438409616747,-6.60556319250329,
130.829458158858));
#220763=CARTESIAN_POINT('Ctrl Pts',(12.9653933378619,-3.54935298310934,
136.375373844801));
#220764=CARTESIAN_POINT('Ctrl Pts',(12.686945714049,2.76853922222938,136.801800534039));
#220765=CARTESIAN_POINT('Ctrl Pts',(12.4084980902361,6.5422791329992,131.716872931266));
#220766=CARTESIAN_POINT('Ctrl Pts',(12.1300504664232,4.30398412864651,125.793391090908));
#220767=CARTESIAN_POINT('Ctrl Pts',(11.8516028426103,-1.88946202861834,
124.474745446076));
#220768=CARTESIAN_POINT('Ctrl Pts',(11.5731552187974,-6.34658488693473,
128.972706924952));
#220769=CARTESIAN_POINT('Ctrl Pts',(11.2947075949845,-4.97150628206636,
135.153868666082));
#220770=CARTESIAN_POINT('Ctrl Pts',(11.0162599711716,0.972143724437105,
137.338044995907));
#220771=CARTESIAN_POINT('Ctrl Pts',(10.7378123473587,6.0224411400439,133.518084570262));
#220772=CARTESIAN_POINT('Ctrl Pts',(10.4593647235458,5.53840936055655,127.204344404875));
#220773=CARTESIAN_POINT('Ctrl Pts',(10.1809170997329,-0.0351500549433496,
124.198843268382));
#220774=CARTESIAN_POINT('Ctrl Pts',(9.90246947592002,-5.57640828712608,
127.263489878326));
#220775=CARTESIAN_POINT('Ctrl Pts',(9.62402185210712,-5.99321972612948,
133.582023716479));
#220776=CARTESIAN_POINT('Ctrl Pts',(9.34557422829421,-0.902555021880531,
137.348020863117));
#220777=CARTESIAN_POINT('Ctrl Pts',(9.06712660448133,5.01751365521256,135.100713919668));
#220778=CARTESIAN_POINT('Ctrl Pts',(8.78867898066847,6.32673240233446,128.905268180115));
#220779=CARTESIAN_POINT('Ctrl Pts',(8.51023135685555,1.82199314977141,124.454995614755));
#220780=CARTESIAN_POINT('Ctrl Pts',(8.23178373304265,-4.35706879811783,
125.839479303254));
#220781=CARTESIAN_POINT('Ctrl Pts',(7.9533361092298,-6.53219737518076,131.786446371669));
#220782=CARTESIAN_POINT('Ctrl Pts',(7.67488848541689,-2.70455568003535,
136.83092460962));
#220783=CARTESIAN_POINT('Ctrl Pts',(7.39644086160398,3.60844056017245,136.337284952891));
#220784=CARTESIAN_POINT('Ctrl Pts',(7.1179932377911,6.60545620770325,130.759158130379));
#220785=CARTESIAN_POINT('Ctrl Pts',(6.83954561397822,3.53238029483008,125.222570185327));
#220786=CARTESIAN_POINT('Ctrl Pts',(6.5610979901653,-2.78678054262086,124.815374961881));
#220787=CARTESIAN_POINT('Ctrl Pts',(6.28265036635242,-6.54502620320144,
129.911764977794));
#220788=CARTESIAN_POINT('Ctrl Pts',(6.00420274253956,-4.28871252534551,
135.828406780936));
#220789=CARTESIAN_POINT('Ctrl Pts',(5.72575511872663,1.90871844804856,137.128195598241));
#220790=CARTESIAN_POINT('Ctrl Pts',(5.44730749491374,6.35213041376593,132.616689004818));
#220791=CARTESIAN_POINT('Ctrl Pts',(5.16885987110085,4.95824484805471,126.439741160674));
#220792=CARTESIAN_POINT('Ctrl Pts',(4.89041224728798,-0.992025509291961,
124.273665373899));
#220793=CARTESIAN_POINT('Ctrl Pts',(4.61196462347505,-6.03067288673954,
128.108979473854));
#220794=CARTESIAN_POINT('Ctrl Pts',(4.33351699966218,-5.52742649602286,
134.421217168191));
#220795=CARTESIAN_POINT('Ctrl Pts',(4.05506937584931,0.0552548147426717,
137.409740385768));
#220796=CARTESIAN_POINT('Ctrl Pts',(3.77662175203639,5.58715965010757,134.328242287108));
#220797=CARTESIAN_POINT('Ctrl Pts',(3.49817412822347,5.98473771494644,128.008469085329));
#220798=CARTESIAN_POINT('Ctrl Pts',(3.21972650441063,0.882634190440881,
124.25798361478));
#220799=CARTESIAN_POINT('Ctrl Pts',(2.94127888059773,-5.03056703600248,
126.523298801495));
#220800=CARTESIAN_POINT('Ctrl Pts',(2.66283125678483,-6.32092291322184,
132.722700655682));
#220801=CARTESIAN_POINT('Ctrl Pts',(2.38438363297192,-1.80265942744139,
137.159241730961));
#220802=CARTESIAN_POINT('Ctrl Pts',(2.10593600915906,4.37216000734877,135.755957516231));
#220803=CARTESIAN_POINT('Ctrl Pts',(1.82748838534615,6.529177987276,129.802397650584));
#220804=CARTESIAN_POINT('Ctrl Pts',(1.54904076153325,2.68620036497402,124.769592802981));
#220805=CARTESIAN_POINT('Ctrl Pts',(1.27059313772038,-3.62526416455594,
125.282444762183));
#220806=CARTESIAN_POINT('Ctrl Pts',(0.992145513907496,-6.60528803085927,
130.869667631896));
#220807=CARTESIAN_POINT('Ctrl Pts',(0.713697890094564,-3.51537488306232,
136.396876545864));
#220808=CARTESIAN_POINT('Ctrl Pts',(0.435250266281723,2.80499604665836,
136.784836531317));
#220809=CARTESIAN_POINT('Ctrl Pts',(0.156802642468823,6.54771264117505,
131.677031314524));
#220810=CARTESIAN_POINT('Ctrl Pts',(-0.121644981344083,4.27340119199728,
125.767284359559));
#220811=CARTESIAN_POINT('Ctrl Pts',(-0.400092605156985,-1.92795718537184,
124.486364410847));
#220812=CARTESIAN_POINT('Ctrl Pts',(-0.678540228969845,-6.35761709532873,
129.011374324836));
#220813=CARTESIAN_POINT('Ctrl Pts',(-0.956987852782752,-4.94493748154019,
135.184051049593));
#220814=CARTESIAN_POINT('Ctrl Pts',(-1.23543547659566,1.01189810415772,
137.332006227089));
#220815=CARTESIAN_POINT('Ctrl Pts',(-1.51388310040852,6.03884876610542,
133.48137398265));
#220816=CARTESIAN_POINT('Ctrl Pts',(-1.79233072422142,5.51639242616521,
127.170697235071));
#220817=CARTESIAN_POINT('Ctrl Pts',(-2.07077834803434,-0.0753590626689394,
124.19917962168));
#220818=CARTESIAN_POINT('Ctrl Pts',(-2.34922597184723,-5.59785925440532,
127.297500662476));
#220819=CARTESIAN_POINT('Ctrl Pts',(-2.6276735956601,-5.97620026197078,
133.618454682368));
#220820=CARTESIAN_POINT('Ctrl Pts',(-2.906121219473,-0.862705182398668,
137.353393732843));
#220821=CARTESIAN_POINT('Ctrl Pts',(-3.18456884328591,5.04357381430661,
135.070091288433));
#220822=CARTESIAN_POINT('Ctrl Pts',(-3.46301646709877,6.31505486794284,
128.866790750024));
#220823=CARTESIAN_POINT('Ctrl Pts',(-3.74146409091167,1.78330900552073,
124.444022264336));
#220824=CARTESIAN_POINT('Ctrl Pts',(-4.01991171472458,-4.38721071348669,
125.866094005463));
#220825=CARTESIAN_POINT('Ctrl Pts',(-4.29835933853748,-6.52609811395827,
131.826191515377));
#220826=CARTESIAN_POINT('Ctrl Pts',(-4.57680696235032,-2.66782016531947,
136.847276349416));
#220827=CARTESIAN_POINT('Ctrl Pts',(-4.85525458616324,3.64205418498746,
136.31521683873));
#220828=CARTESIAN_POINT('Ctrl Pts',(-5.13370220997616,6.60505866352928,
130.718949681087));
#220829=CARTESIAN_POINT('Ctrl Pts',(-5.41214983378902,3.49833690534187,
125.201171001511));
#220830=CARTESIAN_POINT('Ctrl Pts',(-5.69059745760191,-2.82318556559566,
124.832449848059));
#220831=CARTESIAN_POINT('Ctrl Pts',(-5.96904508141481,-6.55033842203324,
129.951622947723));
#220832=CARTESIAN_POINT('Ctrl Pts',(-6.24749270522772,-4.2580502704442,
135.854420307421));
#220833=CARTESIAN_POINT('Ctrl Pts',(-6.52594032904057,1.9471780623631,137.116459521273));
#220834=CARTESIAN_POINT('Ctrl Pts',(-6.80438795285348,6.36304488079526,
132.577988205793));
#220835=CARTESIAN_POINT('Ctrl Pts',(-7.0828355766664,4.93158430580029,126.409639783256));
#220836=CARTESIAN_POINT('Ctrl Pts',(-7.36128320047925,-1.03176132493798,
124.279825113401));
#220837=CARTESIAN_POINT('Ctrl Pts',(-7.63973082429214,-6.04696870240127,
128.145739830595));
#220838=CARTESIAN_POINT('Ctrl Pts',(-7.91817844810507,-5.50530725320171,
134.454797170168));
#220839=CARTESIAN_POINT('Ctrl Pts',(-8.19662607191793,0.09546261247915,
137.40928165164));
#220840=CARTESIAN_POINT('Ctrl Pts',(-8.47507369573082,5.60850700089942,
134.294166371127));
#220841=CARTESIAN_POINT('Ctrl Pts',(-8.75352131954372,5.96760744629241,
127.972090089581));
#220842=CARTESIAN_POINT('Ctrl Pts',(-9.03196894335663,0.842768182373745,
124.252732059145));
#220843=CARTESIAN_POINT('Ctrl Pts',(-9.31041656716948,-5.05653386963193,
126.554000609049));
#220844=CARTESIAN_POINT('Ctrl Pts',(-9.5888641909824,-6.30912832085822,
132.76114236515));
#220845=CARTESIAN_POINT('Ctrl Pts',(-9.86731181479532,-1.76394206326903,
137.170097289323));
#220846=CARTESIAN_POINT('Ctrl Pts',(-10.1457594386081,4.40222077710389,
135.729251195677));
#220847=CARTESIAN_POINT('Ctrl Pts',(-10.424207062421,6.52295778375913,129.762671255026));
#220848=CARTESIAN_POINT('Ctrl Pts',(-10.7026546862339,2.64941525134336,
124.753352949195));
#220849=CARTESIAN_POINT('Ctrl Pts',(-10.9811023100469,-3.65881046592654,
125.304615082438));
#220850=CARTESIAN_POINT('Ctrl Pts',(-11.2595499338597,-6.60476810783814,
130.909874684957));
#220851=CARTESIAN_POINT('Ctrl Pts',(-11.5379975576726,-3.48126651950624,
136.418172014193));
#220852=CARTESIAN_POINT('Ctrl Pts',(-11.8164451814855,2.84134893092756,
136.767650919861));
#220853=CARTESIAN_POINT('Ctrl Pts',(-12.0948928052984,6.5529035214511,131.637157360647));
#220854=CARTESIAN_POINT('Ctrl Pts',(-12.3733404291112,4.2426599028951,125.741364278924));
#220855=CARTESIAN_POINT('Ctrl Pts',(-12.6517880529242,-1.96638090096281,
124.498217491291));
#220856=CARTESIAN_POINT('Ctrl Pts',(-12.9302356767371,-6.36841371988325,
129.050108164486));
#220857=CARTESIAN_POINT('Ctrl Pts',(-13.2086833005499,-4.91818544453708,
135.214071142064));
#220858=CARTESIAN_POINT('Ctrl Pts',(-13.4871309243628,1.05161498762227,
137.325725573964));
#220859=CARTESIAN_POINT('Ctrl Pts',(-13.7655785481758,6.05503262040511,
133.444564197323));
#220860=CARTESIAN_POINT('Ctrl Pts',(-14.0440261719886,5.49417107982388,
127.137184712));
#220861=CARTESIAN_POINT('Ctrl Pts',(-14.3224737958015,-0.115565277936756,
124.199760732389));
#220862=CARTESIAN_POINT('Ctrl Pts',(-14.6009214196144,-5.61910279095105,
127.331641394614));
#220863=CARTESIAN_POINT('Ctrl Pts',(-14.8793690434273,-5.95895934751375,
133.654781370965));
#220864=CARTESIAN_POINT('Ctrl Pts',(-15.1578166672402,-0.822823375059262,
137.358523925738));
#220865=CARTESIAN_POINT('Ctrl Pts',(-15.4362642910531,5.06944708191823,
135.039310588977));
#220866=CARTESIAN_POINT('Ctrl Pts',(-15.714711914866,6.3031433268707,128.828385117298));
#220867=CARTESIAN_POINT('Ctrl Pts',(-15.9931595386788,1.74455878009922,
124.433284598595));
#220868=CARTESIAN_POINT('Ctrl Pts',(-16.2716071624918,-4.41719005914895,
125.892891696959));
#220869=CARTESIAN_POINT('Ctrl Pts',(-16.5500547863046,-6.51975702577033,
131.865898794765));
#220870=CARTESIAN_POINT('Ctrl Pts',(-16.8285024101176,-2.63098579354628,
136.863404166748));
#220871=CARTESIAN_POINT('Ctrl Pts',(-17.1069500339304,3.67553285214529,
136.292944517765));
#220872=CARTESIAN_POINT('Ctrl Pts',(-17.3853976577434,6.60441636647752,
130.678744396729));
#220873=CARTESIAN_POINT('Ctrl Pts',(-17.6638452815562,3.46416388369313,
125.179979445948));
#220874=CARTESIAN_POINT('Ctrl Pts',(-17.9422929053691,-2.8594859743911,
124.849746025587));
#220875=CARTESIAN_POINT('Ctrl Pts',(-18.220740529182,-6.55540791566593,
129.991512516161));
#220876=CARTESIAN_POINT('Ctrl Pts',(-18.4991881529949,-4.22723023192423,
135.880246702087));
#220877=CARTESIAN_POINT('Ctrl Pts',(-18.7776357768078,1.98556552327847,
137.104489547159));
#220878=CARTESIAN_POINT('Ctrl Pts',(-19.0560834006207,6.37372356285652,
132.539221684343));
#220879=CARTESIAN_POINT('Ctrl Pts',(-19.3345310244336,4.90474102187576,
126.379701253833));
#220880=CARTESIAN_POINT('Ctrl Pts',(-19.6129786482465,-1.07145890828896,
124.286226621967));
#220881=CARTESIAN_POINT('Ctrl Pts',(-19.8914262720594,-6.06304044541393,
128.182598703507));
#220882=CARTESIAN_POINT('Ctrl Pts',(-20.1698738958722,-5.48298400919569,
134.488241903877));
#220883=CARTESIAN_POINT('Ctrl Pts',(-20.4483215196851,0.135666872813404,
137.408578169733));
#220884=CARTESIAN_POINT('Ctrl Pts',(-20.7267691434981,5.62964652640204,
134.25996113911));
#220885=CARTESIAN_POINT('Ctrl Pts',(-21.0052167673109,5.95025604574973,
127.935816044659));
#220886=CARTESIAN_POINT('Ctrl Pts',(-21.2836643911238,0.802870945221437,
124.247723276515));
#220887=CARTESIAN_POINT('Ctrl Pts',(-21.5621120149367,-5.08231333153929,
126.584859915257));
#220888=CARTESIAN_POINT('Ctrl Pts',(-21.8405596387496,-6.29709994142449,
132.79951156535));
#220889=CARTESIAN_POINT('Ctrl Pts',(-22.1190072625625,-1.725159335575,137.180716962973));
#220890=CARTESIAN_POINT('Ctrl Pts',(-22.3974548863754,4.43211842094896,
135.702362381491));
#220891=CARTESIAN_POINT('Ctrl Pts',(-22.6759025101882,6.51649586964294,
129.722983459651));
#220892=CARTESIAN_POINT('Ctrl Pts',(-22.9543501340012,2.61253196265622,
124.737337317723));
#220893=CARTESIAN_POINT('Ctrl Pts',(-23.232797757814,-3.6922211887298,125.326989197785));
#220894=CARTESIAN_POINT('Ctrl Pts',(-23.511245381627,-6.60400344270576,
130.950077828156));
#220895=CARTESIAN_POINT('Ctrl Pts',(-23.7896930054398,-3.4470291563393,
136.439259460675));
#220896=CARTESIAN_POINT('Ctrl Pts',(-24.0681406292527,2.87759652796706,
136.75024433649));
#220897=CARTESIAN_POINT('Ctrl Pts',(-24.3465882530656,6.55785158147733,
131.597252547181));
#220898=CARTESIAN_POINT('Ctrl Pts',(-24.6250358768785,4.21176140046998,
125.715631809479));
#220899=CARTESIAN_POINT('Ctrl Pts',(-24.9034835006914,-2.00473175158637,
124.510304248187));
#220900=CARTESIAN_POINT('Ctrl Pts',(-25.1819311245043,-6.3789743605254,
129.088907008606));
#220901=CARTESIAN_POINT('Ctrl Pts',(-25.4603787483172,-4.89125116236366,
135.24392783109));
#220902=CARTESIAN_POINT('Ctrl Pts',(-25.73882637213,1.09129290310671,137.319203269261));
#220903=CARTESIAN_POINT('Ctrl Pts',(-26.017273995943,6.07099210324431,133.407656578282));
#220904=CARTESIAN_POINT('Ctrl Pts',(-26.2957216197559,5.47174614495268,
127.103808077481));
#220905=CARTESIAN_POINT('Ctrl Pts',(-26.5741692435687,-0.155767210890682,
124.200586578976));
#220906=CARTESIAN_POINT('Ctrl Pts',(-26.8526168673816,-5.64013810957666,
127.365910809639));
#220907=CARTESIAN_POINT('Ctrl Pts',(-27.1310644911945,-5.94149762162655,
133.691002436174));
#220908=CARTESIAN_POINT('Ctrl Pts',(-27.4095121150075,-0.782911077696857,
137.363411251701));
#220909=CARTESIAN_POINT('Ctrl Pts',(-27.6879597388203,5.09513249930392,
135.008372961895));
#220910=CARTESIAN_POINT('Ctrl Pts',(-27.9664073626332,6.29099822050462,
128.79005270507));
#220911=CARTESIAN_POINT('Ctrl Pts',(-28.2448549864461,1.70574390941038,
124.422783015417));
#220912=CARTESIAN_POINT('Ctrl Pts',(-28.523302610259,-4.44700572420938,
125.919871384741));
#220913=CARTESIAN_POINT('Ctrl Pts',(-28.8017502340719,-6.51317434558802,
131.905566738465));
#220914=CARTESIAN_POINT('Ctrl Pts',(-29.0801978578848,-2.59405392962697,
136.879307463993));
#220915=CARTESIAN_POINT('Ctrl Pts',(-29.3586454816977,3.7088753210816,136.270468815306));
#220916=CARTESIAN_POINT('Ctrl Pts',(-29.6370931055106,6.6035293403484,130.638543767126));
#220917=CARTESIAN_POINT('Ctrl Pts',(-29.9155407293234,3.42986249617799,
125.158996303897));
#220918=CARTESIAN_POINT('Ctrl Pts',(-30.1939883531365,-2.89568042388203,
124.86726285355));
#220919=CARTESIAN_POINT('Ctrl Pts',(-30.4724359769491,-6.56023449624756,
130.031432204983));
#220920=CARTESIAN_POINT('Ctrl Pts',(-30.7508836007622,-4.19625355183344,
135.905885007927));
#220921=CARTESIAN_POINT('Ctrl Pts',(-31.029331224575,2.02387940833292,137.092286119451));
#220922=CARTESIAN_POINT('Ctrl Pts',(-31.3077788483879,6.38416606424714,
132.50039087698));
#220923=CARTESIAN_POINT('Ctrl Pts',(-31.5862264722008,4.8777159909692,126.349926681791));
#220924=CARTESIAN_POINT('Ctrl Pts',(-31.8646740960137,-1.11111678833609,
124.292869662384));
#220925=CARTESIAN_POINT('Ctrl Pts',(-32.1431217198266,-6.07888752023319,
128.219554726771));
#220926=CARTESIAN_POINT('Ctrl Pts',(-32.4215693436394,-5.46045759120085,
134.52155013001));
#220927=CARTESIAN_POINT('Ctrl Pts',(-32.7000169674524,0.175866105961793,
137.407629966116));
#220928=CARTESIAN_POINT('Ctrl Pts',(-32.9784645912652,5.65057744328232,
134.225627858545));
#220929=CARTESIAN_POINT('Ctrl Pts',(-33.2569122150782,5.93268415628106,
127.89964829471));
#220930=CARTESIAN_POINT('Ctrl Pts',(-33.535359838891,0.762943957391,124.242957452493));
#220931=CARTESIAN_POINT('Ctrl Pts',(-33.813807462704,-5.10790446645711,
126.615875576613));
#220932=CARTESIAN_POINT('Ctrl Pts',(-34.0922550865168,-6.28483822063666,
132.837806834499));
#220933=CARTESIAN_POINT('Ctrl Pts',(-34.3707027103298,-1.68631268146717,
137.191100358392));
#220934=CARTESIAN_POINT('Ctrl Pts',(-34.6491503341426,4.46185183101625,
135.675292070049));
#220935=CARTESIAN_POINT('Ctrl Pts',(-34.9275979579556,6.5097924843757,129.683335735103));
#220936=CARTESIAN_POINT('Ctrl Pts',(-35.2060455817684,2.57555186563646,
124.721546502031));
#220937=CARTESIAN_POINT('Ctrl Pts',(-35.4844932055813,-3.72549509491909,
125.349566279145));
#220938=CARTESIAN_POINT('Ctrl Pts',(-35.7629408293942,-6.60299406379731,
130.990275571749));
#220939=CARTESIAN_POINT('Ctrl Pts',(-36.0413884532071,-3.41266406223907,
136.460138103909));
#220940=CARTESIAN_POINT('Ctrl Pts',(-36.3198360770199,2.91373749460914,
136.73261742621));
#220941=CARTESIAN_POINT('Ctrl Pts',(-36.5982837008328,6.56255663790157,
131.557318352812));
#220942=CARTESIAN_POINT('Ctrl Pts',(-36.8767313246458,4.18070682967726,
125.690087904753));
#220943=CARTESIAN_POINT('Ctrl Pts',(-37.1551789484586,-2.04300831613737,
124.522624233657));
#220944=CARTESIAN_POINT('Ctrl Pts',(-37.4336265722715,-6.38929862592666,
129.12776941949));
#220945=CARTESIAN_POINT('Ctrl Pts',(-37.7120741960844,-4.86413563307991,
135.273620010322));
#220946=CARTESIAN_POINT('Ctrl Pts',(-37.9905218198973,1.13093038033133,
137.312439554669));
#220947=CARTESIAN_POINT('Ctrl Pts',(-38.2689694437102,6.0867266232385,133.370652493151));
#220948=CARTESIAN_POINT('Ctrl Pts',(-38.5474170675231,5.44911845251588,
127.070568568297));
#220949=CARTESIAN_POINT('Ctrl Pts',(-38.825864691336,-0.195963371833029,
124.201657130839));
#220950=CARTESIAN_POINT('Ctrl Pts',(-39.1043123151489,-5.66096443081045,
127.400307637685));
#220951=CARTESIAN_POINT('Ctrl Pts',(-39.3827599389617,-5.92381573136,133.727116535809));
#220952=CARTESIAN_POINT('Ctrl Pts',(-39.6612075627747,-0.742969769276543,
137.368055529631));
#220953=CARTESIAN_POINT('Ctrl Pts',(-39.9396551865875,5.12062911468111,
134.977279553588));
#220954=CARTESIAN_POINT('Ctrl Pts',(-40.2181028104005,6.27861999888597,
128.751794933764));
#220955=CARTESIAN_POINT('Ctrl Pts',(-40.4965504342133,1.66686583175366,
124.412517903944));
#220956=CARTESIAN_POINT('Ctrl Pts',(-40.7749980580263,-4.47665660383728,
125.947032069068));
#220957=CARTESIAN_POINT('Ctrl Pts',(-41.0534456818391,-6.5063503173351,
131.945193876568));
#220958=CARTESIAN_POINT('Ctrl Pts',(-41.3318933056519,-2.55702594208532,
136.894985651848));
#220959=CARTESIAN_POINT('Ctrl Pts',(-41.6103409294649,3.74208035627896,
136.247790564197));
#220960=CARTESIAN_POINT('Ctrl Pts',(-41.8887885532778,6.60239761801125,
130.598349281928));
#220961=CARTESIAN_POINT('Ctrl Pts',(-42.1672361770906,3.39543401384647,
125.138222352896));
#220962=CARTESIAN_POINT('Ctrl Pts',(-42.4456838009036,-2.93176757287012,
124.884999682853));
#220963=CARTESIAN_POINT('Ctrl Pts',(-42.7241314247165,-6.56481798492739,
130.071380534953));
#220964=CARTESIAN_POINT('Ctrl Pts',(-43.0025790485293,-4.16512137802412,
135.931334274905));
#220965=CARTESIAN_POINT('Ctrl Pts',(-43.2810266723423,2.06211829779186,
137.079849690351));
#220966=CARTESIAN_POINT('Ctrl Pts',(-43.5594742961552,6.39437199801655,
132.461497222591));
#220967=CARTESIAN_POINT('Ctrl Pts',(-43.837921919968,4.85051021450257,126.320317170437));
#220968=CARTESIAN_POINT('Ctrl Pts',(-44.116369543781,-1.150733495542,124.299753988494));
#220969=CARTESIAN_POINT('Ctrl Pts',(-44.3948171675938,-6.09450933963988,
128.256606530968));
#220970=CARTESIAN_POINT('Ctrl Pts',(-44.6732647914067,-5.43772883394191,
134.554720614319));
#220971=CARTESIAN_POINT('Ctrl Pts',(-44.9517124152196,0.216058822326645,
137.406437075925));
#220972=CARTESIAN_POINT('Ctrl Pts',(-45.2301600390324,5.67129897593744,
134.191167801664));
#220973=CARTESIAN_POINT('Ctrl Pts',(-45.5086076628454,5.91489242901924,
127.863588179946));
#220974=CARTESIAN_POINT('Ctrl Pts',(-45.7870552866582,0.722988698391639,
124.238434763679));
#220975=CARTESIAN_POINT('Ctrl Pts',(-46.0655029104712,-5.13330632609627,
126.647046443824));
#220976=CARTESIAN_POINT('Ctrl Pts',(-46.343950534284,-6.27234361285742,
132.876026753548));
#220977=CARTESIAN_POINT('Ctrl Pts',(-46.622398158097,-1.64740354042306,
137.201247090823));
#220978=CARTESIAN_POINT('Ctrl Pts',(-46.9008457819097,4.49141990552312,
135.64804126445));
#220979=CARTESIAN_POINT('Ctrl Pts',(-47.1792934057228,6.50284787635396,
129.643729550545));
#220980=CARTESIAN_POINT('Ctrl Pts',(-47.4577410295356,2.53847633059532,
124.705981087252));
#220981=CARTESIAN_POINT('Ctrl Pts',(-47.7361886533485,-3.75863095151733,
125.372345489915));
#220982=CARTESIAN_POINT('Ctrl Pts',(-48.0146362771614,-6.60174000851572,
131.030466426196));
#220983=CARTESIAN_POINT('Ctrl Pts',(-48.2930839009743,-3.37817251061699,
136.480807170229));
#220984=CARTESIAN_POINT('Ctrl Pts',(-48.5715315247872,2.94977049163681,
136.714770842195));
#220985=CARTESIAN_POINT('Ctrl Pts',(-48.8499791486,6.56701851637621,131.517356257317));
#220986=CARTESIAN_POINT('Ctrl Pts',(-49.128426772413,4.14949734125552,125.664733511282));
#220987=CARTESIAN_POINT('Ctrl Pts',(-49.4068743962258,-2.08120917626415,
124.535176991179));
#220988=CARTESIAN_POINT('Ctrl Pts',(-49.6853220200388,-6.39938613351776,
129.166693957078));
#220989=CARTESIAN_POINT('Ctrl Pts',(-49.9637696438516,-4.83683986146123,
135.303146579501));
#220990=CARTESIAN_POINT('Ctrl Pts',(-50.2422172676646,1.17052595051479,
137.305434680818));
#220991=CARTESIAN_POINT('Ctrl Pts',(-50.5206648914774,6.10223559733929,
133.333553313131));
#220992=CARTESIAN_POINT('Ctrl Pts',(-50.7991125152903,5.42628884099088,
127.03746741615));
#220993=CARTESIAN_POINT('Ctrl Pts',(-51.0775601391032,-0.236152271280866,
124.202972348307));
#220994=CARTESIAN_POINT('Ctrl Pts',(-51.3560077629162,-5.68158098292544,
127.434830604167));
#220995=CARTESIAN_POINT('Ctrl Pts',(-51.634455386729,-5.90591433192304,
133.763122331648));
#220996=CARTESIAN_POINT('Ctrl Pts',(-51.9129030105419,-0.703000929838195,
137.372456587432));
#220997=CARTESIAN_POINT('Ctrl Pts',(-52.1913506343548,5.14593598326309,
134.946031516236));
#220998=CARTESIAN_POINT('Ctrl Pts',(-52.4697982581677,6.26600912069438,
128.713613221033));
#220999=CARTESIAN_POINT('Ctrl Pts',(-52.7482458819806,1.62792598777083,
124.402489644555));
#221000=CARTESIAN_POINT('Ctrl Pts',(-53.0266935057934,-4.50614159930848,
125.97437274349));
#221001=CARTESIAN_POINT('Ctrl Pts',(-53.3051411296064,-6.49928519387843,
131.984778740675));
#221002=CARTESIAN_POINT('Ctrl Pts',(-53.5835887534191,-2.51990320300721,
136.910438149353));
#221003=CARTESIAN_POINT('Ctrl Pts',(-53.8620363772322,3.7751467273123,136.22491060479));
#221004=CARTESIAN_POINT('Ctrl Pts',(-54.140484001045,6.60102124140245,130.558162430556));
#221005=CARTESIAN_POINT('Ctrl Pts',(-54.418931624858,3.36087971245889,125.117658362733));
#221006=CARTESIAN_POINT('Ctrl Pts',(-54.6973792486707,-2.96774608413265,
124.902955856252));
#221007=CARTESIAN_POINT('Ctrl Pts',(-54.9758268724838,-6.56915821186243,
130.111356025769));
#221008=CARTESIAN_POINT('Ctrl Pts',(-55.2542744962966,-4.13383486411065,
135.956593559989));
#221009=CARTESIAN_POINT('Ctrl Pts',(-55.5327221201095,2.10028077469877,
137.067180720695));
#221010=CARTESIAN_POINT('Ctrl Pts',(-55.8111697439224,6.40434098598004,
132.422542162396));
#221011=CARTESIAN_POINT('Ctrl Pts',(-56.0896173677353,4.82312470059616,
126.29087381696));
#221012=CARTESIAN_POINT('Ctrl Pts',(-56.3680649915482,-1.19030756189505,
124.306879345194));
#221013=CARTESIAN_POINT('Ctrl Pts',(-56.646512615361,-6.10990532476174,
128.293752743129));
#221014=CARTESIAN_POINT('Ctrl Pts',(-56.924960239174,-5.41479857964128,
134.587752127659));
#221015=CARTESIAN_POINT('Ctrl Pts',(-57.2034078629868,0.256243532552689,
137.404999543363));
#221016=CARTESIAN_POINT('Ctrl Pts',(-57.4818554867998,5.69181035652338,
134.156582245398));
#221017=CARTESIAN_POINT('Ctrl Pts',(-57.7603031106126,5.89688152324325,
127.827637036585));
#221018=CARTESIAN_POINT('Ctrl Pts',(-58.0387507344255,0.683006648780185,
124.234155377662));
#221019=CARTESIAN_POINT('Ctrl Pts',(-58.3171983582384,-5.15851796918197,
126.67837136184));
#221020=CARTESIAN_POINT('Ctrl Pts',(-58.5956459820513,-6.25961658107885,
132.91416990625));
#221021=CARTESIAN_POINT('Ctrl Pts',(-58.8740936058642,-1.60843335423465,
137.211156784272));
#221022=CARTESIAN_POINT('Ctrl Pts',(-59.1525412296771,4.52082154881365,
135.620610974484));
#221023=CARTESIAN_POINT('Ctrl Pts',(-59.4309888534899,6.49566230291273,
129.604166373598));
#221024=CARTESIAN_POINT('Ctrl Pts',(-59.7094364773029,2.50130673138007,
124.69064165017));
#221025=CARTESIAN_POINT('Ctrl Pts',(-59.9878841011157,-3.79162753066369,
125.395325986002));
#221026=CARTESIAN_POINT('Ctrl Pts',(-60.2663317249287,-6.60024132333016,
131.070648902209));
#221027=CARTESIAN_POINT('Ctrl Pts',(-60.5447793487415,-3.34355577957023,
136.501265893734));
#221028=CARTESIAN_POINT('Ctrl Pts',(-60.8232269725544,2.98569418383416,
136.696705245755));
#221029=CARTESIAN_POINT('Ctrl Pts',(-61.1016745963673,6.57123705156454,
131.477367741508));
#221030=CARTESIAN_POINT('Ctrl Pts',(-61.3801222201802,4.11813409168408,
125.639569568584));
#221031=CARTESIAN_POINT('Ctrl Pts',(-61.6585698439931,-2.11933291641938,
124.547962055604));
#221032=CARTESIAN_POINT('Ctrl Pts',(-61.937017467806,-6.40923650950231,
129.205679179005));
#221033=CARTESIAN_POINT('Ctrl Pts',(-62.2154650916189,-4.80936485896274,
135.332506444514));
#221034=CARTESIAN_POINT('Ctrl Pts',(-62.4939127154318,1.21007814642843,
137.298188907278));
#221035=CARTESIAN_POINT('Ctrl Pts',(-62.7723603392447,6.1175184508558,133.296360412945));
#221036=CARTESIAN_POINT('Ctrl Pts',(-63.0508079630576,5.40325815633759,
127.004505847616));
#221037=CARTESIAN_POINT('Ctrl Pts',(-63.3292555868704,-0.276332420019459,
124.204532182646));
#221038=CARTESIAN_POINT('Ctrl Pts',(-63.6077032106833,-5.70198700196771,
127.469478429822));
#221039=CARTESIAN_POINT('Ctrl Pts',(-63.8861508344962,-5.8877940866586,
133.799018489484));
#221040=CARTESIAN_POINT('Ctrl Pts',(-64.1645984583092,-0.663006040441876,
137.376614262022));
#221041=CARTESIAN_POINT('Ctrl Pts',(-64.4430460821219,5.17105216729505,
134.914630007745));
#221042=CARTESIAN_POINT('Ctrl Pts',(-64.721493705935,6.25316605323042,128.675508981716));
#221043=CARTESIAN_POINT('Ctrl Pts',(-64.9999413297477,1.58892582039159,
124.392698608848));
#221044=CARTESIAN_POINT('Ctrl Pts',(-65.2783889535607,-4.53545961804555,
126.00189239489));
#221045=CARTESIAN_POINT('Ctrl Pts',(-65.5568365773735,-6.49197923701883,
132.024319863954));
#221046=CARTESIAN_POINT('Ctrl Pts',(-65.8352842011867,-2.48268708798906,
136.92566438391));
#221047=CARTESIAN_POINT('Ctrl Pts',(-66.1137318249993,3.80807320889562,
136.201829784909));
#221048=CARTESIAN_POINT('Ctrl Pts',(-66.3921794488124,6.59940026152389,
130.517984702147));
#221049=CARTESIAN_POINT('Ctrl Pts',(-66.6706270726251,3.3262008724376,125.097305095413));
#221050=CARTESIAN_POINT('Ctrl Pts',(-66.9490746964381,-3.00361462447264,
124.921130708376));
#221051=CARTESIAN_POINT('Ctrl Pts',(-67.227522320251,-6.57325501622426,
130.151357196124));
#221052=CARTESIAN_POINT('Ctrl Pts',(-67.5059699440638,-4.10239516942585,
135.981661927186));
#221053=CARTESIAN_POINT('Ctrl Pts',(-67.7844175678767,2.13836542492937,
137.054279679937));
#221054=CARTESIAN_POINT('Ctrl Pts',(-68.0628651916897,6.41407265873309,
132.383527139888));
#221055=CARTESIAN_POINT('Ctrl Pts',(-68.3413128155024,4.79556046403026,
126.261597712398));
#221056=CARTESIAN_POINT('Ctrl Pts',(-68.6197604393155,-1.22983752096341,
124.314245468451));
#221057=CARTESIAN_POINT('Ctrl Pts',(-68.8982080631282,-6.12507490509475,
128.330991986789));
#221058=CARTESIAN_POINT('Ctrl Pts',(-69.1766556869413,-5.39166767798822,
134.620643446035));
#221059=CARTESIAN_POINT('Ctrl Pts',(-69.455103310754,0.296418747580413,
137.403317421698));
#221060=CARTESIAN_POINT('Ctrl Pts',(-69.733550934567,5.7121108249834,134.121872471326));
#221061=CARTESIAN_POINT('Ctrl Pts',(-70.0119985583799,5.87865210635384,
127.791796196812));
#221062=CARTESIAN_POINT('Ctrl Pts',(-70.2904461821926,0.642999290106501,
124.230119453016));
#221063=CARTESIAN_POINT('Ctrl Pts',(-70.5688938060058,-5.18353846148724,
126.709849169906));
#221064=CARTESIAN_POINT('Ctrl Pts',(-70.8473414298183,-6.24665759690589,
132.95223487919));
#221065=CARTESIAN_POINT('Ctrl Pts',(-71.1257890536316,-1.56940356695681,
137.220829071533));
#221066=CARTESIAN_POINT('Ctrl Pts',(-71.4042366774442,4.55005567139915,
135.593002216589));
#221067=CARTESIAN_POINT('Ctrl Pts',(-71.6826843012574,6.48823603031619,
129.56464767029));
#221068=CARTESIAN_POINT('Ctrl Pts',(-71.9611319250699,2.46404444532374,
124.675528759193));
#221069=CARTESIAN_POINT('Ctrl Pts',(-72.2395795488831,-3.82448360965763,
125.418506915858));
#221070=CARTESIAN_POINT('Ctrl Pts',(-72.518027172696,-6.59849806377525,
131.110821510811));
#221071=CARTESIAN_POINT('Ctrl Pts',(-72.7964747965087,-3.30881515183405,
136.52151351632));
#221072=CARTESIAN_POINT('Ctrl Pts',(-73.0749224203217,3.02150724003593,
136.678421306317));
#221073=CARTESIAN_POINT('Ctrl Pts',(-73.3533700441346,6.57521208714753,
131.437354287172));
#221074=CARTESIAN_POINT('Ctrl Pts',(-73.6318176679474,4.08661824313884,
125.614597009117));
#221075=CARTESIAN_POINT('Ctrl Pts',(-73.9102652917603,-2.15737812391465,
124.56097895318));
#221076=CARTESIAN_POINT('Ctrl Pts',(-74.1887129155733,-6.41884938887091,
129.244723640663));
#221077=CARTESIAN_POINT('Ctrl Pts',(-74.4671605393861,-4.78171164368069,
135.361698517417));
#221078=CARTESIAN_POINT('Ctrl Pts',(-74.745608163199,1.24958550245192,137.290702502541));
#221079=CARTESIAN_POINT('Ctrl Pts',(-75.0240557870119,6.13257461747648,
133.25907517079));
#221080=CARTESIAN_POINT('Ctrl Pts',(-75.3025034108249,5.380027251966,126.971685084098));
#221081=CARTESIAN_POINT('Ctrl Pts',(-75.5809510346376,-0.31650232915867,
124.206336576053));
#221082=CARTESIAN_POINT('Ctrl Pts',(-75.8593986584506,-5.72218173178456,
127.504249830764));
#221083=CARTESIAN_POINT('Ctrl Pts',(-76.1378462822634,-5.86945566701928,
133.83480367917));
#221084=CARTESIAN_POINT('Ctrl Pts',(-76.4162939060764,-0.622986583113102,
137.380528399336));
#221085=CARTESIAN_POINT('Ctrl Pts',(-76.6947415298893,5.19597673608708,
134.88307619171));
#221086=CARTESIAN_POINT('Ctrl Pts',(-76.9731891537022,6.24009127239896,
128.637483627779));
#221087=CARTESIAN_POINT('Ctrl Pts',(-77.2516367775151,1.54986677478153,
124.383145159635));
#221088=CARTESIAN_POINT('Ctrl Pts',(-77.5300844013279,-4.56460957365852,
126.029590003516));
#221089=CARTESIAN_POINT('Ctrl Pts',(-77.8085320251407,-6.48443271748106,
132.063815781194));
#221090=CARTESIAN_POINT('Ctrl Pts',(-78.0869796489538,-2.44537897608793,
136.940663791305));
#221091=CARTESIAN_POINT('Ctrl Pts',(-78.3654272727665,3.84085858092573,
136.178548959823));
#221092=CARTESIAN_POINT('Ctrl Pts',(-78.6438748965796,6.5975347384416,130.477817585504));
#221093=CARTESIAN_POINT('Ctrl Pts',(-78.9223225203923,3.29139877882003,
125.077163305135));
#221094=CARTESIAN_POINT('Ctrl Pts',(-79.2007701442053,-3.03937186476788,
124.939523565746));
#221095=CARTESIAN_POINT('Ctrl Pts',(-79.4792177680182,-6.57710824620412,
130.191382563762));
#221096=CARTESIAN_POINT('Ctrl Pts',(-79.7576653918309,-4.07080345897965,
136.00653844758));
#221097=CARTESIAN_POINT('Ctrl Pts',(-80.036113015644,2.17637083724304,137.041147046131));
#221098=CARTESIAN_POINT('Ctrl Pts',(-80.314560639457,6.42356665566488,132.344453600785));
#221099=CARTESIAN_POINT('Ctrl Pts',(-80.5930082632696,4.76781852620778,
126.232489941585));
#221100=CARTESIAN_POINT('Ctrl Pts',(-80.8714558870828,-1.26932190795047,
124.321852085313));
#221101=CARTESIAN_POINT('Ctrl Pts',(-81.1499035108954,-6.14001751852468,
128.368322882032));
#221102=CARTESIAN_POINT('Ctrl Pts',(-81.4283511347085,-5.36833698610627,
134.653393350648));
#221103=CARTESIAN_POINT('Ctrl Pts',(-81.7067987585213,0.336582978702201,
137.401390773263));
#221104=CARTESIAN_POINT('Ctrl Pts',(-81.9852463823341,5.73219962907597,
134.087039765632));
#221105=CARTESIAN_POINT('Ctrl Pts',(-82.2636940061471,5.86020485384888,
127.756066988721));
#221106=CARTESIAN_POINT('Ctrl Pts',(-82.54214162996,0.602968104857597,124.226327139294));
#221107=CARTESIAN_POINT('Ctrl Pts',(-82.8205892537728,-5.20836687586887,
126.741478701599));
#221108=CARTESIAN_POINT('Ctrl Pts',(-83.0990368775859,-6.23346714053832,
132.990220261861));
#221109=CARTESIAN_POINT('Ctrl Pts',(-83.3774845013985,-1.53031562485268,
137.230263594196));
#221110=CARTESIAN_POINT('Ctrl Pts',(-83.6559321252116,4.57912118999838,
135.56521601382));
#221111=CARTESIAN_POINT('Ctrl Pts',(-83.9343797490243,6.48056933374724,
129.525174905002));
#221112=CARTESIAN_POINT('Ctrl Pts',(-84.2128273728376,2.42669085319518,
124.660642974335));
#221113=CARTESIAN_POINT('Ctrl Pts',(-84.4912749966499,-3.85719797100462,
125.441887420503));
#221114=CARTESIAN_POINT('Ctrl Pts',(-84.7697226204634,-6.59651029444787,
131.150982763393));
#221115=CARTESIAN_POINT('Ctrl Pts',(-85.0481702442759,-3.27395191473627,
136.541549287701));
#221116=CARTESIAN_POINT('Ctrl Pts',(-85.326617868089,3.05720833317481,136.659919701402));
#221117=CARTESIAN_POINT('Ctrl Pts',(-85.6050654919017,6.57894347582879,
131.397317377022));
#221118=CARTESIAN_POINT('Ctrl Pts',(-85.8835131157147,4.05495096345227,
125.58981675825));
#221119=CARTESIAN_POINT('Ctrl Pts',(-86.1619607395276,-2.19534338896908,
124.574227201559));
#221120=CARTESIAN_POINT('Ctrl Pts',(-86.4404083633404,-6.42822441541511,
129.283825895241));
#221121=CARTESIAN_POINT('Ctrl Pts',(-86.7188559871533,-4.75388124031539,
135.390721716488));
#221122=CARTESIAN_POINT('Ctrl Pts',(-86.9973036109663,1.28904655462414,
137.282975744021));
#221123=CARTESIAN_POINT('Ctrl Pts',(-87.2757512347791,6.14740353928957,
133.221698968287));
#221124=CARTESIAN_POINT('Ctrl Pts',(-87.554198858592,5.35659698870609,126.939006341782));
#221125=CARTESIAN_POINT('Ctrl Pts',(-87.8326464824051,-0.356660510187587,
124.208385461669));
#221126=CARTESIAN_POINT('Ctrl Pts',(-88.1110941062178,-5.74216442405318,
127.539143518524));
#221127=CARTESIAN_POINT('Ctrl Pts',(-88.3895417300309,-5.85089975254147,
133.870476574676));
#221128=CARTESIAN_POINT('Ctrl Pts',(-88.6679893538435,-0.582944040787213,
137.384198854334));
#221129=CARTESIAN_POINT('Ctrl Pts',(-88.9464369776566,5.22070876605056,
134.851371237371));
#221130=CARTESIAN_POINT('Ctrl Pts',(-89.2248846014694,6.22678526269035,
128.599538568266));
#221131=CARTESIAN_POINT('Ctrl Pts',(-89.5033322252823,1.51075029828878,
124.373829650922));
#221132=CARTESIAN_POINT('Ctrl Pts',(-89.7817798490951,-4.59359038598471,
126.057464543021));
#221133=CARTESIAN_POINT('Ctrl Pts',(-90.0602274729082,-6.47664591490472,
132.103265028861));
#221134=CARTESIAN_POINT('Ctrl Pts',(-90.338675096721,-2.40798024976945,
136.955435815729));
#221135=CARTESIAN_POINT('Ctrl Pts',(-90.6171227205338,3.87350162852866,
136.155068992212));
#221136=CARTESIAN_POINT('Ctrl Pts',(-90.8955703443469,6.59542474128344,
130.437662569033));
#221137=CARTESIAN_POINT('Ctrl Pts',(-91.1740179681596,3.25647472121003,
125.057233738258));
#221138=CARTESIAN_POINT('Ctrl Pts',(-91.4524655919725,-3.07501648002118,
124.958133746811));
#221139=CARTESIAN_POINT('Ctrl Pts',(-91.7309132157855,-6.58071775901922,
130.231430645527));
#221140=CARTESIAN_POINT('Ctrl Pts',(-92.0093608395982,-4.03906090341396,
136.031222199361));
#221141=CARTESIAN_POINT('Ctrl Pts',(-92.2878084634112,2.21429560333469,
137.027783305909));
#221142=CARTESIAN_POINT('Ctrl Pts',(-92.5662560872241,6.4328226249721,132.305322992969));
#221143=CARTESIAN_POINT('Ctrl Pts',(-92.844703711037,4.73989991511645,126.203551583122));
#221144=CARTESIAN_POINT('Ctrl Pts',(-93.1231513348499,-1.30875925974737,
124.329698913911));
#221145=CARTESIAN_POINT('Ctrl Pts',(-93.4015989586628,-6.15473261134757,
128.40574404555));
#221146=CARTESIAN_POINT('Ctrl Pts',(-93.6800465824757,-5.34480736852315,
134.686000627937));
#221147=CARTESIAN_POINT('Ctrl Pts',(-93.9584942062885,0.37673473761816,
137.399219669449));
#221148=CARTESIAN_POINT('Ctrl Pts',(-94.2369418301014,5.75207602440345,
134.052085419056));
#221149=CARTESIAN_POINT('Ctrl Pts',(-94.5153894539144,5.84154044929785,
127.720450736271));
#221150=CARTESIAN_POINT('Ctrl Pts',(-94.7938370777271,0.56291457640357,
124.222778577022));
#221151=CARTESIAN_POINT('Ctrl Pts',(-95.0722847015402,-5.23300229230026,
126.773258784876));
#221152=CARTESIAN_POINT('Ctrl Pts',(-95.350732325353,-6.22004570075364,
133.028124646699));
#221153=CARTESIAN_POINT('Ctrl Pts',(-95.6291799491659,-1.49117097634027,
137.239460002661));
#221154=CARTESIAN_POINT('Ctrl Pts',(-95.9076275729788,4.60801702757804,
135.537253395802));
#221155=CARTESIAN_POINT('Ctrl Pts',(-96.1860751967916,6.47266249729856,
129.48574954041));
#221156=CARTESIAN_POINT('Ctrl Pts',(-96.4645228206046,2.38924733914408,
124.645984847192));
#221157=CARTESIAN_POINT('Ctrl Pts',(-96.7429704444176,-3.88976940246256,
125.465466633565));
#221158=CARTESIAN_POINT('Ctrl Pts',(-97.0214180682302,-6.59427808900543,
131.191131171763));
#221159=CARTESIAN_POINT('Ctrl Pts',(-97.2998656920433,-3.23896736014657,
136.561372465446));
#221160=CARTESIAN_POINT('Ctrl Pts',(-97.5783133158561,3.09279614033489,
136.641201116591));
#221161=CARTESIAN_POINT('Ctrl Pts',(-97.856760939669,6.58243107933991,131.357258494642));
#221162=CARTESIAN_POINT('Ctrl Pts',(-98.135208563482,4.02313342606635,125.565229734223));
#221163=CARTESIAN_POINT('Ctrl Pts',(-98.4136561872948,-2.2332273047675,
124.587706309824));
#221164=CARTESIAN_POINT('Ctrl Pts',(-98.6921038111079,-6.43736124173946,
129.322984493793));
#221165=CARTESIAN_POINT('Ctrl Pts',(-98.9705514349205,-4.72587468013238,
135.419574966262));
#221166=CARTESIAN_POINT('Ctrl Pts',(-99.2489990587337,1.32845984070286,
137.275008918035));
#221167=CARTESIAN_POINT('Ctrl Pts',(-99.5274466825463,6.16200466680371,
133.184233190419));
#221168=CARTESIAN_POINT('Ctrl Pts',(-99.8058943063594,5.3329682347749,126.906470831589));
#221169=CARTESIAN_POINT('Ctrl Pts',(-100.084341930172,-0.396805475030165,
124.210678763569));
#221170=CARTESIAN_POINT('Ctrl Pts',(-100.362789553985,-5.76193433830736,
127.574158200105));
#221171=CARTESIAN_POINT('Ctrl Pts',(-100.641237177798,-5.83212703082168,
133.906035854126));
#221172=CARTESIAN_POINT('Ctrl Pts',(-100.919684801611,-0.542879897255484,
137.387625491007));
#221173=CARTESIAN_POINT('Ctrl Pts',(-101.198132425424,5.24524734073077,
134.819516319564));
#221174=CARTESIAN_POINT('Ctrl Pts',(-101.476580049237,6.21324851716398,
128.561675209245));
#221175=CARTESIAN_POINT('Ctrl Pts',(-101.75502767305,1.47157784038775,124.3647524279));
#221176=CARTESIAN_POINT('Ctrl Pts',(-102.033475296863,-4.62240098113028,
126.085514980508));
#221177=CARTESIAN_POINT('Ctrl Pts',(-102.311922920676,-6.4686191178319,
132.142666145147));
#221178=CARTESIAN_POINT('Ctrl Pts',(-102.590370544489,-2.3704922948573,
136.969979909799));
#221179=CARTESIAN_POINT('Ctrl Pts',(-102.868818168302,3.90600114210426,
136.131390752135));
#221180=CARTESIAN_POINT('Ctrl Pts',(-103.147265792114,6.59307034823604,
130.397521140692));
#221181=CARTESIAN_POINT('Ctrl Pts',(-103.425713415927,3.22142999373166,
125.037517133282));
#221182=CARTESIAN_POINT('Ctrl Pts',(-103.70416103974,-3.11054714940797,
124.976960561963));
#221183=CARTESIAN_POINT('Ctrl Pts',(-103.982608663553,-6.58408342091771,
130.271499957422));
#221184=CARTESIAN_POINT('Ctrl Pts',(-104.261056287366,-4.00716867896111,
136.055712267864));
#221185=CARTESIAN_POINT('Ctrl Pts',(-104.539503911179,2.25213831788793,
137.014188954471));
#221186=CARTESIAN_POINT('Ctrl Pts',(-104.817951534992,6.44184022367115,
132.266136766442));
#221187=CARTESIAN_POINT('Ctrl Pts',(-105.096399158805,4.71180566529118,
126.17478370933));
#221188=CARTESIAN_POINT('Ctrl Pts',(-105.374846782618,-1.34814811498862,
124.337785663482));
#221189=CARTESIAN_POINT('Ctrl Pts',(-105.65329440643,-6.16921963829011,
128.443254090687));
#221190=CARTESIAN_POINT('Ctrl Pts',(-105.931742030243,-5.32107969713743,
134.718464069627));
#221191=CARTESIAN_POINT('Ctrl Pts',(-106.210189654056,0.416872536489867,
137.396804190707));
#221192=CARTESIAN_POINT('Ctrl Pts',(-106.488637277869,5.77173927443855,
134.017010726842));
#221193=CARTESIAN_POINT('Ctrl Pts',(-106.767084901682,5.82265958431723,
127.684948759235));
#221194=CARTESIAN_POINT('Ctrl Pts',(-107.045532525495,0.52284018894291,
124.219473897692));
#221195=CARTESIAN_POINT('Ctrl Pts',(-107.323980149308,-5.25744379790729,
126.805188242113));
#221196=CARTESIAN_POINT('Ctrl Pts',(-107.602427773121,-6.20639377488812,
133.065946629143));
#221197=CARTESIAN_POINT('Ctrl Pts',(-107.880875396933,-1.45197107193893,
137.248417956151));
#221198=CARTESIAN_POINT('Ctrl Pts',(-108.159323020746,4.63674211339212,
135.509115398702));
#221199=CARTESIAN_POINT('Ctrl Pts',(-108.437770644559,6.46451581396073,
129.446373037437));
#221200=CARTESIAN_POINT('Ctrl Pts',(-108.716218268372,2.35171529065418,
124.631554920928));
#221201=CARTESIAN_POINT('Ctrl Pts',(-108.994665892185,-3.92219669708481,
125.489243681306));
#221202=CARTESIAN_POINT('Ctrl Pts',(-109.273113515998,-6.59180153016358,
131.231265248209));
#221203=CARTESIAN_POINT('Ctrl Pts',(-109.551561139811,-3.20386278442967,
136.580982315001));
#221204=CARTESIAN_POINT('Ctrl Pts',(-109.830008763624,3.12826934279688,
136.622266245509));
#221205=CARTESIAN_POINT('Ctrl Pts',(-110.108456387437,6.5856747684467,131.317179124427));
#221206=CARTESIAN_POINT('Ctrl Pts',(-110.38690401125,3.99116680999183,125.540836848117));
#221207=CARTESIAN_POINT('Ctrl Pts',(-110.665351635062,-2.27102846750687,
124.601415778499));
#221208=CARTESIAN_POINT('Ctrl Pts',(-110.943799258875,-6.44625952927566,
129.362197985281));
#221209=CARTESIAN_POINT('Ctrl Pts',(-111.222246882688,-4.69769300092514,
135.448257197571));
#221210=CARTESIAN_POINT('Ctrl Pts',(-111.500694506501,1.36782390021364,
137.266802319797));
#221211=CARTESIAN_POINT('Ctrl Pts',(-111.779142130314,6.17637745896884,
133.1466792255));
#221212=CARTESIAN_POINT('Ctrl Pts',(-112.057589754127,5.30914186574463,
126.874079759138));
#221213=CARTESIAN_POINT('Ctrl Pts',(-112.33603737794,-0.436935736099303,
124.213216396775));
#221214=CARTESIAN_POINT('Ctrl Pts',(-112.614485001753,-5.78149074196569,
127.609292578024));
#221215=CARTESIAN_POINT('Ctrl Pts',(-112.892932625565,-5.81313819748998,
133.94148019986));
#221216=CARTESIAN_POINT('Ctrl Pts',(-113.171380249379,-0.502795637109545,
137.390808182378));
#221217=CARTESIAN_POINT('Ctrl Pts',(-113.449827873191,5.26959155084185,
134.787512618686));
#221218=CARTESIAN_POINT('Ctrl Pts',(-113.728275497004,6.19948153742887,
128.523894953756));
#221219=CARTESIAN_POINT('Ctrl Pts',(-114.006723120817,1.43235085262869,
124.355913826926));
#221220=CARTESIAN_POINT('Ctrl Pts',(-114.28517074463,-4.65104029150761,
126.113740276555));
#221221=CARTESIAN_POINT('Ctrl Pts',(-114.563618368443,-6.46035262369882,
132.182017670029));
#221222=CARTESIAN_POINT('Ctrl Pts',(-114.842065992256,-2.33291650048142,
136.984295534578));
#221223=CARTESIAN_POINT('Ctrl Pts',(-115.120513616069,3.93835591737112,
136.107515116997));
#221224=CARTESIAN_POINT('Ctrl Pts',(-115.398961239881,6.59047164654225,
130.357394787938));
#221225=CARTESIAN_POINT('Ctrl Pts',(-115.677408863695,3.18626589498021,
125.018014220813));
#221226=CARTESIAN_POINT('Ctrl Pts',(-115.955856487507,-3.14596255632626,
124.996003313566));
#221227=CARTESIAN_POINT('Ctrl Pts',(-116.23430411132,-6.58720510718372,
130.311589014666));
#221228=CARTESIAN_POINT('Ctrl Pts',(-116.512751735133,-3.97512796739924,
136.0800077456));
#221229=CARTESIAN_POINT('Ctrl Pts',(-116.791199358946,2.28989757862811,
137.00036449556));
#221230=CARTESIAN_POINT('Ctrl Pts',(-117.069646982759,6.45061911761184,
132.226896373261));
#221231=CARTESIAN_POINT('Ctrl Pts',(-117.348094606572,4.68353681777373,
126.146187386213));
#221232=CARTESIAN_POINT('Ctrl Pts',(-117.626542230384,-1.38748701410568,
124.346112034364));
#221233=CARTESIAN_POINT('Ctrl Pts',(-117.904989854198,-6.18347806253024,
128.480851627495));
#221234=CARTESIAN_POINT('Ctrl Pts',(-118.18343747801,-5.29715485118671,
134.750782472776));
#221235=CARTESIAN_POINT('Ctrl Pts',(-118.461885101824,0.45699488799644,
137.394144426544));
#221236=CARTESIAN_POINT('Ctrl Pts',(-118.740332725636,5.79118865055225,
133.981816988697));
#221237=CARTESIAN_POINT('Ctrl Pts',(-119.018780349449,5.80356295854445,
127.649562373154));
#221238=CARTESIAN_POINT('Ctrl Pts',(-119.297227973262,0.482746427446748,
124.216413223762));
#221239=CARTESIAN_POINT('Ctrl Pts',(-119.575675597075,-5.28169048700048,
126.837265890154));
#221240=CARTESIAN_POINT('Ctrl Pts',(-119.854123220888,-6.19251186881905,
133.103684807684));
#221241=CARTESIAN_POINT('Ctrl Pts',(-120.132570844701,-1.41271736421608,
137.257137122728));
#221242=CARTESIAN_POINT('Ctrl Pts',(-120.411018468513,4.66529538302207,
135.480803065184));
#221243=CARTESIAN_POINT('Ctrl Pts',(-120.689466092327,6.45612958561205,
129.407046855192));
#221244=CARTESIAN_POINT('Ctrl Pts',(-120.967913716139,2.31409609848935,
124.61735373025));
#221245=CARTESIAN_POINT('Ctrl Pts',(-121.246361339953,-3.95447865326606,
125.51321768266));
#221246=CARTESIAN_POINT('Ctrl Pts',(-121.524808963765,-6.5890807096919,
131.271383505546));
#221247=CARTESIAN_POINT('Ctrl Pts',(-121.803256587578,-3.16863948839908,
136.600378109714));
#221248=CARTESIAN_POINT('Ctrl Pts',(-122.081704211391,3.16362662608795,
136.603115789794));
#221249=CARTESIAN_POINT('Ctrl Pts',(-122.360151835204,6.58867442295306,
131.277080751534));
#221250=CARTESIAN_POINT('Ctrl Pts',(-122.638599459017,3.9590522997634,125.51663900382));
#221251=CARTESIAN_POINT('Ctrl Pts',(-122.91704708283,-2.30874547645122,
124.615355099576));
#221252=CARTESIAN_POINT('Ctrl Pts',(-123.195494706643,-6.45491894829438,
129.401464916637));
#221253=CARTESIAN_POINT('Ctrl Pts',(-123.473942330455,-4.66933724697619,
135.476767347585));
#221254=CARTESIAN_POINT('Ctrl Pts',(-123.752389954268,1.40713727450679,
137.258356253404));
#221255=CARTESIAN_POINT('Ctrl Pts',(-124.030837578081,6.19052138319586,
133.109038465103));
#221256=CARTESIAN_POINT('Ctrl Pts',(-124.309285201894,5.28511876451003,
126.841834324687));
#221257=CARTESIAN_POINT('Ctrl Pts',(-124.587732825707,-0.477049806354697,
124.215998267256));
#221258=CARTESIAN_POINT('Ctrl Pts',(-124.86618044952,-5.80083291035842,
127.644545350364));
#221259=CARTESIAN_POINT('Ctrl Pts',(-125.144628073333,-5.79393395618462,
133.976808298475));
#221260=CARTESIAN_POINT('Ctrl Pts',(-125.423075697146,-0.462692745686338,
137.393746810514));
#221261=CARTESIAN_POINT('Ctrl Pts',(-125.701523320958,5.2937404943001,134.755361320645));
#221262=CARTESIAN_POINT('Ctrl Pts',(-125.979970944772,6.18548483362552,
128.486199201761));
#221263=CARTESIAN_POINT('Ctrl Pts',(-126.258418568584,1.39307078858202,
124.34731417552));
#221264=CARTESIAN_POINT('Ctrl Pts',(-126.536866192397,-4.67950725587653,
126.142139385264));
#221265=CARTESIAN_POINT('Ctrl Pts',(-126.81531381621,-6.45184673882346,
132.221318145323));
#221266=CARTESIAN_POINT('Ctrl Pts',(-127.093761440023,-2.29525425902701,
136.998382159598));
#221267=CARTESIAN_POINT('Ctrl Pts',(-127.372209063836,3.97056475541062,
136.083442971518));
#221268=CARTESIAN_POINT('Ctrl Pts',(-127.650656687649,6.58762873249828,
130.317284997668));
#221269=CARTESIAN_POINT('Ctrl Pts',(-127.929104311462,3.15098372797424,
124.998725723536));
#221270=CARTESIAN_POINT('Ctrl Pts',(-128.207551935275,-3.18126138844507,
125.015261295985));
#221271=CARTESIAN_POINT('Ctrl Pts',(-128.485999559087,-6.59008270214206,
130.351696331743));
#221272=CARTESIAN_POINT('Ctrl Pts',(-128.764447182901,-3.94293995600869,
136.104107732291));
#221273=CARTESIAN_POINT('Ctrl Pts',(-129.042894806713,2.32757198637139,
136.986310441447));
#221274=CARTESIAN_POINT('Ctrl Pts',(-129.321342430526,6.45915898148892,
132.187603267495));
#221275=CARTESIAN_POINT('Ctrl Pts',(-129.599790054339,4.6550944200771,126.117763673416));
#221276=CARTESIAN_POINT('Ctrl Pts',(-129.878237678152,-1.42677449938118,
124.354677718024));
#221277=CARTESIAN_POINT('Ctrl Pts',(-130.156685301965,-6.19750735571679,
128.518535262782));
#221278=CARTESIAN_POINT('Ctrl Pts',(-130.435132925778,-5.27303371721495,
134.782954639811));
#221279=CARTESIAN_POINT('Ctrl Pts',(-130.713580549591,0.497100305389368,
137.391240475519));
#221280=CARTESIAN_POINT('Ctrl Pts',(-130.992028173403,5.81042343204081,
133.946505508738));
#221281=CARTESIAN_POINT('Ctrl Pts',(-131.270475797217,5.78425127961196,
127.614292889281));
#221282=CARTESIAN_POINT('Ctrl Pts',(-131.548923421029,0.442634777604211,
124.213596668645));
#221283=CARTESIAN_POINT('Ctrl Pts',(-131.827371044842,-5.30574146111081,
126.869490540348));
#221284=CARTESIAN_POINT('Ctrl Pts',(-132.105818668655,-6.17840049694519,
133.141337783923));
#221285=CARTESIAN_POINT('Ctrl Pts',(-132.384266292468,-1.37341130773126,
137.265617179298));
#221286=CARTESIAN_POINT('Ctrl Pts',(-132.662713916281,4.69367577841589,
135.45231744437));
#221287=CARTESIAN_POINT('Ctrl Pts',(-132.941161540094,6.44750412300737,
129.367772450924));
#221288=CARTESIAN_POINT('Ctrl Pts',(-133.219609163907,2.27639115664257,
124.603381801387));
#221289=CARTESIAN_POINT('Ctrl Pts',(-133.49805678772,-3.98661407478655,
125.537387749261));
#221290=CARTESIAN_POINT('Ctrl Pts',(-133.776504411532,-6.58611572841139,
131.311484457178));
#221291=CARTESIAN_POINT('Ctrl Pts',(-134.054952035345,-3.13329877726696,
136.619559130867));
#221292=CARTESIAN_POINT('Ctrl Pts',(-134.333399659158,3.19886668003099,
136.583750459073));
#221293=CARTESIAN_POINT('Ctrl Pts',(-134.611847282971,6.59142993170542,
131.236964861823));
#221294=CARTESIAN_POINT('Ctrl Pts',(-134.890294906784,3.92679108539655,
125.492637097993));
#221295=CARTESIAN_POINT('Ctrl Pts',(-135.168742530597,-2.34637693398254,
124.629523756529));
#221296=CARTESIAN_POINT('Ctrl Pts',(-135.44719015441,-6.46333917791768,
129.440783832808));
#221297=CARTESIAN_POINT('Ctrl Pts',(-135.725637778223,-4.64080846901838,
135.505104359849));
#221298=CARTESIAN_POINT('Ctrl Pts',(-136.004085402036,1.44639850681073,
137.24967103183));
#221299=CARTESIAN_POINT('Ctrl Pts',(-136.282533025848,6.20443591537649,
133.07131230402));
#221300=CARTESIAN_POINT('Ctrl Pts',(-136.560980649661,5.26089982125598,
126.809735723105));
#221301=CARTESIAN_POINT('Ctrl Pts',(-136.839428273474,-0.517146199354053,
124.219024271924));
#221302=CARTESIAN_POINT('Ctrl Pts',(-137.117875897287,-5.81996012675442,
127.679915210822));
#221303=CARTESIAN_POINT('Ctrl Pts',(-137.3963235211,-5.77451501852576,134.012018840873));
#221304=CARTESIAN_POINT('Ctrl Pts',(-137.674771144913,-0.422572709013315,
137.396441266521));
#221305=CARTESIAN_POINT('Ctrl Pts',(-137.953218768726,5.31769327625758,
134.723063616821));
#221306=CARTESIAN_POINT('Ctrl Pts',(-138.231666392539,6.17125892440694,
128.448589350091));
#221307=CARTESIAN_POINT('Ctrl Pts',(-138.510114016352,1.35373910378499,
124.338953792345));
#221308=CARTESIAN_POINT('Ctrl Pts',(-138.788561640165,-4.70780081938319,
126.170711254294));
#221309=CARTESIAN_POINT('Ctrl Pts',(-139.067009263977,-6.44310177839452,
132.260566114734));
#221310=CARTESIAN_POINT('Ctrl Pts',(-139.34545688779,-2.25750696608163,
137.012239262869));
#221311=CARTESIAN_POINT('Ctrl Pts',(-139.623904511603,4.00262646271346,
136.059175207703));
#221312=CARTESIAN_POINT('Ctrl Pts',(-139.902352135416,6.5845417114487,130.277193256163));
#221313=CARTESIAN_POINT('Ctrl Pts',(-140.180799759229,3.11558480010749,
124.979652356196));
#221314=CARTESIAN_POINT('Ctrl Pts',(-140.459247383042,-3.21644233775325,
125.034733795609));
#221315=CARTESIAN_POINT('Ctrl Pts',(-140.737695006855,-6.59271609916233,
130.391820422461));
#221316=CARTESIAN_POINT('Ctrl Pts',(-141.016142630668,-3.91060583752806,
136.128011334905));
#221317=CARTESIAN_POINT('Ctrl Pts',(-141.294590254481,2.36516014507876,
136.97202731291));
#221318=CARTESIAN_POINT('Ctrl Pts',(-141.573037878293,6.46745949885459,
132.148258905163));
#221319=CARTESIAN_POINT('Ctrl Pts',(-141.851485502106,4.62647952614482,
126.089513624195));
#221320=CARTESIAN_POINT('Ctrl Pts',(-142.129933125919,-1.4660091150024,
124.363482397054));
#221321=CARTESIAN_POINT('Ctrl Pts',(-142.408380749732,-6.21130699798892,
128.556303600169));
#221322=CARTESIAN_POINT('Ctrl Pts',(-142.686828373545,-5.24871718904012,
134.814979378581));
#221323=CARTESIAN_POINT('Ctrl Pts',(-142.965275997358,0.537187302547703,
137.388092445238));
#221324=CARTESIAN_POINT('Ctrl Pts',(-143.243723621171,5.82944290615228,
133.911077595444));
#221325=CARTESIAN_POINT('Ctrl Pts',(-143.522171244983,5.76472526312116,
127.579141614542));
#221326=CARTESIAN_POINT('Ctrl Pts',(-143.800618868797,0.402506725767204,
124.21102433671));
#221327=CARTESIAN_POINT('Ctrl Pts',(-144.079066492609,-5.32959582902011,
126.901860998601));
#221328=CARTESIAN_POINT('Ctrl Pts',(-144.357514116423,-6.1640601821688,
133.178904162615));
#221329=CARTESIAN_POINT('Ctrl Pts',(-144.635961740235,-1.33405435898536,
137.27385781163));
#221330=CARTESIAN_POINT('Ctrl Pts',(-144.914409364048,4.72188224792766,
135.423659591808));
#221331=CARTESIAN_POINT('Ctrl Pts',(-145.192856987861,6.43863974576633,
129.328551279958));
#221332=CARTESIAN_POINT('Ctrl Pts',(-145.471304611674,2.23860186228433,
124.589639652074));
#221333=CARTESIAN_POINT('Ctrl Pts',(-145.749752235487,-4.01860177085642,
125.56175298548));
#221334=CARTESIAN_POINT('Ctrl Pts',(-146.0281998593,-6.58290669619051,131.35156661715));
#221335=CARTESIAN_POINT('Ctrl Pts',(-146.306647483113,-3.09784196059638,
136.638524667701));
#221336=CARTESIAN_POINT('Ctrl Pts',(-146.585095106925,3.2339881987928,136.564170970937));
#221337=CARTESIAN_POINT('Ctrl Pts',(-146.863542730738,6.59394119259793,
131.196832941802));
#221338=CARTESIAN_POINT('Ctrl Pts',(-147.141990354551,3.89438436234147,
125.468832020033));
#221339=CARTESIAN_POINT('Ctrl Pts',(-147.420437978364,-2.38392144565404,
124.643921224334));
#221340=CARTESIAN_POINT('Ctrl Pts',(-147.698885602177,-6.47151990613084,
129.480153276819));
#221341=CARTESIAN_POINT('Ctrl Pts',(-147.97733322599,-4.61210772419611,
135.533267184325));
#221342=CARTESIAN_POINT('Ctrl Pts',(-148.255780849803,1.48560614228611,
137.240746976909));
#221343=CARTESIAN_POINT('Ctrl Pts',(-148.534228473616,6.21812053990256,
133.033502140209));
#221344=CARTESIAN_POINT('Ctrl Pts',(-148.812676097428,5.23648593342438,
126.777785143819));
#221345=CARTESIAN_POINT('Ctrl Pts',(-149.091123721242,-0.557223429310831,
124.222294298654));
#221346=CARTESIAN_POINT('Ctrl Pts',(-149.369571345054,-5.83887168238761,
127.715400848752));
#221347=CARTESIAN_POINT('Ctrl Pts',(-149.648018968867,-5.75488210408933,
134.047110522317));
#221348=CARTESIAN_POINT('Ctrl Pts',(-149.92646659268,-0.382437013753756,
137.398891450554));
#221349=CARTESIAN_POINT('Ctrl Pts',(-150.204914216493,5.34144900913504,
134.690620704017));
#221350=CARTESIAN_POINT('Ctrl Pts',(-150.483361840306,6.15680433691945,
128.411066792389));
#221351=CARTESIAN_POINT('Ctrl Pts',(-150.761809464119,1.31435725568762,
124.330832987197));
#221352=CARTESIAN_POINT('Ctrl Pts',(-151.040257087932,-4.73591993359918,
126.199454824906));
#221353=CARTESIAN_POINT('Ctrl Pts',(-151.318704711745,-6.43411806645975,
132.299760123916));
#221354=CARTESIAN_POINT('Ctrl Pts',(-151.597152335558,-2.21967602038541,
137.025866330917));
#221355=CARTESIAN_POINT('Ctrl Pts',(-151.87559995937,4.03453985122072,136.034712724799));
#221356=CARTESIAN_POINT('Ctrl Pts',(-152.154047583183,6.58121069778455,
130.237121049039));
#221357=CARTESIAN_POINT('Ctrl Pts',(-152.432495206996,3.08007042310019,
124.960794825562));
#221358=CARTESIAN_POINT('Ctrl Pts',(-152.710942830809,-3.25150410060774,
125.054420090877));
#221359=CARTESIAN_POINT('Ctrl Pts',(-152.989390454622,-6.59510520066311,
130.431959800007));
#221360=CARTESIAN_POINT('Ctrl Pts',(-153.267838078435,-3.87812681010997,
136.151717667683));
#221361=CARTESIAN_POINT('Ctrl Pts',(-153.546285702248,2.40266066190714,
136.957515639215));
#221362=CARTESIAN_POINT('Ctrl Pts',(-153.824733326061,6.47552036213011,
132.108864744186));
#221363=CARTESIAN_POINT('Ctrl Pts',(-154.103180949873,4.59769319631231,
126.061438285362));
#221364=CARTESIAN_POINT('Ctrl Pts',(-154.381628573686,-1.50518940711724,
124.372525745196));
#221365=CARTESIAN_POINT('Ctrl Pts',(-154.660076197499,-6.22487647799626,
128.594155240135));
#221366=CARTESIAN_POINT('Ctrl Pts',(-154.938523821312,-5.22420616771914,
134.846855502398));
#221367=CARTESIAN_POINT('Ctrl Pts',(-155.216971445125,0.577254394032953,
137.384700452354));
#221368=CARTESIAN_POINT('Ctrl Pts',(-155.495419068938,5.84824636811312,
133.87553456161));
#221369=CARTESIAN_POINT('Ctrl Pts',(-155.773866692751,5.74498563261573,
127.544109851479));
#221370=CARTESIAN_POINT('Ctrl Pts',(-156.052314316564,0.362363758895462,
124.208696323275));
#221371=CARTESIAN_POINT('Ctrl Pts',(-156.330761940377,-5.353252706796,126.934376065411));
#221372=CARTESIAN_POINT('Ctrl Pts',(-156.60920956419,-6.14949145587554,
133.216382551721));
#221373=CARTESIAN_POINT('Ctrl Pts',(-156.887657188002,-1.29464797636456,
137.281858714364));
#221374=CARTESIAN_POINT('Ctrl Pts',(-157.166104811815,4.74991374635575,
135.394830569423));
#221375=CARTESIAN_POINT('Ctrl Pts',(-157.444552435628,6.42953678236183,
129.28938479565));
#221376=CARTESIAN_POINT('Ctrl Pts',(-157.723000059441,2.20072961571137,
124.576127791533));
#221377=CARTESIAN_POINT('Ctrl Pts',(-158.001447683254,-4.05044055615985,
125.586312488451));
#221378=CARTESIAN_POINT('Ctrl Pts',(-158.279895307067,-6.57945373194114,
131.391628500203));
#221379=CARTESIAN_POINT('Ctrl Pts',(-158.55834293088,-3.06227035225273,
136.657274017441));
#221380=CARTESIAN_POINT('Ctrl Pts',(-158.836790554693,3.2689898809326,136.54437805091));
#221381=CARTESIAN_POINT('Ctrl Pts',(-159.115238178505,6.59620811257463,
131.156686478575));
#221382=CARTESIAN_POINT('Ctrl Pts',(-159.393685802319,3.86183333144169,
125.445224652049));
#221383=CARTESIAN_POINT('Ctrl Pts',(-159.672133426131,-2.42137762023968,
124.658546969484));
#221384=CARTESIAN_POINT('Ctrl Pts',(-159.950581049944,-6.47946082979399,
129.519571789819));
#221385=CARTESIAN_POINT('Ctrl Pts',(-160.229028673757,-4.58323607602601,
135.56125477743));
#221386=CARTESIAN_POINT('Ctrl Pts',(-160.50747629757,1.52475872807955,137.231584419323));
#221387=CARTESIAN_POINT('Ctrl Pts',(-160.785923921383,6.23157474968534,
132.99560937474));
#221388=CARTESIAN_POINT('Ctrl Pts',(-161.064371545196,5.2118780056808,126.745983770767));
#221389=CARTESIAN_POINT('Ctrl Pts',(-161.342819169009,-0.597280011148509,
124.225808226271));
#221390=CARTESIAN_POINT('Ctrl Pts',(-161.621266792821,-5.85756687648338,
127.751000949223));
#221391=CARTESIAN_POINT('Ctrl Pts',(-161.899714416635,-5.73503594038016,
134.08208204247));
#221392=CARTESIAN_POINT('Ctrl Pts',(-162.178162040447,-0.342287147149402,
137.401097271823));
#221393=CARTESIAN_POINT('Ctrl Pts',(-162.45660966426,5.36500681265522,134.658033784415));
#221394=CARTESIAN_POINT('Ctrl Pts',(-162.735057288073,6.14212160678308,
128.373632919072));
#221395=CARTESIAN_POINT('Ctrl Pts',(-163.013504911886,1.27492670359879,
124.322952060995));
#221396=CARTESIAN_POINT('Ctrl Pts',(-163.291952535699,-4.76386355656041,
126.228369031995));
#221397=CARTESIAN_POINT('Ctrl Pts',(-163.570400159512,-6.42489593591386,
132.338898720518));
#221398=CARTESIAN_POINT('Ctrl Pts',(-163.848847783325,-2.18176282377798,
137.039262858781));
#221399=CARTESIAN_POINT('Ctrl Pts',(-164.127295407138,4.06630373837012,
136.010056429275));
#221400=CARTESIAN_POINT('Ctrl Pts',(-164.405743030951,6.57763581493773,
130.197069861187));
#221401=CARTESIAN_POINT('Ctrl Pts',(-164.684190654763,3.04444191295097,
124.942153830408));
#221402=CARTESIAN_POINT('Ctrl Pts',(-164.962638278576,-3.28644537778151,
125.074319452304));
#221403=CARTESIAN_POINT('Ctrl Pts',(-165.241085902389,-6.59724991811553,
130.472112977002));
#221404=CARTESIAN_POINT('Ctrl Pts',(-165.519533526202,-3.84550407727676,
136.175225852179));
#221405=CARTESIAN_POINT('Ctrl Pts',(-165.797981150015,2.44007214726114,
136.942775958099));
#221406=CARTESIAN_POINT('Ctrl Pts',(-166.076428773828,6.48334127261722,
132.069422244329));
#221407=CARTESIAN_POINT('Ctrl Pts',(-166.354876397641,4.56873649726763,
126.03353869726));
#221408=CARTESIAN_POINT('Ctrl Pts',(-166.633324021454,-1.54431392388507,
124.381807427344));
#221409=CARTESIAN_POINT('Ctrl Pts',(-166.911771645267,-6.23821529291649,
128.632088780075));
#221410=CARTESIAN_POINT('Ctrl Pts',(-167.19021926908,-5.19950156151742,
134.878581830081));
#221411=CARTESIAN_POINT('Ctrl Pts',(-167.468666892892,0.617300095144361,
137.381064622557));
#221412=CARTESIAN_POINT('Ctrl Pts',(-167.747114516705,5.86683312115408,
133.839877724298));
#221413=CARTESIAN_POINT('Ctrl Pts',(-168.025562140518,5.72503311955499,
127.509198898206));
#221414=CARTESIAN_POINT('Ctrl Pts',(-168.304009764331,0.32220736450136,
124.206612714607));
#221415=CARTESIAN_POINT('Ctrl Pts',(-168.582457388144,-5.37671121782417,
126.967034535923));
#221416=CARTESIAN_POINT('Ctrl Pts',(-168.860905011957,-6.1346948579149,
133.253771562468));
#221417=CARTESIAN_POINT('Ctrl Pts',(-169.13935263577,-1.25519362008691,
137.289619591024));
#221418=CARTESIAN_POINT('Ctrl Pts',(-169.417800259582,4.77776923498369,
135.365831445486));
#221419=CARTESIAN_POINT('Ctrl Pts',(-169.696247883396,6.42019557010726,
129.250274449328));
#221420=CARTESIAN_POINT('Ctrl Pts',(-169.974695507208,2.16277582029264,
124.562846720449));
#221421=CARTESIAN_POINT('Ctrl Pts',(-170.253143131021,-4.08212925089891,
125.611065348116));
#221422=CARTESIAN_POINT('Ctrl Pts',(-170.531590754834,-6.57575696361412,
131.431668621828));
#221423=CARTESIAN_POINT('Ctrl Pts',(-170.810038378647,-3.02658527035502,
136.675806485322));
#221424=CARTESIAN_POINT('Ctrl Pts',(-171.08848600246,3.30387042945021,136.524372432426));
#221425=CARTESIAN_POINT('Ctrl Pts',(-171.366933626273,6.59823060763395,
131.116526959784));
#221426=CARTESIAN_POINT('Ctrl Pts',(-171.645381250086,3.82913919888762,
125.421815868818));
#221427=CARTESIAN_POINT('Ctrl Pts',(-171.923828873899,-2.45874406978715,
124.673400450021));
#221428=CARTESIAN_POINT('Ctrl Pts',(-172.202276497711,-6.48716165465291,
129.559037911142));
#221429=CARTESIAN_POINT('Ctrl Pts',(-172.480724121525,-4.55419459435809,
135.589066102071));
#221430=CARTESIAN_POINT('Ctrl Pts',(-172.759171745337,1.5638548133772,137.222183698596));
#221431=CARTESIAN_POINT('Ctrl Pts',(-173.03761936915,6.24479804617409,132.957635411742));
#221432=CARTESIAN_POINT('Ctrl Pts',(-173.316066992963,5.18707694988104,
126.714332782362));
#221433=CARTESIAN_POINT('Ctrl Pts',(-173.594514616776,-0.637314460555731,
124.229565924566));
#221434=CARTESIAN_POINT('Ctrl Pts',(-173.872962240589,-5.8760450162844,
127.786714193059));
#221435=CARTESIAN_POINT('Ctrl Pts',(-174.151409864401,-5.71497726280517,
134.11693210545));
#221436=CARTESIAN_POINT('Ctrl Pts',(-174.429857488215,-0.302124596968923,
137.403058648589));
#221437=CARTESIAN_POINT('Ctrl Pts',(-174.708305112027,5.38836581387496,
134.625304065538));
#221438=CARTESIAN_POINT('Ctrl Pts',(-174.98675273584,6.1272112780718,128.336289117263));
#221439=CARTESIAN_POINT('Ctrl Pts',(-175.265200359654,1.2354489086321,124.315311305772));
#221440=CARTESIAN_POINT('Ctrl Pts',(-175.543647983466,-4.79163065280562,
126.257452804136));
#221441=CARTESIAN_POINT('Ctrl Pts',(-175.822095607279,-6.41543572848632,
132.377980454247));
#221442=CARTESIAN_POINT('Ctrl Pts',(-176.100543231092,-2.14376878114676,
137.05242835005));
#221443=CARTESIAN_POINT('Ctrl Pts',(-176.378990854905,4.09791694713909,
135.985207234778));
#221444=CARTESIAN_POINT('Ctrl Pts',(-176.657438478718,6.57381719537689,
130.157041176716));
#221445=CARTESIAN_POINT('Ctrl Pts',(-176.93588610253,3.00870058988678,124.923730061481));
#221446=CARTESIAN_POINT('Ctrl Pts',(-177.214333726344,-3.32126487451375,
125.094431142515));
#221447=CARTESIAN_POINT('Ctrl Pts',(-177.492781350156,-6.59915017204588,
130.512278465557));
#221448=CARTESIAN_POINT('Ctrl Pts',(-177.771228973969,-3.81273884787578,
136.198535017289));
#221449=CARTESIAN_POINT('Ctrl Pts',(-178.049676597782,2.47739321484437,
136.927808815745));
#221450=CARTESIAN_POINT('Ctrl Pts',(-178.328124221595,6.49092194050925,
132.029932867148));
#221451=CARTESIAN_POINT('Ctrl Pts',(-178.606571845408,4.53961050201187,
126.005815893719));
#221452=CARTESIAN_POINT('Ctrl Pts',(-178.885019469221,-1.58338121553252,
124.391327099562));
#221453=CARTESIAN_POINT('Ctrl Pts',(-179.163467093034,-6.25132294847495,
128.670102814346));
#221454=CARTESIAN_POINT('Ctrl Pts',(-179.441914716847,-5.1746042858732,
134.910157185999));
#221455=CARTESIAN_POINT('Ctrl Pts',(-179.72036234066,0.657322921973241,
137.377185090575));
#221456=CARTESIAN_POINT('Ctrl Pts',(-179.998809964472,5.88520247653593,
133.804108404782));
#221457=CARTESIAN_POINT('Ctrl Pts',(-180.277257588285,5.70486846328706,
127.474410048364));
#221458=CARTESIAN_POINT('Ctrl Pts',(-180.555705212098,0.282039030594865,
124.204773587913));
#221459=CARTESIAN_POINT('Ctrl Pts',(-180.834152835911,-5.39997049284089,
126.999835199963));
#221460=CARTESIAN_POINT('Ctrl Pts',(-181.112600459724,-6.11967093658025,
133.291069809391));
#221461=CARTESIAN_POINT('Ctrl Pts',(-181.391048083537,-1.21569275214809,
137.297140154028));
#221462=CARTESIAN_POINT('Ctrl Pts',(-181.669495707349,4.8054476816156,135.336663294571));
#221463=CARTESIAN_POINT('Ctrl Pts',(-181.947943331163,6.41061645514481,
129.21122169024));
#221464=CARTESIAN_POINT('Ctrl Pts',(-182.226390954976,2.12474188242055,
124.549796930959));
#221465=CARTESIAN_POINT('Ctrl Pts',(-182.504838578788,-4.11366668083735,
125.636010647245));
#221466=CARTESIAN_POINT('Ctrl Pts',(-182.783286202602,-6.5718165281946,
131.471685498325));
#221467=CARTESIAN_POINT('Ctrl Pts',(-183.061733826414,-2.99078803722709,
136.694121384618));
#221468=CARTESIAN_POINT('Ctrl Pts',(-183.340181450227,3.33862855183402,
136.5041548568));
#221469=CARTESIAN_POINT('Ctrl Pts',(-183.61862907404,6.60000860283161,131.076355873553));
#221470=CARTESIAN_POINT('Ctrl Pts',(-183.897076697853,3.79630317617236,
125.398606537762));
#221471=CARTESIAN_POINT('Ctrl Pts',(-184.175524321666,-2.49601940966891,
124.68848111554));
#221472=CARTESIAN_POINT('Ctrl Pts',(-184.453971945479,-6.49462209535141,
129.598550178357));
#221473=CARTESIAN_POINT('Ctrl Pts',(-184.732419569291,-4.52498435533419,
135.616700127691));
#221474=CARTESIAN_POINT('Ctrl Pts',(-185.010867193105,1.60289294946002,
137.212545163075));
#221475=CARTESIAN_POINT('Ctrl Pts',(-185.289314816917,6.25778993937471,
132.919581658354));
#221476=CARTESIAN_POINT('Ctrl Pts',(-185.56776244073,5.16208368503734,126.682833351442));
#221477=CARTESIAN_POINT('Ctrl Pts',(-185.846210064543,-0.677325294041226,
124.233567254297));
#221478=CARTESIAN_POINT('Ctrl Pts',(-186.124657688356,-5.89430541707644,
127.822539256894));
#221479=CARTESIAN_POINT('Ctrl Pts',(-186.403105312169,-5.69470681464601,
134.151659419877));
#221480=CARTESIAN_POINT('Ctrl Pts',(-186.681552935982,-0.261950851450417,
137.404775508174));
#221481=CARTESIAN_POINT('Ctrl Pts',(-186.960000559794,5.41152514721792,
134.592432760195));
#221482=CARTESIAN_POINT('Ctrl Pts',(-187.238448183608,6.11207390329327,
128.299036770752));
#221483=CARTESIAN_POINT('Ctrl Pts',(-187.51689580742,1.19592533365239,124.307911004657));
#221484=CARTESIAN_POINT('Ctrl Pts',(-187.795343431234,-4.81922019341476,
126.286705063617));
#221485=CARTESIAN_POINT('Ctrl Pts',(-188.073791055046,-6.40573779472858,
132.417003876913));
#221486=CARTESIAN_POINT('Ctrl Pts',(-188.352238678859,-2.10569530037498,
137.065362316871));
#221487=CARTESIAN_POINT('Ctrl Pts',(-188.630686302672,4.12937830608858,
135.960166062105));
#221488=CARTESIAN_POINT('Ctrl Pts',(-188.909133926485,6.56975498060235,
130.117036478904));
#221489=CARTESIAN_POINT('Ctrl Pts',(-189.187581550298,2.97284777831579,
124.905524201484));
#221490=CARTESIAN_POINT('Ctrl Pts',(-189.466029174111,-3.35596130055467,
125.114754416262));
#221491=CARTESIAN_POINT('Ctrl Pts',(-189.744476797923,-6.60080589203976,
130.552454777323));
#221492=CARTESIAN_POINT('Ctrl Pts',(-190.022924421737,-3.77983233603489,
136.221644299282));
#221493=CARTESIAN_POINT('Ctrl Pts',(-190.301372045549,2.5146224817104,136.912614766765));
#221494=CARTESIAN_POINT('Ctrl Pts',(-190.579819669362,6.49826208490189,
131.990398075938));
#221495=CARTESIAN_POINT('Ctrl Pts',(-190.858267293175,4.51031628981952,
125.978270902017));
#221496=CARTESIAN_POINT('Ctrl Pts',(-191.136714916988,-1.62238983440674,
124.401084409096));
#221497=CARTESIAN_POINT('Ctrl Pts',(-191.415162540801,-6.26419895896261,
128.708195934325));
#221498=CARTESIAN_POINT('Ctrl Pts',(-191.693610164614,-5.14951526336424,
134.941580400114));
#221499=CARTESIAN_POINT('Ctrl Pts',(-191.972057788427,0.697321391460013,
137.373062000163));
#221500=CARTESIAN_POINT('Ctrl Pts',(-192.25050541224,5.90335375357599,133.768227928508));
#221501=CARTESIAN_POINT('Ctrl Pts',(-192.528953036052,5.68449241101982,
127.439744591064));
#221502=CARTESIAN_POINT('Ctrl Pts',(-192.807400659866,0.241860245628379,
124.203179011344));
#221503=CARTESIAN_POINT('Ctrl Pts',(-193.085848283678,-5.42302966996514,
127.032776842093));
#221504=CARTESIAN_POINT('Ctrl Pts',(-193.364295907491,-6.10442024858855,
133.32827591039));
#221505=CARTESIAN_POINT('Ctrl Pts',(-193.642743531304,-1.17614683626724,
137.304420124699));
#221506=CARTESIAN_POINT('Ctrl Pts',(-193.921191155117,4.83294806061645,
135.307327197512));
#221507=CARTESIAN_POINT('Ctrl Pts',(-194.19963877893,6.40079979243214,129.172227965502));
#221508=CARTESIAN_POINT('Ctrl Pts',(-194.478086402743,2.08662921145659,
124.536978906625));
#221509=CARTESIAN_POINT('Ctrl Pts',(-194.756534026555,-4.14505167734362,
125.661147461485));
#221510=CARTESIAN_POINT('Ctrl Pts',(-195.034981650369,-6.5676325716969,
131.511677646851));
#221511=CARTESIAN_POINT('Ctrl Pts',(-195.313429274181,-2.95487997934909,
136.712218036662));
#221512=CARTESIAN_POINT('Ctrl Pts',(-195.591876897994,3.3732629601091,136.483726073203));
#221513=CARTESIAN_POINT('Ctrl Pts',(-195.870324521807,6.60154203228333,
131.03617470844));
#221514=CARTESIAN_POINT('Ctrl Pts',(-196.14877214562,3.76332648004682,125.375597518911));
#221515=CARTESIAN_POINT('Ctrl Pts',(-196.427219769433,-2.53320225863353,
124.703788407225));
#221516=CARTESIAN_POINT('Ctrl Pts',(-196.705667393246,-6.50184187543975,
129.63810712732));
#221517=CARTESIAN_POINT('Ctrl Pts',(-196.984115017059,-4.49560644135098,
135.644155830301));
#221518=CARTESIAN_POINT('Ctrl Pts',(-197.262562640871,1.64187168975517,
137.202669169918));
#221519=CARTESIAN_POINT('Ctrl Pts',(-197.541010264685,6.27054994786743,
132.881449524674));
#221520=CARTESIAN_POINT('Ctrl Pts',(-197.819457888497,5.13689913728475,
126.651486645231));
#221521=CARTESIAN_POINT('Ctrl Pts',(-198.097905512311,-0.717311028988463,
124.237812067191));
#221522=CARTESIAN_POINT('Ctrl Pts',(-198.376353136123,-5.91234740221361,
127.858474813215));
#221523=CARTESIAN_POINT('Ctrl Pts',(-198.654800759936,-5.67422534703162,
134.186262698915));
#221524=CARTESIAN_POINT('Ctrl Pts',(-198.933248383749,-0.221767399246752,
137.406247786956));
#221525=CARTESIAN_POINT('Ctrl Pts',(-199.211696007562,5.43448395450644,
134.559421086446));
#221526=CARTESIAN_POINT('Ctrl Pts',(-199.490143631375,6.09671004336861,
128.261877259937));
#221527=CARTESIAN_POINT('Ctrl Pts',(-199.768591255188,1.15635744321901,
124.300751431872));
#221528=CARTESIAN_POINT('Ctrl Pts',(-200.047038879001,-4.84663115604747,
126.316124726487));
#221529=CARTESIAN_POINT('Ctrl Pts',(-200.325486502814,-6.39580249400115,
132.455967542492));
#221530=CARTESIAN_POINT('Ctrl Pts',(-200.603934126626,-2.06754379228947,
137.078064279972));
#221531=CARTESIAN_POINT('Ctrl Pts',(-200.882381750439,4.16068664940635,
135.934933839164));
#221532=CARTESIAN_POINT('Ctrl Pts',(-201.160829374253,6.56544932114097,
130.077057250143));
#221533=CARTESIAN_POINT('Ctrl Pts',(-201.439276998065,2.9368848067771,124.887536925038));
#221534=CARTESIAN_POINT('Ctrl Pts',(-201.717724621878,-3.39053337021544,
125.13528852046));
#221535=CARTESIAN_POINT('Ctrl Pts',(-201.996172245691,-6.60221701674386,
130.592640423553));
#221536=CARTESIAN_POINT('Ctrl Pts',(-202.274619869504,-3.74678576111652,
136.244552841837));
#221537=CARTESIAN_POINT('Ctrl Pts',(-202.553067493317,2.55175856831618,
136.897194374181));
#221538=CARTESIAN_POINT('Ctrl Pts',(-202.83151511713,6.50536143380309,131.950819335672));
#221539=CARTESIAN_POINT('Ctrl Pts',(-203.109962740942,4.48085494619837,
125.950904742844));
#221540=CARTESIAN_POINT('Ctrl Pts',(-203.388410364755,-1.66133833502902,
124.411078994385));
#221541=CARTESIAN_POINT('Ctrl Pts',(-203.666857988568,-6.27684284725421,
128.746366728457));
#221542=CARTESIAN_POINT('Ctrl Pts',(-203.945305612381,-5.12423542367342,
134.97285030803));
#221543=CARTESIAN_POINT('Ctrl Pts',(-204.223753236194,0.737294021446153,
137.368695504108));
#221544=CARTESIAN_POINT('Ctrl Pts',(-204.502200860007,5.9212862796718,133.732237625041));
#221545=CARTESIAN_POINT('Ctrl Pts',(-204.78064848382,5.66390571779574,127.405203810847));
#221546=CARTESIAN_POINT('Ctrl Pts',(-205.059096107633,0.20167249844203,
124.201829043986));
#221547=CARTESIAN_POINT('Ctrl Pts',(-205.337543731446,-5.44588789473034,
127.065858241646));
#221548=CARTESIAN_POINT('Ctrl Pts',(-205.615991355258,-6.08894335906002,
133.36538848678));
#221549=CARTESIAN_POINT('Ctrl Pts',(-205.894438979071,-1.13655733783284,
137.311459233274));
#221550=CARTESIAN_POINT('Ctrl Pts',(-206.172886602884,4.86026935294961,
135.277824241371));
#221551=CARTESIAN_POINT('Ctrl Pts',(-206.451334226697,6.39074594572923,
129.133294720038));
#221552=CARTESIAN_POINT('Ctrl Pts',(-206.72978185051,2.04843921967989,124.524393122426));
#221553=CARTESIAN_POINT('Ctrl Pts',(-207.008229474323,-4.17628307743617,
125.686474859378));
#221554=CARTESIAN_POINT('Ctrl Pts',(-207.286677098136,-6.56320524915893,
131.551643585487));
#221555=CARTESIAN_POINT('Ctrl Pts',(-207.565124721949,-2.9188624273063,
136.730095770877));
#221556=CARTESIAN_POINT('Ctrl Pts',(-207.843572345762,3.40777237088467,
136.463086838631));
#221557=CARTESIAN_POINT('Ctrl Pts',(-208.122019969575,6.60283083916734,
130.995984953369));
#221558=CARTESIAN_POINT('Ctrl Pts',(-208.400467593387,3.73021033247459,
125.352789664874));
#221559=CARTESIAN_POINT('Ctrl Pts',(-208.678915217201,-2.57029123885685,
124.719321757855));
#221560=CARTESIAN_POINT('Ctrl Pts',(-208.957362841013,-6.50882072738636,
129.677707292235));
#221561=CARTESIAN_POINT('Ctrl Pts',(-209.235810464827,-4.4660619410178,
135.671432192519));
#221562=CARTESIAN_POINT('Ctrl Pts',(-209.514258088639,1.68078958989102,
137.192556085085));
#221563=CARTESIAN_POINT('Ctrl Pts',(-209.792705712452,6.28307759882623,
132.8432404237));
#221564=CARTESIAN_POINT('Ctrl Pts',(-210.071153336265,5.11152423984512,
126.620293825292));
#221565=CARTESIAN_POINT('Ctrl Pts',(-210.349600960078,-0.757270183712145,
124.242300205957));
#221566=CARTESIAN_POINT('Ctrl Pts',(-210.62804858389,-5.93017030314353,
127.894519530418));
#221567=CARTESIAN_POINT('Ctrl Pts',(-210.906496207704,-5.65353361891029,
134.220740660327));
#221568=CARTESIAN_POINT('Ctrl Pts',(-211.184943831516,-0.181575729370575,
137.407475430382));
#221569=CARTESIAN_POINT('Ctrl Pts',(-211.463391455329,5.4572413849935,134.52627026755));
#221570=CARTESIAN_POINT('Ctrl Pts',(-211.741839079142,6.08112026761121,
128.224811961777));
#221571=CARTESIAN_POINT('Ctrl Pts',(-212.020286702955,1.11674670353533,
124.293832852717));
#221572=CARTESIAN_POINT('Ctrl Pts',(-212.298734326768,-4.87386252498038,
126.345710702588));
#221573=CARTESIAN_POINT('Ctrl Pts',(-212.577181950581,-6.38563019446009,
132.494870007167));
#221574=CARTESIAN_POINT('Ctrl Pts',(-212.855629574394,-2.02931567060901,
137.090533768676));
#221575=CARTESIAN_POINT('Ctrl Pts',(-213.134077198207,4.19184081695006,
135.909511500946));
#221576=CARTESIAN_POINT('Ctrl Pts',(-213.412524822019,6.56090037654053,
130.037104971874));
#221577=CARTESIAN_POINT('Ctrl Pts',(-213.690972445832,2.90081300789186,
124.869768898671));
#221578=CARTESIAN_POINT('Ctrl Pts',(-213.969420069645,-3.42497980241531,
125.156032694208));
#221579=CARTESIAN_POINT('Ctrl Pts',(-214.247867693459,-6.60338349386843,
130.632833915152));
#221580=CARTESIAN_POINT('Ctrl Pts',(-214.52631531727,-3.71360034767391,
136.267259796069));
#221581=CARTESIAN_POINT('Ctrl Pts',(-214.804762941084,2.58880009856982,
136.881548209402));
#221582=CARTESIAN_POINT('Ctrl Pts',(-215.083210564897,6.51221972414398,
131.911198112957));
#221583=CARTESIAN_POINT('Ctrl Pts',(-215.36165818871,4.45122756284936,125.923718430264));
#221584=CARTESIAN_POINT('Ctrl Pts',(-215.640105812523,-1.70022527414834,
124.421310485075));
#221585=CARTESIAN_POINT('Ctrl Pts',(-215.918553436335,-6.28925414482577,
128.784613782311));
#221586=CARTESIAN_POINT('Ctrl Pts',(-216.197001060149,-5.09876570355457,
135.003965751026));
#221587=CARTESIAN_POINT('Ctrl Pts',(-216.475448683961,0.77723933073121,
137.364085764208));
#221588=CARTESIAN_POINT('Ctrl Pts',(-216.753896307774,5.93899939032692,
133.696138828015));
#221589=CARTESIAN_POINT('Ctrl Pts',(-217.032343931587,5.64310914646246,
127.370788987637));
#221590=CARTESIAN_POINT('Ctrl Pts',(-217.3107915554,0.161477278206604,124.200723735865));
#221591=CARTESIAN_POINT('Ctrl Pts',(-217.589239179213,-5.46854432011718,
127.099078172778));
#221592=CARTESIAN_POINT('Ctrl Pts',(-217.867686803026,-6.07324084149572,
133.402406163341));
#221593=CARTESIAN_POINT('Ctrl Pts',(-218.146134426838,-1.09692572384833,
137.318257218917));
#221594=CARTESIAN_POINT('Ctrl Pts',(-218.424582050652,4.88741054621452,
135.24815551939));
#221595=CARTESIAN_POINT('Ctrl Pts',(-218.703029674464,6.38045528758512,
129.094423396537));
#221596=CARTESIAN_POINT('Ctrl Pts',(-218.981477298277,2.01017332223456,
124.512040044732));
#221597=CARTESIAN_POINT('Ctrl Pts',(-219.25992492209,-4.20735972382344,
125.711991902411));
#221598=CARTESIAN_POINT('Ctrl Pts',(-219.538372545903,-6.55853472463687,
131.591581833275));
#221599=CARTESIAN_POINT('Ctrl Pts',(-219.816820169716,-2.8827367157428,
136.747753924796));
#221600=CARTESIAN_POINT('Ctrl Pts',(-220.095267793529,3.44215550540127,
136.442237917877));
#221601=CARTESIAN_POINT('Ctrl Pts',(-220.373715417342,6.60387497572639,
130.955788097589));
#221602=CARTESIAN_POINT('Ctrl Pts',(-220.652163041155,3.69695596058723,
125.330183820803));
#221603=CARTESIAN_POINT('Ctrl Pts',(-220.930610664968,-2.60728497599312,
124.735080591838));
#221604=CARTESIAN_POINT('Ctrl Pts',(-221.20905828878,-6.51555839258729,
129.717349205704));
#221605=CARTESIAN_POINT('Ctrl Pts',(-221.487505912593,-4.43635194911701,
135.698528203611));
#221606=CARTESIAN_POINT('Ctrl Pts',(-221.765953536406,1.71964520775051,
137.182206283321));
#221607=CARTESIAN_POINT('Ctrl Pts',(-222.044401160219,6.295372428034,132.804955771283));
#221608=CARTESIAN_POINT('Ctrl Pts',(-222.322848784032,5.08595993299503,
126.589256047487));
#221609=CARTESIAN_POINT('Ctrl Pts',(-222.601296407845,-0.797201277510683,
124.247031504286));
#221610=CARTESIAN_POINT('Ctrl Pts',(-222.879744031658,-5.94777345943203,
127.930672072853));
#221611=CARTESIAN_POINT('Ctrl Pts',(-223.158191655471,-5.63263239702162,
134.255092026522));
#221612=CARTESIAN_POINT('Ctrl Pts',(-223.436639279283,-0.141377331138957,
137.40845839296));
#221613=CARTESIAN_POINT('Ctrl Pts',(-223.715086903097,5.47979659539413,
134.492981531924));
#221614=CARTESIAN_POINT('Ctrl Pts',(-223.993534526909,6.06530515370598,
128.187842249741));
#221615=CARTESIAN_POINT('Ctrl Pts',(-224.271982150722,1.07709458239186,
124.287155523561));
#221616=CARTESIAN_POINT('Ctrl Pts',(-224.550429774535,-4.90091329114502,
126.375461895601));
#221617=CARTESIAN_POINT('Ctrl Pts',(-224.828877398348,-6.37522127304402,
132.533709829396));
#221618=CARTESIAN_POINT('Ctrl Pts',(-225.107325022161,-1.99101235188949,
137.102770320923));
#221619=CARTESIAN_POINT('Ctrl Pts',(-225.385772645974,4.22283965429091,
135.883899989486));
#221620=CARTESIAN_POINT('Ctrl Pts',(-225.664220269787,6.55610831536389,
129.997181124546));
#221621=CARTESIAN_POINT('Ctrl Pts',(-225.9426678936,2.86463371831382,124.852220780782));
#221622=CARTESIAN_POINT('Ctrl Pts',(-226.221115517412,-3.45929932072906,
125.176986168825));
#221623=CARTESIAN_POINT('Ctrl Pts',(-226.499563141226,-6.60430528018926,
130.673033762736));
#221624=CARTESIAN_POINT('Ctrl Pts',(-226.778010765038,-3.68027732540471,
136.289764320562));
#221625=CARTESIAN_POINT('Ctrl Pts',(-227.056458388851,2.62574569988376,
136.865676852203));
#221626=CARTESIAN_POINT('Ctrl Pts',(-227.334906012664,6.51883670178814,
131.871535875972));
#221627=CARTESIAN_POINT('Ctrl Pts',(-227.613353636477,4.42143523762624,
125.896712971676));
#221628=CARTESIAN_POINT('Ctrl Pts',(-227.89180126029,-1.73904921079426,
124.431778502036));
#221629=CARTESIAN_POINT('Ctrl Pts',(-228.170248884103,-6.30143239177224,
128.822935678624));
#221630=CARTESIAN_POINT('Ctrl Pts',(-228.448696507916,-5.07310704679746,
135.034925576111));
#221631=CARTESIAN_POINT('Ctrl Pts',(-228.727144131728,0.81715583912702,
137.359232951281));
#221632=CARTESIAN_POINT('Ctrl Pts',(-229.005591755541,5.95649242917557,
133.659932875084));
#221633=CARTESIAN_POINT('Ctrl Pts',(-229.284039379354,5.62210346764449,
127.336501396687));
#221634=CARTESIAN_POINT('Ctrl Pts',(-229.562487003167,0.121276074371264,
124.199863127936));
#221635=CARTESIAN_POINT('Ctrl Pts',(-229.84093462698,-5.4909981065832,127.132435404515));
#221636=CARTESIAN_POINT('Ctrl Pts',(-230.119382250793,-6.0573132777586,
133.439327568368));
#221637=CARTESIAN_POINT('Ctrl Pts',(-230.397829874606,-1.05725346287773,
137.324813829725));
#221638=CARTESIAN_POINT('Ctrl Pts',(-230.676277498418,4.91437063468431,
135.218322130955));
#221639=CARTESIAN_POINT('Ctrl Pts',(-230.954725122232,6.3699281993239,129.055615435388));
#221640=CARTESIAN_POINT('Ctrl Pts',(-231.233172746044,1.97183293707754,
124.49992013129));
#221641=CARTESIAN_POINT('Ctrl Pts',(-231.511620369858,-4.23828046494889,
125.73769764504));
#221642=CARTESIAN_POINT('Ctrl Pts',(-231.79006799367,-6.55362117119865,
131.631490910294));
#221643=CARTESIAN_POINT('Ctrl Pts',(-232.068515617483,-2.84650418331021,
136.765191844092));
#221644=CARTESIAN_POINT('Ctrl Pts',(-232.346963241296,3.47641108958031,
136.421180083507));
#221645=CARTESIAN_POINT('Ctrl Pts',(-232.625410865109,6.60467440326965,
130.915585630608));
#221646=CARTESIAN_POINT('Ctrl Pts',(-232.903858488922,3.66356459663667,
125.307780824367));
#221647=CARTESIAN_POINT('Ctrl Pts',(-233.182306112735,-2.64418209922576,
124.751064325225));
#221648=CARTESIAN_POINT('Ctrl Pts',(-233.460753736548,-6.52205462137589,
129.75703139878));
#221649=CARTESIAN_POINT('Ctrl Pts',(-233.73920136036,-4.40647756656326,
135.725442859523));
#221650=CARTESIAN_POINT('Ctrl Pts',(-234.017648984174,1.75843710352442,
137.17162014814));
#221651=CARTESIAN_POINT('Ctrl Pts',(-234.296096607986,6.30743397990132,
132.766596986079));
#221652=CARTESIAN_POINT('Ctrl Pts',(-234.574544231799,5.06020716402928,
126.558374461932));
#221653=CARTESIAN_POINT('Ctrl Pts',(-234.852991855612,-0.837102830722735,
124.252005786856));
#221654=CARTESIAN_POINT('Ctrl Pts',(-235.131439479425,-5.96515621878728,
127.966931100874));
#221655=CARTESIAN_POINT('Ctrl Pts',(-235.409887103238,-5.6115224558684,
134.289315524594));
#221656=CARTESIAN_POINT('Ctrl Pts',(-235.688334727051,-0.101173694118813,
137.409196638266));
#221657=CARTESIAN_POINT('Ctrl Pts',(-235.966782350864,5.50214874991674,
134.459556113093));
#221658=CARTESIAN_POINT('Ctrl Pts',(-236.245229974676,6.04926528768773,
128.150969493757));
#221659=CARTESIAN_POINT('Ctrl Pts',(-236.52367759849,1.03740254911254,124.280719691838));
#221660=CARTESIAN_POINT('Ctrl Pts',(-236.802125222302,-4.92778245216537,
126.405377203086));
#221661=CARTESIAN_POINT('Ctrl Pts',(-237.080572846115,-6.36457611545918,
132.572485569954));
#221662=CARTESIAN_POINT('Ctrl Pts',(-237.359020469928,-1.95263525547508,
137.114773483282));
#221663=CARTESIAN_POINT('Ctrl Pts',(-237.637468093741,4.25368201275546,
135.858100253825));
#221664=CARTESIAN_POINT('Ctrl Pts',(-237.915915717553,6.55107331518259,
129.957287187551));
#221665=CARTESIAN_POINT('Ctrl Pts',(-238.194363341367,2.8283482786799,124.834893221623));
#221666=CARTESIAN_POINT('Ctrl Pts',(-238.47281096518,-3.49349065343433,
125.198148167872));
#221667=CARTESIAN_POINT('Ctrl Pts',(-238.751258588993,-6.60498234154917,
130.713238476685));
#221668=CARTESIAN_POINT('Ctrl Pts',(-239.029706212805,-3.64681792910581,
136.312065581403));
#221669=CARTESIAN_POINT('Ctrl Pts',(-239.308153836619,2.66259400322518,
136.8495808907));
#221670=CARTESIAN_POINT('Ctrl Pts',(-239.586601460431,6.52521212154101,
131.831834094415));
#221671=CARTESIAN_POINT('Ctrl Pts',(-239.865049084244,4.39147907449425,
125.869889367774));
#221672=CARTESIAN_POINT('Ctrl Pts',(-240.143496708057,-1.77780870633274,
124.44248265737));
#221673=CARTESIAN_POINT('Ctrl Pts',(-240.42194433187,-6.31337713682396,
128.861330997368));
#221674=CARTESIAN_POINT('Ctrl Pts',(-240.700391955683,-5.04726040419313,
135.065728636055));
#221675=CARTESIAN_POINT('Ctrl Pts',(-240.978839579496,0.857042067512721,
137.354137245149));
#221676=CARTESIAN_POINT('Ctrl Pts',(-241.257287203309,5.97376474800676,
133.623621107872));
#221677=CARTESIAN_POINT('Ctrl Pts',(-241.535734827122,5.60088945971499,
127.302342308534));
#221678=CARTESIAN_POINT('Ctrl Pts',(-241.814182450934,0.0810703766063902,
124.199247252091));
#221679=CARTESIAN_POINT('Ctrl Pts',(-242.092630074747,-5.51324842209508,
127.165928700792));
#221680=CARTESIAN_POINT('Ctrl Pts',(-242.37107769856,-6.04116125805038,
133.476151333726));
#221681=CARTESIAN_POINT('Ctrl Pts',(-242.649525322373,-1.01754202499167,
137.331128822742));
#221682=CARTESIAN_POINT('Ctrl Pts',(-242.927972946186,4.94114861934255,
135.188325181553));
#221683=CARTESIAN_POINT('Ctrl Pts',(-243.206420569999,6.35916507103108,
129.016872274634));
#221684=CARTESIAN_POINT('Ctrl Pts',(-243.484868193812,1.93341948492588,
124.488033831209));
#221685=CARTESIAN_POINT('Ctrl Pts',(-243.763315817625,-4.26904415503308,
125.763591134728));
#221686=CARTESIAN_POINT('Ctrl Pts',(-244.041763441437,-6.54846477091785,
131.671369337695));
#221687=CARTESIAN_POINT('Ctrl Pts',(-244.320211065251,-2.8101661726183,
136.782408882594));
#221688=CARTESIAN_POINT('Ctrl Pts',(-244.598658689063,3.51053785406796,
136.399914115825));
#221689=CARTESIAN_POINT('Ctrl Pts',(-244.877106312876,6.60522909217403,
130.875379042142));
#221690=CARTESIAN_POINT('Ctrl Pts',(-245.155553936689,3.6300374779527,125.285581505715));
#221691=CARTESIAN_POINT('Ctrl Pts',(-245.434001560502,-2.68098124131831,
124.767272365732));
#221692=CARTESIAN_POINT('Ctrl Pts',(-245.712449184315,-6.528309173032,129.796752401026));
#221693=CARTESIAN_POINT('Ctrl Pts',(-245.990896808128,-4.37643990036281,
135.752175162922));
#221694=CARTESIAN_POINT('Ctrl Pts',(-246.269344431941,1.79716383976481,
137.160798071814));
#221695=CARTESIAN_POINT('Ctrl Pts',(-246.547792055753,6.31926180748295,
132.728165489484));
#221696=CARTESIAN_POINT('Ctrl Pts',(-246.826239679567,5.03426688722615,
126.527650212955));
#221697=CARTESIAN_POINT('Ctrl Pts',(-247.104687303379,-0.876973364781528,
124.257222869343));
#221698=CARTESIAN_POINT('Ctrl Pts',(-247.383134927193,-5.98231793708558,
128.003295270889));
#221699=CARTESIAN_POINT('Ctrl Pts',(-247.661582551005,-5.59020457768662,
134.32340988638));
#221700=CARTESIAN_POINT('Ctrl Pts',(-247.940030174818,-0.0609663080697638,
137.409690138946));
#221701=CARTESIAN_POINT('Ctrl Pts',(-248.218477798631,5.524297020294,134.425995249648));
#221702=CARTESIAN_POINT('Ctrl Pts',(-248.496925422444,6.03300126391963,
128.114195060156));
#221703=CARTESIAN_POINT('Ctrl Pts',(-248.775373046256,0.997672074500306,
124.274525596028));
#221704=CARTESIAN_POINT('Ctrl Pts',(-249.05382067007,-4.95446901239483,
126.435455516518));
#221705=CARTESIAN_POINT('Ctrl Pts',(-249.332268293882,-6.35369511616563,
132.611195791991));
#221706=CARTESIAN_POINT('Ctrl Pts',(-249.610715917695,-1.91418580344349,
137.126542810973));
#221707=CARTESIAN_POINT('Ctrl Pts',(-249.889163541508,4.28436674946925,
135.832113249982));
#221708=CARTESIAN_POINT('Ctrl Pts',(-250.167611165321,6.54579556256923,
129.917424639176));
#221709=CARTESIAN_POINT('Ctrl Pts',(-250.446058789134,2.79195803356287,
124.817786863269));
#221710=CARTESIAN_POINT('Ctrl Pts',(-250.724506412947,-3.52755253356211,
125.219517907192));
#221711=CARTESIAN_POINT('Ctrl Pts',(-251.00295403676,-6.60541465285253,
130.75344656718));
#221712=CARTESIAN_POINT('Ctrl Pts',(-251.281401660573,-3.61322339864049,
136.334162752248));
#221713=CARTESIAN_POINT('Ctrl Pts',(-251.559849284386,2.6993436431913,136.83326092127));
#221714=CARTESIAN_POINT('Ctrl Pts',(-251.838296908198,6.53134574711249,
131.792094239578));
#221715=CARTESIAN_POINT('Ctrl Pts',(-252.116744532012,4.3613601835781,125.843248612281));
#221716=CARTESIAN_POINT('Ctrl Pts',(-252.395192155824,-1.81650232468185,
124.453422554885));
#221717=CARTESIAN_POINT('Ctrl Pts',(-252.673639779637,-6.32508793705065,
128.899798314935));
#221718=CARTESIAN_POINT('Ctrl Pts',(-252.95208740345,-5.02122673409033,
135.096373791053));
#221719=CARTESIAN_POINT('Ctrl Pts',(-253.230535027263,0.896896539007115,
137.348798831588));
#221720=CARTESIAN_POINT('Ctrl Pts',(-253.508982651076,5.99081570467794,
133.587204877683));
#221721=CARTESIAN_POINT('Ctrl Pts',(-253.787430274889,5.57946791275175,
127.26831297809));
#221722=CARTESIAN_POINT('Ctrl Pts',(-254.065877898701,0.0408616672245685,
124.198876151673));
#221723=CARTESIAN_POINT('Ctrl Pts',(-254.344325522515,-5.53529442795169,
127.199556781751));
#221724=CARTESIAN_POINT('Ctrl Pts',(-254.622773146327,-6.0247854077167,
133.512876168065));
#221725=CARTESIAN_POINT('Ctrl Pts',(-254.90122077014,-0.977792831057213,
137.337201825807));
#221726=CARTESIAN_POINT('Ctrl Pts',(-255.179668393953,4.96774341227684,
135.158166043599));
#221727=CARTESIAN_POINT('Ctrl Pts',(-255.458116017766,6.34816648213513,
128.97819485735));
#221728=CARTESIAN_POINT('Ctrl Pts',(-255.736563641579,1.89493404819936,
124.476382515012));
#221729=CARTESIAN_POINT('Ctrl Pts',(-256.015011265392,-4.29964901022966,
125.789669655819));
#221730=CARTESIAN_POINT('Ctrl Pts',(-256.293458889205,-6.54306693065544,
131.711218953762));
#221731=CARTESIAN_POINT('Ctrl Pts',(-256.571906513018,-2.77372173452912,
136.799398141047));
#221732=CARTESIAN_POINT('Ctrl Pts',(-256.85035413683,3.54453019961847,136.378452625405));
#221733=CARTESIAN_POINT('Ctrl Pts',(-257.128801760644,6.60554720661629,
130.835147498674));
#221734=CARTESIAN_POINT('Ctrl Pts',(-257.407249384456,3.5963603924579,125.263628838565));
#221735=CARTESIAN_POINT('Ctrl Pts',(-257.685697008269,-2.71765185753996,
124.783624522784));
#221736=CARTESIAN_POINT('Ctrl Pts',(-257.964144632082,-6.53437691572335,
129.836661023534));
#221737=CARTESIAN_POINT('Ctrl Pts',(-258.242592255895,-4.34613602341029,
135.778440351053));
#221738=CARTESIAN_POINT('Ctrl Pts',(-258.521039879708,1.83562753012831,
137.150276335207));
#221739=CARTESIAN_POINT('Ctrl Pts',(-258.799487503521,6.33122643152078,
132.688650362788));
#221740=CARTESIAN_POINT('Ctrl Pts',(-259.077935127334,5.00743946241547,
126.498999976245));
#221741=CARTESIAN_POINT('Ctrl Pts',(-259.356382751147,-0.915487258132909,
124.259032700089));
#221742=CARTESIAN_POINT('Ctrl Pts',(-259.634830374959,-6.00176822571329,
128.046924274587));
#221743=CARTESIAN_POINT('Ctrl Pts',(-259.86687006147,-5.63687269779404,
133.292521465648));
#221744=CARTESIAN_POINT('Ctrl Pts',(-260.052531023546,-2.79481741349804,
135.900547185714));
#221745=CARTESIAN_POINT('Ctrl Pts',(-260.145376111017,-0.946914048523564,
136.386386345067));
#221746=CARTESIAN_POINT('Ctrl Pts',(-260.191813261187,-0.0157913329746497,
136.389009763222));
#221747=CARTESIAN_POINT('Ctrl Pts',(210.190947297731,3.04870273111253,135.077142573452));
#221748=CARTESIAN_POINT('Ctrl Pts',(210.144529434129,3.76080111712433,134.569051946243));
#221749=CARTESIAN_POINT('Ctrl Pts',(210.051703633225,4.91317831978039,133.192256847685));
#221750=CARTESIAN_POINT('Ctrl Pts',(209.866061957716,5.67455722768035,129.648049455111));
#221751=CARTESIAN_POINT('Ctrl Pts',(209.634022271206,3.10293383059235,125.427666478792));
#221752=CARTESIAN_POINT('Ctrl Pts',(209.355574647392,-2.85596866243967,
125.28812524467));
#221753=CARTESIAN_POINT('Ctrl Pts',(209.07712702358,-6.17973736462657,130.225196103446));
#221754=CARTESIAN_POINT('Ctrl Pts',(208.798679399767,-3.83016968018938,
135.690661498217));
#221755=CARTESIAN_POINT('Ctrl Pts',(208.520231775954,2.04205955310628,136.667868212554));
#221756=CARTESIAN_POINT('Ctrl Pts',(208.241784152142,6.03618933210081,132.255733564264));
#221757=CARTESIAN_POINT('Ctrl Pts',(207.963336528328,4.48417485225333,126.510421532214));
#221758=CARTESIAN_POINT('Ctrl Pts',(207.684888904515,-1.18901089957204,
124.710731370568));
#221759=CARTESIAN_POINT('Ctrl Pts',(207.406441280703,-5.76932406256156,
128.510946815645));
#221760=CARTESIAN_POINT('Ctrl Pts',(207.12799365689,-5.04803188696711,134.418613818075));
#221761=CARTESIAN_POINT('Ctrl Pts',(206.849546033077,0.312219397189005,
137.005003016302));
#221762=CARTESIAN_POINT('Ctrl Pts',(206.571098409264,5.38552219392035,133.893281295751));
#221763=CARTESIAN_POINT('Ctrl Pts',(206.292650785451,5.50981125882569,127.943004805273));
#221764=CARTESIAN_POINT('Ctrl Pts',(206.014203161638,0.570843377758803,
124.622167937696));
#221765=CARTESIAN_POINT('Ctrl Pts',(205.735755537825,-4.89269661278007,
126.982467612715));
#221766=CARTESIAN_POINT('Ctrl Pts',(205.457307914013,-5.86009012142741,
132.854898402769));
#221767=CARTESIAN_POINT('Ctrl Pts',(205.178860290199,-1.44234566848361,
136.842986120511));
#221768=CARTESIAN_POINT('Ctrl Pts',(204.900412666387,4.30084323855829,135.281871486376));
#221769=CARTESIAN_POINT('Ctrl Pts',(204.621965042573,6.09176771588946,129.606143376667));
#221770=CARTESIAN_POINT('Ctrl Pts',(204.343517418761,2.28465505058828,125.031518229909));
#221771=CARTESIAN_POINT('Ctrl Pts',(204.065069794948,-3.62194388278553,
125.761853295313));
#221772=CARTESIAN_POINT('Ctrl Pts',(203.786622171135,-6.20015338889199,
131.126006208945));
#221773=CARTESIAN_POINT('Ctrl Pts',(203.508174547322,-3.08072479357708,
136.194582558939));
#221774=CARTESIAN_POINT('Ctrl Pts',(203.229726923509,2.86973936865286,136.309808260363));
#221775=CARTESIAN_POINT('Ctrl Pts',(202.951279299696,6.1830532544492,131.365796540178));
#221776=CARTESIAN_POINT('Ctrl Pts',(202.672831675884,3.81444325369211,125.905852631576));
#221777=CARTESIAN_POINT('Ctrl Pts',(202.39438405207,-2.05945374882828,124.947398258377));
#221778=CARTESIAN_POINT('Ctrl Pts',(202.115936428258,-6.04081336739099,
129.371206163854));
#221779=CARTESIAN_POINT('Ctrl Pts',(201.837488804444,-4.47096061076856,
135.112012999282));
#221780=CARTESIAN_POINT('Ctrl Pts',(201.559041180632,1.20748652821524,136.894297736177));
#221781=CARTESIAN_POINT('Ctrl Pts',(201.280593556819,5.77631253695961,133.08022777117));
#221782=CARTESIAN_POINT('Ctrl Pts',(201.002145933006,5.03698951269057,127.174747074221));
#221783=CARTESIAN_POINT('Ctrl Pts',(200.723698309193,-0.331080803069094,
124.604703907164));
#221784=CARTESIAN_POINT('Ctrl Pts',(200.44525068538,-5.39490403503349,127.731842386878));
#221785=CARTESIAN_POINT('Ctrl Pts',(200.166803061567,-5.50107401450091,
133.682475019745));
#221786=CARTESIAN_POINT('Ctrl Pts',(199.888355437754,-0.552025717056,136.988261120707));
#221787=CARTESIAN_POINT('Ctrl Pts',(199.609907813942,4.90430724641216,134.611344759621));
#221788=CARTESIAN_POINT('Ctrl Pts',(199.331460190128,5.85382143915379,128.735995953499));
#221789=CARTESIAN_POINT('Ctrl Pts',(199.053012566316,1.42395970438994,124.761373228423));
#221790=CARTESIAN_POINT('Ctrl Pts',(198.774564942502,-4.31445143441004,
126.339960697623));
#221791=CARTESIAN_POINT('Ctrl Pts',(198.49611731869,-6.088092477657,132.02111359519));
#221792=CARTESIAN_POINT('Ctrl Pts',(198.217669694877,-2.26707395378944,
136.584129948007));
#221793=CARTESIAN_POINT('Ctrl Pts',(197.939222071064,3.6372747808909,135.835820643578));
#221794=CARTESIAN_POINT('Ctrl Pts',(197.660774447251,6.19914568268399,130.46384537573));
#221795=CARTESIAN_POINT('Ctrl Pts',(197.382326823438,3.06430454719326,125.404786980035));
#221796=CARTESIAN_POINT('Ctrl Pts',(197.103879199626,-2.88648276756863,
125.307672973393));
#221797=CARTESIAN_POINT('Ctrl Pts',(196.825431575812,-6.1847334314575,130.261746383626));
#221798=CARTESIAN_POINT('Ctrl Pts',(196.546983952,-3.79951621286212,135.71445576667));
#221799=CARTESIAN_POINT('Ctrl Pts',(196.268536328187,2.07727078866752,136.65502757917));
#221800=CARTESIAN_POINT('Ctrl Pts',(195.990088704374,6.04514741573133,132.219122274927));
#221801=CARTESIAN_POINT('Ctrl Pts',(195.711641080561,4.45782888960729,126.483120122517));
#221802=CARTESIAN_POINT('Ctrl Pts',(195.433193456748,-1.22601660901765,
124.718126880723));
#221803=CARTESIAN_POINT('Ctrl Pts',(195.154745832935,-5.78321273819644,
128.54608511404));
#221804=CARTESIAN_POINT('Ctrl Pts',(194.876298209123,-5.02591888662151,
134.449288212205));
#221805=CARTESIAN_POINT('Ctrl Pts',(194.597850585309,0.349948891971121,
137.002980915508));
#221806=CARTESIAN_POINT('Ctrl Pts',(194.319402961497,5.40423073479611,133.860444384439));
#221807=CARTESIAN_POINT('Ctrl Pts',(194.040955337684,5.49228854369214,127.909516169605));
#221808=CARTESIAN_POINT('Ctrl Pts',(193.762507713871,0.533201494146887,
124.618808581434));
#221809=CARTESIAN_POINT('Ctrl Pts',(193.484060090058,-4.91587168017823,
127.012321133451));
#221810=CARTESIAN_POINT('Ctrl Pts',(193.205612466245,-5.84749893410212,
132.890532719942));
#221811=CARTESIAN_POINT('Ctrl Pts',(192.927164842432,-1.40556033379022,
136.851654059523));
#221812=CARTESIAN_POINT('Ctrl Pts',(192.648717218619,4.32801954783523,135.255608152653));
#221813=CARTESIAN_POINT('Ctrl Pts',(192.370269594806,6.08436090050943,129.569083216569));
#221814=CARTESIAN_POINT('Ctrl Pts',(192.091821970994,2.24947182316989,125.017717865345));
#221815=CARTESIAN_POINT('Ctrl Pts',(191.81337434718,-3.65257196685492,125.783994510198));
#221816=CARTESIAN_POINT('Ctrl Pts',(191.534926723368,-6.19808055740059,
131.163742349203));
#221817=CARTESIAN_POINT('Ctrl Pts',(191.256479099555,-3.04785590876364,
136.213235933607));
#221818=CARTESIAN_POINT('Ctrl Pts',(190.978031475742,2.90319942398833,136.292237340818));
#221819=CARTESIAN_POINT('Ctrl Pts',(190.699583851929,6.18635631527163,131.328148137043));
#221820=CARTESIAN_POINT('Ctrl Pts',(190.421136228116,3.7845539731278,125.882723791311));
#221821=CARTESIAN_POINT('Ctrl Pts',(190.142688604304,-2.09506858458051,
124.960043253581));
#221822=CARTESIAN_POINT('Ctrl Pts',(189.86424098049,-6.04942546284962,129.408004862578));
#221823=CARTESIAN_POINT('Ctrl Pts',(189.585793356678,-4.44465587162338,
135.139149194637));
#221824=CARTESIAN_POINT('Ctrl Pts',(189.307345732864,1.24453533211424,136.886834590562));
#221825=CARTESIAN_POINT('Ctrl Pts',(189.028898109051,5.79005936456987,133.045023550676));
#221826=CARTESIAN_POINT('Ctrl Pts',(188.750450485239,5.01480170111087,127.144152737732));
#221827=CARTESIAN_POINT('Ctrl Pts',(188.472002861426,-0.368813738986236,
124.606834155258));
#221828=CARTESIAN_POINT('Ctrl Pts',(188.193555237613,-5.41350737050784,
127.764739625646));
#221829=CARTESIAN_POINT('Ctrl Pts',(187.9151076138,-5.48345219307025,133.715908293866));
#221830=CARTESIAN_POINT('Ctrl Pts',(187.636659989987,-0.51437233173317,
136.991506884579));
#221831=CARTESIAN_POINT('Ctrl Pts',(187.358212366174,4.92739057398128,134.581420314804));
#221832=CARTESIAN_POINT('Ctrl Pts',(187.079764742362,5.84112225861874,128.700400402891));
#221833=CARTESIAN_POINT('Ctrl Pts',(186.801317118548,1.38714794227173,124.752817144095));
#221834=CARTESIAN_POINT('Ctrl Pts',(186.522869494736,-4.34154756707868,
126.366306703083));
#221835=CARTESIAN_POINT('Ctrl Pts',(186.244421870923,-6.08057295867359,
132.058150998494));
#221836=CARTESIAN_POINT('Ctrl Pts',(185.96597424711,-2.23184885375068,136.597823184897));
#221837=CARTESIAN_POINT('Ctrl Pts',(185.687526623297,3.66783531589119,135.813586298303));
#221838=CARTESIAN_POINT('Ctrl Pts',(185.409078999484,6.19695801394562,130.42611572539));
#221839=CARTESIAN_POINT('Ctrl Pts',(185.130631375671,3.03137903541329,125.386233730096));
#221840=CARTESIAN_POINT('Ctrl Pts',(184.852183751858,-2.9198891855651,125.325345654173));
#221841=CARTESIAN_POINT('Ctrl Pts',(184.573736128045,-6.18792188952598,
130.299404664846));
#221842=CARTESIAN_POINT('Ctrl Pts',(184.295288504232,-3.76955667380246,
135.737493527599));
#221843=CARTESIAN_POINT('Ctrl Pts',(184.01684088042,2.11284697206427,136.642274242971));
#221844=CARTESIAN_POINT('Ctrl Pts',(183.738393256607,6.05364746891681,132.182297534532));
#221845=CARTESIAN_POINT('Ctrl Pts',(183.459945632794,4.43144167895468,126.456064115361));
#221846=CARTESIAN_POINT('Ctrl Pts',(183.181498008981,-1.2630425260055,124.725702755623));
#221847=CARTESIAN_POINT('Ctrl Pts',(182.903050385168,-5.79685235262429,
128.581331012064));
#221848=CARTESIAN_POINT('Ctrl Pts',(182.624602761355,-5.00363805916239,
134.479814874928));
#221849=CARTESIAN_POINT('Ctrl Pts',(182.346155137542,0.387675169361259,
137.000735831198));
#221850=CARTESIAN_POINT('Ctrl Pts',(182.06770751373,5.42273385622678,133.827490675898));
#221851=CARTESIAN_POINT('Ctrl Pts',(181.789259889916,5.47456504449634,127.876136685104));
#221852=CARTESIAN_POINT('Ctrl Pts',(181.510812266103,0.495538404244469,
124.615677436551));
#221853=CARTESIAN_POINT('Ctrl Pts',(181.232364642291,-4.93886382111119,
127.042315697369));
#221854=CARTESIAN_POINT('Ctrl Pts',(180.953917018477,-5.83469147177671,
132.926089453735));
#221855=CARTESIAN_POINT('Ctrl Pts',(180.675469394665,-1.36872270040423,
136.860098061879));
#221856=CARTESIAN_POINT('Ctrl Pts',(180.397021770852,4.35503536681857,135.229179797918));
#221857=CARTESIAN_POINT('Ctrl Pts',(180.118574147039,6.07672868724052,129.532068871648));
#221858=CARTESIAN_POINT('Ctrl Pts',(179.840126523226,2.21420520878857,125.004131904969));
#221859=CARTESIAN_POINT('Ctrl Pts',(179.561678899413,-3.68306468660213,
125.80632176824));
#221860=CARTESIAN_POINT('Ctrl Pts',(179.2832312756,-6.19577806271818,131.20146516627));
#221861=CARTESIAN_POINT('Ctrl Pts',(179.004783651788,-3.01487407978163,
136.231688883676));
#221862=CARTESIAN_POINT('Ctrl Pts',(178.726336027974,2.93655189768736,136.274463064253));
#221863=CARTESIAN_POINT('Ctrl Pts',(178.447888404162,6.18943013971724,131.290480325685));
#221864=CARTESIAN_POINT('Ctrl Pts',(178.169440780348,3.75452445381909,125.859777323623));
#221865=CARTESIAN_POINT('Ctrl Pts',(177.890993156536,-2.13060578642238,
124.972904812372));
#221866=CARTESIAN_POINT('Ctrl Pts',(177.612545532723,-6.05781339482078,
129.44485530364));
#221867=CARTESIAN_POINT('Ctrl Pts',(177.33409790891,-4.41818643401566,135.166124762878));
#221868=CARTESIAN_POINT('Ctrl Pts',(177.055650285097,1.28153801924328,136.879146056599));
#221869=CARTESIAN_POINT('Ctrl Pts',(176.777202661284,5.80359163943039,133.009736301615));
#221870=CARTESIAN_POINT('Ctrl Pts',(176.498755037472,4.99242806419446,127.113694031581));
#221871=CARTESIAN_POINT('Ctrl Pts',(176.220307413658,-0.406533008366379,
124.60919405498));
#221872=CARTESIAN_POINT('Ctrl Pts',(175.941859789846,-5.43191010648008,
127.797749498684));
#221873=CARTESIAN_POINT('Ctrl Pts',(175.663412166033,-5.46562718029972,
133.749233679521));
#221874=CARTESIAN_POINT('Ctrl Pts',(175.38496454222,-0.476699886155768,
136.994523381468));
#221875=CARTESIAN_POINT('Ctrl Pts',(175.106516918407,4.95029131528126,134.551355909651));
#221876=CARTESIAN_POINT('Ctrl Pts',(174.828069294595,5.82820663315002,128.664882815304));
#221877=CARTESIAN_POINT('Ctrl Pts',(174.549621670781,1.35028477887665,124.744485301934));
#221878=CARTESIAN_POINT('Ctrl Pts',(174.271174046969,-4.36848282210566,
126.392817162263));
#221879=CARTESIAN_POINT('Ctrl Pts',(173.992726423155,-6.07282812182305,
132.095141942134));
#221880=CARTESIAN_POINT('Ctrl Pts',(173.714278799343,-2.19654105173196,
136.611301742902));
#221881=CARTESIAN_POINT('Ctrl Pts',(173.435831175529,3.69825993790488,135.791166334329));
#221882=CARTESIAN_POINT('Ctrl Pts',(173.157383551717,6.19454071464915,130.388400091055));
#221883=CARTESIAN_POINT('Ctrl Pts',(172.878935927904,2.99834119476844,125.367881250842));
#221884=CARTESIAN_POINT('Ctrl Pts',(172.600488304091,-2.95318740599396,
125.343221361866));
#221885=CARTESIAN_POINT('Ctrl Pts',(172.322040680278,-6.1908810518732,130.337081657394));
#221886=CARTESIAN_POINT('Ctrl Pts',(172.043593056465,-3.7394574524341,135.760348489473));
#221887=CARTESIAN_POINT('Ctrl Pts',(171.765145432652,2.14834486313941,136.629304580736));
#221888=CARTESIAN_POINT('Ctrl Pts',(171.486697808839,6.06192320196904,132.145421734178));
#221889=CARTESIAN_POINT('Ctrl Pts',(171.208250185027,4.40489025960108,126.42916923593));
#221890=CARTESIAN_POINT('Ctrl Pts',(170.929802561213,-1.30002164048796,
124.733503877423));
#221891=CARTESIAN_POINT('Ctrl Pts',(170.651354937401,-5.81027716255637,
128.616659285268));
#221892=CARTESIAN_POINT('Ctrl Pts',(170.372907313588,-4.98117182005496,
134.510205342342));
#221893=CARTESIAN_POINT('Ctrl Pts',(170.094459689775,0.42538708130529,136.998261137926));
#221894=CARTESIAN_POINT('Ctrl Pts',(169.816012065962,5.44103603626017,133.794424944161));
#221895=CARTESIAN_POINT('Ctrl Pts',(169.537564442149,5.45663868327959,127.842865707018));
#221896=CARTESIAN_POINT('Ctrl Pts',(169.259116818336,0.457856951984399,
124.612775615598));
#221897=CARTESIAN_POINT('Ctrl Pts',(168.980669194523,-4.9616729506289,127.072449665244));
#221898=CARTESIAN_POINT('Ctrl Pts',(168.702221570711,-5.82166780281318,
132.961567566087));
#221899=CARTESIAN_POINT('Ctrl Pts',(168.423773946897,-1.33183434849535,
136.868317666657));
#221900=CARTESIAN_POINT('Ctrl Pts',(168.145326323085,4.38188980836473,135.202587479883));
#221901=CARTESIAN_POINT('Ctrl Pts',(167.866878699272,6.06887129855542,129.495101671966));
#221902=CARTESIAN_POINT('Ctrl Pts',(167.588431075459,2.17885654621902,124.9907608742));
#221903=CARTESIAN_POINT('Ctrl Pts',(167.309983451646,-3.71342092903282,
125.82883423045));
#221904=CARTESIAN_POINT('Ctrl Pts',(167.031535827833,-6.19324598120115,
131.239173268482));
#221905=CARTESIAN_POINT('Ctrl Pts',(166.75308820402,-2.98178053353198,136.249940722101));
#221906=CARTESIAN_POINT('Ctrl Pts',(166.474640580207,2.96979555637586,136.25648609103));
#221907=CARTESIAN_POINT('Ctrl Pts',(166.196192956395,6.19227461255283,131.252794500981));
#221908=CARTESIAN_POINT('Ctrl Pts',(165.917745332582,3.7243558092261,125.837014079288));
#221909=CARTESIAN_POINT('Ctrl Pts',(165.639297708769,-2.16606403788322,
124.985982457902));
#221910=CARTESIAN_POINT('Ctrl Pts',(165.360850084956,-6.06597685228888,
129.481756121673));
#221911=CARTESIAN_POINT('Ctrl Pts',(165.082402461143,-4.39155327888481,
135.192938704347));
#221912=CARTESIAN_POINT('Ctrl Pts',(164.80395483733,1.31849321850979,136.871232419228));
#221913=CARTESIAN_POINT('Ctrl Pts',(164.525507213517,5.81690886006848,132.974367331546));
#221914=CARTESIAN_POINT('Ctrl Pts',(164.247059589704,4.96986943102014,127.083372084437));
#221915=CARTESIAN_POINT('Ctrl Pts',(163.968611965891,-0.444237213516358,
124.611783518878));
#221916=CARTESIAN_POINT('Ctrl Pts',(163.690164342078,-5.45011156102575,
127.830870782803));
#221917=CARTESIAN_POINT('Ctrl Pts',(163.411716718265,-5.44759963670407,
133.782449941821));
#221918=CARTESIAN_POINT('Ctrl Pts',(163.133269094453,-0.439009776288703,
136.9973104996));
#221919=CARTESIAN_POINT('Ctrl Pts',(162.85482147064,4.97300862171615,134.52115265821));
#221920=CARTESIAN_POINT('Ctrl Pts',(162.576373846827,5.81507504134112,128.629444506854));
#221921=CARTESIAN_POINT('Ctrl Pts',(162.297926223014,1.31337158018249,124.736378010682));
#221922=CARTESIAN_POINT('Ctrl Pts',(162.019478599201,-4.39525620139515,
126.419491092807));
#221923=CARTESIAN_POINT('Ctrl Pts',(161.741030975388,-6.06485825409316,
132.132085055398));
#221924=CARTESIAN_POINT('Ctrl Pts',(161.462583351575,-2.16115185607673,
136.624565122567));
#221925=CARTESIAN_POINT('Ctrl Pts',(161.184135727762,3.72854751953661,135.768561582436));
#221926=CARTESIAN_POINT('Ctrl Pts',(160.905688103949,6.19189387436843,130.350699870288));
#221927=CARTESIAN_POINT('Ctrl Pts',(160.627240480137,2.96519224948793,125.349730222329));
#221928=CARTESIAN_POINT('Ctrl Pts',(160.348792856324,-2.9863761949775,125.361299434083));
#221929=CARTESIAN_POINT('Ctrl Pts',(160.070345232511,-6.19361080884636,
130.374775965136));
#221930=CARTESIAN_POINT('Ctrl Pts',(159.791897608698,-3.70921966409463,
135.783019805394));
#221931=CARTESIAN_POINT('Ctrl Pts',(159.513449984885,2.18376314650564,136.616119073061));
#221932=CARTESIAN_POINT('Ctrl Pts',(159.235002361072,6.06997430822783,132.108496240312));
#221933=CARTESIAN_POINT('Ctrl Pts',(158.956554737259,4.37817561541891,126.402436480826));
#221934=CARTESIAN_POINT('Ctrl Pts',(158.678107113446,-1.3369525821905,124.741529957054));
#221935=CARTESIAN_POINT('Ctrl Pts',(158.399659489633,-5.82348667053154,
128.652068624549));
#221936=CARTESIAN_POINT('Ctrl Pts',(158.121211865821,-4.95852100179383,
134.540458488317));
#221937=CARTESIAN_POINT('Ctrl Pts',(157.842764242008,0.463083230374652,
136.995556927392));
#221938=CARTESIAN_POINT('Ctrl Pts',(157.564316618195,5.45913659670229,133.761248414491));
#221939=CARTESIAN_POINT('Ctrl Pts',(157.285868994382,5.43851012430973,127.809704468215));
#221940=CARTESIAN_POINT('Ctrl Pts',(157.007421370569,0.420158533666468,
124.610103226106));
#221941=CARTESIAN_POINT('Ctrl Pts',(156.728973746756,-4.98429822353081,
127.102721920452));
#221942=CARTESIAN_POINT('Ctrl Pts',(156.450526122943,-5.80842840980828,
132.996965742341));
#221943=CARTESIAN_POINT('Ctrl Pts',(156.172078499131,-1.2948966449748,136.876312569277));
#221944=CARTESIAN_POINT('Ctrl Pts',(155.893630875317,4.40858187737264,135.175832183934));
#221945=CARTESIAN_POINT('Ctrl Pts',(155.615183251505,6.06078902561252,129.458182987356));
#221946=CARTESIAN_POINT('Ctrl Pts',(155.336735627692,2.14342714531882,124.977605268507));
#221947=CARTESIAN_POINT('Ctrl Pts',(155.058288003879,-3.74363956928552,
125.85153106262));
#221948=CARTESIAN_POINT('Ctrl Pts',(154.779840380066,-6.19048440667673,
131.276865258552));
#221949=CARTESIAN_POINT('Ctrl Pts',(154.501392756253,-2.94857649630798,
136.267990772552));
#221950=CARTESIAN_POINT('Ctrl Pts',(154.22294513244,3.00292916819795,136.238307087292));
#221951=CARTESIAN_POINT('Ctrl Pts',(153.944497508627,6.19488962837548,131.215092059396));
#221952=CARTESIAN_POINT('Ctrl Pts',(153.666049884815,3.69404915725887,125.814434901805));
#221953=CARTESIAN_POINT('Ctrl Pts',(153.387602261001,-2.20144202504465,
124.999275705575));
#221954=CARTESIAN_POINT('Ctrl Pts',(153.109154637189,-6.07391553275397,
129.518705949301));
#221955=CARTESIAN_POINT('Ctrl Pts',(152.830707013376,-4.36475739313218,
135.219590025439));
#221956=CARTESIAN_POINT('Ctrl Pts',(152.552259389563,1.3553995605252,136.863093971691));
#221957=CARTESIAN_POINT('Ctrl Pts',(152.27381176575,5.83001053300956,132.93891795108));
#221958=CARTESIAN_POINT('Ctrl Pts',(151.995364141937,4.94712663750637,127.053188019893));
#221959=CARTESIAN_POINT('Ctrl Pts',(151.716916518124,-0.481924957293099,
124.614602450997));
#221960=CARTESIAN_POINT('Ctrl Pts',(151.438468894311,-5.46811105968323,
127.864102250682));
#221961=CARTESIAN_POINT('Ctrl Pts',(151.160021270498,-5.4293702303005,133.815555849925));
#221962=CARTESIAN_POINT('Ctrl Pts',(150.881573646685,-0.40130339875292,
136.999868135696));
#221963=CARTESIAN_POINT('Ctrl Pts',(150.603126022873,4.99554165148768,134.490811679673));
#221964=CARTESIAN_POINT('Ctrl Pts',(150.324678399059,5.80172796978809,128.59408679072));
#221965=CARTESIAN_POINT('Ctrl Pts',(150.046230775247,1.27640971402146,124.728495570759));
#221966=CARTESIAN_POINT('Ctrl Pts',(149.767783151434,-4.42186671284978,
126.446327506304));
#221967=CARTESIAN_POINT('Ctrl Pts',(149.489335527621,-6.05666365081033,
132.168978969345));
#221968=CARTESIAN_POINT('Ctrl Pts',(149.210887903808,-2.12568257814469,
136.637612832414));
#221969=CARTESIAN_POINT('Ctrl Pts',(148.932440279995,3.75869693846883,135.74577288025));
#221970=CARTESIAN_POINT('Ctrl Pts',(148.653992656183,6.18901759118317,130.313016460088));
#221971=CARTESIAN_POINT('Ctrl Pts',(148.375545032369,2.93193342791814,125.331781317152));
#221972=CARTESIAN_POINT('Ctrl Pts',(148.097097408557,-3.01945432269288,
125.379579200934));
#221973=CARTESIAN_POINT('Ctrl Pts',(147.818649784743,-6.19611105929333,
130.412486191295));
#221974=CARTESIAN_POINT('Ctrl Pts',(147.540202160931,-3.67884442925635,
135.805506635269));
#221975=CARTESIAN_POINT('Ctrl Pts',(147.261754537118,2.21910050972548,136.602718208539));
#221976=CARTESIAN_POINT('Ctrl Pts',(146.983306913305,6.07780048935632,132.071522421221));
#221977=CARTESIAN_POINT('Ctrl Pts',(146.704859289492,4.35129873632927,126.375866840638));
#221978=CARTESIAN_POINT('Ctrl Pts',(146.426411665679,-1.37383398262348,
124.749780697104));
#221979=CARTESIAN_POINT('Ctrl Pts',(146.147964041867,-5.83648038706648,
128.687557717801));
#221980=CARTESIAN_POINT('Ctrl Pts',(145.869516418053,-4.93568644371351,
134.570573191811));
#221981=CARTESIAN_POINT('Ctrl Pts',(145.591068794241,0.500762219724632,
136.992623299802));
#221982=CARTESIAN_POINT('Ctrl Pts',(145.312621170428,5.47703486683029,133.727962316256));
#221983=CARTESIAN_POINT('Ctrl Pts',(145.034173546615,5.42018003934715,127.776654197497));
#221984=CARTESIAN_POINT('Ctrl Pts',(144.755725922802,0.382444546219556,
124.607660367099));
#221985=CARTESIAN_POINT('Ctrl Pts',(144.477278298989,-5.00673880142907,
127.133131341243));
#221986=CARTESIAN_POINT('Ctrl Pts',(144.198830675176,-5.79497378335261,
133.032282670807));
#221987=CARTESIAN_POINT('Ctrl Pts',(143.920383051363,-1.25791095858285,
136.884082473484));
#221988=CARTESIAN_POINT('Ctrl Pts',(143.64193542755,4.43511058475782,135.148914901497));
#221989=CARTESIAN_POINT('Ctrl Pts',(143.363487803737,6.05248216790344,129.421314185853));
#221990=CARTESIAN_POINT('Ctrl Pts',(143.085040179924,2.10791831893749,124.964665575378));
#221991=CARTESIAN_POINT('Ctrl Pts',(142.806592556112,-3.77371948759721,
125.87441142371));
#221992=CARTESIAN_POINT('Ctrl Pts',(142.528144932299,-6.18749344147606,
131.314539739788));
#221993=CARTESIAN_POINT('Ctrl Pts',(142.249697308486,-2.91526319849757,
136.285838366179));
#221994=CARTESIAN_POINT('Ctrl Pts',(141.971249684673,3.03595150537554,136.219926726669));
#221995=CARTESIAN_POINT('Ctrl Pts',(141.69280206086,6.19727509028471,131.177374398005));
#221996=CARTESIAN_POINT('Ctrl Pts',(141.414354437047,3.6636056209416,125.792040627854));
#221997=CARTESIAN_POINT('Ctrl Pts',(141.135906813234,-2.23673843696229,
125.012784062803));
#221998=CARTESIAN_POINT('Ctrl Pts',(140.857459189421,-6.0816291420453,129.555703417335));
#221999=CARTESIAN_POINT('Ctrl Pts',(140.579011565609,-4.33779976968917,
135.246077738584));
#222000=CARTESIAN_POINT('Ctrl Pts',(140.300563941795,1.39225567771152,136.854731015561));
#222001=CARTESIAN_POINT('Ctrl Pts',(140.022116317983,5.84289617276637,132.903389473806));
#222002=CARTESIAN_POINT('Ctrl Pts',(139.74366869417,4.92420052639575,127.023142956427));
#222003=CARTESIAN_POINT('Ctrl Pts',(139.465221070357,-0.519594843163371,
124.617650746882));
#222004=CARTESIAN_POINT('Ctrl Pts',(139.186773446544,-5.48590793547459,
127.897442670915));
#222005=CARTESIAN_POINT('Ctrl Pts',(138.908325822731,-5.41093963658633,
133.848550177083));
#222006=CARTESIAN_POINT('Ctrl Pts',(138.629878198918,-0.363582150772119,
137.002196194983));
#222007=CARTESIAN_POINT('Ctrl Pts',(138.351430575105,5.0178895696262,134.460334098336));
#222008=CARTESIAN_POINT('Ctrl Pts',(138.072982951292,5.78816591307159,128.558810977095));
#222009=CARTESIAN_POINT('Ctrl Pts',(137.79453532748,1.23940055002892,124.720838274248));
#222010=CARTESIAN_POINT('Ctrl Pts',(137.516087703667,-4.44831337040726,
126.473325408321));
#222011=CARTESIAN_POINT('Ctrl Pts',(137.237640079854,-6.0482446156285,132.205822316857));
#222012=CARTESIAN_POINT('Ctrl Pts',(136.959192456041,-2.09013453226308,
136.650444388955));
#222013=CARTESIAN_POINT('Ctrl Pts',(136.680744832228,3.78870707750376,135.722801072215));
#222014=CARTESIAN_POINT('Ctrl Pts',(136.402297208415,6.18591197167502,130.275351256826));
#222015=CARTESIAN_POINT('Ctrl Pts',(136.123849584602,2.89856596247695,125.314035200413));
#222016=CARTESIAN_POINT('Ctrl Pts',(135.845401960789,-3.05242056341787,
125.398059985055));
#222017=CARTESIAN_POINT('Ctrl Pts',(135.566954336976,-6.19838171056633,
130.450210938505));
#222018=CARTESIAN_POINT('Ctrl Pts',(135.288506713164,-3.64833287348497,
135.827808145838));
#222019=CARTESIAN_POINT('Ctrl Pts',(135.01005908935,2.25435564335981,136.589102483743));
#222020=CARTESIAN_POINT('Ctrl Pts',(134.731611465538,6.08540145535266,132.034501646982));
#222021=CARTESIAN_POINT('Ctrl Pts',(134.453163841725,4.32426061826468,126.349461299917));
#222022=CARTESIAN_POINT('Ctrl Pts',(134.174716217912,-1.41066447513297,
124.75825579184));
#222023=CARTESIAN_POINT('Ctrl Pts',(133.896268594099,-5.84925783067434,
128.723125249964));
#222024=CARTESIAN_POINT('Ctrl Pts',(133.617820970286,-4.91266899195694,
134.600548336913));
#222025=CARTESIAN_POINT('Ctrl Pts',(133.339373346473,0.538422653146471,
136.989460363863));
#222026=CARTESIAN_POINT('Ctrl Pts',(133.06092572266,5.49473018341705,133.694567882885));
#222027=CARTESIAN_POINT('Ctrl Pts',(132.782478098847,5.40164910761999,127.743716119554));
#222028=CARTESIAN_POINT('Ctrl Pts',(132.504030475035,0.344716387149417,
124.605447129098));
#222029=CARTESIAN_POINT('Ctrl Pts',(132.225582851222,-5.02899385277987,
127.163676800786));
#222030=CARTESIAN_POINT('Ctrl Pts',(131.947135227409,-5.78130442201224,
133.067517042801));
#222031=CARTESIAN_POINT('Ctrl Pts',(131.668687603596,-1.22087865983776,
136.891627091362));
#222032=CARTESIAN_POINT('Ctrl Pts',(131.390239979783,4.46147494748924,135.121836630005));
#222033=CARTESIAN_POINT('Ctrl Pts',(131.11179235597,6.04395103324181,129.384496633644));
#222034=CARTESIAN_POINT('Ctrl Pts',(130.833344732157,2.07233138286776,124.951942274296));
#222035=CARTESIAN_POINT('Ctrl Pts',(130.554897108344,-3.80365956934553,
125.897474465882));
#222036=CARTESIAN_POINT('Ctrl Pts',(130.276449484532,-6.18427319643048,
131.35219531615));
#222037=CARTESIAN_POINT('Ctrl Pts',(129.998001860718,-2.88184187453723,
136.303482841632));
#222038=CARTESIAN_POINT('Ctrl Pts',(129.719554236906,3.0688613442533,136.201345690253));
#222039=CARTESIAN_POINT('Ctrl Pts',(129.441106613093,6.1994309098865,131.139642914452));
#222040=CARTESIAN_POINT('Ctrl Pts',(129.16265898928,3.63302632837089,125.769832087263));
#222041=CARTESIAN_POINT('Ctrl Pts',(128.884211365467,-2.27195196571463,
125.026507029031));
#222042=CARTESIAN_POINT('Ctrl Pts',(128.605763741654,-6.08911739433215,
129.592747154821));
#222043=CARTESIAN_POINT('Ctrl Pts',(128.327316117841,-4.31068140748063,
135.272400862266));
#222044=CARTESIAN_POINT('Ctrl Pts',(128.048868494028,1.42906020435147,136.846143860731));
#222045=CARTESIAN_POINT('Ctrl Pts',(127.770420870216,5.85556530185681,132.867783216248));
#222046=CARTESIAN_POINT('Ctrl Pts',(127.491973246402,4.9010919472237,126.993238007373));
#222047=CARTESIAN_POINT('Ctrl Pts',(127.21352562259,-0.557245475255655,
124.620928293575));
#222048=CARTESIAN_POINT('Ctrl Pts',(126.935077998777,-5.50350152892981,
127.930890808061));
#222049=CARTESIAN_POINT('Ctrl Pts',(126.656630374964,-5.39230853851415,
133.881431700678));
#222050=CARTESIAN_POINT('Ctrl Pts',(126.378182751151,-0.325847430121078,
137.004294591193));
#222051=CARTESIAN_POINT('Ctrl Pts',(126.099735127338,5.04005154802147,134.429721043558));
#222052=CARTESIAN_POINT('Ctrl Pts',(125.821287503525,5.77438937373851,128.523618373138));
#222053=CARTESIAN_POINT('Ctrl Pts',(125.542839879712,1.20234545959337,124.713406404895));
#222054=CARTESIAN_POINT('Ctrl Pts',(125.264392255899,-4.47459519407686,
126.50048379844));
#222055=CARTESIAN_POINT('Ctrl Pts',(124.985944632086,-6.03960146051831,
132.24261373269));
#222056=CARTESIAN_POINT('Ctrl Pts',(124.707497008274,-2.05450903567761,
136.663059316712));
#222057=CARTESIAN_POINT('Ctrl Pts',(124.429049384461,3.81857682460466,135.69964700956));
#222058=CARTESIAN_POINT('Ctrl Pts',(124.150601760648,6.18257713092382,130.237705656202));
#222059=CARTESIAN_POINT('Ctrl Pts',(123.872154136835,2.86509108960817,125.296492529702));
#222060=CARTESIAN_POINT('Ctrl Pts',(123.593706513022,-3.08527369557641,
125.416741101634));
#222061=CARTESIAN_POINT('Ctrl Pts',(123.315258889209,-6.20042267852561,
130.487948808862));
#222062=CARTESIAN_POINT('Ctrl Pts',(123.036811265396,-3.61768612739718,
135.849923510712));
#222063=CARTESIAN_POINT('Ctrl Pts',(122.758363641583,2.28952724101679,136.575272403211));
#222064=CARTESIAN_POINT('Ctrl Pts',(122.47991601777,6.09277692456002,131.997435289415));
#222065=CARTESIAN_POINT('Ctrl Pts',(122.201468393958,4.29706226313277,126.323220837128));
#222066=CARTESIAN_POINT('Ctrl Pts',(121.923020770144,-1.44744269495155,
124.766954927214));
#222067=CARTESIAN_POINT('Ctrl Pts',(121.644573146332,-5.86181852788225,
128.758769903068));
#222068=CARTESIAN_POINT('Ctrl Pts',(121.366125522519,-4.88946949944416,
134.630382812884));
#222069=CARTESIAN_POINT('Ctrl Pts',(121.087677898706,0.576063135118759,
136.986068236777));
#222070=CARTESIAN_POINT('Ctrl Pts',(120.809230274893,5.51222189075617,133.661066351821));
#222071=CARTESIAN_POINT('Ctrl Pts',(120.53078265108,5.38291801579874,127.710891454918));
#222072=CARTESIAN_POINT('Ctrl Pts',(120.252335027267,0.306975454486648,
124.603463594118));
#222073=CARTESIAN_POINT('Ctrl Pts',(119.973887403454,-5.05106255291402,
127.194357167205));
#222074=CARTESIAN_POINT('Ctrl Pts',(119.695439779642,-5.76742083231046,
133.102667552701));
#222075=CARTESIAN_POINT('Ctrl Pts',(119.416992155829,-1.18380112098488,
136.898946143343));
#222076=CARTESIAN_POINT('Ctrl Pts',(119.138544532016,4.48767398862585,135.09459837285));
#222077=CARTESIAN_POINT('Ctrl Pts',(118.860096908203,6.03519593775195,129.347731695017));
#222078=CARTESIAN_POINT('Ctrl Pts',(118.58164928439,2.0366676557964,124.939435836727));
#222079=CARTESIAN_POINT('Ctrl Pts',(118.303201660577,-3.83345870508974,
125.920719334523));
#222080=CARTESIAN_POINT('Ctrl Pts',(118.024754036764,-6.18082379086727,
131.389830592295));
#222081=CARTESIAN_POINT('Ctrl Pts',(117.746306412951,-2.84831376286653,
136.320923545089));
#222082=CARTESIAN_POINT('Ctrl Pts',(117.467858789138,3.10165746534553,136.18256466657));
#222083=CARTESIAN_POINT('Ctrl Pts',(117.189411165326,6.20135700729606,131.101899006891));
#222084=CARTESIAN_POINT('Ctrl Pts',(116.910963541513,3.60231241267338,125.747810102979));
#222085=CARTESIAN_POINT('Ctrl Pts',(116.6325159177,-2.30708130645123,125.040444095748));
#222086=CARTESIAN_POINT('Ctrl Pts',(116.354068293887,-6.09638001213474,
129.62983578909));
#222087=CARTESIAN_POINT('Ctrl Pts',(116.075620670074,-4.28340331138726,
135.298558421074));
#222088=CARTESIAN_POINT('Ctrl Pts',(115.797173046261,1.46581177664024,136.837332825402));
#222089=CARTESIAN_POINT('Ctrl Pts',(115.518725422448,5.86801745082159,132.832100497806));
#222090=CARTESIAN_POINT('Ctrl Pts',(115.240277798635,4.87780175628715,126.963474280869));
#222091=CARTESIAN_POINT('Ctrl Pts',(114.961830174822,-0.594875458411799,
124.624434969628));
#222092=CARTESIAN_POINT('Ctrl Pts',(114.68338255101,-5.52089118811201,127.964445422689));
#222093=CARTESIAN_POINT('Ctrl Pts',(114.404934927196,-5.37347762646609,
133.914199202272));
#222094=CARTESIAN_POINT('Ctrl Pts',(114.126487303384,-0.288100635073559,
137.006163246571));
#222095=CARTESIAN_POINT('Ctrl Pts',(113.848039679571,5.06202676545313,134.398973649715));
#222096=CARTESIAN_POINT('Ctrl Pts',(113.569592055758,5.76039886228364,128.488510282924));
#222097=CARTESIAN_POINT('Ctrl Pts',(113.291144431945,1.16524581580469,124.706200238089));
#222098=CARTESIAN_POINT('Ctrl Pts',(113.012696808132,-4.50071120997606,
126.527801670297));
#222099=CARTESIAN_POINT('Ctrl Pts',(112.734249184319,-6.03073450575487,
132.279351853526));
#222100=CARTESIAN_POINT('Ctrl Pts',(112.455801560506,-2.01880740850426,
136.675457148234));
#222101=CARTESIAN_POINT('Ctrl Pts',(112.177353936694,3.84830507293705,135.676311550269));
#222102=CARTESIAN_POINT('Ctrl Pts',(111.898906312881,6.17901319250346,130.200081053184));
#222103=CARTESIAN_POINT('Ctrl Pts',(111.620458689068,2.8315100497353,125.279153955068));
#222104=CARTESIAN_POINT('Ctrl Pts',(111.342011065255,-3.11801250178361,
125.435621858436));
#222105=CARTESIAN_POINT('Ctrl Pts',(111.063563441442,-6.20223388754234,
130.525698403974));
#222106=CARTESIAN_POINT('Ctrl Pts',(110.785115817629,-3.58690532661952,
135.871851910398));
#222107=CARTESIAN_POINT('Ctrl Pts',(110.506668193816,2.32461399939974,136.56122847942));
#222108=CARTESIAN_POINT('Ctrl Pts',(110.228220570003,6.09992662367788,131.960324722029));
#222109=CARTESIAN_POINT('Ctrl Pts',(109.94977294619,4.26970467877848,126.297146424621));
#222110=CARTESIAN_POINT('Ctrl Pts',(109.671325322378,-1.48416727924886,
124.775877780875));
#222111=CARTESIAN_POINT('Ctrl Pts',(109.392877698565,-5.8741620132489,128.794490356288));
#222112=CARTESIAN_POINT('Ctrl Pts',(109.114430074752,-4.86608882584101,
134.660075514194));
#222113=CARTESIAN_POINT('Ctrl Pts',(108.835982450939,0.61368227085971,136.982447044243));
#222114=CARTESIAN_POINT('Ctrl Pts',(108.557534827126,5.52950934068608,133.627458964475));
#222115=CARTESIAN_POINT('Ctrl Pts',(108.279087203313,5.36398745797076,127.67818141992));
#222116=CARTESIAN_POINT('Ctrl Pts',(108.0006395795,0.269223146735527,124.601709835656));
#222117=CARTESIAN_POINT('Ctrl Pts',(107.722191955687,-5.07294408406776,
127.225171303631));
#222118=CARTESIAN_POINT('Ctrl Pts',(107.443744331874,-5.75332352870873,
133.137732897993));
#222119=CARTESIAN_POINT('Ctrl Pts',(107.165296708062,-1.14667971594628,
136.906039358215));
#222120=CARTESIAN_POINT('Ctrl Pts',(106.886849084249,4.51370673735246,135.067201139359));
#222121=CARTESIAN_POINT('Ctrl Pts',(106.608401460436,6.02621720585718,129.31102073231));
#222122=CARTESIAN_POINT('Ctrl Pts',(106.329953836623,2.00092845925606,124.927146726103));
#222123=CARTESIAN_POINT('Ctrl Pts',(106.05150621281,-3.86311579061174,125.944145168289));
#222124=CARTESIAN_POINT('Ctrl Pts',(105.773058588997,-6.17714535260555,
131.427444173636));
#222125=CARTESIAN_POINT('Ctrl Pts',(105.494610965184,-2.81468010588189,
136.338159830278));
#222126=CARTESIAN_POINT('Ctrl Pts',(105.216163341371,3.13433865337982,136.163584351558));
#222127=CARTESIAN_POINT('Ctrl Pts',(104.937715717558,6.20305331114115,131.064144073934));
#222128=CARTESIAN_POINT('Ctrl Pts',(104.659268093745,3.57146501196475,125.725975491034));
#222129=CARTESIAN_POINT('Ctrl Pts',(104.380820469933,-2.34212515744159,
125.054594746511));
#222130=CARTESIAN_POINT('Ctrl Pts',(104.10237284612,-6.10341672633411,129.666967945808));
#222131=CARTESIAN_POINT('Ctrl Pts',(103.823925222307,-4.25596649220884,
135.324549445729));
#222132=CARTESIAN_POINT('Ctrl Pts',(103.545477598494,1.50250903273456,136.828298236068));
#222133=CARTESIAN_POINT('Ctrl Pts',(103.267029974681,5.88025215824177,132.796342640716));
#222134=CARTESIAN_POINT('Ctrl Pts',(102.988582350868,4.85433081661274,126.933852879821));
#222135=CARTESIAN_POINT('Ctrl Pts',(102.710134727055,-0.63248339823904,
124.628170645098));
#222136=CARTESIAN_POINT('Ctrl Pts',(102.431687103242,-5.53807626864099,
127.998105271418));
#222137=CARTESIAN_POINT('Ctrl Pts',(102.153239479429,-5.35444759822839,
133.946851467654));
#222138=CARTESIAN_POINT('Ctrl Pts',(101.874791855617,-0.250343164351048,
137.00780209187));
#222139=CARTESIAN_POINT('Ctrl Pts',(101.596344231803,5.0838144076213,134.368093056165));
#222140=CARTESIAN_POINT('Ctrl Pts',(101.317896607991,5.74619489713063,128.453488007394));
#222141=CARTESIAN_POINT('Ctrl Pts',(101.039448984178,1.12810299340375,124.69922004086));
#222142=CARTESIAN_POINT('Ctrl Pts',(100.761001360365,-4.52666045036627,
126.55527801162));
#222143=CARTESIAN_POINT('Ctrl Pts',(100.482553736552,-6.0216440799065,132.316035318018));
#222144=CARTESIAN_POINT('Ctrl Pts',(100.204106112739,-1.98303097367997,
136.687637424115));
#222145=CARTESIAN_POINT('Ctrl Pts',(99.9256584889259,3.87789072090961,135.652795559044));
#222146=CARTESIAN_POINT('Ctrl Pts',(99.6472108651132,6.17522028847693,130.162478841968));
#222147=CARTESIAN_POINT('Ctrl Pts',(99.3687632413001,2.79782408721636,125.262020118999));
#222148=CARTESIAN_POINT('Ctrl Pts',(99.0903156174874,-3.15063576889091,
125.454701555827));
#222149=CARTESIAN_POINT('Ctrl Pts',(98.8118679936743,-6.20381527050148,
130.563458325018));
#222150=CARTESIAN_POINT('Ctrl Pts',(98.5334203698616,-3.55599161174595,
135.89359253233));
#222151=CARTESIAN_POINT('Ctrl Pts',(98.2549727460486,2.35961461835606,136.546971232774));
#222152=CARTESIAN_POINT('Ctrl Pts',(97.9765251222358,6.10685028777152,131.923171319966));
#222153=CARTESIAN_POINT('Ctrl Pts',(97.6980774984228,4.24218887894701,126.271239028595));
#222154=CARTESIAN_POINT('Ctrl Pts',(97.4196298746099,-1.52083686718185,
124.785024022185));
#222155=CARTESIAN_POINT('Ctrl Pts',(97.141182250797,-5.88628782938184,128.830285285991));
#222156=CARTESIAN_POINT('Ctrl Pts',(96.8627346269842,-4.842527837527,134.689625340572));
#222157=CARTESIAN_POINT('Ctrl Pts',(96.5842870031713,0.651278666378471,
136.978596920444));
#222158=CARTESIAN_POINT('Ctrl Pts',(96.3058393793584,5.54659189261388,133.593746966183));
#222159=CARTESIAN_POINT('Ctrl Pts',(96.0273917555454,5.34485813561491,127.645587226641));
#222160=CARTESIAN_POINT('Ctrl Pts',(95.7489441317327,0.231460862821695,
124.6001859187));
#222161=CARTESIAN_POINT('Ctrl Pts',(95.4704965079195,-5.09463763541278,
127.256118068232));
#222162=CARTESIAN_POINT('Ctrl Pts',(95.192048884107,-5.73901303358793,133.172711779316));
#222163=CARTESIAN_POINT('Ctrl Pts',(94.9136012602939,-1.10951582026908,
136.912906473138));
#222164=CARTESIAN_POINT('Ctrl Pts',(94.635153636481,4.53957222901603,135.039645944743));
#222165=CARTESIAN_POINT('Ctrl Pts',(94.3567060126683,6.01701517026768,129.274365105863));
#222166=CARTESIAN_POINT('Ctrl Pts',(94.0782583888551,1.96511511757592,124.915075397801));
#222167=CARTESIAN_POINT('Ctrl Pts',(93.7998107650425,-3.89262972695748,
125.967751099126));
#222168=CARTESIAN_POINT('Ctrl Pts',(93.5213631412293,-6.17323801795121,
131.465034666385));
#222169=CARTESIAN_POINT('Ctrl Pts',(93.2429155174167,-2.7809421498907,136.355191058501));
#222170=CARTESIAN_POINT('Ctrl Pts',(92.9644678936037,3.16690369734264,136.14440544854));
#222171=CARTESIAN_POINT('Ctrl Pts',(92.6860202697908,6.20451975856463,131.026379514606));
#222172=CARTESIAN_POINT('Ctrl Pts',(92.4075726459779,3.54048526930663,125.704329060518));
#222173=CARTESIAN_POINT('Ctrl Pts',(92.129125022165,-2.37708222012305,125.068958456964));
#222174=CARTESIAN_POINT('Ctrl Pts',(91.850677398352,-6.1102272761821,129.70414224903));
#222175=CARTESIAN_POINT('Ctrl Pts',(91.5722297745392,-4.22837196662692,
135.350372973126));
#222176=CARTESIAN_POINT('Ctrl Pts',(91.2937821507264,1.53915061280415,136.819040427511));
#222177=CARTESIAN_POINT('Ctrl Pts',(91.0153345269133,5.89226897075567,132.76051097));
#222178=CARTESIAN_POINT('Ctrl Pts',(90.7368869031008,4.8306799979248,126.90437490186));
#222179=CARTESIAN_POINT('Ctrl Pts',(90.4584392792875,-0.670067901161403,
124.632135181558));
#222180=CARTESIAN_POINT('Ctrl Pts',(90.1799916554748,-5.5550561337172,128.031869106972));
#222181=CARTESIAN_POINT('Ctrl Pts',(89.9015440316619,-5.3352191589658,133.979387286881));
#222182=CARTESIAN_POINT('Ctrl Pts',(89.6230964078489,-0.212576417070642,
137.009211066365));
#222183=CARTESIAN_POINT('Ctrl Pts',(89.3446487840362,5.10541366717708,134.337080407198));
#222184=CARTESIAN_POINT('Ctrl Pts',(89.0662011602232,5.73177800461257,128.418552844315));
#222185=CARTESIAN_POINT('Ctrl Pts',(88.7877535364103,1.09091836873142,124.69246607186));
#222186=CARTESIAN_POINT('Ctrl Pts',(88.5093059125973,-4.5524419536888,126.58291180426));
#222187=CARTESIAN_POINT('Ctrl Pts',(88.2308582887847,-6.0123305198223,132.352662766849));
#222188=CARTESIAN_POINT('Ctrl Pts',(87.9524106649715,-1.94718105691378,
136.69959969301));
#222189=CARTESIAN_POINT('Ctrl Pts',(87.6739630411587,3.90733267221543,135.629099907278));
#222190=CARTESIAN_POINT('Ctrl Pts',(87.395515417346,6.17119855939173,130.124900415918));
#222191=CARTESIAN_POINT('Ctrl Pts',(87.1170677935327,2.76403445029686,125.245091656395));
#222192=CARTESIAN_POINT('Ctrl Pts',(86.8386201697203,-3.18314228803115,
125.473979486801));
#222193=CARTESIAN_POINT('Ctrl Pts',(86.5601725459069,-6.20516676880425,
130.601227172784));
#222194=CARTESIAN_POINT('Ctrl Pts',(86.2817249220945,-3.52494612829556,
135.915144570902));
#222195=CARTESIAN_POINT('Ctrl Pts',(86.0032772982812,2.394527800925,136.532501191579));
#222196=CARTESIAN_POINT('Ctrl Pts',(85.7248296744686,6.11354766028192,131.885976459962));
#222197=CARTESIAN_POINT('Ctrl Pts',(85.4463820506556,4.21451588324655,126.245499609054));
#222198=CARTESIAN_POINT('Ctrl Pts',(85.1679344268427,-1.55745009994542,
124.794393312227));
#222199=CARTESIAN_POINT('Ctrl Pts',(84.8894868030298,-5.89819552695468,
128.86615336578));
#222200=CARTESIAN_POINT('Ctrl Pts',(84.611039179217,-4.81878740756302,134.719031197036));
#222201=CARTESIAN_POINT('Ctrl Pts',(84.332591555404,0.68885092852684,136.974518008049));
#222202=CARTESIAN_POINT('Ctrl Pts',(84.0541439315912,5.56346891353935,133.559931606153));
#222203=CARTESIAN_POINT('Ctrl Pts',(83.7756963077782,5.32553075757526,127.613110082872));
#222204=CARTESIAN_POINT('Ctrl Pts',(83.4972486839655,0.193690002040587,
124.598891899719));
#222205=CARTESIAN_POINT('Ctrl Pts',(83.2188010601524,-5.11614240308669,
127.287196314267));
#222206=CARTESIAN_POINT('Ctrl Pts',(82.9403534363397,-5.72448987722869,
133.207602900518));
#222207=CARTESIAN_POINT('Ctrl Pts',(82.6619058125266,-1.07231081107503,
136.919547233648));
#222208=CARTESIAN_POINT('Ctrl Pts',(82.3834581887138,4.56526950516122,135.011933810073));
#222209=CARTESIAN_POINT('Ctrl Pts',(82.1050105649009,6.00759017196827,129.237766173961));
#222210=CARTESIAN_POINT('Ctrl Pts',(81.826562941088,1.92922895783247,124.903222299129));
#222211=CARTESIAN_POINT('Ctrl Pts',(81.5481153172751,-3.92199942047723,
125.991536252305));
#222212=CARTESIAN_POINT('Ctrl Pts',(81.2696676934623,-6.16910193169181,
131.502600677615));
#222213=CARTESIAN_POINT('Ctrl Pts',(80.9912200696492,-2.74710114506546,
136.372016598662));
#222214=CARTESIAN_POINT('Ctrl Pts',(80.7127724458365,3.19935139052435,136.125028668197));
#222215=CARTESIAN_POINT('Ctrl Pts',(80.4343248220235,6.20575629522666,130.988606728286));
#222216=CARTESIAN_POINT('Ctrl Pts',(80.1558771982107,3.50937433266497,125.682871613546));
#222217=CARTESIAN_POINT('Ctrl Pts',(79.8774295743978,-2.41195119914859,
125.083534694853));
#222218=CARTESIAN_POINT('Ctrl Pts',(79.5989819505849,-6.11681140931136,
129.741357321249));
#222219=CARTESIAN_POINT('Ctrl Pts',(79.320534326772,-4.20062075716678,135.376028046362));
#222220=CARTESIAN_POINT('Ctrl Pts',(79.0420867029591,1.57573515908161,136.809559742781));
#222221=CARTESIAN_POINT('Ctrl Pts',(78.7636390791462,5.90406744307602,132.724606813414));
#222222=CARTESIAN_POINT('Ctrl Pts',(78.4851914553333,4.80685017661309,126.875041439303));
#222223=CARTESIAN_POINT('Ctrl Pts',(78.2067438315204,-0.707627574471386,
124.636328432103));
#222224=CARTESIAN_POINT('Ctrl Pts',(77.9282962077074,-5.57183015414549,
128.065735678218));
#222225=CARTESIAN_POINT('Ctrl Pts',(77.6498485838947,-5.31579302119528,
134.011805454327));
#222226=CARTESIAN_POINT('Ctrl Pts',(77.3714009600817,-0.174801792692954,
137.010390117845));
#222227=CARTESIAN_POINT('Ctrl Pts',(77.0929533362689,5.12682374375196,134.305936852001));
#222228=CARTESIAN_POINT('Ctrl Pts',(76.814505712456,5.7171487189526,128.38370608822));
#222229=CARTESIAN_POINT('Ctrl Pts',(76.536058088643,1.05369331967776,124.68593858136));
#222230=CARTESIAN_POINT('Ctrl Pts',(76.2576104648302,-4.57805476460059,
126.610702024239));
#222231=CARTESIAN_POINT('Ctrl Pts',(75.9791628410172,-6.00279417061961,
132.389232842773));
#222232=CARTESIAN_POINT('Ctrl Pts',(75.7007152172044,-1.91125898663751,
136.711343511654));
#222233=CARTESIAN_POINT('Ctrl Pts',(75.4222675933915,3.93662983587222,135.605225473025));
#222234=CARTESIAN_POINT('Ctrl Pts',(75.1438199695785,6.16694815427437,130.087347167514));
#222235=CARTESIAN_POINT('Ctrl Pts',(74.8653723457658,2.73014239106432,125.228369194547));
#222236=CARTESIAN_POINT('Ctrl Pts',(74.5869247219528,-3.21553085466319,
125.493454937009));
#222237=CARTESIAN_POINT('Ctrl Pts',(74.3084770981399,-6.20628833237051,
130.639003547736));
#222238=CARTESIAN_POINT('Ctrl Pts',(74.0300294743271,-3.49377002667009,
135.936507227495));
#222239=CARTESIAN_POINT('Ctrl Pts',(73.7515818505141,2.42935225338577,136.517818892029));
#222240=CARTESIAN_POINT('Ctrl Pts',(73.4731342267013,6.1200184930355,131.848741520285));
#222241=CARTESIAN_POINT('Ctrl Pts',(73.1946866028884,4.18668671711015,126.219929119786));
#222242=CARTESIAN_POINT('Ctrl Pts',(72.9162389790755,-1.59400562082267,
124.803985303816));
#222243=CARTESIAN_POINT('Ctrl Pts',(72.6377913552626,-5.90988466472314,
128.902093266552));
#222244=CARTESIAN_POINT('Ctrl Pts',(72.3593437314497,-4.79486841565966,
134.748291993943));
#222245=CARTESIAN_POINT('Ctrl Pts',(72.0808961076369,0.726397665050741,
136.970210458201));
#222246=CARTESIAN_POINT('Ctrl Pts',(71.8024484838239,5.58013977807825,133.526014137426));
#222247=CARTESIAN_POINT('Ctrl Pts',(71.524000860011,5.30600604003494,127.580751192065));
#222248=CARTESIAN_POINT('Ctrl Pts',(71.2455532361981,0.155911964005252,
124.597827826664));
#222249=CARTESIAN_POINT('Ctrl Pts',(70.9671056123853,-5.13745759022245,
127.318404890117));
#222250=CARTESIAN_POINT('Ctrl Pts',(70.6886579885723,-5.70975459779179,
133.242404968692));
#222251=CARTESIAN_POINT('Ctrl Pts',(70.4102103647595,-1.03506606700937,
136.925961393668));
#222252=CARTESIAN_POINT('Ctrl Pts',(70.1317627409465,4.59079761356593,134.98406576223));
#222253=CARTESIAN_POINT('Ctrl Pts',(69.8533151171337,5.99794256020584,129.201225292793));
#222254=CARTESIAN_POINT('Ctrl Pts',(69.5748674933208,1.89327130980037,124.891587869307));
#222255=CARTESIAN_POINT('Ctrl Pts',(69.2964198695077,-3.95122378286636,
126.015499746463));
#222256=CARTESIAN_POINT('Ctrl Pts',(69.0179722456952,-6.16473724709165,
131.540140815303));
#222257=CARTESIAN_POINT('Ctrl Pts',(68.7395246218819,-2.71315834539685,
136.388635827283));
#222258=CARTESIAN_POINT('Ctrl Pts',(68.4610769980694,3.23168053056381,136.105454728543));
#222259=CARTESIAN_POINT('Ctrl Pts',(68.1826293742561,6.20676287530703,130.950827114659));
#222260=CARTESIAN_POINT('Ctrl Pts',(67.9041817504435,3.47813335486666,125.661603945233));
#222261=CARTESIAN_POINT('Ctrl Pts',(67.6257341266304,-2.44673080243567,
125.09832292005));
#222262=CARTESIAN_POINT('Ctrl Pts',(67.3472865028177,-6.12316888174425,
129.778611783445));
#222263=CARTESIAN_POINT('Ctrl Pts',(67.0688388790048,-4.17271389215982,
135.401513714782));
#222264=CARTESIAN_POINT('Ctrl Pts',(66.7903912551918,1.61226131591331,136.799856533191));
#222265=CARTESIAN_POINT('Ctrl Pts',(66.511943631379,5.91564713800617,132.688631501398));
#222266=CARTESIAN_POINT('Ctrl Pts',(66.233496007566,4.78284223570014,126.845853579115));
#222267=CARTESIAN_POINT('Ctrl Pts',(65.9550483837533,-0.745161026381345,
124.640750241348));
#222268=CARTESIAN_POINT('Ctrl Pts',(65.6766007599402,-5.58839770835831,
128.099703730218));
#222269=CARTESIAN_POINT('Ctrl Pts',(65.3981531361275,-5.2961699047596,134.044104768727));
#222270=CARTESIAN_POINT('Ctrl Pts',(65.1197055123145,-0.137020690970298,
137.011339202618));
#222271=CARTESIAN_POINT('Ctrl Pts',(64.8412578885016,5.14804384398771,134.274663544608));
#222272=CARTESIAN_POINT('Ctrl Pts',(64.5628102646887,5.70230758224426,128.348949030369));
#222273=CARTESIAN_POINT('Ctrl Pts',(64.2843626408759,1.01642922563077,124.679637811238));
#222274=CARTESIAN_POINT('Ctrl Pts',(64.0059150170629,-4.60349793400934,
126.638647641779));
#222275=CARTESIAN_POINT('Ctrl Pts',(63.72746739325,-5.9930353856715,132.425744190676));
#222276=CARTESIAN_POINT('Ctrl Pts',(63.4490197694371,-1.87526609395646,
136.722868444874));
#222277=CARTESIAN_POINT('Ctrl Pts',(63.1705721456243,3.96578112626272,135.581173140958));
#222278=CARTESIAN_POINT('Ctrl Pts',(62.8921245218114,6.16246923062527,130.049820488308));
#222279=CARTESIAN_POINT('Ctrl Pts',(62.6136768979985,2.69614916540168,125.211853353112));
#222280=CARTESIAN_POINT('Ctrl Pts',(62.3352292741856,-3.24780026861702,
125.513127184779));
#222281=CARTESIAN_POINT('Ctrl Pts',(62.0567816503727,-6.20717991964031,
130.676786050054));
#222282=CARTESIAN_POINT('Ctrl Pts',(61.7783340265599,-3.46246446211126,
135.957679710507));
#222283=CARTESIAN_POINT('Ctrl Pts',(61.4998864027468,2.46408668530527,136.502924878181));
#222284=CARTESIAN_POINT('Ctrl Pts',(61.2214387789342,6.12626254625314,131.81146788069));
#222285=CARTESIAN_POINT('Ctrl Pts',(60.942991155121,4.15870241175792,126.194528508313));
#222286=CARTESIAN_POINT('Ctrl Pts',(60.6645435313083,-1.63050207523548,
124.813799641521));
#222287=CARTESIAN_POINT('Ctrl Pts',(60.3860959074953,-5.92135480954196,
128.938103656541));
#222288=CARTESIAN_POINT('Ctrl Pts',(60.1076482836825,-4.77077174814381,
134.777406647022));
#222289=CARTESIAN_POINT('Ctrl Pts',(59.8292006598696,0.763917484641806,
136.965674430521));
#222290=CARTESIAN_POINT('Ctrl Pts',(59.5507530360567,5.59660386848551,133.491995816827));
#222291=CARTESIAN_POINT('Ctrl Pts',(59.2723054122438,5.28628470648961,127.548511753291));
#222292=CARTESIAN_POINT('Ctrl Pts',(58.9938577884309,0.11812814859451,124.596993738963));
#222293=CARTESIAN_POINT('Ctrl Pts',(58.715410164618,-5.15858240697801,127.34974263934));
#222294=CARTESIAN_POINT('Ctrl Pts',(58.4369625408051,-5.69480774129836,
133.277116694236));
#222295=CARTESIAN_POINT('Ctrl Pts',(58.1585149169922,-0.997782968190397,
136.932148715521));
#222296=CARTESIAN_POINT('Ctrl Pts',(57.8800672931793,4.61615560827684,134.956042833877));
#222297=CARTESIAN_POINT('Ctrl Pts',(57.6016196693665,5.98807269247603,129.164743816393));
#222298=CARTESIAN_POINT('Ctrl Pts',(57.3231720455535,1.85724350590365,124.880172539454));
#222299=CARTESIAN_POINT('Ctrl Pts',(57.0447244217407,-3.98030173120474,
126.039640693622));
#222300=CARTESIAN_POINT('Ctrl Pts',(56.7662767979277,-6.16014412588574,
131.577653688385));
#222301=CARTESIAN_POINT('Ctrl Pts',(56.4878291741149,-2.67911500864857,
136.405048128532));
#222302=CARTESIAN_POINT('Ctrl Pts',(56.209381550302,3.26388991949243,136.085684354897));
#222303=CARTESIAN_POINT('Ctrl Pts',(55.9309339264891,6.20753946150667,130.913042073662));
#222304=CARTESIAN_POINT('Ctrl Pts',(55.6524863026762,3.44676349355797,125.640526843659));
#222305=CARTESIAN_POINT('Ctrl Pts',(55.3740386788633,-2.48141974121268,
125.113322584571));
#222306=CARTESIAN_POINT('Ctrl Pts',(55.0955910550504,-6.12929945790263,
129.815904255142));
#222307=CARTESIAN_POINT('Ctrl Pts',(54.8171434312375,-4.14465240570495,
135.426829034002));
#222308=CARTESIAN_POINT('Ctrl Pts',(54.5386958074246,1.64872772980914,136.789931158292));
#222309=CARTESIAN_POINT('Ctrl Pts',(54.2602481836117,5.92700762645589,132.652586367033));
#222310=CARTESIAN_POINT('Ctrl Pts',(53.9818005597989,4.75865706480954,126.81681240286));
#222311=CARTESIAN_POINT('Ctrl Pts',(53.703352935986,-0.78266686607524,124.645400445441));
#222312=CARTESIAN_POINT('Ctrl Pts',(53.4249053121731,-5.604758182439,128.133772004274));
#222313=CARTESIAN_POINT('Ctrl Pts',(53.1464576883601,-5.27635053680027,
134.076284033214));
#222314=CARTESIAN_POINT('Ctrl Pts',(52.8680100645473,-0.0992345118958833,
137.012058285519));
#222315=CARTESIAN_POINT('Ctrl Pts',(52.5895624407343,5.1690731815654,134.243261643865));
#222316=CARTESIAN_POINT('Ctrl Pts',(52.3111148169216,5.68725514443172,128.314282958697));
#222317=CARTESIAN_POINT('Ctrl Pts',(52.0326671931086,0.979127467424884,
124.673563994973));
#222318=CARTESIAN_POINT('Ctrl Pts',(51.7542195692957,-4.62877051910935,
126.666747621346));
#222319=CARTESIAN_POINT('Ctrl Pts',(51.4757719454828,-5.98305452659317,
132.462195457613));
#222320=CARTESIAN_POINT('Ctrl Pts',(51.1973243216699,-1.83920371260068,
136.734174065611));
#222321=CARTESIAN_POINT('Ctrl Pts',(50.9188766978571,3.99478546317524,135.556943802347));
#222322=CARTESIAN_POINT('Ctrl Pts',(50.6404290740441,6.15776195441257,130.012321768865));
#222323=CARTESIAN_POINT('Ctrl Pts',(50.3619814502312,2.66205603294,125.195544744091));
#222324=CARTESIAN_POINT('Ctrl Pts',(50.0835338264184,-3.27994933413751,
125.532995501151));
#222325=CARTESIAN_POINT('Ctrl Pts',(49.8050862026055,-6.20784149757545,
130.714573279694));
#222326=CARTESIAN_POINT('Ctrl Pts',(49.5266385787925,-3.43103059465853,
135.978661235386));
#222327=CARTESIAN_POINT('Ctrl Pts',(49.2481909549797,2.4987298095866,136.487819701939));
#222328=CARTESIAN_POINT('Ctrl Pts',(48.9697433311668,6.13227958855924,131.774156922365));
#222329=CARTESIAN_POINT('Ctrl Pts',(48.6912957073539,4.13056400415832,126.169298715863));
#222330=CARTESIAN_POINT('Ctrl Pts',(48.412848083541,-1.66693811079436,124.823835961664));
#222331=CARTESIAN_POINT('Ctrl Pts',(48.1344004597282,-5.93260553638082,
128.974183201367));
#222332=CARTESIAN_POINT('Ctrl Pts',(47.8559528359152,-4.7464982979263,134.806374077418));
#222333=CARTESIAN_POINT('Ctrl Pts',(47.5775052121024,0.801408996989757,
136.960910093092));
#222334=CARTESIAN_POINT('Ctrl Pts',(47.2990575882894,5.61286057467834,133.457877904919));
#222335=CARTESIAN_POINT('Ctrl Pts',(47.0206099644766,5.26636748772036,127.516392961194));
#222336=CARTESIAN_POINT('Ctrl Pts',(46.7421623406636,0.0803399559020909,
124.596389667526));
#222337=CARTESIAN_POINT('Ctrl Pts',(46.4637147168508,-5.17951607056515,
127.381208400702));
#222338=CARTESIAN_POINT('Ctrl Pts',(46.1852670930379,-5.67964986161014,
133.311736790894));
#222339=CARTESIAN_POINT('Ctrl Pts',(45.9068194692249,-0.960462896156299,
136.938108969933));
#222340=CARTESIAN_POINT('Ctrl Pts',(45.6283718454121,4.64134254964412,134.927866063412));
#222341=CARTESIAN_POINT('Ctrl Pts',(45.3499242215992,5.97798093451044,129.128323096598));
#222342=CARTESIAN_POINT('Ctrl Pts',(45.0714765977863,1.82114688116607,124.868976732569));
#222343=CARTESIAN_POINT('Ctrl Pts',(44.7930289739735,-4.00923218799886,
126.063958199228));
#222344=CARTESIAN_POINT('Ctrl Pts',(44.5145813501605,-6.15532273827383,
131.615137906808));
#222345=CARTESIAN_POINT('Ctrl Pts',(44.2361337263477,-2.644972396308,136.421252894246));
#222346=CARTESIAN_POINT('Ctrl Pts',(43.9576861025347,3.29597836378001,136.065718279858));
#222347=CARTESIAN_POINT('Ctrl Pts',(43.6792384787219,6.20808602504863,130.875253005433));
#222348=CARTESIAN_POINT('Ctrl Pts',(43.4007908549089,3.41526591116036,125.619641089845));
#222349=CARTESIAN_POINT('Ctrl Pts',(43.1223432310961,-2.5160167300689,125.128533132602));
#222350=CARTESIAN_POINT('Ctrl Pts',(42.8438956072832,-6.13520291061547,
129.853233354452));
#222351=CARTESIAN_POINT('Ctrl Pts',(42.5654479834703,-4.11643733763101,
135.451973065955));
#222352=CARTESIAN_POINT('Ctrl Pts',(42.2870003596574,1.68513304949262,136.779783985877));
#222353=CARTESIAN_POINT('Ctrl Pts',(42.0085527358444,5.93814848745852,132.616472745983));
#222354=CARTESIAN_POINT('Ctrl Pts',(41.7301051120316,4.73429556013123,126.787918986671));
#222355=CARTESIAN_POINT('Ctrl Pts',(41.4516574882187,-0.820143703760798,
124.65027887207));
#222356=CARTESIAN_POINT('Ctrl Pts',(41.1732098644058,-5.62091097014408,
128.167939237972));
#222357=CARTESIAN_POINT('Ctrl Pts',(40.8947622405929,-5.25633565173145,
134.108342055376));
#222358=CARTESIAN_POINT('Ctrl Pts',(40.61631461678,-0.0614446556499193,
137.012547339898));
#222359=CARTESIAN_POINT('Ctrl Pts',(40.3378669929672,5.18991097723558,134.211732313379));
#222360=CARTESIAN_POINT('Ctrl Pts',(40.0594193691542,5.67199196328813,128.279709157768));
#222361=CARTESIAN_POINT('Ctrl Pts',(39.7809717453414,0.941789427290636,
124.66771735763));
#222362=CARTESIAN_POINT('Ctrl Pts',(39.5025241215285,-4.65387158341555,
126.695000921683));
#222363=CARTESIAN_POINT('Ctrl Pts',(39.2240764977156,-5.97285196322902,
132.49858529287));
#222364=CARTESIAN_POINT('Ctrl Pts',(38.9456288739027,-1.80307317887526,
136.745259954929));
#222365=CARTESIAN_POINT('Ctrl Pts',(38.6671812500898,4.02364177184326,135.532538355018));
#222366=CARTESIAN_POINT('Ctrl Pts',(38.3887336262769,6.15282650006613,129.974852398711));
#222367=CARTESIAN_POINT('Ctrl Pts',(38.110286002464,2.62786425701304,125.179443971804));
#222368=CARTESIAN_POINT('Ctrl Pts',(37.8318383786511,-3.31197685992897,
125.553059149895));
#222369=CARTESIAN_POINT('Ctrl Pts',(37.5533907548383,-6.20827304166094,
130.752363836438));
#222370=CARTESIAN_POINT('Ctrl Pts',(37.2749431310254,-3.3994695891056,135.999451024653));
#222371=CARTESIAN_POINT('Ctrl Pts',(36.9964955072125,2.53328034251594,136.47250392303));
#222372=CARTESIAN_POINT('Ctrl Pts',(36.7180478833995,6.13806939699002,131.73681002788));
#222373=CARTESIAN_POINT('Ctrl Pts',(36.4396002595867,4.10227253699055,126.144240677337));
#222374=CARTESIAN_POINT('Ctrl Pts',(36.1611526357737,-1.70331237734853,
124.834093892349));
#222375=CARTESIAN_POINT('Ctrl Pts',(35.8827050119609,-5.94363642833981,
129.01033056409));
#222376=CARTESIAN_POINT('Ctrl Pts',(35.604257388148,-4.72204896446884,134.835193211735));
#222377=CARTESIAN_POINT('Ctrl Pts',(35.3258097643351,0.838870812832614,
136.955917622458));
#222378=CARTESIAN_POINT('Ctrl Pts',(35.0473621405222,5.62890929425843,133.423661665951));
#222379=CARTESIAN_POINT('Ctrl Pts',(34.7689145167094,5.24625512176713,127.484396005948));
#222380=CARTESIAN_POINT('Ctrl Pts',(34.4904668928964,0.0425487861828518,
124.596015634733));
#222381=CARTESIAN_POINT('Ctrl Pts',(34.2120192690835,-5.20025780527969,
127.412801008228));
#222382=CARTESIAN_POINT('Ctrl Pts',(33.9335716452707,-5.66428152040741,
133.346263975806));
#222383=CARTESIAN_POINT('Ctrl Pts',(33.6551240214578,-0.923107233816384,
136.943841936043));
#222384=CARTESIAN_POINT('Ctrl Pts',(33.3766763976448,4.66635750435639,134.899536494936));
#222385=CARTESIAN_POINT('Ctrl Pts',(33.098228773832,5.96766766026296,129.091964482989));
#222386=CARTESIAN_POINT('Ctrl Pts',(32.8197811500191,1.78498277316083,124.858000863516));
#222387=CARTESIAN_POINT('Ctrl Pts',(32.5413335262063,-4.03801408121996,
126.08845136219));
#222388=CARTESIAN_POINT('Ctrl Pts',(32.2628859023933,-6.15027326291425,
131.65259208158));
#222389=CARTESIAN_POINT('Ctrl Pts',(31.9844382785804,-2.6107317735426,136.437249523951));
#222390=CARTESIAN_POINT('Ctrl Pts',(31.7059906547675,3.32794467437699,136.045557243275));
#222391=CARTESIAN_POINT('Ctrl Pts',(31.4275430309546,6.20840254567991,130.837461310262));
#222392=CARTESIAN_POINT('Ctrl Pts',(31.1490954071417,3.3836417748287,125.598947457719));
#222393=CARTESIAN_POINT('Ctrl Pts',(30.8706477833288,-2.55052048699994,
125.143954000505));
#222394=CARTESIAN_POINT('Ctrl Pts',(30.5922001595159,-6.14087902112821,
129.890597698133));
#222395=CARTESIAN_POINT('Ctrl Pts',(30.3137525357031,-4.08806973345779,
135.476944878919));
#222396=CARTESIAN_POINT('Ctrl Pts',(30.0353049118902,1.72147592595096,136.769415391952));
#222397=CARTESIAN_POINT('Ctrl Pts',(29.7568572880773,5.94906930818524,132.58029197645));
#222398=CARTESIAN_POINT('Ctrl Pts',(29.4784096642643,4.70975862438989,126.759174401203));
#222399=CARTESIAN_POINT('Ctrl Pts',(29.1999620404515,-0.857590150719802,
124.65538534046));
#222400=CARTESIAN_POINT('Ctrl Pts',(28.9215144166386,-5.63685547292606,
128.202204165235));
#222401=CARTESIAN_POINT('Ctrl Pts',(28.6430667928257,-5.23612599121204,
134.140277647291));
#222402=CARTESIAN_POINT('Ctrl Pts',(28.3646191690128,-0.0236525225496446,
137.012806347637));
#222403=CARTESIAN_POINT('Ctrl Pts',(28.0861715451999,5.2105564588459,134.180076721482));
#222404=CARTESIAN_POINT('Ctrl Pts',(27.807723921387,5.65651860439647,128.245228908728));
#222405=CARTESIAN_POINT('Ctrl Pts',(27.5292762975741,0.904416488802812,
124.662098115861));
#222406=CARTESIAN_POINT('Ctrl Pts',(27.2508286737613,-4.67880019679877,
126.723406495856));
#222407=CARTESIAN_POINT('Ctrl Pts',(26.9723810499484,-5.96242807363892,
132.53491234801));
#222408=CARTESIAN_POINT('Ctrl Pts',(26.6939334261354,-1.76687583160983,
136.756125702037));
#222409=CARTESIAN_POINT('Ctrl Pts',(26.4154858023226,4.05234898298581,135.507957703324));
#222410=CARTESIAN_POINT('Ctrl Pts',(26.1370381785097,6.14766305047102,129.937413766291));
#222411=CARTESIAN_POINT('Ctrl Pts',(25.8585905546968,2.59357510460964,125.163551632871));
#222412=CARTESIAN_POINT('Ctrl Pts',(25.5801429308839,-3.34388165920016,
125.573317387547));
#222413=CARTESIAN_POINT('Ctrl Pts',(25.301695307071,-6.2084745359058,130.790156319941));
#222414=CARTESIAN_POINT('Ctrl Pts',(25.0232476832582,-3.36778261495664,
136.020048307934));
#222415=CARTESIAN_POINT('Ctrl Pts',(24.7448000594452,2.56773700381057,136.456978108987));
#222416=CARTESIAN_POINT('Ctrl Pts',(24.4663524356323,6.14363175700203,131.69942858114));
#222417=CARTESIAN_POINT('Ctrl Pts',(24.1879048118195,4.07382905860539,126.11935532127));
#222418=CARTESIAN_POINT('Ctrl Pts',(23.9094571880065,-1.73962352703587,
124.844573053462));
#222419=CARTESIAN_POINT('Ctrl Pts',(23.6310095641937,-5.95444707666522,
129.046544405257));
#222420=CARTESIAN_POINT('Ctrl Pts',(23.3525619403807,-4.69742465375045,
134.863862982068));
#222421=CARTESIAN_POINT('Ctrl Pts',(23.0741143165679,0.876301544009003,
136.950697203617));
#222422=CARTESIAN_POINT('Ctrl Pts',(22.795666692755,5.64474943253441,133.389348367819));
#222423=CARTESIAN_POINT('Ctrl Pts',(22.5172190689421,5.22594835390121,127.452522073212));
#222424=CARTESIAN_POINT('Ctrl Pts',(22.2387714451292,0.0047560398029127,
124.595871654449));
#222425=CARTESIAN_POINT('Ctrl Pts',(21.9603238213163,-5.22080684252888,
127.444519291243));
#222426=CARTESIAN_POINT('Ctrl Pts',(21.6818761975034,-5.64870328716988,
133.380696969555));
#222427=CARTESIAN_POINT('Ctrl Pts',(21.4034285736905,-0.885717365398449,
136.949347401415));
#222428=CARTESIAN_POINT('Ctrl Pts',(21.1249809498776,4.69119954547528,134.871055178212));
#222429=CARTESIAN_POINT('Ctrl Pts',(20.8465333260648,5.95713325189572,129.055669322849));
#222430=CARTESIAN_POINT('Ctrl Pts',(20.5680857022518,1.74875252196249,124.847245339011));
#222431=CARTESIAN_POINT('Ctrl Pts',(20.289638078439,-4.06664634434428,126.113119274905));
#222432=CARTESIAN_POINT('Ctrl Pts',(20.011190454626,-6.14499588691713,131.690014824823));
#222433=CARTESIAN_POINT('Ctrl Pts',(19.7327428308132,-2.57639440915122,
136.453037424885));
#222434=CARTESIAN_POINT('Ctrl Pts',(19.4542952070003,3.35978766676044,136.025201992224));
#222435=CARTESIAN_POINT('Ctrl Pts',(19.1758475831874,6.20848901167171,130.799668388532));
#222436=CARTESIAN_POINT('Ctrl Pts',(18.8973999593745,3.3518922564065,125.578446714094));
#222437=CARTESIAN_POINT('Ctrl Pts',(18.6189523355616,-2.58492973345636,
125.159584616859));
#222438=CARTESIAN_POINT('Ctrl Pts',(18.3405047117487,-6.14632757911053,
129.927995901635));
#222439=CARTESIAN_POINT('Ctrl Pts',(18.0620570879358,-4.05955064435711,
135.501743547556));
#222440=CARTESIAN_POINT('Ctrl Pts',(17.7836094641229,1.75775501248606,136.758825760728));
#222441=CARTESIAN_POINT('Ctrl Pts',(17.5051618403101,5.95976968396092,132.544045399129));
#222442=CARTESIAN_POINT('Ctrl Pts',(17.2267142164972,4.68504716681072,126.730579711598));
#222443=CARTESIAN_POINT('Ctrl Pts',(16.9482665926842,-0.8950048193604,124.660719661391));
#222444=CARTESIAN_POINT('Ctrl Pts',(16.6698189688713,-5.65259109995534,
128.236565516362));
#222445=CARTESIAN_POINT('Ctrl Pts',(16.3913713450585,-5.21572230411858,
134.172089625574));
#222446=CARTESIAN_POINT('Ctrl Pts',(16.1129237212456,0.0141404870033325,
137.012835299135));
#222447=CARTESIAN_POINT('Ctrl Pts',(15.8344760974327,5.23100886137047,134.148296041183));
#222448=CARTESIAN_POINT('Ctrl Pts',(15.5560284736198,5.64083564112771,128.210843489254));
#222449=CARTESIAN_POINT('Ctrl Pts',(15.2775808498069,0.8670100368296,124.656706477888));
#222450=CARTESIAN_POINT('Ctrl Pts',(14.999133225994,-4.70355543551987,126.751963291284));
#222451=CARTESIAN_POINT('Ctrl Pts',(14.7206856021811,-5.95178324408404,
132.571175276918));
#222452=CARTESIAN_POINT('Ctrl Pts',(14.4422379783683,-1.73061301211068,
136.766770904302));
#222453=CARTESIAN_POINT('Ctrl Pts',(14.1637903545553,4.08090603284655,135.48320275811));
#222454=CARTESIAN_POINT('Ctrl Pts',(13.8853427307424,6.14227179696077,129.900007258904));
#222455=CARTESIAN_POINT('Ctrl Pts',(13.6068951069296,2.55918984632695,125.147868316191));
#222456=CARTESIAN_POINT('Ctrl Pts',(13.3284474831167,-3.37566254970675,
125.593769463429));
#222457=CARTESIAN_POINT('Ctrl Pts',(13.0499998593037,-6.20844597284355,
130.827949329789));
#222458=CARTESIAN_POINT('Ctrl Pts',(12.7715522354909,-3.33597084638438,
136.04045232199));
#222459=CARTESIAN_POINT('Ctrl Pts',(12.493104611678,2.60209851666622,136.441242835124));
#222460=CARTESIAN_POINT('Ctrl Pts',(12.2146569878651,6.14896646247997,131.662013967328));
#222461=CARTESIAN_POINT('Ctrl Pts',(11.9362093640522,4.04523462298623,126.094643569795));
#222462=CARTESIAN_POINT('Ctrl Pts',(11.6577617402393,-1.77587021433397,
124.855273056695));
#222463=CARTESIAN_POINT('Ctrl Pts',(11.3793141164265,-5.96503708076441,
129.08282338295));
#222464=CARTESIAN_POINT('Ctrl Pts',(11.1008664926135,-4.67262627823404,
134.892382326048));
#222465=CARTESIAN_POINT('Ctrl Pts',(10.8224188688007,0.913699803509421,
136.945249030013));
#222466=CARTESIAN_POINT('Ctrl Pts',(10.5439712449878,5.6603804025445,133.354939282016));
#222467=CARTESIAN_POINT('Ctrl Pts',(10.2655236211749,5.20544793659703,127.420772344084));
#222468=CARTESIAN_POINT('Ctrl Pts',(9.98707599736195,-0.0330368828140487,
124.595957732005));
#222469=CARTESIAN_POINT('Ctrl Pts',(9.70862837354909,-5.24116242086055,
127.476362074414));
#222470=CARTESIAN_POINT('Ctrl Pts',(9.43018074973619,-5.63291573915475,
133.415034496211));
#222471=CARTESIAN_POINT('Ctrl Pts',(9.15173312592329,-0.848294676398009,
136.954625162043));
#222472=CARTESIAN_POINT('Ctrl Pts',(8.87328550211039,4.71586775246963,134.842423168626));
#222473=CARTESIAN_POINT('Ctrl Pts',(8.59483787829755,5.94637809976527,129.019438961107));
#222474=CARTESIAN_POINT('Ctrl Pts',(8.3163902544846,1.71245747009635,124.836710557603));
#222475=CARTESIAN_POINT('Ctrl Pts',(8.03794263067172,-4.09512791639282,
126.137961023291));
#222476=CARTESIAN_POINT('Ctrl Pts',(7.75949500685887,-6.1394908058375,131.727404749824));
#222477=CARTESIAN_POINT('Ctrl Pts',(7.48104738304595,-2.54196157551782,
136.468616012024));
#222478=CARTESIAN_POINT('Ctrl Pts',(7.20259975923305,3.39150616097622,136.004653280976));
#222479=CARTESIAN_POINT('Ctrl Pts',(6.92415213542018,6.20834541982004,130.761875640674));
#222480=CARTESIAN_POINT('Ctrl Pts',(6.64570451160728,3.32001853238404,125.558139618628));
#222481=CARTESIAN_POINT('Ctrl Pts',(6.36725688779438,-2.61924319439064,
125.175424402463));
#222482=CARTESIAN_POINT('Ctrl Pts',(6.08880926398148,-6.15154838266407,
129.965426579154));
#222483=CARTESIAN_POINT('Ctrl Pts',(5.81036164016863,-4.03088112711464,
135.52636815294));
#222484=CARTESIAN_POINT('Ctrl Pts',(5.53191401635571,1.79396896476278,136.748015484609));
#222485=CARTESIAN_POINT('Ctrl Pts',(5.2534663925428,5.97024921827925,132.507734357147));
#222486=CARTESIAN_POINT('Ctrl Pts',(4.97501876872993,4.66016210308585,126.702135977443));
#222487=CARTESIAN_POINT('Ctrl Pts',(4.69657114491704,-0.932386323268277,
124.666281637197));
#222488=CARTESIAN_POINT('Ctrl Pts',(4.41812352110413,-5.66811726814286,
128.27102201808));
#222489=CARTESIAN_POINT('Ctrl Pts',(4.13967589729124,-5.19512534651691,
134.203776811419));
#222490=CARTESIAN_POINT('Ctrl Pts',(3.86122827347838,0.051932972575587,
137.012634193321));
#222491=CARTESIAN_POINT('Ctrl Pts',(3.58278064966546,5.25126742693796,134.116391450127));
#222492=CARTESIAN_POINT('Ctrl Pts',(3.30433302585255,5.62494365461986,128.176554173511));
#222493=CARTESIAN_POINT('Ctrl Pts',(3.02588540203969,0.829571457480427,
124.651542643499));
#222494=CARTESIAN_POINT('Ctrl Pts',(2.74743777822681,-4.72813638226476,
126.780670249786));
#222495=CARTESIAN_POINT('Ctrl Pts',(2.46899015441389,-5.9409178690121,132.607372735859));
#222496=CARTESIAN_POINT('Ctrl Pts',(2.19054253060099,-1.69428606410994,
136.77719516726));
#222497=CARTESIAN_POINT('Ctrl Pts',(1.91209490678813,4.10931186323347,135.458274436681));
#222498=CARTESIAN_POINT('Ctrl Pts',(1.63364728297522,6.13665293931019,129.862634262664));
#222499=CARTESIAN_POINT('Ctrl Pts',(1.35519965916232,2.52470975632363,125.132394602912));
#222500=CARTESIAN_POINT('Ctrl Pts',(1.07675203534945,-3.40731835379603,
125.614414619682));
#222501=CARTESIAN_POINT('Ctrl Pts',(0.798304411536565,-6.20818735353264,
130.86574146555));
#222502=CARTESIAN_POINT('Ctrl Pts',(0.519856787723634,-3.30403546218559,
136.060662310741));
#222503=CARTESIAN_POINT('Ctrl Pts',(0.241409163910791,2.63636360780418,
136.425298684517));
#222504=CARTESIAN_POINT('Ctrl Pts',(-0.0370384599021062,6.15407331574431,
131.624567572855));
#222505=CARTESIAN_POINT('Ctrl Pts',(-0.315486083715014,4.01649028971072,
126.070106338619));
#222506=CARTESIAN_POINT('Ctrl Pts',(-0.593933707527915,-1.81205109610819,
124.866193505555));
#222507=CARTESIAN_POINT('Ctrl Pts',(-0.872381331340776,-5.97540604822092,
129.119166152838));
#222508=CARTESIAN_POINT('Ctrl Pts',(-1.15082895515369,-4.6476547568326,
134.920750186879));
#222509=CARTESIAN_POINT('Ctrl Pts',(-1.42927657896659,0.951064205527318,
136.939573303531));
#222510=CARTESIAN_POINT('Ctrl Pts',(-1.70772420277945,5.67580162507719,
133.320435683583));
#222511=CARTESIAN_POINT('Ctrl Pts',(-1.98617182659235,5.18475462950527,
127.389147995065));
#222512=CARTESIAN_POINT('Ctrl Pts',(-2.26461945040527,-0.0708285812371651,
124.596273864213));
#222513=CARTESIAN_POINT('Ctrl Pts',(-2.54306707421816,-5.26132378599129,
127.508328177794));
#222514=CARTESIAN_POINT('Ctrl Pts',(-2.82151469803103,-5.61691946137538,
133.449275283389));
#222515=CARTESIAN_POINT('Ctrl Pts',(-3.09996232184393,-0.810840553526189,
136.959675022356));
#222516=CARTESIAN_POINT('Ctrl Pts',(-3.37840994565684,4.74036121125036,
134.813641527147));
#222517=CARTESIAN_POINT('Ctrl Pts',(-3.6568575694697,5.93540260240737,128.983274740293));
#222518=CARTESIAN_POINT('Ctrl Pts',(-3.9353051932826,1.6760989624889,124.826396909662));
#222519=CARTESIAN_POINT('Ctrl Pts',(-4.21375281709551,-4.12345774197041,
126.162975686831));
#222520=CARTESIAN_POINT('Ctrl Pts',(-4.49220044090841,-6.13375822366836,
131.764760471086));
#222521=CARTESIAN_POINT('Ctrl Pts',(-4.77064806472125,-2.50743454856317,
136.483984708096));
#222522=CARTESIAN_POINT('Ctrl Pts',(-5.04909568853418,3.4230989816841,135.983911870971));
#222523=CARTESIAN_POINT('Ctrl Pts',(-5.32754331234708,6.20797177544568,
130.724084467112));
#222524=CARTESIAN_POINT('Ctrl Pts',(-5.60599093615995,3.28802178385396,
125.538026923812));
#222525=CARTESIAN_POINT('Ctrl Pts',(-5.88443855997284,-2.65345959830539,
125.191472770368));
#222526=CARTESIAN_POINT('Ctrl Pts',(-6.16288618378574,-6.15654123833006,
130.002888343683));
#222527=CARTESIAN_POINT('Ctrl Pts',(-6.44133380759864,-4.00206224408943,
135.550817782599));
#222528=CARTESIAN_POINT('Ctrl Pts',(-6.71978143141151,1.83011644085978,
136.736984964173));
#222529=CARTESIAN_POINT('Ctrl Pts',(-6.9982290552244,5.98050752281724,132.471360196026));
#222530=CARTESIAN_POINT('Ctrl Pts',(-7.27667667903734,4.63510435534053,
126.673844252731));
#222531=CARTESIAN_POINT('Ctrl Pts',(-7.55512430285017,-0.969733277257762,
124.672071061776));
#222532=CARTESIAN_POINT('Ctrl Pts',(-7.83357192666308,-5.68343340216059,
128.305572393592));
#222533=CARTESIAN_POINT('Ctrl Pts',(-8.112019550476,-5.17433588163501,134.235338030648));
#222534=CARTESIAN_POINT('Ctrl Pts',(-8.39046717428886,0.0897235337524442,
137.012203037646));
#222535=CARTESIAN_POINT('Ctrl Pts',(-8.66891479810176,5.27133140485959,
134.084364130551));
#222536=CARTESIAN_POINT('Ctrl Pts',(-8.94736242191464,5.60884323375645,
128.142362232103));
#222537=CARTESIAN_POINT('Ctrl Pts',(-9.22581004572757,0.792102138056052,
124.646606804043));
#222538=CARTESIAN_POINT('Ctrl Pts',(-9.50425766954039,-4.75254212617725,
126.809526307613));
#222539=CARTESIAN_POINT('Ctrl Pts',(-9.78270529335335,-5.92983235104376,
132.643503383524));
#222540=CARTESIAN_POINT('Ctrl Pts',(-10.0611529171662,-1.65789633371603,
136.787398104638));
#222541=CARTESIAN_POINT('Ctrl Pts',(-10.3396005409791,4.13756542155812,
135.433173662763));
#222542=CARTESIAN_POINT('Ctrl Pts',(-10.618048164792,6.13080668572826,129.82529616244));
#222543=CARTESIAN_POINT('Ctrl Pts',(-10.8964957886049,2.49013611227157,
125.11713106642));
#222544=CARTESIAN_POINT('Ctrl Pts',(-11.1749434124178,-3.4388478984508,
125.635252091294));
#222545=CARTESIAN_POINT('Ctrl Pts',(-11.4533910362307,-6.20769868755626,
130.90353132682));
#222546=CARTESIAN_POINT('Ctrl Pts',(-11.7318386600436,-3.2719776457377,
136.080677525301));
#222547=CARTESIAN_POINT('Ctrl Pts',(-12.0102862838565,2.67053100751937,
136.409146247984));
#222548=CARTESIAN_POINT('Ctrl Pts',(-12.2887339076694,6.15895212755882,
131.587090785312));
#222549=CARTESIAN_POINT('Ctrl Pts',(-12.5671815314823,3.98759712391021,
126.045744536976));
#222550=CARTESIAN_POINT('Ctrl Pts',(-12.8456291552951,-1.84816483166266,
124.877333995382));
#222551=CARTESIAN_POINT('Ctrl Pts',(-13.1240767791081,-5.98555359480885,
129.155571368227));
#222552=CARTESIAN_POINT('Ctrl Pts',(-13.4025244029209,-4.62251101487491,
134.948965513381));
#222553=CARTESIAN_POINT('Ctrl Pts',(-13.6809720267338,0.988393365511613,
136.933670234486));
#222554=CARTESIAN_POINT('Ctrl Pts',(-13.9594196505467,5.69101252869335,
133.285838851062));
#222555=CARTESIAN_POINT('Ctrl Pts',(-14.2378672743596,5.16386919942402,
127.357650198006));
#222556=CARTESIAN_POINT('Ctrl Pts',(-14.5163148981725,-0.108617655081171,
124.59682003936));
#222557=CARTESIAN_POINT('Ctrl Pts',(-14.7947625219854,-5.28129019083405,
127.540416416869));
#222558=CARTESIAN_POINT('Ctrl Pts',(-15.0732101457983,-5.60071504657988,
133.483418062279));
#222559=CARTESIAN_POINT('Ctrl Pts',(-15.3516577696111,-0.77335638465969,
136.96449679523));
#222560=CARTESIAN_POINT('Ctrl Pts',(-15.6301053934241,4.76467901420313,
134.784711320289));
#222561=CARTESIAN_POINT('Ctrl Pts',(-15.908553017237,5.92420716652329,128.947178000488));
#222562=CARTESIAN_POINT('Ctrl Pts',(-16.1870006410499,1.63967834641818,
124.816304777366));
#222563=CARTESIAN_POINT('Ctrl Pts',(-16.4654482648627,-4.15163477130477,
126.188162338596));
#222564=CARTESIAN_POINT('Ctrl Pts',(-16.7438958886757,-6.12779835283271,
131.802080604377));
#222565=CARTESIAN_POINT('Ctrl Pts',(-17.0223435124885,-2.4728146076992,
136.499142943608));
#222566=CARTESIAN_POINT('Ctrl Pts',(-17.3007911363014,3.45456495820035,
135.96297853079));
#222567=CARTESIAN_POINT('Ctrl Pts',(-17.5792387601143,6.20736809239421,
130.686296268213));
#222568=CARTESIAN_POINT('Ctrl Pts',(-17.8576863839272,3.25590319646751,
125.518109374927));
#222569=CARTESIAN_POINT('Ctrl Pts',(-18.13613400774,-2.6875776772989,125.207729125896));
#222570=CARTESIAN_POINT('Ctrl Pts',(-18.414581631553,-6.16130596109642,
130.040379807061));
#222571=CARTESIAN_POINT('Ctrl Pts',(-18.6930292553659,-3.97309506317598,
135.575091530542));
#222572=CARTESIAN_POINT('Ctrl Pts',(-18.9714768791788,1.86619610131902,
136.72573460816));
#222573=CARTESIAN_POINT('Ctrl Pts',(-19.2499245029916,5.99054421744964,
132.434924263623));
#222574=CARTESIAN_POINT('Ctrl Pts',(-19.5283721268046,4.6098748520987,126.645705585822));
#222575=CARTESIAN_POINT('Ctrl Pts',(-19.8068197506174,-1.00704429742433,
124.678087720601));
#222576=CARTESIAN_POINT('Ctrl Pts',(-20.0852673744304,-5.6985389344635,
128.340215362621));
#222577=CARTESIAN_POINT('Ctrl Pts',(-20.3637149982432,-5.15335467983417,
134.266772113748));
#222578=CARTESIAN_POINT('Ctrl Pts',(-20.6421626220562,0.127510770190762,
137.011541848088));
#222579=CARTESIAN_POINT('Ctrl Pts',(-20.920610245869,5.29120005165768,134.05221526924));
#222580=CARTESIAN_POINT('Ctrl Pts',(-21.1990578696819,5.59253497514422,
128.108268932023));
#222581=CARTESIAN_POINT('Ctrl Pts',(-21.4775054934948,0.754603466995427,
124.64189914242));
#222582=CARTESIAN_POINT('Ctrl Pts',(-21.7559531173077,-4.77677176289349,
126.838530395495));
#222583=CARTESIAN_POINT('Ctrl Pts',(-22.0344007411205,-5.91852710095694,
132.679565881077));
#222584=CARTESIAN_POINT('Ctrl Pts',(-22.3128483649335,-1.62144516936395,
136.797379338361));
#222585=CARTESIAN_POINT('Ctrl Pts',(-22.5912959887463,4.16566566087426,
135.407901366475));
#222586=CARTESIAN_POINT('Ctrl Pts',(-22.8697436125593,6.12473325285015,
129.787994341809));
#222587=CARTESIAN_POINT('Ctrl Pts',(-23.1481912363721,2.45547019531011,
125.102078272311));
#222588=CARTESIAN_POINT('Ctrl Pts',(-23.426638860185,-3.47025001533206,
125.656281106122));
#222589=CARTESIAN_POINT('Ctrl Pts',(-23.7050864839979,-6.20697999302203,
130.941317513284));
#222590=CARTESIAN_POINT('Ctrl Pts',(-23.9835341078108,-3.23979858495512,
136.100497223997));
#222591=CARTESIAN_POINT('Ctrl Pts',(-24.2619817316237,2.70459944972584,
136.392786124057));
#222592=CARTESIAN_POINT('Ctrl Pts',(-24.5404293554366,6.16360271713728,
131.549584993415));
#222593=CARTESIAN_POINT('Ctrl Pts',(-24.8188769792495,3.95855619623184,
126.021559067602));
#222594=CARTESIAN_POINT('Ctrl Pts',(-25.0973246030624,-1.88421008278963,
124.88869411336));
#222595=CARTESIAN_POINT('Ctrl Pts',(-25.3757722268753,-5.99547934450715,
129.192037680109));
#222596=CARTESIAN_POINT('Ctrl Pts',(-25.6542198506882,-4.59719598407162,
134.977027260026));
#222597=CARTESIAN_POINT('Ctrl Pts',(-25.932667474501,1.02568590021626,136.92754004162));
#222598=CARTESIAN_POINT('Ctrl Pts',(-26.211115098314,5.7060125497474,133.251150066453));
#222599=CARTESIAN_POINT('Ctrl Pts',(-26.4895627221268,5.14279242027056,
127.326280120068));
#222600=CARTESIAN_POINT('Ctrl Pts',(-26.7680103459397,-0.146402704058008,
124.597596237205));
#222601=CARTESIAN_POINT('Ctrl Pts',(-27.0464579697526,-5.30106089552683,
127.572625602596));
#222602=CARTESIAN_POINT('Ctrl Pts',(-27.3249055935655,-5.58430309522854,
133.517461567711));
#222603=CARTESIAN_POINT('Ctrl Pts',(-27.6033532173784,-0.735843558787732,
136.969090301993));
#222604=CARTESIAN_POINT('Ctrl Pts',(-27.8818008411913,4.78882026022281,
134.755633620073));
#222605=CARTESIAN_POINT('Ctrl Pts',(-28.1602484650042,5.91279220696403,
128.911150079267));
#222606=CARTESIAN_POINT('Ctrl Pts',(-28.4386960888171,1.60319697146318,
124.806434534681));
#222607=CARTESIAN_POINT('Ctrl Pts',(-28.7171437126299,-4.17965796028613,
126.213520045287));
#222608=CARTESIAN_POINT('Ctrl Pts',(-28.9955913364429,-6.12161141417542,
131.839363766787));
#222609=CARTESIAN_POINT('Ctrl Pts',(-29.2740389602557,-2.43810303578058,
136.514090156867));
#222610=CARTESIAN_POINT('Ctrl Pts',(-29.5524865840687,3.48590292454168,
135.941854036124));
#222611=CARTESIAN_POINT('Ctrl Pts',(-29.8309342078815,6.20653439303521,
130.648512444231));
#222612=CARTESIAN_POINT('Ctrl Pts',(-30.1093818316944,3.22366396039099,
125.498387710026));
#222613=CARTESIAN_POINT('Ctrl Pts',(-30.3878294555073,-2.72159616711309,
125.224192866663));
#222614=CARTESIAN_POINT('Ctrl Pts',(-30.6662770793202,-6.16584237440457,
130.077899580028));
#222615=CARTESIAN_POINT('Ctrl Pts',(-30.9447247031331,-3.94398065776386,
135.599188497297));
#222616=CARTESIAN_POINT('Ctrl Pts',(-31.2231723269461,1.90220660919519,
136.714264833456));
#222617=CARTESIAN_POINT('Ctrl Pts',(-31.5016199507588,6.00035893026297,
132.398427910084));
#222618=CARTESIAN_POINT('Ctrl Pts',(-31.7800675745718,4.58447452824918,
126.617721019404));
#222619=CARTESIAN_POINT('Ctrl Pts',(-32.0585151983846,-1.04431800119413,
124.68433139072));
#222620=CARTESIAN_POINT('Ctrl Pts',(-32.3369628221976,-5.71343330531054,
128.374949641459));
#222621=CARTESIAN_POINT('Ctrl Pts',(-32.6154104460104,-5.1321825185805,
134.298077895915));
#222622=CARTESIAN_POINT('Ctrl Pts',(-32.8938580698234,0.165293281670594,
137.010650649146));
#222623=CARTESIAN_POINT('Ctrl Pts',(-33.1723056936362,5.31087263109202,
134.019946057479));
#222624=CARTESIAN_POINT('Ctrl Pts',(-33.4507533174492,5.57601948309184,
128.074275536613));
#222625=CARTESIAN_POINT('Ctrl Pts',(-33.729200941262,0.717076833825826,
124.637419833072));
#222626=CARTESIAN_POINT('Ctrl Pts',(-34.0076485650749,-4.80082439457541,
126.867681438675));
#222627=CARTESIAN_POINT('Ctrl Pts',(-34.2860961888878,-5.90700253767186,
132.715558892209));
#222628=CARTESIAN_POINT('Ctrl Pts',(-34.5645438127007,-1.58493392176466,
136.807138498572));
#222629=CARTESIAN_POINT('Ctrl Pts',(-34.8429914365135,4.19361153991761,
135.382458484293));
#222630=CARTESIAN_POINT('Ctrl Pts',(-35.1214390603265,6.11843286572883,
129.750730183006));
#222631=CARTESIAN_POINT('Ctrl Pts',(-35.3998866841394,2.42071328999757,
125.087236778371));
#222632=CARTESIAN_POINT('Ctrl Pts',(-35.6783343079523,-3.50152354082281,
125.677500884929));
#222633=CARTESIAN_POINT('Ctrl Pts',(-35.9567819317651,-6.20603129656164,
130.979098624759));
#222634=CARTESIAN_POINT('Ctrl Pts',(-36.2352295555781,-3.2074994722443,
136.120120672404));
#222635=CARTESIAN_POINT('Ctrl Pts',(-36.5136771793909,2.73856767200523,
136.376218918968));
#222636=CARTESIAN_POINT('Ctrl Pts',(-36.7921248032039,6.1680249121504,131.512051586954));
#222637=CARTESIAN_POINT('Ctrl Pts',(-37.0705724270167,3.92936858279784,
125.997550826698));
#222638=CARTESIAN_POINT('Ctrl Pts',(-37.3490200508296,-1.92018551381882,
124.900273438536));
#222639=CARTESIAN_POINT('Ctrl Pts',(-37.6274676746425,-6.00518292951342,
129.228563737208));
#222640=CARTESIAN_POINT('Ctrl Pts',(-37.9059152984554,-4.57171060248077,
135.004934386972));
#222641=CARTESIAN_POINT('Ctrl Pts',(-38.1843629222683,1.0629404277527,136.921182952087));
#222642=CARTESIAN_POINT('Ctrl Pts',(-38.4628105460811,5.72080113240803,
133.216370615161));
#222643=CARTESIAN_POINT('Ctrl Pts',(-38.7412581698941,5.12152507305273,
127.295038923683));
#222644=CARTESIAN_POINT('Ctrl Pts',(-39.0197057937069,-0.184182328028525,
124.598602428988));
#222645=CARTESIAN_POINT('Ctrl Pts',(-39.2981534175199,-5.32063516745863,
127.604954541453));
#222646=CARTESIAN_POINT('Ctrl Pts',(-39.5766010413327,-5.56768421547239,
133.55140453819));
#222647=CARTESIAN_POINT('Ctrl Pts',(-39.8550486651457,-0.698303465962086,
136.973455372429));
#222648=CARTESIAN_POINT('Ctrl Pts',(-40.1334962889585,4.81278405474664,
134.726409503982));
#222649=CARTESIAN_POINT('Ctrl Pts',(-40.4119439127715,5.90115814671511,
128.875192311658));
#222650=CARTESIAN_POINT('Ctrl Pts',(-40.6903915365843,1.56665618945481,
124.796786547352));
#222651=CARTESIAN_POINT('Ctrl Pts',(-40.9688391603973,-4.20752627050468,
126.239047867263));
#222652=CARTESIAN_POINT('Ctrl Pts',(-41.2472867842101,-6.11519763695597,
131.876608576776));
#222653=CARTESIAN_POINT('Ctrl Pts',(-41.5257344080229,-2.40330111905734,
136.528825793999));
#222654=CARTESIAN_POINT('Ctrl Pts',(-41.8041820318359,3.51711171946819,
135.920539169751));
#222655=CARTESIAN_POINT('Ctrl Pts',(-42.0826296556488,6.20547070826194,
130.610734395262));
#222656=CARTESIAN_POINT('Ctrl Pts',(-42.3610772794617,3.19130527026066,
125.478862659902));
#222657=CARTESIAN_POINT('Ctrl Pts',(-42.6395249032745,-2.75551380718057,
125.240863382598));
#222658=CARTESIAN_POINT('Ctrl Pts',(-42.9179725270875,-6.17015031015604,
130.115446272278));
#222659=CARTESIAN_POINT('Ctrl Pts',(-43.1964201509003,-3.91472010669807,
135.623107789941));
#222660=CARTESIAN_POINT('Ctrl Pts',(-43.4748677747133,1.93814663010615,
136.702576065077));
#222661=CARTESIAN_POINT('Ctrl Pts',(-43.7533153985261,6.00995129756958,
132.361872487794));
#222662=CARTESIAN_POINT('Ctrl Pts',(-44.031763022339,4.55890432500984,126.589891590455));
#222663=CARTESIAN_POINT('Ctrl Pts',(-44.3102106461518,-1.08155300737633,
124.690801840773));
#222664=CARTESIAN_POINT('Ctrl Pts',(-44.5886582699649,-5.72811596278534,
128.409773943013));
#222665=CARTESIAN_POINT('Ctrl Pts',(-44.8671058937777,-5.11082018241628,
134.329254217104));
#222666=CARTESIAN_POINT('Ctrl Pts',(-45.1455535175906,0.2030696681468,137.009529473845));
#222667=CARTESIAN_POINT('Ctrl Pts',(-45.4240011414034,5.33034841418793,
133.987557691017));
#222668=CARTESIAN_POINT('Ctrl Pts',(-45.7024487652165,5.55929736958694,
128.040383305508));
#222669=CARTESIAN_POINT('Ctrl Pts',(-45.9808963890292,0.679523629110432,
124.633169041983));
#222670=CARTESIAN_POINT('Ctrl Pts',(-46.2593440128422,-4.82469912994364,
126.896978356949));
#222671=CARTESIAN_POINT('Ctrl Pts',(-46.537791636655,-5.89525908823553,
132.751481083186));
#222672=CARTESIAN_POINT('Ctrl Pts',(-46.816239260468,-1.54836394385628,
136.816675223641));
#222673=CARTESIAN_POINT('Ctrl Pts',(-47.0946868842807,4.22140202314317,
135.35684595901));
#222674=CARTESIAN_POINT('Ctrl Pts',(-47.3731345080937,6.11190575782758,
129.713505066864));
#222675=CARTESIAN_POINT('Ctrl Pts',(-47.6515821319066,2.38586668426401,
125.072607134557));
#222676=CARTESIAN_POINT('Ctrl Pts',(-47.9300297557195,-3.53266731607082,
125.69891064141));
#222677=CARTESIAN_POINT('Ctrl Pts',(-48.2084773795324,-6.20485263332943,
131.016873261253));
#222678=CARTESIAN_POINT('Ctrl Pts',(-48.4869250033452,-3.17508150446096,
136.139547143367));
#222679=CARTESIAN_POINT('Ctrl Pts',(-48.7653726271582,2.77243441565242,
136.359445246621));
#222680=CARTESIAN_POINT('Ctrl Pts',(-49.043820250971,6.1722185487321,131.474491956744));
#222681=CARTESIAN_POINT('Ctrl Pts',(-49.322267874784,3.900035365166,125.973720703898));
#222682=CARTESIAN_POINT('Ctrl Pts',(-49.6007154985968,-1.95608979166789,
124.912071541833));
#222683=CARTESIAN_POINT('Ctrl Pts',(-49.8791631224098,-6.0146639902579,
129.265148186042));
#222684=CARTESIAN_POINT('Ctrl Pts',(-50.1576107462225,-4.54605581447205,
135.032685860113));
#222685=CARTESIAN_POINT('Ctrl Pts',(-50.4360583700356,1.10015556764067,
136.914599201455));
#222686=CARTESIAN_POINT('Ctrl Pts',(-50.7145059938484,5.73537772867887,
133.181501785951));
#222687=CARTESIAN_POINT('Ctrl Pts',(-50.9929536176612,5.10006794583985,
127.263927766504));
#222688=CARTESIAN_POINT('Ctrl Pts',(-51.2714012414742,-0.221955127055423,
124.599838577421));
#222689=CARTESIAN_POINT('Ctrl Pts',(-51.5498488652871,-5.34001228129766,
127.637402035479));
#222690=CARTESIAN_POINT('Ctrl Pts',(-51.8282964891,-5.5508590231301,133.585245715947));
#222691=CARTESIAN_POINT('Ctrl Pts',(-52.1067441129128,-0.660737497244709,
136.977591844792));
#222692=CARTESIAN_POINT('Ctrl Pts',(-52.3851917367258,4.8365695097872,134.697040054928));
#222693=CARTESIAN_POINT('Ctrl Pts',(-52.6636393605386,5.889305416881,128.83930603009));
#222694=CARTESIAN_POINT('Ctrl Pts',(-52.9420869843516,1.53005735442545,
124.78736117289));
#222695=CARTESIAN_POINT('Ctrl Pts',(-53.2205346081644,-4.23523866929,126.264744858582));
#222696=CARTESIAN_POINT('Ctrl Pts',(-53.4989822319774,-6.1085572588392,
131.913813654221));
#222697=CARTESIAN_POINT('Ctrl Pts',(-53.7774298557902,-2.36841014712749,
136.543349308967));
#222698=CARTESIAN_POINT('Ctrl Pts',(-54.0558774796031,3.54819018652628,
135.8990347215));
#222699=CARTESIAN_POINT('Ctrl Pts',(-54.334325103416,6.20417707748961,130.572963521183));
#222700=CARTESIAN_POINT('Ctrl Pts',(-54.6127727272289,3.15882832513996,
125.459534948064));
#222701=CARTESIAN_POINT('Ctrl Pts',(-54.8912203510417,-2.7893293406706,
125.257740055968));
#222702=CARTESIAN_POINT('Ctrl Pts',(-55.1696679748547,-6.17422960871856,
130.153018492501));
#222703=CARTESIAN_POINT('Ctrl Pts',(-55.4481155986676,-3.88531449423931,
135.646848522136));
#222704=CARTESIAN_POINT('Ctrl Pts',(-55.7265632224805,1.97401483228084,
136.690668736158));
#222705=CARTESIAN_POINT('Ctrl Pts',(-56.0050108462934,6.01932096392068,
132.32525935133));
#222706=CARTESIAN_POINT('Ctrl Pts',(-56.2834584701062,4.53316518989421,
126.562218330207));
#222707=CARTESIAN_POINT('Ctrl Pts',(-56.5619060939192,-1.11874793621411,
124.697498830995));
#222708=CARTESIAN_POINT('Ctrl Pts',(-56.840353717732,-5.74258636281662,
128.444686976857));
#222709=CARTESIAN_POINT('Ctrl Pts',(-57.118801341545,-5.08926846293066,
134.360299922064));
#222710=CARTESIAN_POINT('Ctrl Pts',(-57.3972489653578,0.240838529802063,
137.00817836373));
#222711=CARTESIAN_POINT('Ctrl Pts',(-57.6756965891708,5.34962667926312,
133.955051370017));
#222712=CARTESIAN_POINT('Ctrl Pts',(-57.9541442129836,5.54236925427356,
128.0065934946));
#222713=CARTESIAN_POINT('Ctrl Pts',(-58.2325918367966,0.641945244397073,
124.629146926667));
#222714=CARTESIAN_POINT('Ctrl Pts',(-58.5110394606094,-4.84839508431156,
126.92642006471));
#222715=CARTESIAN_POINT('Ctrl Pts',(-58.7894870844223,-5.88329718780563,
132.787331122898));
#222716=CARTESIAN_POINT('Ctrl Pts',(-59.0679347082352,-1.5117365907523,
136.825989160181));
#222717=CARTESIAN_POINT('Ctrl Pts',(-59.3463823320481,4.24903608076433,
135.331064739709));
#222718=CARTESIAN_POINT('Ctrl Pts',(-59.624829955861,6.10515217101086,129.676320372777));
#222719=CARTESIAN_POINT('Ctrl Pts',(-59.9032775796738,2.3509316693629,125.058189882977));
#222720=CARTESIAN_POINT('Ctrl Pts',(-60.1817252034868,-3.56368018703254,
125.720509582217));
#222721=CARTESIAN_POINT('Ctrl Pts',(-60.4601728272995,-6.20344404700091,
131.054640023013));
#222722=CARTESIAN_POINT('Ctrl Pts',(-60.7386204511126,-3.14254588286485,
136.158775917031));
#222723=CARTESIAN_POINT('Ctrl Pts',(-61.0170680749254,2.80619842572279,
136.342465728569));
#222724=CARTESIAN_POINT('Ctrl Pts',(-61.2955156987383,6.17618347148551,
131.436907494571));
#222725=CARTESIAN_POINT('Ctrl Pts',(-61.5739633225512,3.87055763028967,
125.950069582238));
#222726=CARTESIAN_POINT('Ctrl Pts',(-61.8524109463641,-1.9919215858902,
124.924087986069));
#222727=CARTESIAN_POINT('Ctrl Pts',(-62.130858570177,-6.02392217541635,
129.301789670958));
#222728=CARTESIAN_POINT('Ctrl Pts',(-62.4093061939898,-4.5202325706933,
135.060280651108));
#222729=CARTESIAN_POINT('Ctrl Pts',(-62.6877538178028,1.13732994085927,
136.907789033684));
#222730=CARTESIAN_POINT('Ctrl Pts',(-62.9662014416156,5.74974179841868,
133.146544870902));
#222731=CARTESIAN_POINT('Ctrl Pts',(-63.2446490654287,5.0784218337339,127.232947801366));
#222732=CARTESIAN_POINT('Ctrl Pts',(-63.5230966892413,-0.25971970145348,
124.601304636701));
#222733=CARTESIAN_POINT('Ctrl Pts',(-63.8015443130544,-5.3591915190178,
127.669966882319));
#222734=CARTESIAN_POINT('Ctrl Pts',(-64.0799919368672,-5.53382814166538,
133.618983846983));
#222735=CARTESIAN_POINT('Ctrl Pts',(-64.3584395606801,-0.623147044656387,
136.9814995658));
#222736=CARTESIAN_POINT('Ctrl Pts',(-64.636887184493,4.86017574396616,134.667526361205));
#222737=CARTESIAN_POINT('Ctrl Pts',(-64.9153348083059,5.8772344566688,128.803492564343));
#222738=CARTESIAN_POINT('Ctrl Pts',(-65.1937824321189,1.4934018225579,124.778158760555));
#222739=CARTESIAN_POINT('Ctrl Pts',(-65.4722300559316,-4.26279412974889,
126.290610067033));
#222740=CARTESIAN_POINT('Ctrl Pts',(-65.7506776797446,-6.10169052588679,
131.950977620477));
#222741=CARTESIAN_POINT('Ctrl Pts',(-66.0291253035574,-2.33343141288849,
136.5576601636));
#222742=CARTESIAN_POINT('Ctrl Pts',(-66.3075729273703,3.57913717409239,
135.877341488227));
#222743=CARTESIAN_POINT('Ctrl Pts',(-66.5860205511832,6.20265354865397,
130.535201221608));
#222744=CARTESIAN_POINT('Ctrl Pts',(-66.8644681749961,3.126234328474,125.440405290707));
#222745=CARTESIAN_POINT('Ctrl Pts',(-67.142915798809,-2.82304151453613,
125.274822261403));
#222746=CARTESIAN_POINT('Ctrl Pts',(-67.421363422622,-6.17808011893247,
130.190614848446));
#222747=CARTESIAN_POINT('Ctrl Pts',(-67.6998110464348,-3.85576491002292,
135.670409814162));
#222748=CARTESIAN_POINT('Ctrl Pts',(-67.9782586702478,2.00980988661012,
136.678543287925));
#222749=CARTESIAN_POINT('Ctrl Pts',(-68.2567062940606,6.02846758211988,
132.288589857404));
#222750=CARTESIAN_POINT('Ctrl Pts',(-68.5351539178734,4.50725807667536,
126.534702264101));
#222751=CARTESIAN_POINT('Ctrl Pts',(-68.8136015416864,-1.15590140943545,
124.704422113226));
#222752=CARTESIAN_POINT('Ctrl Pts',(-69.0920491654993,-5.75684396919829,
128.479687449276));
#222753=CARTESIAN_POINT('Ctrl Pts',(-69.3704967893121,-5.0675281587308,
134.391213860386));
#222754=CARTESIAN_POINT('Ctrl Pts',(-69.648944413125,0.278598467097045,
137.006597368867));
#222755=CARTESIAN_POINT('Ctrl Pts',(-69.9273920369379,5.36870671195437,
133.922428299012));
#222756=CARTESIAN_POINT('Ctrl Pts',(-70.2058396607509,5.52523576442926,
127.972907355982));
#222757=CARTESIAN_POINT('Ctrl Pts',(-70.4842872845636,0.604343072166899,
124.625353636165));
#222758=CARTESIAN_POINT('Ctrl Pts',(-70.7627349083767,-4.87191137961658,
126.956005470983));
#222759=CARTESIAN_POINT('Ctrl Pts',(-71.0411825321895,-5.87111727963483,
132.823107682909));
#222760=CARTESIAN_POINT('Ctrl Pts',(-71.3196301560023,-1.47505321969301,
136.835079963061));
#222761=CARTESIAN_POINT('Ctrl Pts',(-71.5980777798154,4.27651268879093,
135.305115781721));
#222762=CARTESIAN_POINT('Ctrl Pts',(-71.8765254036282,6.09817235553532,
129.639177478635));
#222763=CARTESIAN_POINT('Ctrl Pts',(-72.1549730274411,2.31590953982396,
125.043985557866));
#222764=CARTESIAN_POINT('Ctrl Pts',(-72.433420651254,-3.5945610045145,125.742296906994));
#222765=CARTESIAN_POINT('Ctrl Pts',(-72.7118682750669,-6.20180558977201,
131.092397510578));
#222766=CARTESIAN_POINT('Ctrl Pts',(-72.9903158988798,-3.109893813075,136.177806280867));
#222767=CARTESIAN_POINT('Ctrl Pts',(-73.2687635226926,2.8398584510789,136.325280993997));
#222768=CARTESIAN_POINT('Ctrl Pts',(-73.5472111465057,6.17991953348924,
131.399299593141));
#222769=CARTESIAN_POINT('Ctrl Pts',(-73.8256587703184,3.84093647047644,
125.926598338115));
#222770=CARTESIAN_POINT('Ctrl Pts',(-74.1041063941314,-2.02767956872624,
124.93632232597));
#222771=CARTESIAN_POINT('Ctrl Pts',(-74.3825540179442,-6.0329571419232,
129.338486834193));
#222772=CARTESIAN_POINT('Ctrl Pts',(-74.6610016417573,-4.49424182803428,
135.08771773742));
#222773=CARTESIAN_POINT('Ctrl Pts',(-74.9394492655699,1.17446216989917,
136.900752701129));
#222774=CARTESIAN_POINT('Ctrl Pts',(-75.217896889383,5.76389280936176,133.111501165354));
#222775=CARTESIAN_POINT('Ctrl Pts',(-75.4963445131958,5.05658753883907,
127.202100176243));
#222776=CARTESIAN_POINT('Ctrl Pts',(-75.7747921370087,-0.297474651842549,
124.603000552501));
#222777=CARTESIAN_POINT('Ctrl Pts',(-76.0532397608216,-5.37817216992523,
127.702647875272));
#222778=CARTESIAN_POINT('Ctrl Pts',(-76.3316873846344,-5.51659220216403,
133.65261768112));
#222779=CARTESIAN_POINT('Ctrl Pts',(-76.6101350084474,-0.585533501125347,
136.985178390654));
#222780=CARTESIAN_POINT('Ctrl Pts',(-76.8885826322602,4.8836018825454,134.637869516455));
#222781=CARTESIAN_POINT('Ctrl Pts',(-77.1670302560731,5.86494571337264,
128.767753241497));
#222782=CARTESIAN_POINT('Ctrl Pts',(-77.4454778798861,1.4566909521364,124.769179651345));
#222783=CARTESIAN_POINT('Ctrl Pts',(-77.7239255036988,-4.29019163080361,
126.316642534169));
#222784=CARTESIAN_POINT('Ctrl Pts',(-78.0023731275119,-6.09459769254796,
131.988099098418));
#222785=CARTESIAN_POINT('Ctrl Pts',(-78.2808207513247,-2.29836621249045,
136.571757827603));
#222786=CARTESIAN_POINT('Ctrl Pts',(-78.5592683751376,3.60995153541429,
135.855460273781));
#222787=CARTESIAN_POINT('Ctrl Pts',(-78.8377159989505,6.20090017820995,
130.497448895834));
#222788=CARTESIAN_POINT('Ctrl Pts',(-79.1161636227633,3.09352448804556,
125.421474396687));
#222789=CARTESIAN_POINT('Ctrl Pts',(-79.3946112465763,-2.85664907955992,
125.292109365916));
#222790=CARTESIAN_POINT('Ctrl Pts',(-79.6730588703891,-6.18170169811556,
130.228233946967));
#222791=CARTESIAN_POINT('Ctrl Pts',(-79.9515064942021,-3.8260724490201,
135.693790792945));
#222792=CARTESIAN_POINT('Ctrl Pts',(-80.2299541180149,2.04553046669522,
136.666200169693));
#222793=CARTESIAN_POINT('Ctrl Pts',(-80.5084017418279,6.03739081323573,
132.251865364817));
#222794=CARTESIAN_POINT('Ctrl Pts',(-80.7868493656406,4.48118394535095,
126.507344411756));
#222795=CARTESIAN_POINT('Ctrl Pts',(-81.0652969894537,-1.19301205030527,
124.711571430921));
#222796=CARTESIAN_POINT('Ctrl Pts',(-81.3437446132665,-5.77088825360962,
128.514774063314));
#222797=CARTESIAN_POINT('Ctrl Pts',(-81.6221922370794,-5.04560007541116,
134.421994886542));
#222798=CARTESIAN_POINT('Ctrl Pts',(-81.9006398608923,0.316348080823153,
137.00478654784));
#222799=CARTESIAN_POINT('Ctrl Pts',(-82.179087484705,5.38758780524389,133.889689686862));
#222800=CARTESIAN_POINT('Ctrl Pts',(-82.4575351085182,5.50789753494193,
127.939326137905));
#222801=CARTESIAN_POINT('Ctrl Pts',(-82.7359827323308,0.566718505781886,
124.621789311041));
#222802=CARTESIAN_POINT('Ctrl Pts',(-83.0144303561439,-4.89524714445407,
126.985733479472));
#222803=CARTESIAN_POINT('Ctrl Pts',(-83.2928779799568,-5.858719815054,132.858809437506));
#222804=CARTESIAN_POINT('Ctrl Pts',(-83.5713256037696,-1.43831518999427,
136.843947295418));
#222805=CARTESIAN_POINT('Ctrl Pts',(-83.8497732275826,4.30383082906709,
135.279000046597));
#222806=CARTESIAN_POINT('Ctrl Pts',(-84.1282208513953,6.09096657004034,
129.602077760783));
#222807=CARTESIAN_POINT('Ctrl Pts',(-84.4066684752085,2.28080159340614,
125.029994685571));
#222808=CARTESIAN_POINT('Ctrl Pts',(-84.685116099021,-3.6253086242162,125.764271808403));
#222809=CARTESIAN_POINT('Ctrl Pts',(-84.9635637228342,-6.19993732235617,
131.130144324829));
#222810=CARTESIAN_POINT('Ctrl Pts',(-85.242011346647,-3.07712650502686,
136.196637529698));
#222811=CARTESIAN_POINT('Ctrl Pts',(-85.5204589704598,2.87341324443482,
136.307891679689));
#222812=CARTESIAN_POINT('Ctrl Pts',(-85.7989065942728,6.18342659630218,
131.361669646028));
#222813=CARTESIAN_POINT('Ctrl Pts',(-86.0773542180856,3.81117298335027,
125.903307841269));
#222814=CARTESIAN_POINT('Ctrl Pts',(-86.3558018418987,-2.06336241514917,
124.948774108188));
#222815=CARTESIAN_POINT('Ctrl Pts',(-86.6342494657113,-6.04176855498474,
129.375238315919));
#222816=CARTESIAN_POINT('Ctrl Pts',(-86.9126970895244,-4.46808454959173,
135.114996102359));
#222817=CARTESIAN_POINT('Ctrl Pts',(-87.1911447133372,1.2115508788106,136.893490464523));
#222818=CARTESIAN_POINT('Ctrl Pts',(-87.4695923371502,5.77783023713722,
133.076371967865));
#222819=CARTESIAN_POINT('Ctrl Pts',(-87.7480399609628,5.03456587023344,
127.171386034204));
#222820=CARTESIAN_POINT('Ctrl Pts',(-88.026487584776,-0.33521857919891,
124.60492626198));
#222821=CARTESIAN_POINT('Ctrl Pts',(-88.3049352085887,-5.39695353068522,
127.735443803332));
#222822=CARTESIAN_POINT('Ctrl Pts',(-88.5833828324018,-5.49915184330967,
133.686145972045));
#222823=CARTESIAN_POINT('Ctrl Pts',(-88.8618304562145,-0.547898260434929,
136.988628183031));
#222824=CARTESIAN_POINT('Ctrl Pts',(-89.1402780800275,4.90684705746115,
134.608070619623));
#222825=CARTESIAN_POINT('Ctrl Pts',(-89.4187257038403,5.85243964235601,
128.732089385887));
#222826=CARTESIAN_POINT('Ctrl Pts',(-89.6971733276532,1.41992610349655,
124.760424177987));
#222827=CARTESIAN_POINT('Ctrl Pts',(-89.9756209514662,-4.31743015722937,
126.342841295349));
#222828=CARTESIAN_POINT('Ctrl Pts',(-90.254068575279,-6.08727902165076,
132.025176712493));
#222829=CARTESIAN_POINT('Ctrl Pts',(-90.5325161990919,-2.26321584528708,
136.585641778581));
#222830=CARTESIAN_POINT('Ctrl Pts',(-90.8109638229048,3.64063212865448,
135.833391888981));
#222831=CARTESIAN_POINT('Ctrl Pts',(-91.0894114467178,6.19891703112955,
130.459707942787));
#222832=CARTESIAN_POINT('Ctrl Pts',(-91.3678590705306,3.06070001592934,
125.402742967496));
#222833=CARTESIAN_POINT('Ctrl Pts',(-91.6463066943433,-2.89015079040179,
125.309600728926));
#222834=CARTESIAN_POINT('Ctrl Pts',(-91.9247543181566,-6.18509421206894,
130.265874394073));
#222835=CARTESIAN_POINT('Ctrl Pts',(-92.2032019419691,-3.79623821149537,
135.716990592095));
#222836=CARTESIAN_POINT('Ctrl Pts',(-92.4816495657822,2.08117524889636,
136.653639838841));
#222837=CARTESIAN_POINT('Ctrl Pts',(-92.7600971895951,6.04609032661485,
132.21508723441));
#222838=CARTESIAN_POINT('Ctrl Pts',(-93.0385448134079,4.45494376210749,
126.480145786926));
#222839=CARTESIAN_POINT('Ctrl Pts',(-93.3169924372209,-1.23007848367479,
124.718946519161));
#222840=CARTESIAN_POINT('Ctrl Pts',(-93.5954400610337,-5.78471869563455,
128.549945518824));
#222841=CARTESIAN_POINT('Ctrl Pts',(-93.8738876848466,-5.02348502552524,
134.45264185993));
#222842=CARTESIAN_POINT('Ctrl Pts',(-94.1523353086595,0.354085972155003,
137.002745967751));
#222843=CARTESIAN_POINT('Ctrl Pts',(-94.4307829324724,5.40626925948619,
133.85683674671));
#222844=CARTESIAN_POINT('Ctrl Pts',(-94.7092305562852,5.49035520828578,
127.905851084735));
#222845=CARTESIAN_POINT('Ctrl Pts',(-94.9876781800983,0.529072939433998,
124.618454083368));
#222846=CARTESIAN_POINT('Ctrl Pts',(-95.2661258039109,-4.91840151410816,
127.015602988595));
#222847=CARTESIAN_POINT('Ctrl Pts',(-95.5445734277241,-5.84610525345601,
132.894435063746));
#222848=CARTESIAN_POINT('Ctrl Pts',(-95.8230210515366,-1.40152386299717,
136.85259082867));
#222849=CARTESIAN_POINT('Ctrl Pts',(-96.10146867535,4.33098948930923,135.252718502061));
#222850=CARTESIAN_POINT('Ctrl Pts',(-96.3799162991623,6.08353508153927,
129.565022593965));
#222851=CARTESIAN_POINT('Ctrl Pts',(-96.6583639229758,2.245609131046,125.01621778453));
#222852=CARTESIAN_POINT('Ctrl Pts',(-96.9368115467883,-3.65592190677386,
125.786433472156));
#222853=CARTESIAN_POINT('Ctrl Pts',(-97.2152591706015,-6.19783931398261,
131.167879067045));
#222854=CARTESIAN_POINT('Ctrl Pts',(-97.493706794414,-3.04424517292474,
136.215268965725));
#222855=CARTESIAN_POINT('Ctrl Pts',(-97.7721544182274,2.90686156240656,
136.290298430015));
#222856=CARTESIAN_POINT('Ctrl Pts',(-98.0506020420397,6.18670452996842,
131.324019047625));
#222857=CARTESIAN_POINT('Ctrl Pts',(-98.3290496658531,3.78126827180747,
125.880198954735));
#222858=CARTESIAN_POINT('Ctrl Pts',(-98.6074972896656,-2.09896880291958,
124.961442871316));
#222859=CARTESIAN_POINT('Ctrl Pts',(-98.8859449134787,-6.05035608809047,
129.412042754299));
#222860=CARTESIAN_POINT('Ctrl Pts',(-99.1643925372916,-4.44176170463296,
135.142114735114));
#222861=CARTESIAN_POINT('Ctrl Pts',(-99.4428401611044,1.24859469325925,
136.886002592972));
#222862=CARTESIAN_POINT('Ctrl Pts',(-99.7212877849174,5.79155356528836,
133.041158580159));
#222863=CARTESIAN_POINT('Ctrl Pts',(-99.9997354087301,5.01235764393804,
127.140806513377));
#222864=CARTESIAN_POINT('Ctrl Pts',(-100.278183032543,-0.37295008490757,
124.607081693777));
#222865=CARTESIAN_POINT('Ctrl Pts',(-100.556630656356,-5.41553490534739,
127.768353451233));
#222866=CARTESIAN_POINT('Ctrl Pts',(-100.835078280169,-5.48150771136145,
133.719567477352));
#222867=CARTESIAN_POINT('Ctrl Pts',(-101.113525903981,-0.510242717172956,
136.9918488151));
#222868=CARTESIAN_POINT('Ctrl Pts',(-101.391973527794,4.92991040735466,
134.578130774917));
#222869=CARTESIAN_POINT('Ctrl Pts',(-101.670421151607,5.83971670703623,
128.696502319049));
#222870=CARTESIAN_POINT('Ctrl Pts',(-101.94886877542,1.38310863897239,124.751892664915));
#222871=CARTESIAN_POINT('Ctrl Pts',(-102.227316399233,-4.34450869969331,
126.36920537977));
#222872=CARTESIAN_POINT('Ctrl Pts',(-102.505764023046,-6.07973478439049,
132.062209088779));
#222873=CARTESIAN_POINT('Ctrl Pts',(-102.784211646859,-2.22798161378826,
136.599311502058));
#222874=CARTESIAN_POINT('Ctrl Pts',(-103.062659270672,3.6711778169323,135.811137151577));
#222875=CARTESIAN_POINT('Ctrl Pts',(-103.341106894485,6.19670418089893,
130.42197976097));
#222876=CARTESIAN_POINT('Ctrl Pts',(-103.619554518298,3.02776212844844,
125.384211697232));
#222877=CARTESIAN_POINT('Ctrl Pts',(-103.89800214211,-2.92354540564323,
125.327295702285));
#222878=CARTESIAN_POINT('Ctrl Pts',(-104.176449765923,-6.18825753508174,
130.303534794984));
#222879=CARTESIAN_POINT('Ctrl Pts',(-104.454897389736,-3.76626330296762,
135.740008351935));
#222880=CARTESIAN_POINT('Ctrl Pts',(-104.733345013549,2.1167429123828,136.640862760796));
#222881=CARTESIAN_POINT('Ctrl Pts',(-105.011792637362,6.05456579989334,
132.17825682901));
#222882=CARTESIAN_POINT('Ctrl Pts',(-105.290240261175,4.42853849928509,
126.453107397468));
#222883=CARTESIAN_POINT('Ctrl Pts',(-105.568687884988,-1.26709933603374,
124.726547104658));
#222884=CARTESIAN_POINT('Ctrl Pts',(-105.847135508801,-5.79833478278087,
128.585200512514));
#222885=CARTESIAN_POINT('Ctrl Pts',(-106.125583132613,-5.00118382855433,
134.483153644914));
#222886=CARTESIAN_POINT('Ctrl Pts',(-106.404030756427,0.391810742700936,
137.000475704212));
#222887=CARTESIAN_POINT('Ctrl Pts',(-106.682478380239,5.42475038243292,
133.823870695931));
#222888=CARTESIAN_POINT('Ctrl Pts',(-106.960926004052,5.47260943449832,
127.872483436902));
#222889=CARTESIAN_POINT('Ctrl Pts',(-107.239373627865,0.491407768093767,
124.615348076738));
#222890=CARTESIAN_POINT('Ctrl Pts',(-107.517821251678,-4.94137363058539,
127.045612891524));
#222891=CARTESIAN_POINT('Ctrl Pts',(-107.796268875491,-5.83327406227795,
132.929983241508));
#222892=CARTESIAN_POINT('Ctrl Pts',(-108.074716499304,-1.36468060201792,
136.861010242526));
#222893=CARTESIAN_POINT('Ctrl Pts',(-108.353164123117,4.3579876631431,135.22627212199));
#222894=CARTESIAN_POINT('Ctrl Pts',(-108.631611746929,6.07587816540856,
129.528013351273));
#222895=CARTESIAN_POINT('Ctrl Pts',(-108.910059370743,2.21033345681367,
125.00265536525));
#222896=CARTESIAN_POINT('Ctrl Pts',(-109.188506994555,-3.68639971780079,
125.808781077045));
#222897=CARTESIAN_POINT('Ctrl Pts',(-109.466954618368,-6.19551164239422,
131.205600338952));
#222898=CARTESIAN_POINT('Ctrl Pts',(-109.745402242181,-3.01125103519769,
136.233699898554));
#222899=CARTESIAN_POINT('Ctrl Pts',(-110.023849865994,2.94020216555433,
136.272501896897));
#222900=CARTESIAN_POINT('Ctrl Pts',(-110.302297489807,6.18975321302316,
131.286349193086));
#222901=CARTESIAN_POINT('Ctrl Pts',(-110.58074511362,3.75122344397827,125.857272534824));
#222902=CARTESIAN_POINT('Ctrl Pts',(-110.859192737433,-2.13449741262907,
124.974328145912));
#222903=CARTESIAN_POINT('Ctrl Pts',(-111.137640361246,-6.05871942302636,
129.44889878553));
#222904=CARTESIAN_POINT('Ctrl Pts',(-111.416087985058,-4.41527426856075,
135.169072630797));
#222905=CARTESIAN_POINT('Ctrl Pts',(-111.694535608871,1.28559224057236,
136.878289363941));
#222906=CARTESIAN_POINT('Ctrl Pts',(-111.972983232684,5.8050622852923,133.005862307081));
#222907=CARTESIAN_POINT('Ctrl Pts',(-112.251430856497,4.9899636828869,127.110362746893));
#222908=CARTESIAN_POINT('Ctrl Pts',(-112.52987848031,-0.410667770813077,
124.609466768025));
#222909=CARTESIAN_POINT('Ctrl Pts',(-112.808326104123,-5.43391560537209,
127.801375599495));
#222910=CARTESIAN_POINT('Ctrl Pts',(-113.086773727936,-5.46366046012913,
133.752880958598));
#222911=CARTESIAN_POINT('Ctrl Pts',(-113.365221351749,-0.472568266679477,
136.994840167519));
#222912=CARTESIAN_POINT('Ctrl Pts',(-113.643668975562,4.95279107760506,
134.548051091771));
#222913=CARTESIAN_POINT('Ctrl Pts',(-113.922116599375,5.8267773788663,128.660993359675));
#222914=CARTESIAN_POINT('Ctrl Pts',(-114.200564223187,1.34623992284899,
124.74358542827));
#222915=CARTESIAN_POINT('Ctrl Pts',(-114.479011847001,-4.37142625478972,
126.395733810498));
#222916=CARTESIAN_POINT('Ctrl Pts',(-114.757459470813,-6.07196526032194,
132.099194855029));
#222917=CARTESIAN_POINT('Ctrl Pts',(-115.035907094626,-2.19266482361144,
136.612766491501));
#222918=CARTESIAN_POINT('Ctrl Pts',(-115.314354718439,3.70158746836604,
135.788696886227));
#222919=CARTESIAN_POINT('Ctrl Pts',(-115.592802342252,6.19426170951602,
130.384265748418));
#222920=CARTESIAN_POINT('Ctrl Pts',(-115.871249966065,2.99471204612843,
125.36588127258));
#222921=CARTESIAN_POINT('Ctrl Pts',(-116.149697589878,-2.95683168783455,
125.345193630298));
#222922=CARTESIAN_POINT('Ctrl Pts',(-116.428145213691,-6.19119154993583,
130.34121375418));
#222923=CARTESIAN_POINT('Ctrl Pts',(-116.706592837503,-3.73614883416816,
135.762843219532));
#222924=CARTESIAN_POINT('Ctrl Pts',(-116.985040461316,2.1522321391827,136.627869409019));
#222925=CARTESIAN_POINT('Ctrl Pts',(-117.263488085129,6.06281691900968,
132.14137551338));
#222926=CARTESIAN_POINT('Ctrl Pts',(-117.541935708942,4.40196913533955,
126.426230245297));
#222927=CARTESIAN_POINT('Ctrl Pts',(-117.820383332755,-1.30407323556081,
124.73437290577));
#222928=CARTESIAN_POINT('Ctrl Pts',(-118.098830956568,-5.81173601049948,
128.620537737998));
#222929=CARTESIAN_POINT('Ctrl Pts',(-118.377278580381,-4.97869731087745,
134.51352911087));
#222930=CARTESIAN_POINT('Ctrl Pts',(-118.655726204194,0.429520994555717,
136.997975841351));
#222931=CARTESIAN_POINT('Ctrl Pts',(-118.934173828006,5.44303048925927,
133.790792756097));
#222932=CARTESIAN_POINT('Ctrl Pts',(-119.21262145182,5.45466087115571,127.839224430854));
#222933=CARTESIAN_POINT('Ctrl Pts',(-119.491069075632,0.453724387457947,
124.612471406243));
#222934=CARTESIAN_POINT('Ctrl Pts',(-119.769516699445,-4.96416264264509,
127.075762076232));
#222935=CARTESIAN_POINT('Ctrl Pts',(-120.047964323258,-5.82022671698453,
132.965452653541));
#222936=CARTESIAN_POINT('Ctrl Pts',(-120.326411947071,-1.32778677229758,
136.869205225004));
#222937=CARTESIAN_POINT('Ctrl Pts',(-120.604859570884,4.38482435014149,
135.199661886361));
#222938=CARTESIAN_POINT('Ctrl Pts',(-120.883307194697,6.06799610537801,
129.491051404098));
#222939=CARTESIAN_POINT('Ctrl Pts',(-121.16175481851,2.17497587786225,124.989307930291));
#222940=CARTESIAN_POINT('Ctrl Pts',(-121.440202442323,-3.71674092793051,
125.831313794972));
#222941=CARTESIAN_POINT('Ctrl Pts',(-121.718650066136,-6.19295439384353,
131.243306742772));
#222942=CARTESIAN_POINT('Ctrl Pts',(-121.997097689948,-2.97814531445616,
136.251929645219));
#222943=CARTESIAN_POINT('Ctrl Pts',(-122.275545313761,2.97343381842962,
136.254502739794));
#222944=CARTESIAN_POINT('Ctrl Pts',(-122.553992937574,6.19257253249627,
131.248661478285));
#222945=CARTESIAN_POINT('Ctrl Pts',(-122.832440561387,3.72103961318487,
125.83452943108));
#222946=CARTESIAN_POINT('Ctrl Pts',(-123.1108881852,-2.16994692775201,124.987429454503));
#222947=CARTESIAN_POINT('Ctrl Pts',(-123.389335809013,-6.06685824988591,
129.485805043896));
#222948=CARTESIAN_POINT('Ctrl Pts',(-123.667783432826,-4.38862322287681,
135.19586879047));
#222949=CARTESIAN_POINT('Ctrl Pts',(-123.946231056639,1.32254214979223,
136.870351063246));
#222950=CARTESIAN_POINT('Ctrl Pts',(-124.224678680451,5.81835589657845,
132.97048445655));
#222951=CARTESIAN_POINT('Ctrl Pts',(-124.503126304264,4.96738481689638,
127.080055862859));
#222952=CARTESIAN_POINT('Ctrl Pts',(-124.781573928077,-0.448370239273912,
124.612081396343));
#222953=CARTESIAN_POINT('Ctrl Pts',(-125.06002155189,-5.4520949496557,127.834509024472));
#222954=CARTESIAN_POINT('Ctrl Pts',(-125.338469175703,-5.44561075094924,
133.786085181339));
#222955=CARTESIAN_POINT('Ctrl Pts',(-125.616916799516,-0.434876304995071,
136.997602129441));
#222956=CARTESIAN_POINT('Ctrl Pts',(-125.895364423329,4.97548822036069,
134.517832684797));
#222957=CARTESIAN_POINT('Ctrl Pts',(-126.173812047142,5.8136221373178,128.625563823564));
#222958=CARTESIAN_POINT('Ctrl Pts',(-126.452259670955,1.30932132131015,
124.735502775877));
#222959=CARTESIAN_POINT('Ctrl Pts',(-126.730707294768,-4.39818182507867,
126.422425604514));
#222960=CARTESIAN_POINT('Ctrl Pts',(-127.00915491858,-6.0639707373477,132.136132640718));
#222961=CARTESIAN_POINT('Ctrl Pts',(-127.287602542393,-2.15726678343353,
136.626006248326));
#222962=CARTESIAN_POINT('Ctrl Pts',(-127.566050166206,3.73185995611441,
135.766071924465));
#222963=CARTESIAN_POINT('Ctrl Pts',(-127.844497790019,6.19158970748781,
130.346567302635));
#222964=CARTESIAN_POINT('Ctrl Pts',(-128.122945413832,2.96155099365221,
125.34775237278));
#222965=CARTESIAN_POINT('Ctrl Pts',(-128.401393037645,-2.99000840354028,
125.363293849751));
#222966=CARTESIAN_POINT('Ctrl Pts',(-128.679840661458,-6.19389614791022,
130.378909875453));
#222967=CARTESIAN_POINT('Ctrl Pts',(-128.958288285271,-3.70589592099968,
135.785494348734));
#222968=CARTESIAN_POINT('Ctrl Pts',(-129.236735909083,2.18764161422919,
136.614660264981));
#222969=CARTESIAN_POINT('Ctrl Pts',(-129.515183532897,6.07084337821547,
132.104444654172));
#222970=CARTESIAN_POINT('Ctrl Pts',(-129.793631156709,4.37523665480886,
126.399515326358));
#222971=CARTESIAN_POINT('Ctrl Pts',(-130.072078780522,-1.34099881217456,
124.742423632508));
#222972=CARTESIAN_POINT('Ctrl Pts',(-130.350526404335,-5.82492188220296,
128.655955885842));
#222973=CARTESIAN_POINT('Ctrl Pts',(-130.628974028148,-4.95602630574081,
134.543767132223));
#222974=CARTESIAN_POINT('Ctrl Pts',(-130.907421651961,0.467215330352083,
136.995246471799));
#222975=CARTESIAN_POINT('Ctrl Pts',(-131.185869275774,5.46110890258918,
133.757604152921));
#222976=CARTESIAN_POINT('Ctrl Pts',(-131.464316899587,5.43651018334856,
127.80607529902));
#222977=CARTESIAN_POINT('Ctrl Pts',(-131.742764523399,0.416024193898128,
124.60982417848));
#222978=CARTESIAN_POINT('Ctrl Pts',(-132.021212147213,-4.98676770583297,
127.106049425532));
#222979=CARTESIAN_POINT('Ctrl Pts',(-132.299659771025,-5.80696370104951,
133.000841985516));
#222980=CARTESIAN_POINT('Ctrl Pts',(-132.578107394838,-1.2908437409496,
136.877175472434));
#222981=CARTESIAN_POINT('Ctrl Pts',(-132.856555018651,4.41149855586104,
135.172888781227));
#222982=CARTESIAN_POINT('Ctrl Pts',(-133.135002642464,6.05988919352027,
129.454138122079));
#222983=CARTESIAN_POINT('Ctrl Pts',(-133.413450266277,2.13953770437982,
124.976175974248));
#222984=CARTESIAN_POINT('Ctrl Pts',(-133.69189789009,-3.74694441285829,
125.854030790976));
#222985=CARTESIAN_POINT('Ctrl Pts',(-133.970345513903,-6.19016766309031,
131.280996881284));
#222986=CARTESIAN_POINT('Ctrl Pts',(-134.248793137716,-2.94492923744478,
136.269957530209));
#222987=CARTESIAN_POINT('Ctrl Pts',(-134.527240761528,3.00655528962129,
136.236301625668));
#222988=CARTESIAN_POINT('Ctrl Pts',(-134.805688385342,6.19516238391663,
131.210957299752));
#222989=CARTESIAN_POINT('Ctrl Pts',(-135.084136009154,3.69071789790064,
125.811970486258));
#222990=CARTESIAN_POINT('Ctrl Pts',(-135.362583632967,-2.2053160346932,
125.000746311619));
#222991=CARTESIAN_POINT('Ctrl Pts',(-135.64103125678,-6.07477226708194,
129.522760161825));
#222992=CARTESIAN_POINT('Ctrl Pts',(-135.919478880593,-4.36180955514542,
135.222502221193));
#222993=CARTESIAN_POINT('Ctrl Pts',(-136.197926504406,1.35944305172635,
136.862187985044));
#222994=CARTESIAN_POINT('Ctrl Pts',(-136.476374128219,5.83143390654715,
132.935026339502));
#222995=CARTESIAN_POINT('Ctrl Pts',(-136.754821752032,4.9446218826347,127.049886984307));
#222996=CARTESIAN_POINT('Ctrl Pts',(-137.033269375845,-0.486056093210629,
124.614925481843));
#222997=CARTESIAN_POINT('Ctrl Pts',(-137.311716999657,-5.47007226455594,
127.867752498391));
#222998=CARTESIAN_POINT('Ctrl Pts',(-137.59016462347,-5.42735925266033,
133.819178915179));
#222999=CARTESIAN_POINT('Ctrl Pts',(-137.868612247283,-0.397168228809268,
137.000134598521));
#223000=CARTESIAN_POINT('Ctrl Pts',(-138.147059871096,4.99800099457058,
134.487476673751));
#223001=CARTESIAN_POINT('Ctrl Pts',(-138.425507494909,5.80025146986304,
128.590215023569));
#223002=CARTESIAN_POINT('Ctrl Pts',(-138.703955118722,1.27235420238826,
124.727645007244));
#223003=CARTESIAN_POINT('Ctrl Pts',(-138.982402742535,-4.42477441912264,
126.449279772744));
#223004=CARTESIAN_POINT('Ctrl Pts',(-139.260850366348,-6.05575151170779,
132.173021077107));
#223005=CARTESIAN_POINT('Ctrl Pts',(-139.539297990161,-2.12178880494131,
136.639030281933));
#223006=CARTESIAN_POINT('Ctrl Pts',(-139.817745613973,3.76199415842019,
135.743263104665));
#223007=CARTESIAN_POINT('Ctrl Pts',(-140.096193237787,6.18868827382574,
130.308885820552));
#223008=CARTESIAN_POINT('Ctrl Pts',(-140.374640861599,2.92828019981485,
125.329825669606));
#223009=CARTESIAN_POINT('Ctrl Pts',(-140.653088485412,-3.02307432338508,
125.381595689934));
#223010=CARTESIAN_POINT('Ctrl Pts',(-140.931536109225,-6.19637122878504,
130.416621761961));
#223011=CARTESIAN_POINT('Ctrl Pts',(-141.209983733038,-3.675505684495,135.807960900193));
#223012=CARTESIAN_POINT('Ctrl Pts',(-141.488431356851,2.22297002541115,
136.601235818153));
#223013=CARTESIAN_POINT('Ctrl Pts',(-141.766878980664,6.07864488008735,
132.06746561987));
#223014=CARTESIAN_POINT('Ctrl Pts',(-142.045326604476,4.34834204827492,
126.372963630579));
#223015=CARTESIAN_POINT('Ctrl Pts',(-142.32377422829,-1.3778746975837,124.750698986551));
#223016=CARTESIAN_POINT('Ctrl Pts',(-142.602221852102,-5.83789190928377,
128.691453643612));
#223017=CARTESIAN_POINT('Ctrl Pts',(-142.880669475915,-4.93317165322728,
134.573866588494));
#223018=CARTESIAN_POINT('Ctrl Pts',(-143.159117099728,0.504892353312588,
136.992287696695));
#223019=CARTESIAN_POINT('Ctrl Pts',(-143.437564723541,5.47898495252035,
133.72430611622));
#223020=CARTESIAN_POINT('Ctrl Pts',(-143.716012347354,5.4181580436573,127.77303726975));
#223021=CARTESIAN_POINT('Ctrl Pts',(-143.994459971167,0.378308584408798,
124.607406491544));
#223022=CARTESIAN_POINT('Ctrl Pts',(-144.27290759498,-5.00918798250961,
127.136473817112));
#223023=CARTESIAN_POINT('Ctrl Pts',(-144.551355218793,-5.79348550593904,
133.036149926065));
#223024=CARTESIAN_POINT('Ctrl Pts',(-144.829802842605,-1.2538528769121,
136.884920689477));
#223025=CARTESIAN_POINT('Ctrl Pts',(-145.108250466418,4.43800929187927,
135.145953798675));
#223026=CARTESIAN_POINT('Ctrl Pts',(-145.386698090231,6.05155773023994,
129.417274873051));
#223027=CARTESIAN_POINT('Ctrl Pts',(-145.665145714044,2.10402024954095,
124.963259983731));
#223028=CARTESIAN_POINT('Ctrl Pts',(-145.943593337857,-3.77700905338292,
125.876931223274));
#223029=CARTESIAN_POINT('Ctrl Pts',(-146.22204096167,-6.18715155339789,
131.318669357863));
#223030=CARTESIAN_POINT('Ctrl Pts',(-146.500488585483,-2.9116040349975,
136.287782885497));
#223031=CARTESIAN_POINT('Ctrl Pts',(-146.778936209295,3.03956535180104,
136.217899228972));
#223032=CARTESIAN_POINT('Ctrl Pts',(-147.057383833109,6.19752267131684,
131.173238054629));
#223033=CARTESIAN_POINT('Ctrl Pts',(-147.335831456921,3.66025942170698,
125.789596536289));
#223034=CARTESIAN_POINT('Ctrl Pts',(-147.614279080735,-2.24060342283806,
125.014278223797));
#223035=CARTESIAN_POINT('Ctrl Pts',(-147.892726704547,-6.08246118135759,
129.559762769929));
#223036=CARTESIAN_POINT('Ctrl Pts',(-148.17117432836,-4.33483425895693,
135.248971936054));
#223037=CARTESIAN_POINT('Ctrl Pts',(-148.449621952173,1.39629357899829,
136.853800431821));
#223038=CARTESIAN_POINT('Ctrl Pts',(-148.728069575986,5.84429583058792,
132.899489269852));
#223039=CARTESIAN_POINT('Ctrl Pts',(-149.006517199799,4.9216757235908,127.019857229157));
#223040=CARTESIAN_POINT('Ctrl Pts',(-149.284964823612,-0.52372393616008,
124.617998919139));
#223041=CARTESIAN_POINT('Ctrl Pts',(-149.563412447425,-5.48784688391679,
127.901104789406));
#223042=CARTESIAN_POINT('Ctrl Pts',(-149.841860071237,-5.40890664157841,
133.852160933818));
#223043=CARTESIAN_POINT('Ctrl Pts',(-150.12030769505,-0.359445435409253,
137.002437480918));
#223044=CARTESIAN_POINT('Ctrl Pts',(-150.398755318863,5.02032856601553,
134.456984183485));
#223045=CARTESIAN_POINT('Ctrl Pts',(-150.677202942676,5.78666587195703,
128.554948269553));
#223046=CARTESIAN_POINT('Ctrl Pts',(-150.955650566489,1.23533993591347,
124.720012413542));
#223047=CARTESIAN_POINT('Ctrl Pts',(-151.234098190302,-4.45120305152329,
126.476295320094));
#223048=CARTESIAN_POINT('Ctrl Pts',(-151.512545814115,-6.0473078879686,
132.209858797279));
#223049=CARTESIAN_POINT('Ctrl Pts',(-151.790993437928,-2.08623220278462,
136.651838109709));
#223050=CARTESIAN_POINT('Ctrl Pts',(-152.069441061741,3.79198895864895,
135.720271272016));
#223051=CARTESIAN_POINT('Ctrl Pts',(-152.347888685554,6.18555751604382,
130.27122269847));
#223052=CARTESIAN_POINT('Ctrl Pts',(-152.626336309366,2.89490089747778,
125.312101827337));
#223053=CARTESIAN_POINT('Ctrl Pts',(-152.904783933179,-3.05602822209906,
125.400098472666));
#223054=CARTESIAN_POINT('Ctrl Pts',(-153.183231556992,-6.19861670084527,
130.454348016274));
#223055=CARTESIAN_POINT('Ctrl Pts',(-153.461679180805,-3.64497925077551,
135.830242041403));
#223056=CARTESIAN_POINT('Ctrl Pts',(-153.740126804618,2.25821606362131,
136.587596565983));
#223057=CARTESIAN_POINT('Ctrl Pts',(-154.018574428431,6.08622113553776,
132.030439780749));
#223058=CARTESIAN_POINT('Ctrl Pts',(-154.297022052244,4.32128631232727,
126.346576141847));
#223059=CARTESIAN_POINT('Ctrl Pts',(-154.575469676057,-1.41469952533967,
124.759198661251));
#223060=CARTESIAN_POINT('Ctrl Pts',(-154.85391729987,-5.85064561113321,
128.727029695929));
#223061=CARTESIAN_POINT('Ctrl Pts',(-155.132364923682,-4.9101342002235,
134.603826364333));
#223062=CARTESIAN_POINT('Ctrl Pts',(-155.410812547495,0.542550667301237,
136.989099625678));
#223063=CARTESIAN_POINT('Ctrl Pts',(-155.689260171308,5.49665797664923,
133.690899879866));
#223064=CARTESIAN_POINT('Ctrl Pts',(-155.967707795121,5.39960513212718,
127.740111567281));
#223065=CARTESIAN_POINT('Ctrl Pts',(-156.246155418934,0.340578956555753,
124.605218435021));
#223066=CARTESIAN_POINT('Ctrl Pts',(-156.524603042747,-5.03142264188343,
127.167034123586));
#223067=CARTESIAN_POINT('Ctrl Pts',(-156.80305066656,-5.77979263109261,
133.071375166841));
#223068=CARTESIAN_POINT('Ctrl Pts',(-157.081498290373,-1.21681555089514,
136.89244058913));
#223069=CARTESIAN_POINT('Ctrl Pts',(-157.359945914186,4.46435557583064,
135.118857936792));
#223070=CARTESIAN_POINT('Ctrl Pts',(-157.638393537999,6.04300202426259,
129.380463022997));
#223071=CARTESIAN_POINT('Ctrl Pts',(-157.916841161811,2.06842482945845,
124.950560437346));
#223072=CARTESIAN_POINT('Ctrl Pts',(-158.195288785624,-3.80693373544809,
125.900014243279));
#223073=CARTESIAN_POINT('Ctrl Pts',(-158.473736409437,-6.18390617652933,
131.356322776543));
#223074=CARTESIAN_POINT('Ctrl Pts',(-158.75218403325,-2.87817094199197,
136.305405050556));
#223075=CARTESIAN_POINT('Ctrl Pts',(-159.030631657063,3.07246278176887,
136.199296231612));
#223076=CARTESIAN_POINT('Ctrl Pts',(-159.309079280876,6.19965330723533,
131.135505140616));
#223077=CARTESIAN_POINT('Ctrl Pts',(-159.587526904689,3.62966531325439,
125.767408410247));
#223078=CARTESIAN_POINT('Ctrl Pts',(-159.865974528502,-2.27580778459908,
125.028024689608));
#223079=CARTESIAN_POINT('Ctrl Pts',(-160.144422152314,-6.08992470779737,
129.596811497064));
#223080=CARTESIAN_POINT('Ctrl Pts',(-160.422869776128,-4.3076983338908,
135.275276954208));
#223081=CARTESIAN_POINT('Ctrl Pts',(-160.70131739994,1.43309236609815,136.845188714382));
#223082=CARTESIAN_POINT('Ctrl Pts',(-160.979765023753,5.85694119209746,
132.863874564441));
#223083=CARTESIAN_POINT('Ctrl Pts',(-161.258212647566,4.89854719004298,
126.989967710171));
#223084=CARTESIAN_POINT('Ctrl Pts',(-161.536660271379,-0.561372372326459,
124.621301594343));
#223085=CARTESIAN_POINT('Ctrl Pts',(-161.815107895192,-5.50541814909322,
127.934564661631));
#223086=CARTESIAN_POINT('Ctrl Pts',(-162.093555519005,-5.39025360147175,
133.885030015096));
#223087=CARTESIAN_POINT('Ctrl Pts',(-162.372003142818,-0.32170932262588,
137.004510691297));
#223088=CARTESIAN_POINT('Ctrl Pts',(-162.650450766631,5.04247010733932,
134.426356343909));
#223089=CARTESIAN_POINT('Ctrl Pts',(-162.928898390443,5.77286584701905,
128.519764868338));
#223090=CARTESIAN_POINT('Ctrl Pts',(-163.207346014257,1.19827989346308,
124.712605277602));
#223091=CARTESIAN_POINT('Ctrl Pts',(-163.485793638069,-4.47746674295796,
126.503471245498));
#223092=CARTESIAN_POINT('Ctrl Pts',(-163.764241261882,-6.03864017901171,
132.246644436198));
#223093=CARTESIAN_POINT('Ctrl Pts',(-164.042688885695,-2.05059829452646,
136.664429257056));
#223094=CARTESIAN_POINT('Ctrl Pts',(-164.321136509508,3.82184324533235,
135.697097278492));
#223095=CARTESIAN_POINT('Ctrl Pts',(-164.599584133321,6.18219755015336,
130.23357933201));
#223096=CARTESIAN_POINT('Ctrl Pts',(-164.878031757134,2.86141432352365,
125.294581502737));
#223097=CARTESIAN_POINT('Ctrl Pts',(-165.156479380946,-3.08886887856293,
125.418801512319));
#223098=CARTESIAN_POINT('Ctrl Pts',(-165.43492700476,-6.20063248088431,
130.492087240433));
#223099=CARTESIAN_POINT('Ctrl Pts',(-165.713374628572,-3.61431775100944,
135.85233694673));
#223100=CARTESIAN_POINT('Ctrl Pts',(-165.991822252385,2.2933784228048,136.573743013877));
#223101=CARTESIAN_POINT('Ctrl Pts',(-166.270269876198,6.09357186382579,
131.993368508814));
#223102=CARTESIAN_POINT('Ctrl Pts',(-166.548717500011,4.2940704495262,126.320353837957));
#223103=CARTESIAN_POINT('Ctrl Pts',(-166.827165123824,-1.45147193088449,
124.767922341652));
#223104=CARTESIAN_POINT('Ctrl Pts',(-167.105612747637,-5.86318251515793,
128.762682724506));
#223105=CARTESIAN_POINT('Ctrl Pts',(-167.38406037145,-4.88691480039125,
134.633645349573));
#223106=CARTESIAN_POINT('Ctrl Pts',(-167.662507995262,0.580188876875391,
136.985682376883));
#223107=CARTESIAN_POINT('Ctrl Pts',(-167.940955619076,5.51412732009539,
133.657386681736));
#223108=CARTESIAN_POINT('Ctrl Pts',(-168.219403242888,5.38085213624319,
127.707299411689));
#223109=CARTESIAN_POINT('Ctrl Pts',(-168.497850866701,0.302836708424229,
124.60326008999));
#223110=CARTESIAN_POINT('Ctrl Pts',(-168.776298490514,-5.05347086004094,
127.197729212531));
#223111=CARTESIAN_POINT('Ctrl Pts',(-169.054746114327,-5.7658855839047,
133.106516402559));
#223112=CARTESIAN_POINT('Ctrl Pts',(-169.33319373814,-1.17973313533045,
136.899734892741));
#223113=CARTESIAN_POINT('Ctrl Pts',(-169.611641361953,4.49053643144484,
135.091602199623));
#223114=CARTESIAN_POINT('Ctrl Pts',(-169.890088985766,6.03422239262278,
129.34370393599));
#223115=CARTESIAN_POINT('Ctrl Pts',(-170.168536609579,2.03275276313275,
124.938077805679));
#223116=CARTESIAN_POINT('Ctrl Pts',(-170.446984233392,-3.83671735018369,
125.923278995643));
#223117=CARTESIAN_POINT('Ctrl Pts',(-170.725431857205,-6.18043165274327,
131.393955742061));
#223118=CARTESIAN_POINT('Ctrl Pts',(-171.003879481017,-2.84463119730373,
136.32282337239));
#223119=CARTESIAN_POINT('Ctrl Pts',(-171.282327104831,3.10524636049842,
136.180493322929));
#223120=CARTESIAN_POINT('Ctrl Pts',(-171.560774728643,6.20155421272058,
131.097759955922));
#223121=CARTESIAN_POINT('Ctrl Pts',(-171.839222352457,3.59893670621881,
125.745406930321));
#223122=CARTESIAN_POINT('Ctrl Pts',(-172.117669976268,-2.31092781546573,
125.04198519967));
#223123=CARTESIAN_POINT('Ctrl Pts',(-172.396117600082,-6.09716256983718,
129.633904970377));
#223124=CARTESIAN_POINT('Ctrl Pts',(-172.674565223895,-4.2804027854792,
135.301416300912));
#223125=CARTESIAN_POINT('Ctrl Pts',(-172.953012847708,1.469838049433,136.836353151837));
#223126=CARTESIAN_POINT('Ctrl Pts',(-173.23146047152,5.86936952249723,132.828183542982));
#223127=CARTESIAN_POINT('Ctrl Pts',(-173.509908095334,4.8752371390276,126.960219534917));
#223128=CARTESIAN_POINT('Ctrl Pts',(-173.788355719146,-0.599000006633149,
124.624833385073));
#223129=CARTESIAN_POINT('Ctrl Pts',(-174.06680334296,-5.5227854089755,127.968130875202));
#223130=CARTESIAN_POINT('Ctrl Pts',(-174.345250966772,-5.37140082353563,
133.917784941036));
#223131=CARTESIAN_POINT('Ctrl Pts',(-174.623698590585,-0.283961288785237,
137.006354152836));
#223132=CARTESIAN_POINT('Ctrl Pts',(-174.902146214398,5.06442479807889,
134.39559428995));
#223133=CARTESIAN_POINT('Ctrl Pts',(-175.18059383821,5.75885190641417,128.484666123661));
#223134=CARTESIAN_POINT('Ctrl Pts',(-175.459041462024,1.16117544831056,
124.705423873895));
#223135=CARTESIAN_POINT('Ctrl Pts',(-175.737489085836,-4.50356452021585,
126.530806541938));
#223136=CARTESIAN_POINT('Ctrl Pts',(-176.01593670965,-6.02974870602229,
132.28337663076));
#223137=CARTESIAN_POINT('Ctrl Pts',(-176.294384333462,-2.01488840059438,
136.676803257405));
#223138=CARTESIAN_POINT('Ctrl Pts',(-176.572831957276,3.85155591220881,
135.67374198281));
#223139=CARTESIAN_POINT('Ctrl Pts',(-176.851279581088,6.17860850065921,
130.195957116059));
#223140=CARTESIAN_POINT('Ctrl Pts',(-177.129727204901,2.82782171880919,
125.277265345029));
#223141=CARTESIAN_POINT('Ctrl Pts',(-177.408174828714,-3.12159507585506,
125.437704115845));
#223142=CARTESIAN_POINT('Ctrl Pts',(-177.686622452527,-6.20241849420629,
130.529838035997));
#223143=CARTESIAN_POINT('Ctrl Pts',(-177.965070076339,-3.58352232136993,
135.874244797437));
#223144=CARTESIAN_POINT('Ctrl Pts',(-178.243517700153,2.32845580000743,
136.559675675186));
#223145=CARTESIAN_POINT('Ctrl Pts',(-178.521965323965,6.10069679256748,
131.956253177754));
#223146=CARTESIAN_POINT('Ctrl Pts',(-178.800412947778,4.26669546836545,
126.294297690589));
#223147=CARTESIAN_POINT('Ctrl Pts',(-179.078860571591,-1.48819055160311,
124.776869704492));
#223148=CARTESIAN_POINT('Ctrl Pts',(-179.357308195404,-5.8755021567984,
128.798411408209));
#223149=CARTESIAN_POINT('Ctrl Pts',(-179.635755819217,-4.86351431413387,
134.663322439258));
#223150=CARTESIAN_POINT('Ctrl Pts',(-179.91420344303,0.617805587336893,
136.982036076937));
#223151=CARTESIAN_POINT('Ctrl Pts',(-180.192651066843,5.53139233552561,
133.623767763677));
#223152=CARTESIAN_POINT('Ctrl Pts',(-180.471098690656,5.36189975090491,
127.674602018838));
#223153=CARTESIAN_POINT('Ctrl Pts',(-180.749546314469,0.265083238567079,
124.601531529021));
#223154=CARTESIAN_POINT('Ctrl Pts',(-181.027993938281,-5.07533181997731,
127.22855794653));
#223155=CARTESIAN_POINT('Ctrl Pts',(-181.306441562095,-5.75176487970607,
133.141572331048));
#223156=CARTESIAN_POINT('Ctrl Pts',(-181.584889185907,-1.14260700432061,
136.906803330016));
#223157=CARTESIAN_POINT('Ctrl Pts',(-181.86333680972,4.5165508885802,135.064187597142));
#223158=CARTESIAN_POINT('Ctrl Pts',(-182.141784433533,6.02521916065313,
129.306998974155));
#223159=CARTESIAN_POINT('Ctrl Pts',(-182.420232057346,1.99700537240587,
124.925812551278));
#223160=CARTESIAN_POINT('Ctrl Pts',(-182.698679681159,-3.86635879394691,
125.946724618282));
#223161=CARTESIAN_POINT('Ctrl Pts',(-182.977127304972,-6.17672811078948,
131.431566859916));
#223162=CARTESIAN_POINT('Ctrl Pts',(-183.255574928785,-2.81098604376035,
136.340037205557));
#223163=CARTESIAN_POINT('Ctrl Pts',(-183.534022552597,3.13791487318212,
136.161491199671));
#223164=CARTESIAN_POINT('Ctrl Pts',(-183.81247017641,6.20322531733387,131.060003899207));
#223165=CARTESIAN_POINT('Ctrl Pts',(-184.090917800223,3.56807473926006,
125.723592911784));
#223166=CARTESIAN_POINT('Ctrl Pts',(-184.369365424036,-2.34596221405232,
125.056159236672));
#223167=CARTESIAN_POINT('Ctrl Pts',(-184.647813047849,-6.10417449927606,
129.671041815353));
#223168=CARTESIAN_POINT('Ctrl Pts',(-184.926260671662,-4.25294862516783,
135.327389007565));
#223169=CARTESIAN_POINT('Ctrl Pts',(-185.204708295475,1.50652926737877,
136.827294071589));
#223170=CARTESIAN_POINT('Ctrl Pts',(-185.483155919288,5.88158036125089,
132.792417528021));
#223171=CARTESIAN_POINT('Ctrl Pts',(-185.761603543101,4.85174643430717,
126.930613805724));
#223172=CARTESIAN_POINT('Ctrl Pts',(-186.040051166913,-0.6366054447743,
124.628594160457));
#223173=CARTESIAN_POINT('Ctrl Pts',(-186.318498790727,-5.53994802001346,
128.001802186308));
#223174=CARTESIAN_POINT('Ctrl Pts',(-186.596946414539,-5.35234900636664,
133.950424497894));
#223175=CARTESIAN_POINT('Ctrl Pts',(-186.875394038353,-0.246202732654624,
137.007967797222));
#223176=CARTESIAN_POINT('Ctrl Pts',(-187.153841662165,5.08619182469514,
134.364699161505));
#223177=CARTESIAN_POINT('Ctrl Pts',(-187.432289285978,5.744624569434,128.449653336115));
#223178=CARTESIAN_POINT('Ctrl Pts',(-187.71073690979,1.12402797537536,124.698468468532));
#223179=CARTESIAN_POINT('Ctrl Pts',(-187.989184533604,-4.52949541623416,
126.558300196495));
#223180=CARTESIAN_POINT('Ctrl Pts',(-188.267632157416,-6.0206337984771,
132.32005401984));
#223181=CARTESIAN_POINT('Ctrl Pts',(-188.54607978123,-1.97910384423165,
136.688959652232));
#223182=CARTESIAN_POINT('Ctrl Pts',(-188.824527405043,3.88112585826452,
135.650206250412));
#223183=CARTESIAN_POINT('Ctrl Pts',(-189.102975028855,6.17479050055486,
130.158357444724));
#223184=CARTESIAN_POINT('Ctrl Pts',(-189.381422652668,2.79412432812102,
125.260153995869));
#223185=CARTESIAN_POINT('Ctrl Pts',(-189.659870276481,-3.15420560129371,
125.456805582802));
#223186=CARTESIAN_POINT('Ctrl Pts',(-189.938317900294,-6.20397467462999,
130.567599004095));
#223187=CARTESIAN_POINT('Ctrl Pts',(-190.216765524107,-3.55259410299321,
135.89596478172));
#223188=CARTESIAN_POINT('Ctrl Pts',(-190.49521314792,2.36344689542356,136.545395071179));
#223189=CARTESIAN_POINT('Ctrl Pts',(-190.773660771733,6.10759565774615,
131.919095162891));
#223190=CARTESIAN_POINT('Ctrl Pts',(-191.052108395545,4.23916238323504,
126.26840866526));
#223191=CARTESIAN_POINT('Ctrl Pts',(-191.330556019359,-1.52485402687357,
124.786040418225));
#223192=CARTESIAN_POINT('Ctrl Pts',(-191.609003643171,-5.88760407954571,
128.834214423098));
#223193=CARTESIAN_POINT('Ctrl Pts',(-191.887451266984,-4.83993360856504,
134.692856533694));
#223194=CARTESIAN_POINT('Ctrl Pts',(-192.165898890797,0.655399404785621,
136.978160860955));
#223195=CARTESIAN_POINT('Ctrl Pts',(-192.44434651461,5.54845238317892,133.59004437145));
#223196=CARTESIAN_POINT('Ctrl Pts',(-192.722794138423,5.34274867839911,
127.642020600343));
#223197=CARTESIAN_POINT('Ctrl Pts',(-193.001241762236,0.227319945953055,
124.600032816164));
#223198=CARTESIAN_POINT('Ctrl Pts',(-193.279689386049,-5.09700471162664,
127.259519183211));
#223199=CARTESIAN_POINT('Ctrl Pts',(-193.558137009861,-5.73743104174462,
133.176541653297));
#223200=CARTESIAN_POINT('Ctrl Pts',(-193.836584633675,-1.105438533588,136.913645639033));
#223201=CARTESIAN_POINT('Ctrl Pts',(-194.115032257487,4.5423979832614,135.036615145204));
#223202=CARTESIAN_POINT('Ctrl Pts',(-194.3934798813,6.01599266197172,129.270349497605));
#223203=CARTESIAN_POINT('Ctrl Pts',(-194.671927505113,1.96118398191049,
124.913765128639));
#223204=CARTESIAN_POINT('Ctrl Pts',(-194.950375128926,-3.89585696836267,
125.970350242409));
#223205=CARTESIAN_POINT('Ctrl Pts',(-195.228822752739,-6.17279568790409,
131.469154736412));
#223206=CARTESIAN_POINT('Ctrl Pts',(-195.507270376552,-2.77723672809589,
136.357045912194));
#223207=CARTESIAN_POINT('Ctrl Pts',(-195.785718000365,3.17046710927626,
136.142290565968));
#223208=CARTESIAN_POINT('Ctrl Pts',(-196.064165624178,6.20466655915177,
131.022238369536));
#223209=CARTESIAN_POINT('Ctrl Pts',(-196.342613247991,3.5370805559797,125.701967162963));
#223210=CARTESIAN_POINT('Ctrl Pts',(-196.621060871803,-2.38090968214636,
125.070546275391));
#223211=CARTESIAN_POINT('Ctrl Pts',(-196.899508495616,-6.11096023628406,
129.708220655875));
#223212=CARTESIAN_POINT('Ctrl Pts',(-197.177956119429,-4.22533687028115,
135.353194111738));
#223213=CARTESIAN_POINT('Ctrl Pts',(-197.456403743242,1.54316466032852,
136.818011809327));
#223214=CARTESIAN_POINT('Ctrl Pts',(-197.734851367055,5.89357325588093,
132.75657784488));
#223215=CARTESIAN_POINT('Ctrl Pts',(-198.013298990868,4.82807594633875,
126.901151619645));
#223216=CARTESIAN_POINT('Ctrl Pts',(-198.291746614681,-0.674187293266194,
124.632583781138));
#223217=CARTESIAN_POINT('Ctrl Pts',(-198.570194238494,-5.55690534624021,
128.035577347248));
#223218=CARTESIAN_POINT('Ctrl Pts',(-198.848641862306,-5.33309885593691,
133.982947476197));
#223219=CARTESIAN_POINT('Ctrl Pts',(-199.12708948612,-0.2084350533912,137.009351564664));
#223220=CARTESIAN_POINT('Ctrl Pts',(-199.405537109932,5.10777038060287,
134.333672103408));
#223221=CARTESIAN_POINT('Ctrl Pts',(-199.683984733745,5.7301843632779,128.414727803113));
#223222=CARTESIAN_POINT('Ctrl Pts',(-199.962432357558,1.08683885116959,
124.691739319248));
#223223=CARTESIAN_POINT('Ctrl Pts',(-200.240879981371,-4.5552584701342,
126.585951190383));
#223224=CARTESIAN_POINT('Ctrl Pts',(-200.519327605184,-6.01129579413245,
132.356675244344));
#223225=CARTESIAN_POINT('Ctrl Pts',(-200.797775228997,-1.94324595144814,
136.700897991079));
#223226=CARTESIAN_POINT('Ctrl Pts',(-201.076222852809,3.91055198777426,
135.626490953421));
#223227=CARTESIAN_POINT('Ctrl Pts',(-201.354670476623,6.17074369131775,
130.120781711275));
#223228=CARTESIAN_POINT('Ctrl Pts',(-201.633118100435,2.76032340012831,
125.243248089324));
#223229=CARTESIAN_POINT('Ctrl Pts',(-201.911565724248,-3.18669924648382,
125.476105205376));
#223230=CARTESIAN_POINT('Ctrl Pts',(-202.190013348061,-6.20530096449064,
130.605368745483));
#223231=CARTESIAN_POINT('Ctrl Pts',(-202.468460971874,-3.52153424193529,
135.91749609474));
#223232=CARTESIAN_POINT('Ctrl Pts',(-202.746908595687,2.39835041244635,
136.530901731028));
#223233=CARTESIAN_POINT('Ctrl Pts',(-203.0253562195,6.11426820372151,131.881895841131));
#223234=CARTESIAN_POINT('Ctrl Pts',(-203.303803843313,4.21147221438356,
126.242687721299));
#223235=CARTESIAN_POINT('Ctrl Pts',(-203.582251467125,-1.56146099811728,
124.795434143027));
#223236=CARTESIAN_POINT('Ctrl Pts',(-203.860699090939,-5.89948783495869,
128.870090442477));
#223237=CARTESIAN_POINT('Ctrl Pts',(-204.139146714752,-4.81617355747646,
134.722246538484));
#223238=CARTESIAN_POINT('Ctrl Pts',(-204.417594338564,0.69296893616836,
136.974056872534));
#223239=CARTESIAN_POINT('Ctrl Pts',(-204.696041962377,5.56530683088876,
133.556217754686));
#223240=CARTESIAN_POINT('Ctrl Pts',(-204.97448958619,5.32339962837619,127.60955636352));
#223241=CARTESIAN_POINT('Ctrl Pts',(-205.252937210003,0.18954822991528,
124.598764006957));
#223242=CARTESIAN_POINT('Ctrl Pts',(-205.531384833816,-5.11848873189165,
127.290611775294));
#223243=CARTESIAN_POINT('Ctrl Pts',(-205.809832457629,-5.72288460116635,
133.211423073505));
#223244=CARTESIAN_POINT('Ctrl Pts',(-206.088280081441,-1.06822910042401,
136.920261566246));
#223245=CARTESIAN_POINT('Ctrl Pts',(-206.366727705255,4.56807675771487,
135.00888586552));
#223246=CARTESIAN_POINT('Ctrl Pts',(-206.645175329067,6.00654323846982,
129.233756864401));
#223247=CARTESIAN_POINT('Ctrl Pts',(-206.92362295288,1.92528991902147,124.901935984182));
#223248=CARTESIAN_POINT('Ctrl Pts',(-207.202070576693,-3.92521078036628,
125.994154992568));
#223249=CARTESIAN_POINT('Ctrl Pts',(-207.480518200506,-6.16863452980439,
131.506717978718));
#223250=CARTESIAN_POINT('Ctrl Pts',(-207.758965824319,-2.74338450090264,
136.373848862034));
#223251=CARTESIAN_POINT('Ctrl Pts',(-208.037413448132,3.20290186254569,
136.12289213331));
#223252=CARTESIAN_POINT('Ctrl Pts',(-208.315861071945,6.20587788476857,
130.984464766326));
#223253=CARTESIAN_POINT('Ctrl Pts',(-208.594308695758,3.50595530487857,
125.680530485208));
#223254=CARTESIAN_POINT('Ctrl Pts',(-208.872756319571,-2.41576892475653,
125.085145782709));
#223255=CARTESIAN_POINT('Ctrl Pts',(-209.151203943383,-6.11751952941318,
129.745440114266));
#223256=CARTESIAN_POINT('Ctrl Pts',(-209.429651567197,-4.19756854398286,
135.378830657213));
#223257=CARTESIAN_POINT('Ctrl Pts',(-209.708099191009,1.57974287074426,
136.808506709009));
#223258=CARTESIAN_POINT('Ctrl Pts',(-209.986546814822,5.90534776198698,
132.720665821612));
#223259=CARTESIAN_POINT('Ctrl Pts',(-210.264994438635,4.80422655224024,
126.87183406841));
#223260=CARTESIAN_POINT('Ctrl Pts',(-210.543442062448,-0.711744159500396,
124.63680209928));
#223261=CARTESIAN_POINT('Ctrl Pts',(-210.821889686261,-5.57365675929581,
128.06945510647));
#223262=CARTESIAN_POINT('Ctrl Pts',(-211.100337310074,-5.31365108556781,
134.015352670796));
#223263=CARTESIAN_POINT('Ctrl Pts',(-211.378784933887,-0.170659650490228,
137.010505403884));
#223264=CARTESIAN_POINT('Ctrl Pts',(-211.657232557699,5.12915966620077,
134.302514265376));
#223265=CARTESIAN_POINT('Ctrl Pts',(-211.935680181513,5.71553182303293,
128.379890818834));
#223266=CARTESIAN_POINT('Ctrl Pts',(-212.214127805325,1.04960945375051,
124.685236675394));
#223267=CARTESIAN_POINT('Ctrl Pts',(-212.492575429138,-4.58085272725645,
126.613758498985));
#223268=CARTESIAN_POINT('Ctrl Pts',(-212.771023052951,-6.00173503901134,
132.393238947258));
#223269=CARTESIAN_POINT('Ctrl Pts',(-213.049470676764,-1.90731605097184,
136.712617831564));
#223270=CARTESIAN_POINT('Ctrl Pts',(-213.327918300577,3.93983321034183,
135.602596970618));
#223271=CARTESIAN_POINT('Ctrl Pts',(-213.60636592439,6.16646822290386,130.083231308093));
#223272=CARTESIAN_POINT('Ctrl Pts',(-213.884813548203,2.72642018733693,
125.226548251849));
#223273=CARTESIAN_POINT('Ctrl Pts',(-214.163261172015,-3.21907480736146,
125.495602268416));
#223274=CARTESIAN_POINT('Ctrl Pts',(-214.441708795829,-6.20639731464204,
130.643145860587));
#223275=CARTESIAN_POINT('Ctrl Pts',(-214.720156419641,-3.49034388913101,
135.938837938644));
#223276=CARTESIAN_POINT('Ctrl Pts',(-214.998604043455,2.43316505771265,
136.516196191791));
#223277=CARTESIAN_POINT('Ctrl Pts',(-215.277051667267,6.12071418324004,
131.844656590906));
#223278=CARTESIAN_POINT('Ctrl Pts',(-215.55549929108,4.18362598788043,126.217135811804));
#223279=CARTESIAN_POINT('Ctrl Pts',(-215.833946914893,-1.59801010884951,
124.805050530808));
#223280=CARTESIAN_POINT('Ctrl Pts',(-216.112394538706,-5.91115298268039,
128.90603813695));
#223281=CARTESIAN_POINT('Ctrl Pts',(-216.390842162519,-4.79223504130557,
134.75149136457));
#223282=CARTESIAN_POINT('Ctrl Pts',(-216.669289786332,0.730512789332353,
136.969724263749));
#223283=CARTESIAN_POINT('Ctrl Pts',(-216.947737410145,5.5819550541073,133.522289166845));
#223284=CARTESIAN_POINT('Ctrl Pts',(-217.226185033957,5.3038533178224,127.577210511344));
#223285=CARTESIAN_POINT('Ctrl Pts',(-217.50463265777,0.151769490097695,
124.597725148413));
#223286=CARTESIAN_POINT('Ctrl Pts',(-217.783080281583,-5.13978308467467,
127.321834570635));
#223287=CARTESIAN_POINT('Ctrl Pts',(-218.061527905396,-5.70812609699421,
133.24621529913));
#223288=CARTESIAN_POINT('Ctrl Pts',(-218.339975529209,-1.03098008363786,
136.9266508665));
#223289=CARTESIAN_POINT('Ctrl Pts',(-218.618423153022,4.59358626040416,
134.981000785606));
#223290=CARTESIAN_POINT('Ctrl Pts',(-218.896870776835,5.99687124029931,
129.197222430498));
#223291=CARTESIAN_POINT('Ctrl Pts',(-219.175318400648,1.88932451380644,
124.890325556239));
#223292=CARTESIAN_POINT('Ctrl Pts',(-219.45376602446,-3.95441914224089,
126.018137986666));
#223293=CARTESIAN_POINT('Ctrl Pts',(-219.732213648274,-6.16424479068368,
131.544255194914));
#223294=CARTESIAN_POINT('Ctrl Pts',(-220.010661272086,-2.70943061658779,
136.390445432439));
#223295=CARTESIAN_POINT('Ctrl Pts',(-220.289108895899,3.23521793110825,
136.103296620509));
#223296=CARTESIAN_POINT('Ctrl Pts',(-220.567556519712,6.20685924929812,
130.94668448929));
#223297=CARTESIAN_POINT('Ctrl Pts',(-220.846004143525,3.47470013931478,
125.659283672863));
#223298=CARTESIAN_POINT('Ctrl Pts',(-221.124451767337,-2.45053865016082,
125.099957217636));
#223299=CARTESIAN_POINT('Ctrl Pts',(-221.402899391151,-6.12385213560643,
129.782698811345));
#223300=CARTESIAN_POINT('Ctrl Pts',(-221.681347014963,-4.16964467523852,
135.404297694017));
#223301=CARTESIAN_POINT('Ctrl Pts',(-221.959794638777,1.61626254320698,
136.79877912285));
#223302=CARTESIAN_POINT('Ctrl Pts',(-222.238242262589,5.91690344326002,
132.684682788949));
#223303=CARTESIAN_POINT('Ctrl Pts',(-222.516689886402,4.7801991357601,126.842662238393));
#223304=CARTESIAN_POINT('Ctrl Pts',(-222.795137510215,-0.749274651793031,
124.64124895857));
#223305=CARTESIAN_POINT('Ctrl Pts',(-223.073585134028,-5.59020163845046,
128.103434208622));
#223306=CARTESIAN_POINT('Ctrl Pts',(-223.352032757841,-5.29400641590365,
134.047638880903));
#223307=CARTESIAN_POINT('Ctrl Pts',(-223.630480381654,-0.132877923733138,
137.011429272127));
#223308=CARTESIAN_POINT('Ctrl Pts',(-223.908928005467,5.15035888890098,
134.271226801972));
#223309=CARTESIAN_POINT('Ctrl Pts',(-224.187375629279,5.70066749165438,
128.345143674176));
#223310=CARTESIAN_POINT('Ctrl Pts',(-224.465823253093,1.01234116266713,
124.678960777928));
#223311=CARTESIAN_POINT('Ctrl Pts',(-224.744270876905,-4.60627723919628,
126.641721091889));
#223312=CARTESIAN_POINT('Ctrl Pts',(-225.022718500718,-5.99195188739136,
132.4297437737));
#223313=CARTESIAN_POINT('Ctrl Pts',(-225.301166124531,-1.87131547419729,
136.724118739406));
#223314=CARTESIAN_POINT('Ctrl Pts',(-225.579613748344,3.96896844094108,
135.578525187401));
#223315=CARTESIAN_POINT('Ctrl Pts',(-225.858061372157,6.16196425374224,
130.045707626623));
#223316=CARTESIAN_POINT('Ctrl Pts',(-226.13650899597,2.69241594604283,125.210055102262));
#223317=CARTESIAN_POINT('Ctrl Pts',(-226.414956619783,-3.25133108423828,
125.515296049447));
#223318=CARTESIAN_POINT('Ctrl Pts',(-226.693404243596,-6.20726368445854,
130.680928949564));
#223319=CARTESIAN_POINT('Ctrl Pts',(-226.971851867408,-3.45902420035033,
135.959989522602));
#223320=CARTESIAN_POINT('Ctrl Pts',(-227.250299491222,2.46788954115291,
136.501278998386));
#223321=CARTESIAN_POINT('Ctrl Pts',(-227.528747115034,6.12693335744362,
131.80737879213));
#223322=CARTESIAN_POINT('Ctrl Pts',(-227.807194738847,4.15562473557794,
126.191753883612));
#223323=CARTESIAN_POINT('Ctrl Pts',(-228.08564236266,-1.63450000472891,
124.81488922523));
#223324=CARTESIAN_POINT('Ctrl Pts',(-228.364089986473,-5.9225990904546,
128.942056174461));
#223325=CARTESIAN_POINT('Ctrl Pts',(-228.642537610286,-4.76811894710285,
134.780589928275));
#223326=CARTESIAN_POINT('Ctrl Pts',(-228.920985234099,0.768029573076269,
136.965163195147));
#223327=CARTESIAN_POINT('Ctrl Pts',(-229.199432857912,5.59839643592858,
133.48825986516));
#223328=CARTESIAN_POINT('Ctrl Pts',(-229.477880481725,5.28411047103341,
127.544984242401));
#223329=CARTESIAN_POINT('Ctrl Pts',(-229.756328105537,0.11398512640586,
124.59691627903));
#223330=CARTESIAN_POINT('Ctrl Pts',(-230.03477572935,-5.16088698090536,
127.353186412258));
#223331=CARTESIAN_POINT('Ctrl Pts',(-230.313223353163,-5.69315607611037,
133.280917040931));
#223332=CARTESIAN_POINT('Ctrl Pts',(-230.591670976976,-0.993692863505588,
136.932813303039));
#223333=CARTESIAN_POINT('Ctrl Pts',(-230.870118600789,4.6189255460653,134.952960938754));
#223334=CARTESIAN_POINT('Ctrl Pts',(-231.148566224602,5.98697702585963,
129.160747549691));
#223335=CARTESIAN_POINT('Ctrl Pts',(-231.427013848415,1.85328909897679,
124.878934275042));
#223336=CARTESIAN_POINT('Ctrl Pts',(-231.705461472227,-3.98348097165998,
126.042298336002));
#223337=CARTESIAN_POINT('Ctrl Pts',(-231.983909096041,-6.15962663320533,
131.581764994044));
#223338=CARTESIAN_POINT('Ctrl Pts',(-232.262356719853,-2.6753763333251,
136.406835008417));
#223339=CARTESIAN_POINT('Ctrl Pts',(-232.540804343666,3.26741411748112,
136.083504753687));
#223340=CARTESIAN_POINT('Ctrl Pts',(-232.819251967479,6.20761061637562,
130.90889893839));
#223341=CARTESIAN_POINT('Ctrl Pts',(-233.097699591292,3.44331621745904,
125.638227513236));
#223342=CARTESIAN_POINT('Ctrl Pts',(-233.376147215105,-2.48521756995422,
125.114980031328));
#223343=CARTESIAN_POINT('Ctrl Pts',(-233.654594838918,-6.12995782020675,
129.819995366479));
#223344=CARTESIAN_POINT('Ctrl Pts',(-233.933042462731,-4.14156629877734,
135.429594278462));
#223345=CARTESIAN_POINT('Ctrl Pts',(-234.211490086544,1.65272232446679,
136.788829411307));
#223346=CARTESIAN_POINT('Ctrl Pts',(-234.489937710357,5.92823987150001,
132.648630080257));
#223347=CARTESIAN_POINT('Ctrl Pts',(-234.768385334169,4.75599458724306,
126.813637210565));
#223348=CARTESIAN_POINT('Ctrl Pts',(-235.046832957982,-0.786777379437916,
124.64592419423));
#223349=CARTESIAN_POINT('Ctrl Pts',(-235.325280581795,-5.6065393706272,
128.137513394595));
#223350=CARTESIAN_POINT('Ctrl Pts',(-235.603728205608,-5.27416557488518,
134.079804910139));
#223351=CARTESIAN_POINT('Ctrl Pts',(-235.882175829421,-0.0950912731361558,
137.012123135159));
#223352=CARTESIAN_POINT('Ctrl Pts',(-236.160623453234,5.17136726315852,
134.239810872567));
#223353=CARTESIAN_POINT('Ctrl Pts',(-236.439071077047,5.68559191994549,
128.310487656705));
#223354=CARTESIAN_POINT('Ctrl Pts',(-236.71751870086,0.975035358909668,
124.672911859406));
#223355=CARTESIAN_POINT('Ctrl Pts',(-236.995966324673,-4.63153106383903,
126.669837932931));
#223356=CARTESIAN_POINT('Ctrl Pts',(-237.274413948486,-5.98194670179065,
132.466188370973));
#223357=CARTESIAN_POINT('Ctrl Pts',(-237.552861572298,-1.83524555513966,
136.735400288432));
#223358=CARTESIAN_POINT('Ctrl Pts',(-237.831309196112,3.99795659995517,
135.554276495761));
#223359=CARTESIAN_POINT('Ctrl Pts',(-238.109756819924,6.15723195072914,
130.008212057319));
#223360=CARTESIAN_POINT('Ctrl Pts',(-238.388204443737,2.65831193628575,
125.193769251723));
#223361=CARTESIAN_POINT('Ctrl Pts',(-238.66665206755,-3.28346688184612,
125.535185818711));
#223362=CARTESIAN_POINT('Ctrl Pts',(-238.945099691363,-6.20790004183648,
130.718716612347));
#223363=CARTESIAN_POINT('Ctrl Pts',(-239.223547315176,-3.42757633615586,
135.980950062836));
#223364=CARTESIAN_POINT('Ctrl Pts',(-239.501994938989,2.50252257603867,
136.486150703575));
#223365=CARTESIAN_POINT('Ctrl Pts',(-239.780442562802,6.13292549587844,
131.770063826148));
#223366=CARTESIAN_POINT('Ctrl Pts',(-240.058890186614,4.12746949507249,
126.166542877259));
#223367=CARTESIAN_POINT('Ctrl Pts',(-240.337337810428,-1.67092933361012,
124.824949861719));
#223368=CARTESIAN_POINT('Ctrl Pts',(-240.61578543424,-5.93382573414137,
128.978143220346));
#223369=CARTESIAN_POINT('Ctrl Pts',(-240.894233058053,-4.74382616849909,
134.80954115134));
#223370=CARTESIAN_POINT('Ctrl Pts',(-241.172680681866,0.805517897201924,
136.960373835741));
#223371=CARTESIAN_POINT('Ctrl Pts',(-241.451128305679,5.6146303671111,133.454131110603));
#223372=CARTESIAN_POINT('Ctrl Pts',(-241.729575929492,5.26417181958768,
127.512878750849));
#223373=CARTESIAN_POINT('Ctrl Pts',(-242.008023553305,0.0761965389532375,
124.596337428779));
#223374=CARTESIAN_POINT('Ctrl Pts',(-242.286471177117,-5.18179963857104,
127.384666138411));
#223375=CARTESIAN_POINT('Ctrl Pts',(-242.564918800931,-5.67797509323448,
133.315527013022));
#223376=CARTESIAN_POINT('Ctrl Pts',(-242.843366424743,-0.956368821719198,
136.938748647509));
#223377=CARTESIAN_POINT('Ctrl Pts',(-243.121814048556,4.64409367574132,
134.924767363992));
#223378=CARTESIAN_POINT('Ctrl Pts',(-243.400261672369,5.9768609617849,129.124333573571));
#223379=CARTESIAN_POINT('Ctrl Pts',(-243.678709296182,1.81718500983798,
124.867762562695));
#223380=CARTESIAN_POINT('Ctrl Pts',(-243.957156919995,-4.01239519172672,
126.066635145309));
#223381=CARTESIAN_POINT('Ctrl Pts',(-244.235604543808,-6.15478022849689,
131.619245986169));
#223382=CARTESIAN_POINT('Ctrl Pts',(-244.514052167621,-2.64122291300849,
136.423016982646));
#223383=CARTESIAN_POINT('Ctrl Pts',(-244.792499791433,3.29948922862226,
136.063517266237));
#223384=CARTESIAN_POINT('Ctrl Pts',(-245.070947415247,6.20813195815889,
130.871109513785));
#223385=CARTESIAN_POINT('Ctrl Pts',(-245.349395039059,3.41180470225455,
125.617362786572));
#223386=CARTESIAN_POINT('Ctrl Pts',(-245.627842662872,-2.51980439909662,
125.13021366711));
#223387=CARTESIAN_POINT('Ctrl Pts',(-245.906290286685,-6.13583635696575,
129.857328397629));
#223388=CARTESIAN_POINT('Ctrl Pts',(-246.184737910498,-4.1133344550539,
135.454719473173));
#223389=CARTESIAN_POINT('Ctrl Pts',(-246.463185534311,1.68912086349306,
136.778657943074));
#223390=CARTESIAN_POINT('Ctrl Pts',(-246.741633158124,5.93935662663147,
132.612509031482));
#223391=CARTESIAN_POINT('Ctrl Pts',(-247.020080781937,4.73161380359756,
126.784760060463));
#223392=CARTESIAN_POINT('Ctrl Pts',(-247.29852840575,-0.824250952757648,
124.650827633015));
#223393=CARTESIAN_POINT('Ctrl Pts',(-247.576976029562,-5.62266935042617,
128.171691401572));
#223394=CARTESIAN_POINT('Ctrl Pts',(-247.855423653376,-5.25412929772145,
134.111849566585));
#223395=CARTESIAN_POINT('Ctrl Pts',(-248.133871277188,-0.0573010988966442,
137.012586967267));
#223396=CARTESIAN_POINT('Ctrl Pts',(-248.412318901001,5.19218401050035,
134.208267641291));
#223397=CARTESIAN_POINT('Ctrl Pts',(-248.690766524814,5.67030566653712,
128.275924050614));
#223398=CARTESIAN_POINT('Ctrl Pts',(-248.969214148627,0.937693424858449,
124.667090143972));
#223399=CARTESIAN_POINT('Ctrl Pts',(-249.24766177244,-4.65661326539506,
126.698107980232));
#223400=CARTESIAN_POINT('Ctrl Pts',(-249.526109396252,-5.97171985295489,
132.502571388608));
#223401=CARTESIAN_POINT('Ctrl Pts',(-249.804557020066,-1.79910763038337,
136.746462060605));
#223402=CARTESIAN_POINT('Ctrl Pts',(-250.083004643878,4.02679661321771,
135.52985179424));
#223403=CARTESIAN_POINT('Ctrl Pts',(-250.361452267692,6.15227148922063,
129.970745989595));
#223404=CARTESIAN_POINT('Ctrl Pts',(-250.639899891504,2.62410942180459,
125.177691303707));
#223405=CARTESIAN_POINT('Ctrl Pts',(-250.918347515317,-3.31548100938434,
125.555270839195));
#223406=CARTESIAN_POINT('Ctrl Pts',(-251.19679513913,-6.20830636318893,
130.756507448682));
#223407=CARTESIAN_POINT('Ctrl Pts',(-251.475242762943,-3.39600146187203,
136.001718782677));
#223408=CARTESIAN_POINT('Ctrl Pts',(-251.753690386756,2.53706287905323,
136.47081186788));
#223409=CARTESIAN_POINT('Ctrl Pts',(-252.032138010569,6.13869037645988,
131.732713075798));
#223410=CARTESIAN_POINT('Ctrl Pts',(-252.310585634382,4.09916130974965,
126.141503726722));
#223411=CARTESIAN_POINT('Ctrl Pts',(-252.589033258195,-1.70729674574642,
124.835232067896));
#223412=CARTESIAN_POINT('Ctrl Pts',(-252.867480882007,-5.94483249743877,
129.014297936587));
#223413=CARTESIAN_POINT('Ctrl Pts',(-253.14592850582,-4.71935760622846,
134.838343962485));
#223414=CARTESIAN_POINT('Ctrl Pts',(-253.424376129633,0.842976373616159,
136.955356360136));
#223415=CARTESIAN_POINT('Ctrl Pts',(-253.702823753446,5.63065624411703,
133.419904173236));
#223416=CARTESIAN_POINT('Ctrl Pts',(-253.981271377259,5.24403810606461,
127.480895216153));
#223417=CARTESIAN_POINT('Ctrl Pts',(-254.259719001072,0.0384051209378723,
124.595988638398));
#223418=CARTESIAN_POINT('Ctrl Pts',(-254.538166624885,-5.20252026939218,
127.416272546179));
#223419=CARTESIAN_POINT('Ctrl Pts',(-254.816614248698,-5.66258373611722,
133.350044001689));
#223420=CARTESIAN_POINT('Ctrl Pts',(-255.095061872511,-0.919009293725241,
136.944456550123));
#223421=CARTESIAN_POINT('Ctrl Pts',(-255.373509496324,4.6690896269236,134.896421351226));
#223422=CARTESIAN_POINT('Ctrl Pts',(-255.651957120136,5.96652359266914,
129.087981388513));
#223423=CARTESIAN_POINT('Ctrl Pts',(-255.93040474395,1.78101326373629,124.856811707331));
#223424=CARTESIAN_POINT('Ctrl Pts',(-256.208852367762,-4.04116012583712,
126.091145862189));
#223425=CARTESIAN_POINT('Ctrl Pts',(-256.487299991575,-6.14970689884083,
131.656699899059));
#223426=CARTESIAN_POINT('Ctrl Pts',(-256.765747615388,-2.60696946356087,
136.438984870644));
#223427=CARTESIAN_POINT('Ctrl Pts',(-257.044195239201,3.33143800190474,
136.043346010603));
#223428=CARTESIAN_POINT('Ctrl Pts',(-257.322642863014,6.2084309480058,130.833296634437));
#223429=CARTESIAN_POINT('Ctrl Pts',(-257.601090486826,3.38015223603414,
125.596729883064));
#223430=CARTESIAN_POINT('Ctrl Pts',(-257.87953811064,-2.5542704291637,125.145582755354));
#223431=CARTESIAN_POINT('Ctrl Pts',(-258.157985734452,-6.14153931545366,
129.894837769574));
#223432=CARTESIAN_POINT('Ctrl Pts',(-258.436433358265,-4.08485240479644,
135.479405634932));
#223433=CARTESIAN_POINT('Ctrl Pts',(-258.714880982078,1.72527217059264,
136.768768758555));
#223434=CARTESIAN_POINT('Ctrl Pts',(-258.993328605892,5.95060195420752,
132.575369498931));
#223435=CARTESIAN_POINT('Ctrl Pts',(-259.271776229703,4.70639920604184,
126.75783223591));
#223436=CARTESIAN_POINT('Ctrl Pts',(-259.550223853517,-0.860449444711704,
124.652528659269));
#223437=CARTESIAN_POINT('Ctrl Pts',(-259.82867147733,-5.64095031490746,
128.212697490595));
#223438=CARTESIAN_POINT('Ctrl Pts',(-260.060711163841,-5.29799179572588,
133.142936715762));
#223439=CARTESIAN_POINT('Ctrl Pts',(-260.246372125917,-2.62679689981868,
135.594171577488));
#223440=CARTESIAN_POINT('Ctrl Pts',(-260.339217213388,-0.889986900407246,
136.05080276614));
#223441=CARTESIAN_POINT('Ctrl Pts',(-260.385654363559,-0.0148419801173944,
136.053268468065));
#223442=CARTESIAN_POINT('Ctrl Pts',(209.997106195361,2.85369542052185,134.803838223542));
#223443=CARTESIAN_POINT('Ctrl Pts',(209.950688331758,3.52024512455777,134.328247120061));
#223444=CARTESIAN_POINT('Ctrl Pts',(209.857862530854,4.598911638141,133.039517383424));
#223445=CARTESIAN_POINT('Ctrl Pts',(209.672220855345,5.31158968331849,129.722011776094));
#223446=CARTESIAN_POINT('Ctrl Pts',(209.440181168834,2.90445768035623,125.771581499823));
#223447=CARTESIAN_POINT('Ctrl Pts',(209.161733545021,-2.67328939945229,
125.640965885288));
#223448=CARTESIAN_POINT('Ctrl Pts',(208.883285921209,-5.78445646322271,
130.262241799363));
#223449=CARTESIAN_POINT('Ctrl Pts',(208.604838297395,-3.58517659481558,
135.378114005881));
#223450=CARTESIAN_POINT('Ctrl Pts',(208.326390673583,1.91144119617671,136.292814641374));
#223451=CARTESIAN_POINT('Ctrl Pts',(208.04794304977,5.65009034124608,132.162897902674));
#223452=CARTESIAN_POINT('Ctrl Pts',(207.769495425957,4.19734896093999,126.785079177362));
#223453=CARTESIAN_POINT('Ctrl Pts',(207.491047802144,-1.1129569716493,125.100504449821));
#223454=CARTESIAN_POINT('Ctrl Pts',(207.212600178331,-5.4002948496084,128.657642803108));
#223455=CARTESIAN_POINT('Ctrl Pts',(206.934152554519,-4.72513942780656,
134.187431620732));
#223456=CARTESIAN_POINT('Ctrl Pts',(206.655704930705,0.292248586550605,
136.608384944684));
#223457=CARTESIAN_POINT('Ctrl Pts',(206.377257306892,5.04104249491135,133.695701483205));
#223458=CARTESIAN_POINT('Ctrl Pts',(206.09880968308,5.15738153042831,128.12602865207));
#223459=CARTESIAN_POINT('Ctrl Pts',(205.820362059267,0.534329935251406,
125.017605890956));
#223460=CARTESIAN_POINT('Ctrl Pts',(205.541914435454,-4.57974002364783,
127.226931288585));
#223461=CARTESIAN_POINT('Ctrl Pts',(205.263466811641,-5.48525514562618,
132.723737743954));
#223462=CARTESIAN_POINT('Ctrl Pts',(204.985019187828,-1.35008742798131,
136.456731302353));
#223463=CARTESIAN_POINT('Ctrl Pts',(204.706571564015,4.02574397595362,134.995471850294));
#223464=CARTESIAN_POINT('Ctrl Pts',(204.428123940202,5.70211370766606,129.682786179275));
#223465=CARTESIAN_POINT('Ctrl Pts',(204.149676316389,2.13851930815143,125.40077248911));
#223466=CARTESIAN_POINT('Ctrl Pts',(203.871228692576,-3.39026975841633,
126.084392381055));
#223467=CARTESIAN_POINT('Ctrl Pts',(203.592781068764,-5.8035665963141,131.105432460946));
#223468=CARTESIAN_POINT('Ctrl Pts',(203.314333444951,-2.88366922283368,
135.849802245147));
#223469=CARTESIAN_POINT('Ctrl Pts',(203.035885821138,2.68617927581077,135.957657646429));
#223470=CARTESIAN_POINT('Ctrl Pts',(202.757438197325,5.78756025537181,131.329884836407));
#223471=CARTESIAN_POINT('Ctrl Pts',(202.478990573512,3.57045609392238,126.219180939555));
#223472=CARTESIAN_POINT('Ctrl Pts',(202.200542949699,-1.92772278905516,
125.322033169903));
#223473=CARTESIAN_POINT('Ctrl Pts',(201.922095325886,-5.6544186046078,129.462876497226));
#223474=CARTESIAN_POINT('Ctrl Pts',(201.643647702073,-4.18497995558374,
134.836478196445));
#223475=CARTESIAN_POINT('Ctrl Pts',(201.36520007826,1.13025082464198,136.504760820331));
#223476=CARTESIAN_POINT('Ctrl Pts',(201.086752454448,5.4068363130258,132.934654138033));
#223477=CARTESIAN_POINT('Ctrl Pts',(200.808304830635,4.71480336828096,127.406911780982));
#223478=CARTESIAN_POINT('Ctrl Pts',(200.529857206822,-0.309903540913717,
125.001258930184));
#223479=CARTESIAN_POINT('Ctrl Pts',(200.251409583008,-5.04982423566531,
127.928373032793));
#223480=CARTESIAN_POINT('Ctrl Pts',(199.972961959197,-5.14920315545485,
133.498379226012));
#223481=CARTESIAN_POINT('Ctrl Pts',(199.694514335383,-0.516715927947778,
136.59271392819));
#223482=CARTESIAN_POINT('Ctrl Pts',(199.416066711571,4.59060799437092,134.367834714685));
#223483=CARTESIAN_POINT('Ctrl Pts',(199.137619087757,5.47938743352869,128.868296891315));
#223484=CARTESIAN_POINT('Ctrl Pts',(198.859171463945,1.33287750423228,125.147907050397));
#223485=CARTESIAN_POINT('Ctrl Pts',(198.580723840131,-4.03848173676817,
126.625521704588));
#223486=CARTESIAN_POINT('Ctrl Pts',(198.302276216319,-5.69867355247927,
131.943285172176));
#223487=CARTESIAN_POINT('Ctrl Pts',(198.023828592506,-2.12206276914206,
136.214432613634));
#223488=CARTESIAN_POINT('Ctrl Pts',(197.745380968693,3.4046200305072,135.513988187415));
#223489=CARTESIAN_POINT('Ctrl Pts',(197.46693334488,5.80262334705539,130.485626102603));
#223490=CARTESIAN_POINT('Ctrl Pts',(197.188485721067,2.86829928156946,125.750165465994));
#223491=CARTESIAN_POINT('Ctrl Pts',(196.910038097254,-2.70185169946893,
125.65926326252));
#223492=CARTESIAN_POINT('Ctrl Pts',(196.631590473441,-5.78913296148881,
130.296454176353));
#223493=CARTESIAN_POINT('Ctrl Pts',(196.353142849628,-3.5564838467683,135.400386297052));
#223494=CARTESIAN_POINT('Ctrl Pts',(196.074695225815,1.94440017923737,136.280795346639));
#223495=CARTESIAN_POINT('Ctrl Pts',(195.796247602003,5.6584754297534,132.128628418917));
#223496=CARTESIAN_POINT('Ctrl Pts',(195.51779997819,4.17268819221861,126.759524075833));
#223497=CARTESIAN_POINT('Ctrl Pts',(195.239352354377,-1.14759564681435,
125.107426913349));
#223498=CARTESIAN_POINT('Ctrl Pts',(194.960904730564,-5.41329514958902,
128.690533514357));
#223499=CARTESIAN_POINT('Ctrl Pts',(194.682457106751,-4.70444086406131,
134.216143957018));
#223500=CARTESIAN_POINT('Ctrl Pts',(194.404009482938,0.327564750825761,
136.606492185605));
#223501=CARTESIAN_POINT('Ctrl Pts',(194.125561859125,5.0585543621317,133.664964953048));
#223502=CARTESIAN_POINT('Ctrl Pts',(193.847114235312,5.14097963875765,128.094682084473));
#223503=CARTESIAN_POINT('Ctrl Pts',(193.568666611499,0.499095778182989,
125.014461412655));
#223504=CARTESIAN_POINT('Ctrl Pts',(193.290218987687,-4.60143272035756,
127.254875257849));
#223505=CARTESIAN_POINT('Ctrl Pts',(193.011771363874,-5.4734693413749,132.757092746623));
#223506=CARTESIAN_POINT('Ctrl Pts',(192.733323740061,-1.31565503151135,
136.464844805061));
#223507=CARTESIAN_POINT('Ctrl Pts',(192.454876116248,4.05118197898966,134.970888425217));
#223508=CARTESIAN_POINT('Ctrl Pts',(192.176428492435,5.69518066204141,129.648096536341));
#223509=CARTESIAN_POINT('Ctrl Pts',(191.897980868622,2.1055865417199,125.38785485147));
#223510=CARTESIAN_POINT('Ctrl Pts',(191.619533244809,-3.4189387468211,126.105117354624));
#223511=CARTESIAN_POINT('Ctrl Pts',(191.341085620997,-5.80162635147675,
131.140754845624));
#223512=CARTESIAN_POINT('Ctrl Pts',(191.062637997183,-2.85290276432908,
135.867262474811));
#223513=CARTESIAN_POINT('Ctrl Pts',(190.784190373371,2.71749909118881,135.941210633695));
#223514=CARTESIAN_POINT('Ctrl Pts',(190.505742749557,5.79065203911519,131.29464457683));
#223515=CARTESIAN_POINT('Ctrl Pts',(190.227295125745,3.54247865217362,126.197531513104));
#223516=CARTESIAN_POINT('Ctrl Pts',(189.948847501932,-1.96105955641241,
125.333869340265));
#223517=CARTESIAN_POINT('Ctrl Pts',(189.670399878119,-5.66247983574075,
129.497321402909));
#223518=CARTESIAN_POINT('Ctrl Pts',(189.391952254306,-4.160357773542,134.861878651407));
#223519=CARTESIAN_POINT('Ctrl Pts',(189.113504630493,1.16492983776554,136.497775047581));
#223520=CARTESIAN_POINT('Ctrl Pts',(188.83505700668,5.41970383815296,132.901701721328));
#223521=CARTESIAN_POINT('Ctrl Pts',(188.556609382867,4.69403477852959,127.378274381527));
#223522=CARTESIAN_POINT('Ctrl Pts',(188.278161759054,-0.345222926215044,
125.003252919028));
#223523=CARTESIAN_POINT('Ctrl Pts',(187.999714135242,-5.0672376268456,127.959166031618));
#223524=CARTESIAN_POINT('Ctrl Pts',(187.721266511429,-5.13270849672517,
133.529673973213));
#223525=CARTESIAN_POINT('Ctrl Pts',(187.442818887616,-0.48147100486422,
136.595752079925));
#223526=CARTESIAN_POINT('Ctrl Pts',(187.164371263803,4.61221481930072,134.339824357932));
#223527=CARTESIAN_POINT('Ctrl Pts',(186.88592363999,5.4675005437485,128.834978175547));
#223528=CARTESIAN_POINT('Ctrl Pts',(186.607476016177,1.29842037074208,125.139898247696));
#223529=CARTESIAN_POINT('Ctrl Pts',(186.329028392364,-4.06384469161484,
126.650182513385));
#223530=CARTESIAN_POINT('Ctrl Pts',(186.050580768551,-5.69163501222784,
131.977953513933));
#223531=CARTESIAN_POINT('Ctrl Pts',(185.772133144738,-2.08909080843167,
136.227249975919));
#223532=CARTESIAN_POINT('Ctrl Pts',(185.493685520926,3.4332257905535,135.493176040453));
#223533=CARTESIAN_POINT('Ctrl Pts',(185.215237897112,5.80057561042411,130.450309792719));
#223534=CARTESIAN_POINT('Ctrl Pts',(184.9367902733,2.83747981818726,125.732798956676));
#223535=CARTESIAN_POINT('Ctrl Pts',(184.658342649487,-2.73312130836828,
125.675805527429));
#223536=CARTESIAN_POINT('Ctrl Pts',(184.379895025674,-5.79211747293216,
130.331703682172));
#223537=CARTESIAN_POINT('Ctrl Pts',(184.101447401861,-3.52844064054064,
135.421950469967));
#223538=CARTESIAN_POINT('Ctrl Pts',(183.822999778048,1.97770076659953,136.26885776521));
#223539=CARTESIAN_POINT('Ctrl Pts',(183.544552154236,5.66643178528845,132.094159137294));
#223540=CARTESIAN_POINT('Ctrl Pts',(183.266104530422,4.14798881387936,126.734198679909));
#223541=CARTESIAN_POINT('Ctrl Pts',(182.98765690661,-1.18225323696583,125.114518204765));
#223542=CARTESIAN_POINT('Ctrl Pts',(182.709209282797,-5.42606231932092,
128.72352494273));
#223543=CARTESIAN_POINT('Ctrl Pts',(182.430761658984,-4.68358520810093,
134.244718011395));
#223544=CARTESIAN_POINT('Ctrl Pts',(182.152314035171,0.362877903506298,
136.604390705933));
#223545=CARTESIAN_POINT('Ctrl Pts',(181.873866411358,5.07587394936235,133.634119096483));
#223546=CARTESIAN_POINT('Ctrl Pts',(181.595418787545,5.12438980598236,128.063437686296));
#223547=CARTESIAN_POINT('Ctrl Pts',(181.316971163732,0.463841771263853,
125.011530548415));
#223548=CARTESIAN_POINT('Ctrl Pts',(181.038523539919,-4.62295419131585,
127.282951248603));
#223549=CARTESIAN_POINT('Ctrl Pts',(180.760075916106,-5.46148109594396,
132.790375128456));
#223550=CARTESIAN_POINT('Ctrl Pts',(180.481628292294,-1.2811736815839,136.472748695004));
#223551=CARTESIAN_POINT('Ctrl Pts',(180.203180668481,4.07646975733793,134.946150534538));
#223552=CARTESIAN_POINT('Ctrl Pts',(179.924733044668,5.68803663588505,129.61344977806));
#223553=CARTESIAN_POINT('Ctrl Pts',(179.646285420855,2.07257572209157,125.37513790386));
#223554=CARTESIAN_POINT('Ctrl Pts',(179.367837797042,-3.44748102935117,
126.12601647128));
#223555=CARTESIAN_POINT('Ctrl Pts',(179.089390173229,-5.79947113363144,
131.176064759319));
#223556=CARTESIAN_POINT('Ctrl Pts',(178.810942549416,-2.82203058602,135.884535099843));
#223557=CARTESIAN_POINT('Ctrl Pts',(178.532494925603,2.74871820628535,135.924573271475));
#223558=CARTESIAN_POINT('Ctrl Pts',(178.254047301791,5.79352924936408,131.259386150458));
#223559=CARTESIAN_POINT('Ctrl Pts',(177.975599677977,3.51436994191561,126.176052793945));
#223560=CARTESIAN_POINT('Ctrl Pts',(177.697152054165,-1.99432365563702,
125.345908221933));
#223561=CARTESIAN_POINT('Ctrl Pts',(177.418704430351,-5.6703312417861,129.531814741282));
#223562=CARTESIAN_POINT('Ctrl Pts',(177.140256806539,-4.135581427815,134.887128753614));
#223563=CARTESIAN_POINT('Ctrl Pts',(176.861809182726,1.19956568393359,136.490578303229));
#223564=CARTESIAN_POINT('Ctrl Pts',(176.583361558913,5.43237053418876,132.868671586896));
#223565=CARTESIAN_POINT('Ctrl Pts',(176.3049139351,4.67309224957875,127.349763936946));
#223566=CARTESIAN_POINT('Ctrl Pts',(176.026466311287,-0.380529519146142,
125.005461870054));
#223567=CARTESIAN_POINT('Ctrl Pts',(175.748018687475,-5.08446324967622,
127.990064460173));
#223568=CARTESIAN_POINT('Ctrl Pts',(175.469571063661,-5.11602364359241,
133.560867732924));
#223569=CARTESIAN_POINT('Ctrl Pts',(175.191123439849,-0.446208240696769,
136.59857562952));
#223570=CARTESIAN_POINT('Ctrl Pts',(174.912675816035,4.63365073691483,134.311682993269));
#223571=CARTESIAN_POINT('Ctrl Pts',(174.634228192223,5.45541105372469,128.801732435971));
#223572=CARTESIAN_POINT('Ctrl Pts',(174.35578056841,1.26391512380778,125.132099343732));
#223573=CARTESIAN_POINT('Ctrl Pts',(174.077332944597,-4.089057059202,126.674997256779));
#223574=CARTESIAN_POINT('Ctrl Pts',(173.798885320784,-5.68438556634791,
132.012578367773));
#223575=CARTESIAN_POINT('Ctrl Pts',(173.520437696972,-2.0560414356932,136.239866391045));
#223576=CARTESIAN_POINT('Ctrl Pts',(173.241990073158,3.46170433115548,135.472190147709));
#223577=CARTESIAN_POINT('Ctrl Pts',(172.963542449346,5.79831293133042,130.41500660232));
#223578=CARTESIAN_POINT('Ctrl Pts',(172.685094825533,2.80655521094699,125.715620375941));
#223579=CARTESIAN_POINT('Ctrl Pts',(172.40664720172,-2.76428964045241,125.692537832834));
#223580=CARTESIAN_POINT('Ctrl Pts',(172.128199577907,-5.79488735533246,
130.366970702468));
#223581=CARTESIAN_POINT('Ctrl Pts',(171.849751954094,-3.50026668664755,
135.443343536393));
#223582=CARTESIAN_POINT('Ctrl Pts',(171.571304330281,2.01092806953244,136.256717694829));
#223583=CARTESIAN_POINT('Ctrl Pts',(171.292856706468,5.6741781691098,132.059642061713));
#223584=CARTESIAN_POINT('Ctrl Pts',(171.014409082656,4.12313573028927,126.709024105332));
#223585=CARTESIAN_POINT('Ctrl Pts',(170.735961458842,-1.21686701828875,
125.121820335384));
#223586=CARTESIAN_POINT('Ctrl Pts',(170.45751383503,-5.43862842431808,128.756593477234));
#223587=CARTESIAN_POINT('Ctrl Pts',(170.179066211217,-4.66255600016836,
134.273164582064));
#223588=CARTESIAN_POINT('Ctrl Pts',(169.900618587404,0.398177609612544,
136.602074304013));
#223589=CARTESIAN_POINT('Ctrl Pts',(169.62217096359,5.09300544821711,133.603168382178));
#223590=CARTESIAN_POINT('Ctrl Pts',(169.343723339778,5.10761008705837,128.032294854024));
#223591=CARTESIAN_POINT('Ctrl Pts',(169.065275715965,0.428570576517446,
125.008814339624));
#223592=CARTESIAN_POINT('Ctrl Pts',(168.786828092152,-4.64430435700642,
127.311157726477));
#223593=CARTESIAN_POINT('Ctrl Pts',(168.508380468339,-5.4492904733226,132.823583917792));
#223594=CARTESIAN_POINT('Ctrl Pts',(168.229932844526,-1.24664485729461,
136.480442540741));
#223595=CARTESIAN_POINT('Ctrl Pts',(167.951485220714,4.10160648060013,134.92125916831));
#223596=CARTESIAN_POINT('Ctrl Pts',(167.673037596901,5.6806818374394,129.578847149419));
#223597=CARTESIAN_POINT('Ctrl Pts',(167.394589973088,2.03948810240773,125.362622138095));
#223598=CARTESIAN_POINT('Ctrl Pts',(167.116142349275,-3.47589556420378,
126.147088945699));
#223599=CARTESIAN_POINT('Ctrl Pts',(166.837694725462,-5.79710101425052,
131.21136089938));
#223600=CARTESIAN_POINT('Ctrl Pts',(166.559247101649,-2.79105383632985,
135.901619477142));
#223601=CARTESIAN_POINT('Ctrl Pts',(166.280799477836,2.77983546661788,135.907746177893));
#223602=CARTESIAN_POINT('Ctrl Pts',(166.002351854023,5.79619177825601,131.224110862948));
#223603=CARTESIAN_POINT('Ctrl Pts',(165.72390423021,3.48613100538707,126.154745578436));
#223604=CARTESIAN_POINT('Ctrl Pts',(165.445456606397,-2.02751385446508,
125.358149368562));
#223605=CARTESIAN_POINT('Ctrl Pts',(165.167008982585,-5.67797253162207,
129.566355234311));
#223606=CARTESIAN_POINT('Ctrl Pts',(164.888561358772,-4.11065183659732,
134.912227567346));
#223607=CARTESIAN_POINT('Ctrl Pts',(164.610113734959,1.23415707975413,136.483170853989));
#223608=CARTESIAN_POINT('Ctrl Pts',(164.331666111146,5.44483593173667,132.835564958663));
#223609=CARTESIAN_POINT('Ctrl Pts',(164.053218487333,4.65197655747607,127.321381503715));
#223610=CARTESIAN_POINT('Ctrl Pts',(163.77477086352,-0.415822011415935,
125.007885701408));
#223611=CARTESIAN_POINT('Ctrl Pts',(163.496323239708,-5.10150046585131,
128.021067173507));
#223612=CARTESIAN_POINT('Ctrl Pts',(163.217875615894,-5.09914921432216,
133.591959349252));
#223613=CARTESIAN_POINT('Ctrl Pts',(162.939427992082,-0.41092894211879,
136.601184472346));
#223614=CARTESIAN_POINT('Ctrl Pts',(162.660980368268,4.65491495289691,134.283411663486));
#223615=CARTESIAN_POINT('Ctrl Pts',(162.382532744456,5.443119411438,128.768560904517));
#223616=CARTESIAN_POINT('Ctrl Pts',(162.104085120643,1.22936304203373,125.124510627495));
#223617=CARTESIAN_POINT('Ctrl Pts',(161.82563749683,-4.11411790527609,126.69996501525));
#223618=CARTESIAN_POINT('Ctrl Pts',(161.547189873017,-5.67692548347038,
132.04715845066));
#223619=CARTESIAN_POINT('Ctrl Pts',(161.268742249204,-2.02291587558315,
136.252281391507));
#223620=CARTESIAN_POINT('Ctrl Pts',(160.990294625391,3.49005459703047,135.451031286826));
#223621=CARTESIAN_POINT('Ctrl Pts',(160.711847001578,5.79583539361873,130.379717839577));
#223622=CARTESIAN_POINT('Ctrl Pts',(160.433399377766,2.77552660577121,125.698630360346));
#223623=CARTESIAN_POINT('Ctrl Pts',(160.154951753952,-2.79535554076737,
125.70945955871));
#223624=CARTESIAN_POINT('Ctrl Pts',(159.87650413014,-5.79744250605075,130.402253930408));
#223625=CARTESIAN_POINT('Ctrl Pts',(159.598056506327,-3.47196302908515,
135.4645647036));
#223626=CARTESIAN_POINT('Ctrl Pts',(159.319608882514,2.04408085678626,136.244375585352));
#223627=CARTESIAN_POINT('Ctrl Pts',(159.041161258701,5.68171429417248,132.025078471215));
#223628=CARTESIAN_POINT('Ctrl Pts',(158.762713634888,4.09812986238831,126.684001284956));
#223629=CARTESIAN_POINT('Ctrl Pts',(158.484266011075,-1.25143570815684,
125.129333034622));
#223630=CARTESIAN_POINT('Ctrl Pts',(158.205818387262,-5.450992998939,128.789737892503));
#223631=CARTESIAN_POINT('Ctrl Pts',(157.927370763449,-4.64135401950845,
134.301482614925));
#223632=CARTESIAN_POINT('Ctrl Pts',(157.648923139637,0.43346256110109,136.59954306568));
#223633=CARTESIAN_POINT('Ctrl Pts',(157.370475515823,5.10994822388206,133.572113957021));
#223634=CARTESIAN_POINT('Ctrl Pts',(157.092027892011,5.09064110376424,128.001254741669));
#223635=CARTESIAN_POINT('Ctrl Pts',(156.813580268198,0.39328350093061,125.006312886931));
#223636=CARTESIAN_POINT('Ctrl Pts',(156.535132644385,-4.66548242629113,
127.339493646268));
#223637=CARTESIAN_POINT('Ctrl Pts',(156.256685020572,-5.43689792523874,
132.856717884066));
#223638=CARTESIAN_POINT('Ctrl Pts',(155.978237396759,-1.21206983812162,
136.487926057176));
#223639=CARTESIAN_POINT('Ctrl Pts',(155.699789772946,4.12659121732586,134.896215248893));
#223640=CARTESIAN_POINT('Ctrl Pts',(155.421342149133,5.67311653923917,129.544289932631));
#223641=CARTESIAN_POINT('Ctrl Pts',(155.142894525321,2.0063249087422,125.350308017949));
#223642=CARTESIAN_POINT('Ctrl Pts',(154.864446901507,-3.50418129846815,
126.168333997033));
#223643=CARTESIAN_POINT('Ctrl Pts',(154.585999277695,-5.79451608115961,
131.246641957895));
#223644=CARTESIAN_POINT('Ctrl Pts',(154.307551653882,-2.75997366311328,
135.918514973638));
#223645=CARTESIAN_POINT('Ctrl Pts',(154.029104030069,2.81084971912495,135.890729976482));
#223646=CARTESIAN_POINT('Ctrl Pts',(153.750656406256,5.79863952713012,131.188820021437));
#223647=CARTESIAN_POINT('Ctrl Pts',(153.472208782443,3.457762888992,126.133610656121));
#223648=CARTESIAN_POINT('Ctrl Pts',(153.19376115863,-2.0606289230217,125.370592326552));
#223649=CARTESIAN_POINT('Ctrl Pts',(152.915313534817,-5.68540342209783,
129.600941602086));
#223650=CARTESIAN_POINT('Ctrl Pts',(152.636865911004,-4.08556992366409,
134.937174162558));
#223651=CARTESIAN_POINT('Ctrl Pts',(152.358418287191,1.26870274343019,136.475552974349));
#223652=CARTESIAN_POINT('Ctrl Pts',(152.079970663379,5.45709956888678,132.802383063404));
#223653=CARTESIAN_POINT('Ctrl Pts',(151.801523039566,4.63068848467127,127.293128133558));
#223654=CARTESIAN_POINT('Ctrl Pts',(151.523075415753,-0.451099095248245,
125.010524323271));
#223655=CARTESIAN_POINT('Ctrl Pts',(151.24462779194,-5.11834864405056,128.052173022803));
#223656=CARTESIAN_POINT('Ctrl Pts',(150.966180168127,-5.08208583420252,
133.622947670083));
#223657=CARTESIAN_POINT('Ctrl Pts',(150.687732544314,-0.375634416417742,
136.603578511732));
#223658=CARTESIAN_POINT('Ctrl Pts',(150.409284920501,4.67600667929353,134.255011416186));
#223659=CARTESIAN_POINT('Ctrl Pts',(150.130837296688,5.43062607235983,128.735464810371));
#223660=CARTESIAN_POINT('Ctrl Pts',(149.852389672876,1.19476540576009,125.117132380189));
#223661=CARTESIAN_POINT('Ctrl Pts',(149.573942049063,-4.13902630119825,
126.725084863609));
#223662=CARTESIAN_POINT('Ctrl Pts',(149.29549442525,-5.66925504003138,132.081692481218));
#223663=CARTESIAN_POINT('Ctrl Pts',(149.017046801437,-1.98971535558138,
136.264494517259));
#223664=CARTESIAN_POINT('Ctrl Pts',(148.738599177624,3.5182755376489,135.429700241853));
#223665=CARTESIAN_POINT('Ctrl Pts',(148.460151553811,5.79314308909515,130.344444812129));
#223666=CARTESIAN_POINT('Ctrl Pts',(148.181703929998,2.74439515243632,125.681829539465));
#223667=CARTESIAN_POINT('Ctrl Pts',(147.903256306185,-2.82631785815477,
125.726570078021));
#223668=CARTESIAN_POINT('Ctrl Pts',(147.624808682372,-5.79978283040501,
130.437552058559));
#223669=CARTESIAN_POINT('Ctrl Pts',(147.346361058559,-3.4435307166558,135.48561318523));
#223670=CARTESIAN_POINT('Ctrl Pts',(147.067913434747,2.07715789987228,136.23183189412));
#223671=CARTESIAN_POINT('Ctrl Pts',(146.789465810933,5.68903988122249,131.990469646568));
#223672=CARTESIAN_POINT('Ctrl Pts',(146.511018187121,4.07297213677825,126.65913114601));
#223673=CARTESIAN_POINT('Ctrl Pts',(146.232570563308,-1.2859580256146,125.137056024094));
#223674=CARTESIAN_POINT('Ctrl Pts',(145.954122939495,-5.46315558500969,
128.822956960357));
#223675=CARTESIAN_POINT('Ctrl Pts',(145.675675315682,-4.61998005176852,
134.329671060644));
#223676=CARTESIAN_POINT('Ctrl Pts',(145.397227691869,0.468731450475054,
136.596797084732));
#223677=CARTESIAN_POINT('Ctrl Pts',(145.118780068056,5.12670164853643,133.540956971746));
#223678=CARTESIAN_POINT('Ctrl Pts',(144.840332444244,5.07348348489189,127.970318499433));
#223679=CARTESIAN_POINT('Ctrl Pts',(144.56188482043,0.357981852079004,125.004026283029));
#223680=CARTESIAN_POINT('Ctrl Pts',(144.283437196618,-4.6864876144088,127.367957957979));
#223681=CARTESIAN_POINT('Ctrl Pts',(144.004989572805,-5.42430391090288,
132.889775799486));
#223682=CARTESIAN_POINT('Ctrl Pts',(143.726541948992,-1.17744990525502,
136.495198967004));
#223683=CARTESIAN_POINT('Ctrl Pts',(143.448094325179,4.15142304169647,134.871019704297));
#223684=CARTESIAN_POINT('Ctrl Pts',(143.169646701366,5.66534102161933,129.509779408224));
#223685=CARTESIAN_POINT('Ctrl Pts',(142.891199077553,1.9730873699693,125.338195999729));
#223686=CARTESIAN_POINT('Ctrl Pts',(142.61275145374,-3.53233718400576,126.189750838038));
#223687=CARTESIAN_POINT('Ctrl Pts',(142.334303829928,-5.79171643014443,
131.281906627513));
#223688=CARTESIAN_POINT('Ctrl Pts',(142.055856206114,-2.72879121805762,
135.935220963265));
#223689=CARTESIAN_POINT('Ctrl Pts',(141.777408582302,2.84175981456215,135.873525297782));
#223690=CARTESIAN_POINT('Ctrl Pts',(141.498960958489,5.80087240528401,131.153514933643));
#223691=CARTESIAN_POINT('Ctrl Pts',(141.220513334676,3.42926664392146,126.112648810165));
#223692=CARTESIAN_POINT('Ctrl Pts',(140.942065710863,-2.09366763421581,
125.383236634823));
#223693=CARTESIAN_POINT('Ctrl Pts',(140.66361808705,-5.69262363785895,129.635572562993));
#223694=CARTESIAN_POINT('Ctrl Pts',(140.385170463237,-4.06033661843482,
134.961967614844));
#223695=CARTESIAN_POINT('Ctrl Pts',(140.106722839424,1.30320139485961,136.467724946589));
#223696=CARTESIAN_POINT('Ctrl Pts',(139.828275215611,5.46916099120554,132.769127130691));
#223697=CARTESIAN_POINT('Ctrl Pts',(139.549827591798,4.60922882000175,127.26500487341));
#223698=CARTESIAN_POINT('Ctrl Pts',(139.271379967986,-0.486359463437733,
125.013377637868));
#223699=CARTESIAN_POINT('Ctrl Pts',(138.992932344173,-5.13500715995863,
128.083380855422));
#223700=CARTESIAN_POINT('Ctrl Pts',(138.71448472036,-5.06483413552331,133.653831547135));
#223701=CARTESIAN_POINT('Ctrl Pts',(138.436037096547,-0.340325971445257,
136.605757658967));
#223702=CARTESIAN_POINT('Ctrl Pts',(138.157589472734,4.69692513454305,134.226483303753));
#223703=CARTESIAN_POINT('Ctrl Pts',(137.879141848921,5.41793149943546,128.70244537992));
#223704=CARTESIAN_POINT('Ctrl Pts',(137.600694225109,1.16012349701482,125.109964875215));
#223705=CARTESIAN_POINT('Ctrl Pts',(137.322246601295,-4.16378132397874,
126.750355871033));
#223706=CARTESIAN_POINT('Ctrl Pts',(137.043798977483,-5.66137452026194,
132.116179179772));
#223707=CARTESIAN_POINT('Ctrl Pts',(136.765351353669,-1.95644110594549,
136.276505315742));
#223708=CARTESIAN_POINT('Ctrl Pts',(136.486903729857,3.54636610727348,135.408197803219));
#223709=CARTESIAN_POINT('Ctrl Pts',(136.208456106044,5.79023611752392,130.309188827029));
#223710=CARTESIAN_POINT('Ctrl Pts',(135.930008482231,2.71316200452982,125.665218535856));
#223711=CARTESIAN_POINT('Ctrl Pts',(135.651560858418,-2.85717544529452,
125.743868756725));
#223712=CARTESIAN_POINT('Ctrl Pts',(135.373113234605,-5.80190824167357,
130.472863778936));
#223713=CARTESIAN_POINT('Ctrl Pts',(135.094665610792,-3.41497080292952,
135.506488201326));
#223714=CARTESIAN_POINT('Ctrl Pts',(134.816217986979,2.11015797310843,136.219087085943));
#223715=CARTESIAN_POINT('Ctrl Pts',(134.537770363167,5.69615465880763,131.955816870215));
#223716=CARTESIAN_POINT('Ctrl Pts',(134.259322739353,4.04766348568775,126.634414610068));
#223717=CARTESIAN_POINT('Ctrl Pts',(133.980875115541,-1.32043269142476,
125.144989017623));
#223718=CARTESIAN_POINT('Ctrl Pts',(133.702427491728,-5.47511573184112,
128.856249449853));
#223719=CARTESIAN_POINT('Ctrl Pts',(133.423979867915,-4.59843488896879,
134.357728874689));
#223720=CARTESIAN_POINT('Ctrl Pts',(133.145532244102,0.503982970832797,
136.59383646292));
#223721=CARTESIAN_POINT('Ctrl Pts',(132.867084620289,5.14326510137581,133.509698580887));
#223722=CARTESIAN_POINT('Ctrl Pts',(132.588636996476,5.05613786622328,127.93948727367));
#223723=CARTESIAN_POINT('Ctrl Pts',(132.310189372663,0.322666938078297,
125.001954612649));
#223724=CARTESIAN_POINT('Ctrl Pts',(132.03174174885,-4.70731914300451,127.396549606854));
#223725=CARTESIAN_POINT('Ctrl Pts',(131.753294125038,-5.41150889699075,
132.92275643908));
#223726=CARTESIAN_POINT('Ctrl Pts',(131.474846501225,-1.14278634154918,
136.502261000723));
#223727=CARTESIAN_POINT('Ctrl Pts',(131.196398877412,4.17610103355955,134.845673468154));
#223728=CARTESIAN_POINT('Ctrl Pts',(130.917951253599,5.65735557270449,129.475316855001));
#223729=CARTESIAN_POINT('Ctrl Pts',(130.639503629786,1.93977671771839,125.326286532249));
#223730=CARTESIAN_POINT('Ctrl Pts',(130.361056005973,-3.56036217749005,
126.211338675105));
#223731=CARTESIAN_POINT('Ctrl Pts',(130.08260838216,-5.788702164947,131.317153601487));
#223732=CARTESIAN_POINT('Ctrl Pts',(129.804160758347,-2.69750765663984,
135.951736826975));
#223733=CARTESIAN_POINT('Ctrl Pts',(129.525713134534,2.87256460754407,135.856132779323));
#223734=CARTESIAN_POINT('Ctrl Pts',(129.247265510721,5.80289032997773,131.118196907806));
#223735=CARTESIAN_POINT('Ctrl Pts',(128.968817886909,3.40064332611445,126.091860817314));
#223736=CARTESIAN_POINT('Ctrl Pts',(128.690370263096,-2.12662876378584,
125.396081824838));
#223737=CARTESIAN_POINT('Ctrl Pts',(128.411922639283,-5.69963291135762,
129.670246833772));
#223738=CARTESIAN_POINT('Ctrl Pts',(128.13347501547,-4.03495285593914,134.986607005474));
#223739=CARTESIAN_POINT('Ctrl Pts',(127.855027391657,1.33765175568188,136.459687060782));
#223740=CARTESIAN_POINT('Ctrl Pts',(127.576579767844,5.48101975175251,132.73579839283));
#223741=CARTESIAN_POINT('Ctrl Pts',(127.298132144031,4.5875983586632,127.237012765392));
#223742=CARTESIAN_POINT('Ctrl Pts',(127.019684520218,-0.521601809398458,
125.016445539469));
#223743=CARTESIAN_POINT('Ctrl Pts',(126.741236896406,-5.15147539628782,
128.114689514947));
#223744=CARTESIAN_POINT('Ctrl Pts',(126.462789272592,-5.0473947575527,133.684609835992));
#223745=CARTESIAN_POINT('Ctrl Pts',(126.18434164878,-0.305004915568794,
136.607721833301));
#223746=CARTESIAN_POINT('Ctrl Pts',(125.905894024967,4.71766954350447,134.197828383304));
#223747=CARTESIAN_POINT('Ctrl Pts',(125.627446401154,5.40503616306688,128.669503836711));
#223748=CARTESIAN_POINT('Ctrl Pts',(125.348998777341,1.12543859946687,125.10300837817));
#223749=CARTESIAN_POINT('Ctrl Pts',(125.070551153528,-4.18838205631096,
126.775777101093));
#223750=CARTESIAN_POINT('Ctrl Pts',(124.792103529715,-5.65328421617778,
132.150617268407));
#223751=CARTESIAN_POINT('Ctrl Pts',(124.513655905902,-1.9230943596648,136.288313341892));
#223752=CARTESIAN_POINT('Ctrl Pts',(124.23520828209,3.57432526499779,135.386524767704));
#223753=CARTESIAN_POINT('Ctrl Pts',(123.956760658277,5.78711458662396,130.273951190703));
#223754=CARTESIAN_POINT('Ctrl Pts',(123.678313034464,2.68182831940755,125.648797965047));
#223755=CARTESIAN_POINT('Ctrl Pts',(123.399865410651,-2.88792715874745,
125.761354953818));
#223756=CARTESIAN_POINT('Ctrl Pts',(123.121417786838,-5.8038186610986,130.50818778305));
#223757=CARTESIAN_POINT('Ctrl Pts',(122.842970163025,-3.38628434620416,
135.527188978355));
#223758=CARTESIAN_POINT('Ctrl Pts',(122.564522539212,2.1430798536649,136.206141633086));
#223759=CARTESIAN_POINT('Ctrl Pts',(122.286074915399,5.703058363287,131.921121426228));
#223760=CARTESIAN_POINT('Ctrl Pts',(122.007627291586,4.02220484693838,126.609852593007));
#223761=CARTESIAN_POINT('Ctrl Pts',(121.729179667773,-1.35485842811595,
125.153131721247));
#223762=CARTESIAN_POINT('Ctrl Pts',(121.450732043961,-5.48687299624567,
128.889614127324));
#223763=CARTESIAN_POINT('Ctrl Pts',(121.172284420148,-4.57671932947311,
134.385655017367));
#223764=CARTESIAN_POINT('Ctrl Pts',(120.893836796335,0.539215815916097,
136.59066130995));
#223765=CARTESIAN_POINT('Ctrl Pts',(120.615389172522,5.15963796863542,133.478339942736));
#223766=CARTESIAN_POINT('Ctrl Pts',(120.336941548709,5.0386048905067,127.908762206842));
#223767=CARTESIAN_POINT('Ctrl Pts',(120.058493924896,0.287340067535411,
125.000097952557));
#223768=CARTESIAN_POINT('Ctrl Pts',(119.780046301083,-4.72797624015824,
127.42526753342));
#223769=CARTESIAN_POINT('Ctrl Pts',(119.50159867727,-5.39851335762638,132.955658580739));
#223770=CARTESIAN_POINT('Ctrl Pts',(119.223151053457,-1.10808043147514,
136.509111896649));
#223771=CARTESIAN_POINT('Ctrl Pts',(118.944703429644,4.20062427846316,134.820177479675));
#223772=CARTESIAN_POINT('Ctrl Pts',(118.666255805832,5.64916048839838,129.440903549983));
#223773=CARTESIAN_POINT('Ctrl Pts',(118.387808182019,1.90639418632776,125.314580056818));
#223774=CARTESIAN_POINT('Ctrl Pts',(118.109360558206,-3.58825524044456,
126.23309670829));
#223775=CARTESIAN_POINT('Ctrl Pts',(117.830912934393,-5.785473397262,131.352381573729));
#223776=CARTESIAN_POINT('Ctrl Pts',(117.55246531058,-2.66612413808396,135.968061952766));
#223777=CARTESIAN_POINT('Ctrl Pts',(117.274017686767,2.9032629565882,135.838553065588));
#223778=CARTESIAN_POINT('Ctrl Pts',(116.995570062954,5.80469322643624,131.082867252651));
#223779=CARTESIAN_POINT('Ctrl Pts',(116.717122439142,3.37189399621826,126.071247447876));
#223780=CARTESIAN_POINT('Ctrl Pts',(116.438674815328,-2.15951109034483,
125.409127420613));
#223781=CARTESIAN_POINT('Ctrl Pts',(116.160227191516,-5.70643098286277,
129.704963129555));
#223782=CARTESIAN_POINT('Ctrl Pts',(115.881779567703,-4.00941957678149,
135.011091421425));
#223783=CARTESIAN_POINT('Ctrl Pts',(115.60333194389,1.37205254932662,136.451439614773));
#223784=CARTESIAN_POINT('Ctrl Pts',(115.324884320077,5.49267541109693,132.702398084833));
#223785=CARTESIAN_POINT('Ctrl Pts',(115.046436696264,4.56579790218037,127.20915284676));
#223786=CARTESIAN_POINT('Ctrl Pts',(114.767989072451,-0.556824827212187,
125.019727914392));
#223787=CARTESIAN_POINT('Ctrl Pts',(114.489541448638,-5.1677527428018,128.146097841224));
#223788=CARTESIAN_POINT('Ctrl Pts',(114.211093824825,-5.02976834651319,
133.715281396157));
#223789=CARTESIAN_POINT('Ctrl Pts',(113.932646201012,-0.269672557622912,
136.60947096195));
#223790=CARTESIAN_POINT('Ctrl Pts',(113.6541985772,4.73823913748602,134.169047716661));
#223791=CARTESIAN_POINT('Ctrl Pts',(113.375750953387,5.39194054109557,128.636641401405));
#223792=CARTESIAN_POINT('Ctrl Pts',(113.097303329574,1.09071199837779,125.09626314683));
#223793=CARTESIAN_POINT('Ctrl Pts',(112.818855705761,-4.21282758660586,
126.801347611796));
#223794=CARTESIAN_POINT('Ctrl Pts',(112.540408081948,-5.64498442756793,
132.185005471008));
#223795=CARTESIAN_POINT('Ctrl Pts',(112.261960458135,-1.8896763524154,136.299918158156));
#223796=CARTESIAN_POINT('Ctrl Pts',(111.983512834322,3.60215197478495,135.364681938413));
#223797=CARTESIAN_POINT('Ctrl Pts',(111.705065210509,5.78377861206482,130.238733208892));
#223798=CARTESIAN_POINT('Ctrl Pts',(111.426617586696,2.65039525815055,125.632568435507));
#223799=CARTESIAN_POINT('Ctrl Pts',(111.148169962883,-2.91857185899754,
125.77902802134));
#223800=CARTESIAN_POINT('Ctrl Pts',(110.869722339071,-5.80551401788879,
130.543522761958));
#223801=CARTESIAN_POINT('Ctrl Pts',(110.591274715258,-3.35747240946702,
135.547714749242));
#223802=CARTESIAN_POINT('Ctrl Pts',(110.312827091445,2.17592232160915,136.192996015246));
#223803=CARTESIAN_POINT('Ctrl Pts',(110.034379467632,5.70975073884148,131.886384600257));
#223804=CARTESIAN_POINT('Ctrl Pts',(109.755931843819,3.99659716390926,126.585446004984));
#223805=CARTESIAN_POINT('Ctrl Pts',(109.477484220006,-1.38923396002991,
125.161483833236));
#223806=CARTESIAN_POINT('Ctrl Pts',(109.199036596193,-5.49842694255352,
128.923049756431));
#223807=CARTESIAN_POINT('Ctrl Pts',(108.92058897238,-4.55483417795961,134.413448453863));
#223808=CARTESIAN_POINT('Ctrl Pts',(108.642141348568,0.57442868015902,136.58727174348));
#223809=CARTESIAN_POINT('Ctrl Pts',(108.363693724754,5.17581964361271,133.446882219296));
#223810=CARTESIAN_POINT('Ctrl Pts',(108.085246100942,5.02088520743284,127.878144437479));
#223811=CARTESIAN_POINT('Ctrl Pts',(107.806798477129,0.252002549500665,
124.998456371553));
#223812=CARTESIAN_POINT('Ctrl Pts',(107.528350853316,-4.74845814041369,
127.454110673523));
#223813=CARTESIAN_POINT('Ctrl Pts',(107.249903229503,-5.38531777436419,
132.988481005259));
#223814=CARTESIAN_POINT('Ctrl Pts',(106.97145560569,-1.07333346107335,136.515751400918));
#223815=CARTESIAN_POINT('Ctrl Pts',(106.693007981877,4.22499186768932,134.794532683627));
#223816=CARTESIAN_POINT('Ctrl Pts',(106.414560358064,5.64075607237289,129.406540768369));
#223817=CARTESIAN_POINT('Ctrl Pts',(106.136112734251,1.87294101279944,125.303077007226));
#223818=CARTESIAN_POINT('Ctrl Pts',(105.857665110439,-3.61601533928142,
126.25502413134));
#223819=CARTESIAN_POINT('Ctrl Pts',(105.579217486626,-5.78203024673271,
131.387589238853));
#223820=CARTESIAN_POINT('Ctrl Pts',(105.300769862813,-2.63464182531766,
135.984195735705));
#223821=CARTESIAN_POINT('Ctrl Pts',(105.022322239,2.93385372415587,135.820786808));
#223822=CARTESIAN_POINT('Ctrl Pts',(104.743874615187,5.80628102785255,131.047527277329));
#223823=CARTESIAN_POINT('Ctrl Pts',(104.465426991374,3.34301971955009,126.050809465687));
#223824=CARTESIAN_POINT('Ctrl Pts',(104.186979367561,-2.19231339542621,
125.422372938737));
#223825=CARTESIAN_POINT('Ctrl Pts',(103.908531743748,-5.71301760046937,
129.739720163916));
#223826=CARTESIAN_POINT('Ctrl Pts',(103.630084119935,-3.98373772710686,
135.03541995542));
#223827=CARTESIAN_POINT('Ctrl Pts',(103.351636496123,1.40640250105958,136.442982914176));
#223828=CARTESIAN_POINT('Ctrl Pts',(103.07318887231,5.50412753733405,132.66892744436));
#223829=CARTESIAN_POINT('Ctrl Pts',(102.794741248497,4.54382825837723,127.181426149873));
#223830=CARTESIAN_POINT('Ctrl Pts',(102.516293624684,-0.592027211677165,
125.023224641008));
#223831=CARTESIAN_POINT('Ctrl Pts',(102.237846000871,-5.18383859633749,
128.177604670405));
#223832=CARTESIAN_POINT('Ctrl Pts',(101.959398377058,-5.01195555555783,
133.745845091081));
#223833=CARTESIAN_POINT('Ctrl Pts',(101.680950753245,-0.234330206861215,
136.611004980102));
#223834=CARTESIAN_POINT('Ctrl Pts',(101.402503129432,4.75863315427373,134.140142370299));
#223835=CARTESIAN_POINT('Ctrl Pts',(101.124055505619,5.37864511878468,128.603859291732));
#223836=CARTESIAN_POINT('Ctrl Pts',(100.845607881807,1.05594498055446,125.089729431141));
#223837=CARTESIAN_POINT('Ctrl Pts',(100.567160257994,-4.23711700902531,
126.827066455619));
#223838=CARTESIAN_POINT('Ctrl Pts',(100.288712634181,-5.63647546198416,
132.219342513305));
#223839=CARTESIAN_POINT('Ctrl Pts',(100.010265010368,-1.85618832251382,
136.311319334515));
#223840=CARTESIAN_POINT('Ctrl Pts',(99.731817386555,3.62984520550588,135.342670124737));
#223841=CARTESIAN_POINT('Ctrl Pts',(99.4533697627421,5.78022831746224,130.203536186614));
#223842=CARTESIAN_POINT('Ctrl Pts',(99.1749221389292,2.61886398552269,125.616530548629));
#223843=CARTESIAN_POINT('Ctrl Pts',(98.8964745151164,-2.9491084104941,125.796887304409));
#223844=CARTESIAN_POINT('Ctrl Pts',(98.6180268913035,-5.80699424922206,
130.578867406308));
#223845=CARTESIAN_POINT('Ctrl Pts',(98.3395792674906,-3.32853606035512,
135.568064753397));
#223846=CARTESIAN_POINT('Ctrl Pts',(98.0611316436778,2.20868415995158,136.179650719541));
#223847=CARTESIAN_POINT('Ctrl Pts',(97.7826840198649,5.71623153748262,131.851607679491));
#223848=CARTESIAN_POINT('Ctrl Pts',(97.5042363960519,3.97084138550236,126.561195750394));
#223849=CARTESIAN_POINT('Ctrl Pts',(97.2257887722391,-1.42355801336861,
125.170045044101));
#223850=CARTESIAN_POINT('Ctrl Pts',(96.9473411484261,-5.50977714262889,
128.956555098203));
#223851=CARTESIAN_POINT('Ctrl Pts',(96.6688935246133,-4.53278024539068,
134.441108154283));
#223852=CARTESIAN_POINT('Ctrl Pts',(96.3904459008004,0.609620258735999,
136.583667889112));
#223853=CARTESIAN_POINT('Ctrl Pts',(96.1119982769875,5.19180952668969,133.415326576248));
#223854=CARTESIAN_POINT('Ctrl Pts',(95.8335506531746,5.00297947361121,127.847635100131));
#223855=CARTESIAN_POINT('Ctrl Pts',(95.5551030293618,0.216655693418756,
124.997029930466));
#223856=CARTESIAN_POINT('Ctrl Pts',(95.2766554055487,-4.7687640848064,127.483077958369));
#223857=CARTESIAN_POINT('Ctrl Pts',(94.9982077817361,-5.37192263617151,
133.021222496396));
#223858=CARTESIAN_POINT('Ctrl Pts',(94.7197601579228,-1.03854671790542,
136.522179267501));
#223859=CARTESIAN_POINT('Ctrl Pts',(94.4413125341102,4.24920289828813,134.768740030285));
#223860=CARTESIAN_POINT('Ctrl Pts',(94.1628649102971,5.63214263605674,129.372229783482));
#223861=CARTESIAN_POINT('Ctrl Pts',(93.8844172864844,1.83941843675322,125.29177780972));
#223862=CARTESIAN_POINT('Ctrl Pts',(93.6059696626714,-3.6436414453401,126.277120131727));
#223863=CARTESIAN_POINT('Ctrl Pts',(93.3275220388585,-5.77837284094635,
131.422775292226));
#223864=CARTESIAN_POINT('Ctrl Pts',(93.0490744150458,-2.60306188492951,
136.000137577949));
#223865=CARTESIAN_POINT('Ctrl Pts',(92.7706267912327,2.96433577669487,135.802834664895));
#223866=CARTESIAN_POINT('Ctrl Pts',(92.49217916742,5.80765367539012,131.012178291378));
#223867=CARTESIAN_POINT('Ctrl Pts',(92.213731543607,3.31402156605677,126.030547628085));
#223868=CARTESIAN_POINT('Ctrl Pts',(91.9352839197941,-2.22503446352861,
125.435817888395));
#223869=CARTESIAN_POINT('Ctrl Pts',(91.6568362959812,-5.71939252010779,
129.77451664892));
#223870=CARTESIAN_POINT('Ctrl Pts',(91.3783886721684,-3.95790825856573,
135.059591705955));
#223871=CARTESIAN_POINT('Ctrl Pts',(91.0999410483554,1.44070033803066,136.434317272356));
#223872=CARTESIAN_POINT('Ctrl Pts',(90.8214934245425,5.51537570610103,132.635387711677));
#223873=CARTESIAN_POINT('Ctrl Pts',(90.5430458007297,4.52169024134706,127.153833702157));
#223874=CARTESIAN_POINT('Ctrl Pts',(90.2645981769166,-0.627207658356129,
125.026935589742));
#223875=CARTESIAN_POINT('Ctrl Pts',(89.9861505531037,-5.19973236082766,
128.209208834995));
#223876=CARTESIAN_POINT('Ctrl Pts',(89.707702929291,-4.99395704474619,133.776299788217));
#223877=CARTESIAN_POINT('Ctrl Pts',(89.4292553054779,-0.198979172907652,
136.61232383091));
#223878=CARTESIAN_POINT('Ctrl Pts',(89.1508076816652,4.77885083815996,134.111113415317));
#223879=CARTESIAN_POINT('Ctrl Pts',(88.8723600578521,5.36515038880097,128.571158722445));
#223880=CARTESIAN_POINT('Ctrl Pts',(88.5939124340396,1.02113883430145,125.08340747321));
#223881=CARTESIAN_POINT('Ctrl Pts',(88.3154648102263,-4.26124942351577,
126.85293267954));
#223882=CARTESIAN_POINT('Ctrl Pts',(88.0370171864138,-5.62775763472933,
132.253627122929));
#223883=CARTESIAN_POINT('Ctrl Pts',(87.7585695626006,-1.82263151087143,
136.322516448493));
#223884=CARTESIAN_POINT('Ctrl Pts',(87.480121938788,3.65740393097785,135.320490142334));
#223885=CARTESIAN_POINT('Ctrl Pts',(87.2016743149749,5.77646383437373,130.168361428106));
#223886=CARTESIAN_POINT('Ctrl Pts',(86.9232266911622,2.58723566992664,125.600684898703));
#223887=CARTESIAN_POINT('Ctrl Pts',(86.6447790673492,-2.97953568169397,
125.814932141244));
#223888=CARTESIAN_POINT('Ctrl Pts',(86.3663314435363,-5.80825930024783,
130.614220406392));
#223889=CARTESIAN_POINT('Ctrl Pts',(86.0878838197235,-3.29947637111547,
135.588238236744));
#223890=CARTESIAN_POINT('Ctrl Pts',(85.8094361959104,2.24136415469026,136.166106240484));
#223891=CARTESIAN_POINT('Ctrl Pts',(85.5309885720977,5.72250051906197,131.816791952599));
#223892=CARTESIAN_POINT('Ctrl Pts',(85.2525409482847,3.94493846610766,126.537102727838));
#223893=CARTESIAN_POINT('Ctrl Pts',(84.9740933244718,-1.45782931624159,
125.178815036599));
#223894=CARTESIAN_POINT('Ctrl Pts',(84.6956457006588,-5.52092317588609,
128.990128911089));
#223895=CARTESIAN_POINT('Ctrl Pts',(84.417198076846,-4.51055834898274,134.468633093685));
#223896=CARTESIAN_POINT('Ctrl Pts',(84.138750453033,0.644789247610192,136.579849880389));
#223897=CARTESIAN_POINT('Ctrl Pts',(83.8603028292202,5.20760702535536,133.383674182895));
#223898=CARTESIAN_POINT('Ctrl Pts',(83.5818552054073,4.98488835254533,127.817235325336));
#223899=CARTESIAN_POINT('Ctrl Pts',(83.3034075815944,0.181300809080568,
124.995818682153));
#223900=CARTESIAN_POINT('Ctrl Pts',(83.0249599577814,-4.78889332089225,
127.512168314565));
#223901=CARTESIAN_POINT('Ctrl Pts',(82.7465123339688,-5.35832843941005,
133.053881840899));
#223902=CARTESIAN_POINT('Ctrl Pts',(82.4680647101557,-1.00372149100682,
136.528395258211));
#223903=CARTESIAN_POINT('Ctrl Pts',(82.1896170863428,4.27325647311088,134.742800475408));
#223904=CARTESIAN_POINT('Ctrl Pts',(81.91116946253,5.62332049862395,129.337971866731));
#223905=CARTESIAN_POINT('Ctrl Pts',(81.632721838717,1.80582770038043,125.280682882997));
#223906=CARTESIAN_POINT('Ctrl Pts',(81.3542742149043,-3.67113253492515,
126.299383890674));
#223907=CARTESIAN_POINT('Ctrl Pts',(81.0758265910913,-5.77450131542928,
131.457938430015));
#223908=CARTESIAN_POINT('Ctrl Pts',(80.7973789672785,-2.57138548712596,
136.015886888767));
#223909=CARTESIAN_POINT('Ctrl Pts',(80.5189313434656,2.99470798468153,135.784697301496));
#223910=CARTESIAN_POINT('Ctrl Pts',(80.2404837196526,5.80881111818491,130.976821604667));
#223911=CARTESIAN_POINT('Ctrl Pts',(79.9620360958398,3.2849006102757,126.010462685879));
#223912=CARTESIAN_POINT('Ctrl Pts',(79.6835884720269,-2.25767308216064,
125.449461771377));
#223913=CARTESIAN_POINT('Ctrl Pts',(79.4051408482139,-5.72555550555307,
129.809351295171));
#223914=CARTESIAN_POINT('Ctrl Pts',(79.1266932244012,-3.93193212827854,
135.083605777338));
#223915=CARTESIAN_POINT('Ctrl Pts',(78.8482456005881,1.47494478932078,136.425443010422));
#223916=CARTESIAN_POINT('Ctrl Pts',(78.5697979767754,5.526419500593,132.601780129612));
#223917=CARTESIAN_POINT('Ctrl Pts',(78.2913503529625,4.49938467142216,127.126376526057));
#223918=CARTESIAN_POINT('Ctrl Pts',(78.0129027291494,-0.662364863624755,
125.030860623086));
#223919=CARTESIAN_POINT('Ctrl Pts',(77.7344551053368,-5.21543344732299,
128.240909163888));
#223920=CARTESIAN_POINT('Ctrl Pts',(77.4560074815235,-4.97577348101974,
133.806644359053));
#223921=CARTESIAN_POINT('Ctrl Pts',(77.1775598577108,-0.163620765707691,
136.613427465507));
#223922=CARTESIAN_POINT('Ctrl Pts',(76.8991122338979,4.79889143997102,134.081961927395));
#223923=CARTESIAN_POINT('Ctrl Pts',(76.620664610085,5.35145685119646,128.538540905275));
#223924=CARTESIAN_POINT('Ctrl Pts',(76.3422169862721,0.986294849373407,
125.077297507303));
#223925=CARTESIAN_POINT('Ctrl Pts',(76.0637693624593,-4.28522393584178,
126.878945325076));
#223926=CARTESIAN_POINT('Ctrl Pts',(75.7853217386464,-5.61883126884571,
132.287858029448));
#223927=CARTESIAN_POINT('Ctrl Pts',(75.5068741148335,-1.78900716094817,
136.333509085178));
#223928=CARTESIAN_POINT('Ctrl Pts',(75.2284264910206,3.68482713000219,135.298142813091));
#223929=CARTESIAN_POINT('Ctrl Pts',(74.9499788672077,5.77248530229349,130.133210236781));
#223930=CARTESIAN_POINT('Ctrl Pts',(74.6715312433948,2.55551148336137,125.585032072894));
#223931=CARTESIAN_POINT('Ctrl Pts',(74.3930836195819,-3.0098525451033,125.833161863185));
#223932=CARTESIAN_POINT('Ctrl Pts',(74.1146359957691,-5.80930912408932,
130.649580452192));
#223933=CARTESIAN_POINT('Ctrl Pts',(73.8361883719562,-3.27029441856551,
135.608234451746));
#223934=CARTESIAN_POINT('Ctrl Pts',(73.5577407481433,2.273961094856,136.152363079971));
#223935=CARTESIAN_POINT('Ctrl Pts',(73.2792931243304,5.72855745128013,131.781938709691));
#223936=CARTESIAN_POINT('Ctrl Pts',(73.0008455005175,3.91888936556733,126.513167830092));
#223937=CARTESIAN_POINT('Ctrl Pts',(72.7223978767045,-1.49204659871303,
125.187793485758));
#223938=CARTESIAN_POINT('Ctrl Pts',(72.4439502528918,-5.53186462930466,
129.023769950998));
#223939=CARTESIAN_POINT('Ctrl Pts',(72.1655026290786,-4.48816931217651,
134.496022252122));
#223940=CARTESIAN_POINT('Ctrl Pts',(71.8870550052659,0.679934343581693,
136.575817858786));
#223941=CARTESIAN_POINT('Ctrl Pts',(71.6086073814528,5.22321155422762,133.351926212129));
#223942=CARTESIAN_POINT('Ctrl Pts',(71.3301597576401,4.96661251460835,127.786946239566));
#223943=CARTESIAN_POINT('Ctrl Pts',(71.0517121338272,0.145939206574258,
124.994822671498));
#223944=CARTESIAN_POINT('Ctrl Pts',(70.7732645100143,-4.80884510277506,
127.541380664158));
#223945=CARTESIAN_POINT('Ctrl Pts',(70.4948168862015,-5.34453568781766,
133.086457828568));
#223946=CARTESIAN_POINT('Ctrl Pts',(70.2163692623885,-0.968859070839113,
136.534399142713));
#223947=CARTESIAN_POINT('Ctrl Pts',(69.9379216385757,4.29715170084345,134.716714980192));
#223948=CARTESIAN_POINT('Ctrl Pts',(69.6594740147628,5.61428998698222,129.303768287553));
#223949=CARTESIAN_POINT('Ctrl Pts',(69.3810263909498,1.77217004839796,125.269792638185));
#223950=CARTESIAN_POINT('Ctrl Pts',(69.102578767137,-3.69848758934425,126.321814583191));
#223951=CARTESIAN_POINT('Ctrl Pts',(68.8241311433241,-5.77041581364239,
131.493077349239));
#223952=CARTESIAN_POINT('Ctrl Pts',(68.5456835195112,-2.53961380568736,
136.031443084562));
#223953=CARTESIAN_POINT('Ctrl Pts',(68.2672358956983,3.02496922266262,135.76637538989));
#223954=CARTESIAN_POINT('Ctrl Pts',(67.9887882718854,5.80975331334755,130.94145852735));
#223955=CARTESIAN_POINT('Ctrl Pts',(67.7103406480725,3.25565793129432,125.990555383323));
#223956=CARTESIAN_POINT('Ctrl Pts',(67.4318930242597,-2.29022804188655,
125.463304082106));
#223957=CARTESIAN_POINT('Ctrl Pts',(67.1534454004468,-5.73150632843341,
129.844222811859));
#223958=CARTESIAN_POINT('Ctrl Pts',(66.8749977766338,-3.90581029880048,
135.107461279717));
#223959=CARTESIAN_POINT('Ctrl Pts',(66.5965501528209,1.50913458598933,136.416360457212));
#223960=CARTESIAN_POINT('Ctrl Pts',(66.3181025290079,5.53725851157817,132.568105943505));
#223961=CARTESIAN_POINT('Ctrl Pts',(66.0396549051952,4.47691237514338,127.09905563901));
#223962=CARTESIAN_POINT('Ctrl Pts',(65.7612072813823,-0.69749752471975,
125.034999595595));
#223963=CARTESIAN_POINT('Ctrl Pts',(65.4827596575694,-5.23094127401388,
128.272704482416));
#223964=CARTESIAN_POINT('Ctrl Pts',(65.2043120337565,-4.95740553817722,
133.836877679162));
#223965=CARTESIAN_POINT('Ctrl Pts',(64.9258644099437,-0.128256295479839,
136.614315842995));
#223966=CARTESIAN_POINT('Ctrl Pts',(64.6474167861306,4.81875421709505,134.05268898675));
#223967=CARTESIAN_POINT('Ctrl Pts',(64.3689691623179,5.33756501339024,128.506007048888));
#223968=CARTESIAN_POINT('Ctrl Pts',(64.0905215385049,0.951414316927145,
125.071399759827));
#223969=CARTESIAN_POINT('Ctrl Pts',(63.8120739146922,-4.30903965761881,
126.905103428319));
#223970=CARTESIAN_POINT('Ctrl Pts',(63.5336262908791,-5.60969669510319,
132.322033964426));
#223971=CARTESIAN_POINT('Ctrl Pts',(63.2551786670663,-1.75531651870651,
136.344296837232));
#223972=CARTESIAN_POINT('Ctrl Pts',(62.9767310432534,3.71211378640213,135.275628965096));
#223973=CARTESIAN_POINT('Ctrl Pts',(62.6982834194405,5.76829286864752,130.098083915181));
#223974=CARTESIAN_POINT('Ctrl Pts',(62.4198357956276,2.52369260137852,125.569572651222));
#223975=CARTESIAN_POINT('Ctrl Pts',(62.1413881718147,-3.04005787731984,
125.851575794724));
#223976=CARTESIAN_POINT('Ctrl Pts',(61.8629405480017,-5.81014368184488,
130.684946233427));
#223977=CARTESIAN_POINT('Ctrl Pts',(61.5844929241889,-3.24099128405306,
135.628052657436));
#223978=CARTESIAN_POINT('Ctrl Pts',(61.3060453003759,2.306473772557,136.138421747261));
#223979=CARTESIAN_POINT('Ctrl Pts',(61.0275976765631,5.73440210969521,131.747049242268));
#223980=CARTESIAN_POINT('Ctrl Pts',(60.7491500527502,3.89269504914048,126.489391944074));
#223981=CARTESIAN_POINT('Ctrl Pts',(60.4707024289374,-1.5262085928491,125.196980058879));
#223982=CARTESIAN_POINT('Ctrl Pts',(60.1922548051244,-5.54260109744501,
129.057476971348));
#223983=CARTESIAN_POINT('Ctrl Pts',(59.9138071813117,-4.46561396460588,
134.52327461468));
#223984=CARTESIAN_POINT('Ctrl Pts',(59.6353595574987,0.715054244335847,
136.571571973714));
#223985=CARTESIAN_POINT('Ctrl Pts',(59.3569119336859,5.23862253507484,133.320083840384));
#223986=CARTESIAN_POINT('Ctrl Pts',(59.0784643098728,4.94815263701827,127.756768965196));
#223987=CARTESIAN_POINT('Ctrl Pts',(58.80001668606,0.110572196236736,124.994041935407));
#223988=CARTESIAN_POINT('Ctrl Pts',(58.5215690622471,-4.82861869113419,
127.570713924673));
#223989=CARTESIAN_POINT('Ctrl Pts',(58.2431214384343,-5.3305448924898,133.118949252284));
#223990=CARTESIAN_POINT('Ctrl Pts',(57.9646738146213,-0.933960749242644,
136.54019069853));
#223991=CARTESIAN_POINT('Ctrl Pts',(57.6862261908085,4.32088769603949,134.690484511247));
#223992=CARTESIAN_POINT('Ctrl Pts',(57.4077785669955,5.6050514357603,129.269620313377));
#223993=CARTESIAN_POINT('Ctrl Pts',(57.1293309431827,1.73844672800264,125.259107478825));
#223994=CARTESIAN_POINT('Ctrl Pts',(56.8508833193697,-3.72570559494523,
126.3444113781));
#223995=CARTESIAN_POINT('Ctrl Pts',(56.5724356955568,-5.76611648697549,
131.528190747811));
#223996=CARTESIAN_POINT('Ctrl Pts',(56.293988071744,-2.50774801792579,136.046805588895));
#223997=CARTESIAN_POINT('Ctrl Pts',(56.0155404479311,3.05511836929639,135.747869609001));
#223998=CARTESIAN_POINT('Ctrl Pts',(55.7370928241181,5.81048022596477,130.906090369819));
#223999=CARTESIAN_POINT('Ctrl Pts',(55.4586452003054,3.22629461271119,125.97082645809));
#224000=CARTESIAN_POINT('Ctrl Pts',(55.1801975764924,-2.32269813636975,
125.477344307648));
#224001=CARTESIAN_POINT('Ctrl Pts',(54.9017499526795,-5.73724476823917,
129.879129906805));
#224002=CARTESIAN_POINT('Ctrl Pts',(54.6233023288666,-3.87954373808533,
135.131157329118));
#224003=CARTESIAN_POINT('Ctrl Pts',(54.3448547050537,1.54326846112093,136.407069949284));
#224004=CARTESIAN_POINT('Ctrl Pts',(54.0664070812409,5.54789233741261,132.534366401168));
#224005=CARTESIAN_POINT('Ctrl Pts',(53.7879594574279,4.45427418523046,127.071872053402));
#224006=CARTESIAN_POINT('Ctrl Pts',(53.5095118336151,-0.732604339787292,
125.039352353899));
#224007=CARTESIAN_POINT('Ctrl Pts',(53.2310642098022,-5.24625526625226,
128.304593612394));
#224008=CARTESIAN_POINT('Ctrl Pts',(52.9526165859893,-4.93885389684926,
133.866998628235));
#224009=CARTESIAN_POINT('Ctrl Pts',(52.6741689621764,-0.0928870726681018,
136.614988930455));
#224010=CARTESIAN_POINT('Ctrl Pts',(52.3957213383635,4.83843843350925,134.023295678104));
#224011=CARTESIAN_POINT('Ctrl Pts',(52.1172737145507,5.32347539014984,128.473558358838));
#224012=CARTESIAN_POINT('Ctrl Pts',(51.8388260907377,0.91649852947334,125.065714449322));
#224013=CARTESIAN_POINT('Ctrl Pts',(51.5603784669247,-4.33269570634681,
126.931406019971));
#224014=CARTESIAN_POINT('Ctrl Pts',(51.2819308431118,-5.6003542519866,132.356153661459));
#224015=CARTESIAN_POINT('Ctrl Pts',(51.0034832192991,-1.72156083256576,
136.354879304913));
#224016=CARTESIAN_POINT('Ctrl Pts',(50.7250355954861,3.73926288906064,135.252949432607));
#224017=CARTESIAN_POINT('Ctrl Pts',(50.4465879716733,5.76388668878802,130.062983764924));
#224018=CARTESIAN_POINT('Ctrl Pts',(50.1681403478604,2.49178020303801,125.554307206545));
#224019=CARTESIAN_POINT('Ctrl Pts',(49.8896927240475,-3.07015055907373,
125.870173253527));
#224020=CARTESIAN_POINT('Ctrl Pts',(49.6112451002346,-5.81076294258959,
130.720316439607));
#224021=CARTESIAN_POINT('Ctrl Pts',(49.3327974764216,-3.21156805341676,
135.647692119444));
#224022=CARTESIAN_POINT('Ctrl Pts',(49.0543498526089,2.33890098302428,136.124282758954));
#224023=CARTESIAN_POINT('Ctrl Pts',(48.7759022287959,5.74003427773134,131.712124843171));
#224024=CARTESIAN_POINT('Ctrl Pts',(48.497454604983,3.86635648746696,126.465775950806));
#224025=CARTESIAN_POINT('Ctrl Pts',(48.2190069811701,-1.56031403276457,
125.206374415548));
#224026=CARTESIAN_POINT('Ctrl Pts',(47.9405593573573,-5.55313218246346,
129.091248723115));
#224027=CARTESIAN_POINT('Ctrl Pts',(47.6621117335443,-4.44289314206747,
134.550389171513));
#224028=CARTESIAN_POINT('Ctrl Pts',(47.3836641097315,0.750147648492217,
136.567112382502));
#224029=CARTESIAN_POINT('Ctrl Pts',(47.1052164859186,5.25383939683757,133.288148247589));
#224030=CARTESIAN_POINT('Ctrl Pts',(46.8267688621057,4.92950940381243,127.726704620456));
#224031=CARTESIAN_POINT('Ctrl Pts',(46.5483212382927,0.0752010886061242,
124.993476502813));
#224032=CARTESIAN_POINT('Ctrl Pts',(46.2698736144798,-4.84821335325179,
127.600167009156));
#224033=CARTESIAN_POINT('Ctrl Pts',(45.991425990667,-5.31635657186091,133.151354908068));
#224034=CARTESIAN_POINT('Ctrl Pts',(45.7129783668541,-0.899027819386881,
136.545769711054));
#224035=CARTESIAN_POINT('Ctrl Pts',(45.4345307430412,4.344463579153,134.664110040551));
#224036=CARTESIAN_POINT('Ctrl Pts',(45.1560831192283,5.5956051872961,129.235529209567));
#224037=CARTESIAN_POINT('Ctrl Pts',(44.8776354954154,1.70465898882477,125.248627800858));
#224038=CARTESIAN_POINT('Ctrl Pts',(44.5991878716026,-3.7527855431554,126.367173438067));
#224039=CARTESIAN_POINT('Ctrl Pts',(44.3207402477896,-5.76160349474165,
131.563277324591));
#224040=CARTESIAN_POINT('Ctrl Pts',(44.0422926239769,-2.47578930463884,
136.0619738325));
#224041=CARTESIAN_POINT('Ctrl Pts',(43.7638450001637,3.08515430739569,135.72918064457));
#224042=CARTESIAN_POINT('Ctrl Pts',(43.485397376351,5.8109918291003,130.870718442656));
#224043=CARTESIAN_POINT('Ctrl Pts',(43.206949752538,3.19681174259461,125.951276641244));
#224044=CARTESIAN_POINT('Ctrl Pts',(42.9285021287252,-2.3550821624196,125.491581927739));
#224045=CARTESIAN_POINT('Ctrl Pts',(42.6500545049123,-5.74277061233009,
129.914071286517));
#224046=CARTESIAN_POINT('Ctrl Pts',(42.3716068810994,-3.85313341945026,
135.154693047476));
#224047=CARTESIAN_POINT('Ctrl Pts',(42.0931592572865,1.57734514987214,136.397571830902));
#224048=CARTESIAN_POINT('Ctrl Pts',(41.8147116334736,5.5583205840564,132.50056275283));
#224049=CARTESIAN_POINT('Ctrl Pts',(41.5362640096606,4.43147094054935,127.04482677653));
#224050=CARTESIAN_POINT('Ctrl Pts',(41.2578163858478,-0.767684007931795,
125.043918736703));
#224051=CARTESIAN_POINT('Ctrl Pts',(40.9793687620349,-5.26137485657243,
128.336575372158));
#224052=CARTESIAN_POINT('Ctrl Pts',(40.700921138222,-4.9201192444739,133.897006090131));
#224053=CARTESIAN_POINT('Ctrl Pts',(40.4224735144091,-0.0575144078915333,
136.615446702946));
#224054=CARTESIAN_POINT('Ctrl Pts',(40.1440258905964,4.85794335980812,133.993783090635));
#224055=CARTESIAN_POINT('Ctrl Pts',(39.8655782667833,5.30918850357096,128.441196037522));
#224056=CARTESIAN_POINT('Ctrl Pts',(39.5871306429705,0.8815487808295,125.060241786462));
#224057=CARTESIAN_POINT('Ctrl Pts',(39.3086830191576,-4.35619120544207,
126.957852125381));
#224058=CARTESIAN_POINT('Ctrl Pts',(39.0302353953447,-5.59080428568363,
132.39021585623));
#224059=CARTESIAN_POINT('Ctrl Pts',(38.7517877715318,-1.6877413533555,136.365256096082));
#224060=CARTESIAN_POINT('Ctrl Pts',(38.4733401477189,3.76627343195761,135.230105056025));
#224061=CARTESIAN_POINT('Ctrl Pts',(38.194892523906,5.7592669259876,130.027911086658));
#224062=CARTESIAN_POINT('Ctrl Pts',(37.9164449000932,2.45977547086574,125.539236304527));
#224063=CARTESIAN_POINT('Ctrl Pts',(37.6379972762802,-3.10012947526937,
125.888953550457));
#224064=CARTESIAN_POINT('Ctrl Pts',(37.3595496524674,-5.81116688337655,
130.755689760074));
#224065=CARTESIAN_POINT('Ctrl Pts',(37.0811020286545,-3.18202581694541,
135.667152110023));
#224066=CARTESIAN_POINT('Ctrl Pts',(36.8026544048415,2.3712415246555,136.109946638975));
#224067=CARTESIAN_POINT('Ctrl Pts',(36.5242067810287,5.74545374668639,131.677166806538));
#224068=CARTESIAN_POINT('Ctrl Pts',(36.2457591572158,3.83987465653194,126.442320725389));
#224069=CARTESIAN_POINT('Ctrl Pts',(35.9673115334029,-1.59436165466975,
125.215976207654));
#224070=CARTESIAN_POINT('Ctrl Pts',(35.6888639095901,-5.56345749412674,
129.125083954872));
#224071=CARTESIAN_POINT('Ctrl Pts',(35.4104162857771,-4.42000768648982,
134.57736491788));
#224072=CARTESIAN_POINT('Ctrl Pts',(35.1319686619643,0.785213255651605,
136.562439250406));
#224073=CARTESIAN_POINT('Ctrl Pts',(34.8535210381513,5.26886157564935,133.25612061713));
#224074=CARTESIAN_POINT('Ctrl Pts',(34.5750734143385,4.91068350582282,127.69675431939));
#224075=CARTESIAN_POINT('Ctrl Pts',(34.2966257905255,0.0398271943713243,
124.993126394665));
#224076=CARTESIAN_POINT('Ctrl Pts',(34.0181781667127,-4.86762836304081,
127.629738826211));
#224077=CARTESIAN_POINT('Ctrl Pts',(33.7397305428998,-5.30197125168398,
133.183673595116));
#224078=CARTESIAN_POINT('Ctrl Pts',(33.4612829190869,-0.864061575724654,
136.551135973552));
#224079=CARTESIAN_POINT('Ctrl Pts',(33.182835295274,4.36787847657091,134.637592545421));
#224080=CARTESIAN_POINT('Ctrl Pts',(32.9043876714611,5.58595159162396,129.201496239381));
#224081=CARTESIAN_POINT('Ctrl Pts',(32.6259400476482,1.67080808288091,125.238353992614));
#224082=CARTESIAN_POINT('Ctrl Pts',(32.3474924238352,-3.77972643051725,
126.390099919638));
#224083=CARTESIAN_POINT('Ctrl Pts',(32.0690448000224,-5.75687700417149,
131.598335779433));
#224084=CARTESIAN_POINT('Ctrl Pts',(31.7905971762095,-2.44373885006871,
136.076947253315));
#224085=CARTESIAN_POINT('Ctrl Pts',(31.5121495523967,3.11507592396733,135.71030918912));
#224086=CARTESIAN_POINT('Ctrl Pts',(31.2337019285837,5.81128810379662,130.835344056578));
#224087=CARTESIAN_POINT('Ctrl Pts',(30.9552543047708,3.16721041344351,125.931906657209));
#224088=CARTESIAN_POINT('Ctrl Pts',(30.676806680958,-2.38737892003384,125.506016414799));
#224089=CARTESIAN_POINT('Ctrl Pts',(30.398359057145,-5.74808365594406,129.949045656226));
#224090=CARTESIAN_POINT('Ctrl Pts',(30.1199114333322,-3.82658032153943,
135.178067562667));
#224091=CARTESIAN_POINT('Ctrl Pts',(29.8414638095193,1.61136338951851,136.387866454021));
#224092=CARTESIAN_POINT('Ctrl Pts',(29.5630161857064,5.56854286508694,132.466696251098));
#224093=CARTESIAN_POINT('Ctrl Pts',(29.2845685618935,4.40850348608286,127.017920810568));
#224094=CARTESIAN_POINT('Ctrl Pts',(29.0061209380806,-0.802735229263066,
125.048698574801));
#224095=CARTESIAN_POINT('Ctrl Pts',(28.7276733142678,-5.27629948471241,
128.368648576612));
#224096=CARTESIAN_POINT('Ctrl Pts',(28.4492256904548,-4.90120227527057,
133.926898952911));
#224097=CARTESIAN_POINT('Ctrl Pts',(28.170778066642,-0.0221396118974229,
136.615689143506));
#224098=CARTESIAN_POINT('Ctrl Pts',(27.892330442829,4.87726827322928,133.964152317942));
#224099=CARTESIAN_POINT('Ctrl Pts',(27.6138828190162,5.29470488305963,128.408921284139));
#224100=CARTESIAN_POINT('Ctrl Pts',(27.3354351952032,0.846566366071392,
125.054981974037));
#224101=CARTESIAN_POINT('Ctrl Pts',(27.0569875713904,-4.37952528427021,
126.984440764576));
#224102=CARTESIAN_POINT('Ctrl Pts',(26.7785399475775,-5.58104715007188,
132.424219286554));
#224103=CARTESIAN_POINT('Ctrl Pts',(26.5000923237646,-1.65385933426847,
136.375426826225));
#224104=CARTESIAN_POINT('Ctrl Pts',(26.2216446999517,3.79314441420758,135.207096681855));
#224105=CARTESIAN_POINT('Ctrl Pts',(25.9431970761388,5.75443375143326,129.992867180015));
#224106=CARTESIAN_POINT('Ctrl Pts',(25.6647494523259,2.42767959080881,125.524360503627));
#224107=CARTESIAN_POINT('Ctrl Pts',(25.3863018285131,-3.12999351502748,
125.907915989602));
#224108=CARTESIAN_POINT('Ctrl Pts',(25.1078542047001,-5.81135548923757,
130.791064884058));
#224109=CARTESIAN_POINT('Ctrl Pts',(24.8294065808873,-3.152365669337,135.686431908074));
#224110=CARTESIAN_POINT('Ctrl Pts',(24.5509589570743,2.40349419906,136.095413918554));
#224111=CARTESIAN_POINT('Ctrl Pts',(24.2725113332615,5.75066031573997,131.64217642775));
#224112=CARTESIAN_POINT('Ctrl Pts',(23.9940637094486,3.81325053762949,126.419027136963));
#224113=CARTESIAN_POINT('Ctrl Pts',(23.7156160856357,-1.62835019691723,
125.2257850794));
#224114=CARTESIAN_POINT('Ctrl Pts',(23.4371684618228,-5.57357664982666,
129.158981412844));
#224115=CARTESIAN_POINT('Ctrl Pts',(23.1587208380098,-4.39695844590187,
134.604200854185));
#224116=CARTESIAN_POINT('Ctrl Pts',(22.880273214197,0.820249766445046,136.557552750588));
#224117=CARTESIAN_POINT('Ctrl Pts',(22.6018255903841,5.28368851485763,133.224002135804));
#224118=CARTESIAN_POINT('Ctrl Pts',(22.3233779665712,4.89167564065013,127.666919171818));
#224119=CARTESIAN_POINT('Ctrl Pts',(22.0449303427584,0.00445182432539013,
124.992991623939));
#224120=CARTESIAN_POINT('Ctrl Pts',(21.7664827189454,-4.88686300107076,
127.659428280044));
#224121=CARTESIAN_POINT('Ctrl Pts',(21.4880350951325,-5.28738946501251,
133.215904115845));
#224122=CARTESIAN_POINT('Ctrl Pts',(21.2095874713197,-0.829063313942982,
136.556289287176));
#224123=CARTESIAN_POINT('Ctrl Pts',(20.9311398475068,4.39113152064558,134.610933008472));
#224124=CARTESIAN_POINT('Ctrl Pts',(20.6526922236938,5.57609100646137,129.167522663925));
#224125=CARTESIAN_POINT('Ctrl Pts',(20.374244599881,1.6368952645291,125.228286434793));
#224126=CARTESIAN_POINT('Ctrl Pts',(20.0957969760681,-3.80652725872624,
126.413189973261));
#224127=CARTESIAN_POINT('Ctrl Pts',(19.8173493522552,-5.75193719040684,
131.633364813234));
#224128=CARTESIAN_POINT('Ctrl Pts',(19.5389017284423,-2.41159784185683,
136.091725296493));
#224129=CARTESIAN_POINT('Ctrl Pts',(19.2604541046294,3.14488211025528,135.691255941942));
#224130=CARTESIAN_POINT('Ctrl Pts',(18.9820064808165,5.81136903907515,130.799968522399));
#224131=CARTESIAN_POINT('Ctrl Pts',(18.7035588570036,3.13749172214556,125.912717223747));
#224132=CARTESIAN_POINT('Ctrl Pts',(18.4251112331907,-2.41958721244422,
125.52064723395));
#224133=CARTESIAN_POINT('Ctrl Pts',(18.1466636093778,-5.75318370220431,
129.984051719947));
#224134=CARTESIAN_POINT('Ctrl Pts',(17.868215985565,-3.79988542828747,135.201280008538));
#224135=CARTESIAN_POINT('Ctrl Pts',(17.589768361752,1.64532191950215,136.377954178279));
#224136=CARTESIAN_POINT('Ctrl Pts',(17.3113207379392,5.57855880171371,132.432768150908));
#224137=CARTESIAN_POINT('Ctrl Pts',(17.0328731141263,4.38537267289848,126.991155152525));
#224138=CARTESIAN_POINT('Ctrl Pts',(16.7544254903134,-0.83775670494522,
125.053691691071));
#224139=CARTESIAN_POINT('Ctrl Pts',(16.4759778665005,-5.29102859763445,
128.400812037271));
#224140=CARTESIAN_POINT('Ctrl Pts',(16.1975302426876,-4.88210369021464,
133.956676108886));
#224141=CARTESIAN_POINT('Ctrl Pts',(15.9190826188747,0.013236004487936,
136.61571624315));
#224142=CARTESIAN_POINT('Ctrl Pts',(15.6406349950618,4.89641245768097,133.934404458007));
#224143=CARTESIAN_POINT('Ctrl Pts',(15.3621873712489,5.2800250653117,128.376735294641));
#224144=CARTESIAN_POINT('Ctrl Pts',(15.0837397474361,0.811552581485459,
125.049935206953));
#224145=CARTESIAN_POINT('Ctrl Pts',(14.8052921236231,-4.40269707817821,
127.011170952307));
#224146=CARTESIAN_POINT('Ctrl Pts',(14.5268444998103,-5.57108320670569,
132.458162692417));
#224147=CARTESIAN_POINT('Ctrl Pts',(14.2483968759974,-1.6199160308156,136.385391118461));
#224148=CARTESIAN_POINT('Ctrl Pts',(13.9699492521845,3.81987484009636,135.18392516268));
#224149=CARTESIAN_POINT('Ctrl Pts',(13.6915016283715,5.74938734422005,129.95785334356));
#224150=CARTESIAN_POINT('Ctrl Pts',(13.4130540045587,2.39549375219187,125.509680355073));
#224151=CARTESIAN_POINT('Ctrl Pts',(13.1346063807458,-3.15974157172482,
125.927059868305));
#224152=CARTESIAN_POINT('Ctrl Pts',(12.8561587569329,-5.81132875318382,
130.82644050072));
#224153=CARTESIAN_POINT('Ctrl Pts',(12.57771113312,-3.12258870965941,135.705530799178));
#224154=CARTESIAN_POINT('Ctrl Pts',(12.2992635093071,2.43565781110307,136.080685136208));
#224155=CARTESIAN_POINT('Ctrl Pts',(12.0208158854942,5.75565379196074,131.607155003388));
#224156=CARTESIAN_POINT('Ctrl Pts',(11.7423682616813,3.78648511732596,126.395896048684));
#224157=CARTESIAN_POINT('Ctrl Pts',(11.4639206378685,-1.66227840004959,
125.235800667314));
#224158=CARTESIAN_POINT('Ctrl Pts',(11.1854730140555,-5.58348927459409,
129.192939840948));
#224159=CARTESIAN_POINT('Ctrl Pts',(10.9070253902426,-4.37374627440173,
134.630895986013));
#224160=CARTESIAN_POINT('Ctrl Pts',(10.6285777664298,0.855255882581734,
136.552453064119));
#224161=CARTESIAN_POINT('Ctrl Pts',(10.3501301426169,5.29831966504511,133.19179399377));
#224162=CARTESIAN_POINT('Ctrl Pts',(10.071682518804,4.87248651263752,127.637200283293));
#224163=CARTESIAN_POINT('Ctrl Pts',(9.79323489499104,-0.0309237106847325,
124.993072195629));
#224164=CARTESIAN_POINT('Ctrl Pts',(9.51478727117816,-4.90591655459505,
127.689234270502));
#224165=CARTESIAN_POINT('Ctrl Pts',(9.23633964736526,-5.27261175218,133.248045275945));
#224166=CARTESIAN_POINT('Ctrl Pts',(8.95789202355236,-0.794034330915497,
136.561229460968));
#224167=CARTESIAN_POINT('Ctrl Pts',(8.67944439973947,4.41422184972672,134.584132417584));
#224168=CARTESIAN_POINT('Ctrl Pts',(8.40099677592661,5.56602379719609,129.1336097421));
#224169=CARTESIAN_POINT('Ctrl Pts',(8.12254915211368,1.60292179042129,125.218425500451));
#224170=CARTESIAN_POINT('Ctrl Pts',(7.84410152830078,-3.83318703466779,
126.436442743329));
#224171=CARTESIAN_POINT('Ctrl Pts',(7.56565390448795,-5.74678423649425,
131.668363127979));
#224172=CARTESIAN_POINT('Ctrl Pts',(7.28720628067502,-2.37936747100029,
136.106307414428));
#224173=CARTESIAN_POINT('Ctrl Pts',(7.00875865686212,3.17457176177998,135.672021609062));
#224174=CARTESIAN_POINT('Ctrl Pts',(6.73031103304925,5.81123463193681,130.764593150968));
#224175=CARTESIAN_POINT('Ctrl Pts',(6.45186340923634,3.10765676993803,125.89370905193));
#224176=CARTESIAN_POINT('Ctrl Pts',(6.17341578542346,-2.45170584616043,
125.535473843045));
#224177=CARTESIAN_POINT('Ctrl Pts',(5.89496816161054,-5.75807056212669,
130.019088180515));
#224178=CARTESIAN_POINT('Ctrl Pts',(5.61652053779771,-3.77304972888379,
135.224329524944));
#224179=CARTESIAN_POINT('Ctrl Pts',(5.33807291398477,1.67921948147701,136.367835370977));
#224180=CARTESIAN_POINT('Ctrl Pts',(5.05962529017187,5.58836802279258,132.398779709476));
#224181=CARTESIAN_POINT('Ctrl Pts',(4.781177666359,4.36207935811697,126.964530794212));
#224182=CARTESIAN_POINT('Ctrl Pts',(4.50273004254611,-0.872747137244579,
125.058897900495));
#224183=CARTESIAN_POINT('Ctrl Pts',(4.2242824187332,-5.30556164954619,128.433064562307));
#224184=CARTESIAN_POINT('Ctrl Pts',(3.94583479492031,-4.86282419701095,
133.986336454649));
#224185=CARTESIAN_POINT('Ctrl Pts',(3.66738717110745,0.0486111304084952,
136.615528000873));
#224186=CARTESIAN_POINT('Ctrl Pts',(3.38893954729453,4.91537520376836,133.904540613147));
#224187=CARTESIAN_POINT('Ctrl Pts',(3.11049192348162,5.26514959429328,128.344639261694));
#224188=CARTESIAN_POINT('Ctrl Pts',(2.83204429966877,0.776508724519974,
125.045101672218));
#224189=CARTESIAN_POINT('Ctrl Pts',(2.55359667585587,-4.42570572852705,
127.038041698076));
#224190=CARTESIAN_POINT('Ctrl Pts',(2.27514905204296,-5.56091282480238,
132.492044816037));
#224191=CARTESIAN_POINT('Ctrl Pts',(1.99670142823006,-1.58591270077849,
136.395148603559));
#224192=CARTESIAN_POINT('Ctrl Pts',(1.7182538044172,3.84646371911817,135.160591357131));
#224193=CARTESIAN_POINT('Ctrl Pts',(1.43980618060429,5.7441278913444,129.922870874744));
#224194=CARTESIAN_POINT('Ctrl Pts',(1.16135855679139,2.36321914767325,125.495196402842));
#224195=CARTESIAN_POINT('Ctrl Pts',(0.882910932978526,-3.18937254303613,
125.946384477181));
#224196=CARTESIAN_POINT('Ctrl Pts',(0.604463309165634,-5.81108667620601,
130.861815299204));
#224197=CARTESIAN_POINT('Ctrl Pts',(0.326015685352703,-3.09269604130886,
135.724448075619));
#224198=CARTESIAN_POINT('Ctrl Pts',(0.0475680615398608,2.46773116894999,
136.065760837718));
#224199=CARTESIAN_POINT('Ctrl Pts',(-0.230879562273037,5.76043399031358,
131.572103831187));
#224200=CARTESIAN_POINT('Ctrl Pts',(-0.509327186085944,3.75957938742415,
126.37292831768));
#224201=CARTESIAN_POINT('Ctrl Pts',(-0.787774809898847,-1.69614500684454,
125.246022600264));
#224202=CARTESIAN_POINT('Ctrl Pts',(-1.06622243371171,-5.59319500111311,
129.226957980841));
#224203=CARTESIAN_POINT('Ctrl Pts',(-1.34467005752462,-4.35037203212501,
134.657449324165));
#224204=CARTESIAN_POINT('Ctrl Pts',(-1.62311768133752,0.890230306896913,
136.547140379971));
#224205=CARTESIAN_POINT('Ctrl Pts',(-1.90156530515039,5.31275448404895,
133.159497384516));
#224206=CARTESIAN_POINT('Ctrl Pts',(-2.18001292896328,4.85311683284533,
127.607598755059));
#224207=CARTESIAN_POINT('Ctrl Pts',(-2.4584605527762,-0.0662980998053887,
124.993368106748));
#224208=CARTESIAN_POINT('Ctrl Pts',(-2.73690817658909,-4.92478831757726,
127.719155693111));
#224209=CARTESIAN_POINT('Ctrl Pts',(-3.01535580040196,-5.25763866077998,
133.280095884409));
#224210=CARTESIAN_POINT('Ctrl Pts',(-3.29380342421486,-0.758975924653704,
136.565956311869));
#224211=CARTESIAN_POINT('Ctrl Pts',(-3.57225104802777,4.43714860819409,
134.557191765862));
#224212=CARTESIAN_POINT('Ctrl Pts',(-3.85069867184063,5.55575033687191,
129.099758730564));
#224213=CARTESIAN_POINT('Ctrl Pts',(-4.12914629565353,1.56888891945708,
125.208771554989));
#224214=CARTESIAN_POINT('Ctrl Pts',(-4.40759391946644,-3.85970477045413,
126.459857368199));
#224215=CARTESIAN_POINT('Ctrl Pts',(-4.68604154327934,-5.74141833337845,
131.703329426794));
#224216=CARTESIAN_POINT('Ctrl Pts',(-4.96448916709218,-2.34704893180687,
136.120693066776));
#224217=CARTESIAN_POINT('Ctrl Pts',(-5.24293679090511,3.20414377838073,
135.652606903212));
#224218=CARTESIAN_POINT('Ctrl Pts',(-5.52138441471801,5.81088488736209,
130.729219253137));
#224219=CARTESIAN_POINT('Ctrl Pts',(-5.79983203853088,3.07770666236606,
125.874882846113));
#224220=CARTESIAN_POINT('Ctrl Pts',(-6.07827966234377,-2.48373363101511,
125.550495692676));
#224221=CARTESIAN_POINT('Ctrl Pts',(-6.35672728615668,-5.7627440546269,
130.054153739642));
#224222=CARTESIAN_POINT('Ctrl Pts',(-6.63517490996957,-3.74607421773465,
135.247215257776));
#224223=CARTESIAN_POINT('Ctrl Pts',(-6.91362253378244,1.71305481935644,
136.357510407073));
#224224=CARTESIAN_POINT('Ctrl Pts',(-7.19207015759534,5.59797016483923,
132.36473218626));
#224225=CARTESIAN_POINT('Ctrl Pts',(-7.47051778140826,4.33862440488076,
126.938048722207));
#224226=CARTESIAN_POINT('Ctrl Pts',(-7.74896540522111,-0.907705229577551,
125.064317010151));
#224227=CARTESIAN_POINT('Ctrl Pts',(-8.027413029034,-5.31989810191992,128.46540495659));
#224228=CARTESIAN_POINT('Ctrl Pts',(-8.30586065284694,-4.84336451006833,
134.015878891129));
#224229=CARTESIAN_POINT('Ctrl Pts',(-8.58430827665978,0.0839844550257475,
136.615124423653));
#224230=CARTESIAN_POINT('Ctrl Pts',(-8.86275590047269,4.93415580881975,
133.874561889976));
#224231=CARTESIAN_POINT('Ctrl Pts',(-9.14120352428557,5.25007902122049,
128.312634374625));
#224232=CARTESIAN_POINT('Ctrl Pts',(-9.4196511480985,0.741436093738357,
125.040481548942));
#224233=CARTESIAN_POINT('Ctrl Pts',(-9.69809877191133,-4.44855038272257,
127.065052006178));
#224234=CARTESIAN_POINT('Ctrl Pts',(-9.97654639572428,-5.5505363812293,
132.525864401898));
#224235=CARTESIAN_POINT('Ctrl Pts',(-10.2549940195371,-1.55185060416301,
136.404698919952));
#224236=CARTESIAN_POINT('Ctrl Pts',(-10.53344164335,3.87291006601234,135.137096129849));
#224237=CARTESIAN_POINT('Ctrl Pts',(-10.8118892671629,5.7386555876974,129.887921069854));
#224238=CARTESIAN_POINT('Ctrl Pts',(-11.0903368909758,2.33085697319978,
125.480909183646));
#224239=CARTESIAN_POINT('Ctrl Pts',(-11.3687845147887,-3.21888533097506,
125.965889100148));
#224240=CARTESIAN_POINT('Ctrl Pts',(-11.6472321386015,-5.81062926727439,
130.897187968684));
#224241=CARTESIAN_POINT('Ctrl Pts',(-11.9256797624145,-3.06268877196916,
135.743183036409));
#224242=CARTESIAN_POINT('Ctrl Pts',(-12.2041273862274,2.49971308411117,
136.050641576106));
#224243=CARTESIAN_POINT('Ctrl Pts',(-12.4825750100403,5.76500073366654,
131.537024209977));
#224244=CARTESIAN_POINT('Ctrl Pts',(-12.7610226338531,3.73253434492532,
126.350124795028));
#224245=CARTESIAN_POINT('Ctrl Pts',(-13.039470257666,-1.7299487623625,125.256450499474));
#224246=CARTESIAN_POINT('Ctrl Pts',(-13.3179178814789,-5.60269346973446,
129.261034571969));
#224247=CARTESIAN_POINT('Ctrl Pts',(-13.5963655052918,-4.32683658521273,
134.683859884699));
#224248=CARTESIAN_POINT('Ctrl Pts',(-13.8748131291047,0.925171743400955,
136.541614895008));
#224249=CARTESIAN_POINT('Ctrl Pts',(-14.1532607529176,5.3269924369816,133.127113504801));
#224250=CARTESIAN_POINT('Ctrl Pts',(-14.4317083767304,4.83356731902416,
127.578115684011));
#224251=CARTESIAN_POINT('Ctrl Pts',(-14.7101560005434,-0.101670032225581,
124.99387934633));
#224252=CARTESIAN_POINT('Ctrl Pts',(-14.9886036243562,-4.94347759071707,
127.749191439124));
#224253=CARTESIAN_POINT('Ctrl Pts',(-15.2670512481692,-5.24247074564602,
133.312054753593));
#224254=CARTESIAN_POINT('Ctrl Pts',(-15.545498871982,-0.723889394260118,
136.570469664722));
#224255=CARTESIAN_POINT('Ctrl Pts',(-15.823946495795,4.45991094648802,134.530112051601));
#224256=CARTESIAN_POINT('Ctrl Pts',(-16.1023941196078,5.54527100617588,
129.065970883678));
#224257=CARTESIAN_POINT('Ctrl Pts',(-16.3808417434207,1.53479791273714,
125.199324956138));
#224258=CARTESIAN_POINT('Ctrl Pts',(-16.6592893672336,-3.88607948346057,
126.483432980235));
#224259=CARTESIAN_POINT('Ctrl Pts',(-16.9377369910465,-5.73583967989507,
131.738262413989));
#224260=CARTESIAN_POINT('Ctrl Pts',(-17.2161846148594,-2.31464342185212,
136.134881720468));
#224261=CARTESIAN_POINT('Ctrl Pts',(-17.4946322386723,3.23359706425542,
135.633012543814));
#224262=CARTESIAN_POINT('Ctrl Pts',(-17.7730798624852,5.81031981831091,
130.693848139697));
#224263=CARTESIAN_POINT('Ctrl Pts',(-18.0515274862981,3.04764250924188,
125.856239303907));
#224264=CARTESIAN_POINT('Ctrl Pts',(-18.3299751101109,-2.51566938020671,
125.565712226204));
#224265=CARTESIAN_POINT('Ctrl Pts',(-18.6084227339239,-5.76720400652691,
130.089247097961));
#224266=CARTESIAN_POINT('Ctrl Pts',(-18.8868703577367,-3.71895989442774,
135.269936358996));
#224267=CARTESIAN_POINT('Ctrl Pts',(-19.1653179815497,1.74682667935956,
136.346979669161));
#224268=CARTESIAN_POINT('Ctrl Pts',(-19.4437656053625,5.60736487204277,
132.330626842902));
#224269=CARTESIAN_POINT('Ctrl Pts',(-19.7222132291754,4.31500868232164,
126.91170991781));
#224270=CARTESIAN_POINT('Ctrl Pts',(-20.0006608529883,-0.942629686559699,
125.069948819234));
#224271=CARTESIAN_POINT('Ctrl Pts',(-20.2791084768012,-5.33403742351306,
128.497832021735));
#224272=CARTESIAN_POINT('Ctrl Pts',(-20.5575561006141,-4.82372535047263,
134.045302323618));
#224273=CARTESIAN_POINT('Ctrl Pts',(-20.836003724427,0.119354667568119,
136.614505526443));
#224274=CARTESIAN_POINT('Ctrl Pts',(-21.1144513482399,4.95275357691331,
133.844469399368));
#224275=CARTESIAN_POINT('Ctrl Pts',(-21.3928989720528,5.23481390453873,
128.280721819388));
#224276=CARTESIAN_POINT('Ctrl Pts',(-21.6713465958657,0.706335988769417,
125.036075008324));
#224277=CARTESIAN_POINT('Ctrl Pts',(-21.9497942196786,-4.47123019424771,
127.092200875735));
#224278=CARTESIAN_POINT('Ctrl Pts',(-22.2282418434914,-5.53995426048939,
132.559620196804));
#224279=CARTESIAN_POINT('Ctrl Pts',(-22.5066894673044,-1.5177310031529,
136.41404171375));
#224280=CARTESIAN_POINT('Ctrl Pts',(-22.7851370911172,3.89921290079955,
135.11344035146));
#224281=CARTESIAN_POINT('Ctrl Pts',(-23.0635847149301,5.73297063605735,
129.853005223969));
#224282=CARTESIAN_POINT('Ctrl Pts',(-23.342032338743,2.298408427964,125.466819226899));
#224283=CARTESIAN_POINT('Ctrl Pts',(-23.6204799625559,-3.24827884193431,
125.985573014458));
#224284=CARTESIAN_POINT('Ctrl Pts',(-23.8989275863688,-5.80995654333829,
130.932557198412));
#224285=CARTESIAN_POINT('Ctrl Pts',(-24.1773752101816,-3.03256801357094,
135.761734987319));
#224286=CARTESIAN_POINT('Ctrl Pts',(-24.4558228339946,2.53160237148462,
136.035327911625));
#224287=CARTESIAN_POINT('Ctrl Pts',(-24.7342704578075,5.76935385279724,
131.501917439649));
#224288=CARTESIAN_POINT('Ctrl Pts',(-25.0127180816204,3.70535099199371,
126.327486325724));
#224289=CARTESIAN_POINT('Ctrl Pts',(-25.2911657054332,-1.76368841399288,
125.267083978533));
#224290=CARTESIAN_POINT('Ctrl Pts',(-25.5696133292462,-5.61198432848891,
129.295168351611));
#224291=CARTESIAN_POINT('Ctrl Pts',(-25.8480609530591,-4.30314080577957,
134.71012668896));
#224292=CARTESIAN_POINT('Ctrl Pts',(-26.1265085768719,0.960078897325804,
136.535876813977));
#224293=CARTESIAN_POINT('Ctrl Pts',(-26.4049562006848,5.3410329962505,133.094643554625));
#224294=CARTESIAN_POINT('Ctrl Pts',(-26.6834038244978,4.81383869558843,
127.548752162656));
#224295=CARTESIAN_POINT('Ctrl Pts',(-26.9618514483106,-0.137038197225328,
124.994605895435));
#224296=CARTESIAN_POINT('Ctrl Pts',(-27.2402990721235,-4.96198368147699,
127.779340395554));
#224297=CARTESIAN_POINT('Ctrl Pts',(-27.5187466959364,-5.22710856883054,
133.343920699249));
#224298=CARTESIAN_POINT('Ctrl Pts',(-27.7971943197493,-0.688776039878604,
136.574769352283));
#224299=CARTESIAN_POINT('Ctrl Pts',(-28.0756419435621,4.48250802114168,
134.502894278251));
#224300=CARTESIAN_POINT('Ctrl Pts',(-28.3540895673751,5.53458619342344,
129.032247453463));
#224301=CARTESIAN_POINT('Ctrl Pts',(-28.632537191188,1.50065003351598,125.190086053944));
#224302=CARTESIAN_POINT('Ctrl Pts',(-28.9109848150008,-3.91231019636288,
126.507168705834));
#224303=CARTESIAN_POINT('Ctrl Pts',(-29.1894324388138,-5.73004848276283,
131.773160795109));
#224304=CARTESIAN_POINT('Ctrl Pts',(-29.4678800626266,-2.28215214193419,
136.148872849742));
#224305=CARTESIAN_POINT('Ctrl Pts',(-29.7463276864396,3.26293052800175,
135.613239256942));
#224306=CARTESIAN_POINT('Ctrl Pts',(-30.0247753102524,5.80953944572202,
130.658481121338));
#224307=CARTESIAN_POINT('Ctrl Pts',(-30.3032229340653,3.01746542460398,
125.837779116156));
#224308=CARTESIAN_POINT('Ctrl Pts',(-30.5816705578782,-2.54751191034413,
125.581122879776));
#224309=CARTESIAN_POINT('Ctrl Pts',(-30.8601181816911,-5.77145025256159,
130.124366955075));
#224310=CARTESIAN_POINT('Ctrl Pts',(-31.138565805504,-3.69170776369427,
135.292491986665));
#224311=CARTESIAN_POINT('Ctrl Pts',(-31.4170134293169,1.78053381005746,
136.336243547461));
#224312=CARTESIAN_POINT('Ctrl Pts',(-31.6954610531298,5.6165517962788,132.296464943187));
#224313=CARTESIAN_POINT('Ctrl Pts',(-31.9739086769427,4.29123306552915,
126.885515357016));
#224314=CARTESIAN_POINT('Ctrl Pts',(-32.2523563007555,-0.977519214052166,
125.075793119056));
#224315=CARTESIAN_POINT('Ctrl Pts',(-32.5308039245685,-5.34797909038788,
128.530344556146));
#224316=CARTESIAN_POINT('Ctrl Pts',(-32.8092515483813,-4.80390744596015,
134.07460566182));
#224317=CARTESIAN_POINT('Ctrl Pts',(-33.0876991721943,0.154720457379397,
136.613671332177));
#224318=CARTESIAN_POINT('Ctrl Pts',(-33.3661467960071,4.9711678189017,133.814264256411));
#224319=CARTESIAN_POINT('Ctrl Pts',(-33.64459441982,5.21935480990263,128.248902778514));
#224320=CARTESIAN_POINT('Ctrl Pts',(-33.9230420436329,0.671209710260644,
125.031882213649));
#224321=CARTESIAN_POINT('Ctrl Pts',(-34.2014896674458,-4.49374432269368,
127.119487300736));
#224322=CARTESIAN_POINT('Ctrl Pts',(-34.4799372912587,-5.52916685470707,
132.59331094992));
#224323=CARTESIAN_POINT('Ctrl Pts',(-34.7583849150716,-1.48355516206214,
136.423176638752));
#224324=CARTESIAN_POINT('Ctrl Pts',(-35.0368325388844,3.92537124881898,
135.089624898536));
#224325=CARTESIAN_POINT('Ctrl Pts',(-35.3152801626974,5.72707324708195,
129.818124630907));
#224326=CARTESIAN_POINT('Ctrl Pts',(-35.5937277865103,2.26587471435868,
125.45292705471));
#224327=CARTESIAN_POINT('Ctrl Pts',(-35.8721754103231,-3.27755198672651,
126.005435490714));
#224328=CARTESIAN_POINT('Ctrl Pts',(-36.1506230341361,-5.80906852932597,
130.967921677768));
#224329=CARTESIAN_POINT('Ctrl Pts',(-36.4290706579489,-3.00233488224952,
135.780103240898));
#224330=CARTESIAN_POINT('Ctrl Pts',(-36.7075182817618,2.56339784940132,
136.019820411726));
#224331=CARTESIAN_POINT('Ctrl Pts',(-36.9859659055747,5.77349318639923,
131.466784821096));
#224332=CARTESIAN_POINT('Ctrl Pts',(-37.2644135293876,3.67803033591843,
126.305013748643));
#224333=CARTESIAN_POINT('Ctrl Pts',(-37.5428611532005,-1.79736271150026,
125.277922643415));
#224334=CARTESIAN_POINT('Ctrl Pts',(-37.8213087770133,-5.62106723310019,
129.329358054928));
#224335=CARTESIAN_POINT('Ctrl Pts',(-38.0997564008263,-4.27928557188161,
134.736248763623));
#224336=CARTESIAN_POINT('Ctrl Pts',(-38.3782040246392,0.994950475174061,
136.529926349506));
#224337=CARTESIAN_POINT('Ctrl Pts',(-38.656651648452,5.35487564157755,133.062088737171));
#224338=CARTESIAN_POINT('Ctrl Pts',(-38.9350992722649,4.79393169358958,
127.51950927907));
#224339=CARTESIAN_POINT('Ctrl Pts',(-39.2135468960779,-0.172401284224016,
124.995547727136));
#224340=CARTESIAN_POINT('Ctrl Pts',(-39.4919945198907,-4.98030590410683,
127.809601445221));
#224341=CARTESIAN_POINT('Ctrl Pts',(-39.7704421437036,-5.21155269958477,
133.375692540572));
#224342=CARTESIAN_POINT('Ctrl Pts',(-40.0488897675166,-0.65363716264763,
136.578855215227));
#224343=CARTESIAN_POINT('Ctrl Pts',(-40.3273373913294,4.50493899481217,
134.475539454375));
#224344=CARTESIAN_POINT('Ctrl Pts',(-40.6057850151423,5.52369629454426,
128.998589689552));
#224345=CARTESIAN_POINT('Ctrl Pts',(-40.8842326389552,1.46644654715595,
125.181055190758));
#224346=CARTESIAN_POINT('Ctrl Pts',(-41.1626802627681,-3.93839593717207,
126.531063665459));
#224347=CARTESIAN_POINT('Ctrl Pts',(-41.441127886581,-5.72404495657686,
131.808023276983));
#224348=CARTESIAN_POINT('Ctrl Pts',(-41.7195755103939,-2.24957629602936,
136.162665936149));
#224349=CARTESIAN_POINT('Ctrl Pts',(-41.9980231342068,3.29214308265742,
135.593287775304));
#224350=CARTESIAN_POINT('Ctrl Pts',(-42.2764707580197,5.80854379851262,
130.623119508596));
#224351=CARTESIAN_POINT('Ctrl Pts',(-42.5549183818325,2.98717652667487,
125.81950296691));
#224352=CARTESIAN_POINT('Ctrl Pts',(-42.8333660056454,-2.57926004149102,
125.596727082342));
#224353=CARTESIAN_POINT('Ctrl Pts',(-43.1118136294584,-5.7754826353847,
130.159512009603));
#224354=CARTESIAN_POINT('Ctrl Pts',(-43.3902612532712,-3.66431883537201,
135.314881304976));
#224355=CARTESIAN_POINT('Ctrl Pts',(-43.6687088770841,1.81417496242045,
136.325302439805));
#224356=CARTESIAN_POINT('Ctrl Pts',(-43.947156500897,5.62553059712261,132.262247752997));
#224357=CARTESIAN_POINT('Ctrl Pts',(-44.2256041247099,4.26729843551711,
126.859466010475));
#224358=CARTESIAN_POINT('Ctrl Pts',(-44.5040517485228,-1.01237251921066,
125.081849693053));
#224359=CARTESIAN_POINT('Ctrl Pts',(-44.7824993723357,-5.3617225859308,
128.562941355057));
#224360=CARTESIAN_POINT('Ctrl Pts',(-45.0609469961486,-4.78391153089065,
134.103787819889));
#224361=CARTESIAN_POINT('Ctrl Pts',(-45.3393946199614,0.190080513966956,
136.612621871764));
#224362=CARTESIAN_POINT('Ctrl Pts',(-45.6178422437743,4.98939785243841,
133.783947580368));
#224363=CARTESIAN_POINT('Ctrl Pts',(-45.8962898675873,5.20370231015464,
128.217178431071));
#224364=CARTESIAN_POINT('Ctrl Pts',(-46.1747374914001,0.636058559829223,
125.027903320286));
#224365=CARTESIAN_POINT('Ctrl Pts',(-46.453185115213,-4.51609193379101,
127.146910270074));
#224366=CARTESIAN_POINT('Ctrl Pts',(-46.7316327390259,-5.51817456361365,
132.626935412823));
#224367=CARTESIAN_POINT('Ctrl Pts',(-47.0100803628388,-1.4493243472895,
136.43210335646));
#224368=CARTESIAN_POINT('Ctrl Pts',(-47.2885279866517,3.95138414076325,
135.06565065357));
#224369=CARTESIAN_POINT('Ctrl Pts',(-47.5669756104645,5.72096363930122,
129.783280583183));
#224370=CARTESIAN_POINT('Ctrl Pts',(-47.8454232342775,2.23325703793269,
125.439233181862));
#224371=CARTESIAN_POINT('Ctrl Pts',(-48.1238708580903,-3.30670368062431,
126.025475792906));
#224372=CARTESIAN_POINT('Ctrl Pts',(-48.4023184819033,-5.80796525814313,
131.00328009631));
#224373=CARTESIAN_POINT('Ctrl Pts',(-48.6807661057162,-2.97199049830493,
135.798287116504));
#224374=CARTESIAN_POINT('Ctrl Pts',(-48.9592137295291,2.59509833966803,
136.004119651047));
#224375=CARTESIAN_POINT('Ctrl Pts',(-49.2376613533419,5.77741858108801,
131.431627656171));
#224376=CARTESIAN_POINT('Ctrl Pts',(-49.5161089771548,3.65057338907646,
126.282707896514));
#224377=CARTESIAN_POINT('Ctrl Pts',(-49.7945566009678,-1.8309704070716,
125.288966092489));
#224378=CARTESIAN_POINT('Ctrl Pts',(-50.0730042247805,-5.62994184699806,
129.363602415007));
#224379=CARTESIAN_POINT('Ctrl Pts',(-50.3514518485936,-4.25527176748286,
134.762225140725));
#224380=CARTESIAN_POINT('Ctrl Pts',(-50.6298994724063,1.02978518476655,
136.52376372209));
#224381=CARTESIAN_POINT('Ctrl Pts',(-50.9083470962193,5.36851986001845,
133.029450258773));
#224382=CARTESIAN_POINT('Ctrl Pts',(-51.1867947200322,4.77384705068883,
127.490388116857));
#224383=CARTESIAN_POINT('Ctrl Pts',(-51.465242343845,-0.207757982829986,
124.996704806535));
#224384=CARTESIAN_POINT('Ctrl Pts',(-51.743689967658,-4.99844357966987,
127.839973466791));
#224385=CARTESIAN_POINT('Ctrl Pts',(-52.0221375914708,-5.19580371433717,
133.407369100245));
#224386=CARTESIAN_POINT('Ctrl Pts',(-52.3005852152837,-0.618474064651215,
136.58272710215));
#224387=CARTESIAN_POINT('Ctrl Pts',(-52.5790328390967,4.52720303631132,
134.448048593619));
#224388=CARTESIAN_POINT('Ctrl Pts',(-52.8574804629095,5.51260171306762,
128.964998839148));
#224389=CARTESIAN_POINT('Ctrl Pts',(-53.1359280867224,1.43218872108006,
125.172232701224));
#224390=CARTESIAN_POINT('Ctrl Pts',(-53.4143757105353,-3.96433573927151,
126.555116973674));
#224391=CARTESIAN_POINT('Ctrl Pts',(-53.6928233343482,-5.71782932379997,
131.842848567767));
#224392=CARTESIAN_POINT('Ctrl Pts',(-53.9712709581611,-2.21691709124776,
136.176260468582));
#224393=CARTESIAN_POINT('Ctrl Pts',(-54.249718581974,3.32123364574025,135.573158838211));
#224394=CARTESIAN_POINT('Ctrl Pts',(-54.5281662057869,5.80733291357678,
130.58776461181));
#224395=CARTESIAN_POINT('Ctrl Pts',(-54.8066138295998,2.95677693782102,
125.801411533396));
#224396=CARTESIAN_POINT('Ctrl Pts',(-55.0850614534126,-2.61091259720856,
125.612524255684));
#224397=CARTESIAN_POINT('Ctrl Pts',(-55.3635090772256,-5.77930100557468,
130.194680959234));
#224398=CARTESIAN_POINT('Ctrl Pts',(-55.6419567010384,-3.63679412436797,
135.337103484283));
#224399=CARTESIAN_POINT('Ctrl Pts',(-55.9204043248514,1.8477488898629,136.314156751619));
#224400=CARTESIAN_POINT('Ctrl Pts',(-56.1988519486642,5.63430094186134,
132.227976540264));
#224401=CARTESIAN_POINT('Ctrl Pts',(-56.4772995724772,4.24320567919224,
126.833562843453));
#224402=CARTESIAN_POINT('Ctrl Pts',(-56.7557471962901,-1.04718831053316,
125.088118316796));
#224403=CARTESIAN_POINT('Ctrl Pts',(-57.0341948201028,-5.3752674008715,
128.595621210585));
#224404=CARTESIAN_POINT('Ctrl Pts',(-57.3126424439159,-4.76373834622006,
134.13284771647));
#224405=CARTESIAN_POINT('Ctrl Pts',(-57.5910900677287,0.225433527051438,
136.611357184097));
#224406=CARTESIAN_POINT('Ctrl Pts',(-57.8695376915416,5.00744300200284,
133.753520494635));
#224407=CARTESIAN_POINT('Ctrl Pts',(-58.1479853153544,5.18785698530388,
128.185549952615));
#224408=CARTESIAN_POINT('Ctrl Pts',(-58.4264329391674,0.600883840013963,
125.024138475672));
#224409=CARTESIAN_POINT('Ctrl Pts',(-58.7048805629802,-4.53827219944114,
127.174468767579));
#224410=CARTESIAN_POINT('Ctrl Pts',(-58.9833281867932,-5.5069777945324,
132.660492339548));
#224411=CARTESIAN_POINT('Ctrl Pts',(-59.261775810606,-1.41503982726995,
136.440821536091));
#224412=CARTESIAN_POINT('Ctrl Pts',(-59.540223434419,3.97725061271504,135.041518504932));
#224413=CARTESIAN_POINT('Ctrl Pts',(-59.8186710582318,5.71464203910897,
129.748474371954));
#224414=CARTESIAN_POINT('Ctrl Pts',(-60.0971186820448,2.20055660734573,
125.425738115783));
#224415=CARTESIAN_POINT('Ctrl Pts',(-60.3755663058576,-3.3357328434014,
126.045693178431));
#224416=CARTESIAN_POINT('Ctrl Pts',(-60.6540139296705,-5.80664677067165,
131.038631143817));
#224417=CARTESIAN_POINT('Ctrl Pts',(-60.9324615534834,-2.94153598615947,
135.816285940328));
#224418=CARTESIAN_POINT('Ctrl Pts',(-61.2109091772963,2.62670266761142,
135.988226211385));
#224419=CARTESIAN_POINT('Ctrl Pts',(-61.4893568011092,5.78112989140647,
131.396447247635));
#224420=CARTESIAN_POINT('Ctrl Pts',(-61.767804424922,3.62298116889529,126.260569595891));
#224421=CARTESIAN_POINT('Ctrl Pts',(-62.046252048735,-1.86451025536104,
125.300213916535));
#224422=CARTESIAN_POINT('Ctrl Pts',(-62.3246996725479,-5.63860784133039,
129.39790016291));
#224423=CARTESIAN_POINT('Ctrl Pts',(-62.6031472963608,-4.23110028242386,
134.788054857702));
#224424=CARTESIAN_POINT('Ctrl Pts',(-62.8815949201736,1.0645817352901,136.517389160091));
#224425=CARTESIAN_POINT('Ctrl Pts',(-63.1600425439866,5.38196514598156,
132.99672932886));
#224426=CARTESIAN_POINT('Ctrl Pts',(-63.4384901677994,4.75358551113023,
127.461389755115));
#224427=CARTESIAN_POINT('Ctrl Pts',(-63.7169377916123,-0.243106982887504,
124.998077090756));
#224428=CARTESIAN_POINT('Ctrl Pts',(-63.9953854154252,-5.0163960360679,
127.870455334816));
#224429=CARTESIAN_POINT('Ctrl Pts',(-64.2738330392381,-5.17986219667218,
133.438949204482));
#224430=CARTESIAN_POINT('Ctrl Pts',(-64.552280663051,-0.583288048870894,
136.586384869579));
#224431=CARTESIAN_POINT('Ctrl Pts',(-64.8307282868638,4.54929932063727,
134.420422714664));
#224432=CARTESIAN_POINT('Ctrl Pts',(-65.1091759106768,5.50130286010717,
128.93147614697));
#224433=CARTESIAN_POINT('Ctrl Pts',(-65.3876235344896,1.39787782472419,
125.16361891226));
#224434=CARTESIAN_POINT('Ctrl Pts',(-65.6660711583025,-3.99012864145221,
126.579327739175));
#224435=CARTESIAN_POINT('Ctrl Pts',(-65.9445187821156,-5.71140181475477,
131.877635376998));
#224436=CARTESIAN_POINT('Ctrl Pts',(-66.2229664059283,-2.18417573778792,
136.189655943291));
#224437=CARTESIAN_POINT('Ctrl Pts',(-66.5014140297413,3.35020113928917,
135.552853191544));
#224438=CARTESIAN_POINT('Ctrl Pts',(-66.7798616535541,5.80590683578406,
130.552417741069));
#224439=CARTESIAN_POINT('Ctrl Pts',(-67.0583092773671,2.92626778451039,
125.783505486001));
#224440=CARTESIAN_POINT('Ctrl Pts',(-67.3367569011799,-2.64246840459962,
125.628513814431));
#224441=CARTESIAN_POINT('Ctrl Pts',(-67.6152045249929,-5.78290522164069,
130.229872500769));
#224442=CARTESIAN_POINT('Ctrl Pts',(-67.8936521488056,-3.60913465062,135.359157701137));
#224443=CARTESIAN_POINT('Ctrl Pts',(-68.1720997726187,1.88125434829088,
136.302806895912));
#224444=CARTESIAN_POINT('Ctrl Pts',(-68.4505473964314,5.64286250550667,
132.193652574919));
#224445=CARTESIAN_POINT('Ctrl Pts',(-68.7289950202444,4.21895568932047,
126.807806815805));
#224446=CARTESIAN_POINT('Ctrl Pts',(-69.0074426440573,-1.08196529790749,
125.094598758));
#224447=CARTESIAN_POINT('Ctrl Pts',(-69.2858902678701,-5.38861303330182,
128.628382911763));
#224448=CARTESIAN_POINT('Ctrl Pts',(-69.564337891683,-4.74338863947339,
134.161784274737));
#224449=CARTESIAN_POINT('Ctrl Pts',(-69.8427855154959,0.260778186613682,
136.609877316035));
#224450=CARTESIAN_POINT('Ctrl Pts',(-70.1212331393089,5.02530259892534,
133.722984126697));
#224451=CARTESIAN_POINT('Ctrl Pts',(-70.3996807631217,5.17181942250469,
128.154018515153));
#224452=CARTESIAN_POINT('Ctrl Pts',(-70.6781283869345,0.5656868542273,125.020587819316));
#224453=CARTESIAN_POINT('Ctrl Pts',(-70.9565760107477,-4.56028429774593,
127.202161772061));
#224454=CARTESIAN_POINT('Ctrl Pts',(-71.2350236345604,-5.49557696236377,
132.693980486629));
#224455=CARTESIAN_POINT('Ctrl Pts',(-71.5134712583732,-1.38070287242923,
136.449330854589));
#224456=CARTESIAN_POINT('Ctrl Pts',(-71.7919188821862,4.00296970618273,
135.017229346852));
#224457=CARTESIAN_POINT('Ctrl Pts',(-72.0703665059991,5.70810868075446,
129.71370728698));
#224458=CARTESIAN_POINT('Ctrl Pts',(-72.348814129812,2.16777463432419,125.412442356538));
#224459=CARTESIAN_POINT('Ctrl Pts',(-72.6272617536249,-3.36463839937136,
126.06608689813));
#224460=CARTESIAN_POINT('Ctrl Pts',(-72.9057093774378,-5.80511311576878,
131.073973510343));
#224461=CARTESIAN_POINT('Ctrl Pts',(-73.1841570012506,-2.91097247431594,
135.834099045416));
#224462=CARTESIAN_POINT('Ctrl Pts',(-73.4626046250635,2.65820966212185,
135.972140681676));
#224463=CARTESIAN_POINT('Ctrl Pts',(-73.7410522488765,5.78462697983096,
131.361244899111));
#224464=CARTESIAN_POINT('Ctrl Pts',(-74.0194998726893,3.59525469781404,
126.238599667113));
#224465=CARTESIAN_POINT('Ctrl Pts',(-74.2979474965022,-1.89798101353784,
125.31166569876));
#224466=CARTESIAN_POINT('Ctrl Pts',(-74.5763951203151,-5.64706489497548,
129.432250027724));
#224467=CARTESIAN_POINT('Ctrl Pts',(-74.854842744128,-4.20677201238788,
134.813736957424));
#224468=CARTESIAN_POINT('Ctrl Pts',(-75.1332903679409,1.09933883734644,
136.510802899716));
#224469=CARTESIAN_POINT('Ctrl Pts',(-75.4117379917539,5.39521100124704,
132.963927159917));
#224470=CARTESIAN_POINT('Ctrl Pts',(-75.6901856155667,4.73314782571214,
127.432515268386));
#224471=CARTESIAN_POINT('Ctrl Pts',(-75.9686332393795,-0.278446974526432,
124.99966452895));
#224472=CARTESIAN_POINT('Ctrl Pts',(-76.2470808631926,-5.03416260806588,
127.901045919781));
#224473=CARTESIAN_POINT('Ctrl Pts',(-76.5255284870053,-5.16372873730878,
133.470431683069));
#224474=CARTESIAN_POINT('Ctrl Pts',(-76.8039761108183,-0.548080419137594,
136.589828381972));
#224475=CARTESIAN_POINT('Ctrl Pts',(-77.0824237346311,4.57122702900371,
134.392662841198));
#224476=CARTESIAN_POINT('Ctrl Pts',(-77.360871358444,5.48980015434633,128.898022855216));
#224477=CARTESIAN_POINT('Ctrl Pts',(-77.639318982257,1.36351512949127,125.155214143056));
#224478=CARTESIAN_POINT('Ctrl Pts',(-77.9177666060698,-4.0157736879487,
126.603695064822));
#224479=CARTESIAN_POINT('Ctrl Pts',(-78.1962142298826,-5.70476266761487,
131.91238241564));
#224480=CARTESIAN_POINT('Ctrl Pts',(-78.4746618536957,-2.15135344889296,
136.202851863901));
#224481=CARTESIAN_POINT('Ctrl Pts',(-78.7531094775085,3.37904448990285,
135.532371587738));
#224482=CARTESIAN_POINT('Ctrl Pts',(-79.0315571013213,5.8042656179783,130.517080206165));
#224483=CARTESIAN_POINT('Ctrl Pts',(-79.3100047251342,2.8956501972711,125.765785488239));
#224484=CARTESIAN_POINT('Ctrl Pts',(-79.5884523489472,-2.67392629435197,
125.644695166086));
#224485=CARTESIAN_POINT('Ctrl Pts',(-79.8668999727601,-5.78629515002701,
130.265085330171));
#224486=CARTESIAN_POINT('Ctrl Pts',(-80.1453475965729,-3.58134143906054,
135.38104313831));
#224487=CARTESIAN_POINT('Ctrl Pts',(-80.4237952203859,1.91469009614739,
136.291253293255));
#224488=CARTESIAN_POINT('Ctrl Pts',(-80.7022428441988,5.65121497080658,
132.15927712885));
#224489=CARTESIAN_POINT('Ctrl Pts',(-80.9806904680116,4.19454936449412,
126.782198881926));
#224490=CARTESIAN_POINT('Ctrl Pts',(-81.2591380918246,-1.11670219266007,
125.10129077653));
#224491=CARTESIAN_POINT('Ctrl Pts',(-81.5375857156372,-5.40175898869456,
128.661225244595));
#224492=CARTESIAN_POINT('Ctrl Pts',(-81.8160333394505,-4.72286316471603,
134.190596422436));
#224493=CARTESIAN_POINT('Ctrl Pts',(-82.0944809632629,0.296113182944105,
136.608182322418));
#224494=CARTESIAN_POINT('Ctrl Pts',(-82.3729285870762,5.04297598141181,
133.692339608092));
#224495=CARTESIAN_POINT('Ctrl Pts',(-82.6513762108889,5.15559021603496,
128.122585287091));
#224496=CARTESIAN_POINT('Ctrl Pts',(-82.9298238347018,0.530468906706182,
125.017251482786));
#224497=CARTESIAN_POINT('Ctrl Pts',(-83.2082714585147,-4.58212741303929,
127.229988257347));
#224498=CARTESIAN_POINT('Ctrl Pts',(-83.4867190823277,-5.48397248956967,
132.72739861315));
#224499=CARTESIAN_POINT('Ctrl Pts',(-83.7651667061405,-1.34631475513585,
136.45763099664));
#224500=CARTESIAN_POINT('Ctrl Pts',(-84.0436143299535,4.02854046813582,
134.992784079373));
#224501=CARTESIAN_POINT('Ctrl Pts',(-84.3220619537663,5.70136380633342,
129.678980616565));
#224502=CARTESIAN_POINT('Ctrl Pts',(-84.6005095775792,2.13491233361711,
125.399346396808));
#224503=CARTESIAN_POINT('Ctrl Pts',(-84.8789572013921,-3.39341927742779,
126.086656196302));
#224504=CARTESIAN_POINT('Ctrl Pts',(-85.1574048252049,-5.80336435026449,
131.109305886265));
#224505=CARTESIAN_POINT('Ctrl Pts',(-85.4358524490179,-2.88030109531746,
135.851725771696));
#224506=CARTESIAN_POINT('Ctrl Pts',(-85.7143000728307,2.68961815569484,
135.955863657977));
#224507=CARTESIAN_POINT('Ctrl Pts',(-85.9927476966438,5.78790971677558,
131.326021915035));
#224508=CARTESIAN_POINT('Ctrl Pts',(-86.2711953204564,3.56739500324825,
126.216798924288));
#224509=CARTESIAN_POINT('Ctrl Pts',(-86.5496429442695,-1.93138144132926,
125.323321014816));
#224510=CARTESIAN_POINT('Ctrl Pts',(-86.8280905680822,-5.65531269455438,
129.466650736599));
#224511=CARTESIAN_POINT('Ctrl Pts',(-87.1065381918953,-4.18228785886808,
134.83927048823));
#224512=CARTESIAN_POINT('Ctrl Pts',(-87.3849858157081,1.13405520299706,
136.504005185026));
#224513=CARTESIAN_POINT('Ctrl Pts',(-87.663433439521,5.40825693498488,132.931044967442));
#224514=CARTESIAN_POINT('Ctrl Pts',(-87.9418810633338,4.71253475176078,
127.403765726628));
#224515=CARTESIAN_POINT('Ctrl Pts',(-88.2203286871468,-0.313776648210234,
125.00146706229));
#224516=CARTESIAN_POINT('Ctrl Pts',(-88.4987763109598,-5.05174263731727,
127.931744088139));
#224517=CARTESIAN_POINT('Ctrl Pts',(-88.7772239347726,-5.14740393407785,
133.501815369412));
#224518=CARTESIAN_POINT('Ctrl Pts',(-89.0556715585855,-0.512852480082647,
136.593057511728));
#224519=CARTESIAN_POINT('Ctrl Pts',(-89.3341191823985,4.59298534887173,
134.364770001874));
#224520=CARTESIAN_POINT('Ctrl Pts',(-89.6125668062112,5.47809402202166,
128.864640203508));
#224521=CARTESIAN_POINT('Ctrl Pts',(-89.8910144300243,1.32910190870433,
125.147018705051));
#224522=CARTESIAN_POINT('Ctrl Pts',(-90.169462053837,-4.04126992847403,
126.628218047677));
#224523=CARTESIAN_POINT('Ctrl Pts',(-90.44790967765,-5.69791212839678,131.947088396125));
#224524=CARTESIAN_POINT('Ctrl Pts',(-90.7263573014627,-2.1184514408047,
136.215847741432));
#224525=CARTESIAN_POINT('Ctrl Pts',(-91.0048049252757,3.40776262878029,
135.511714785749));
#224526=CARTESIAN_POINT('Ctrl Pts',(-91.2832525490887,5.80240932097568,
130.48175331654));
#224527=CARTESIAN_POINT('Ctrl Pts',(-91.5617001729014,2.86492531064864,
125.748252196732));
#224528=CARTESIAN_POINT('Ctrl Pts',(-91.8401477967144,-2.70528510078237,
125.661067711041));
#224529=CARTESIAN_POINT('Ctrl Pts',(-92.1185954205271,-5.78947066511866,
130.30031814262));
#224530=CARTESIAN_POINT('Ctrl Pts',(-92.3970430443404,-3.55341551957677,
135.402758984829));
#224531=CARTESIAN_POINT('Ctrl Pts',(-92.6754906681528,1.94805489445803,
136.279496371773));
#224532=CARTESIAN_POINT('Ctrl Pts',(-92.9539382919661,5.6593580282576,132.124851475851));
#224533=CARTESIAN_POINT('Ctrl Pts',(-93.2323859157787,4.16998760909852,
126.75673999073));
#224534=CARTESIAN_POINT('Ctrl Pts',(-93.5108335395918,-1.15139770760221,
125.10819412441));
#224535=CARTESIAN_POINT('Ctrl Pts',(-93.7892811634045,-5.41470477992152,
128.694146992097));
#224536=CARTESIAN_POINT('Ctrl Pts',(-94.0677287872175,-4.70216268252734,
134.219283091922));
#224537=CARTESIAN_POINT('Ctrl Pts',(-94.3461764110305,0.331437206691851,
136.606272266052));
#224538=CARTESIAN_POINT('Ctrl Pts',(-94.6246240348431,5.0604624945689,133.661588074364));
#224539=CARTESIAN_POINT('Ctrl Pts',(-94.9030716586564,5.13916996727372,
128.0912514332));
#224540=CARTESIAN_POINT('Ctrl Pts',(-95.1815192824688,0.495231302464415,
125.014129589715));
#224541=CARTESIAN_POINT('Ctrl Pts',(-95.459966906282,-4.60380073591605,
127.257947192314));
#224542=CARTESIAN_POINT('Ctrl Pts',(-95.7384145300948,-5.47216480615837,
132.760745480792));
#224543=CARTESIAN_POINT('Ctrl Pts',(-96.0168621539077,-1.31187674965409,
136.465721654678));
#224544=CARTESIAN_POINT('Ctrl Pts',(-96.2953097777207,4.05396195104042,
134.96818360832));
#224545=CARTESIAN_POINT('Ctrl Pts',(-96.5737574015334,5.69440766577999,
129.64429564752));
#224546=CARTESIAN_POINT('Ctrl Pts',(-96.8522050253465,2.10197092294792,
125.386450721867));
#224547=CARTESIAN_POINT('Ctrl Pts',(-97.1306526491593,-3.42207441108517,
126.107400310748));
#224548=CARTESIAN_POINT('Ctrl Pts',(-97.4091002729722,-5.80140053895979,
131.144626962327));
#224549=CARTESIAN_POINT('Ctrl Pts',(-97.6875478967851,-2.8495229857029,
135.869165466005));
#224550=CARTESIAN_POINT('Ctrl Pts',(-97.965995520598,2.72092698447821,135.93939574344));
#224551=CARTESIAN_POINT('Ctrl Pts',(-98.2444431444108,5.79097798059694,
131.290779600608));
#224552=CARTESIAN_POINT('Ctrl Pts',(-98.5228907682237,3.53940311754856,
126.195168175249));
#224553=CARTESIAN_POINT('Ctrl Pts',(-98.8013383920368,-1.96471030107164,
125.33517943281));
#224554=CARTESIAN_POINT('Ctrl Pts',(-99.0797860158496,-5.6633509344415,
129.501101014807));
#224555=CARTESIAN_POINT('Ctrl Pts',(-99.3582336396624,-4.15764872913354,
134.864654503967));
#224556=CARTESIAN_POINT('Ctrl Pts',(-99.6366812634755,1.16872954581563,
136.496996267908));
#224557=CARTESIAN_POINT('Ctrl Pts',(-99.9151288872883,5.42110246377302,
132.898083969897));
#224558=CARTESIAN_POINT('Ctrl Pts',(-100.193576511101,4.69174705310118,
127.375142195163));
#224559=CARTESIAN_POINT('Ctrl Pts',(-100.472024134914,-0.34909469478497,
125.003484623986));
#224560=CARTESIAN_POINT('Ctrl Pts',(-100.750471758727,-5.06913547238742,
127.96254870236));
#224561=CARTESIAN_POINT('Ctrl Pts',(-101.02891938254,-5.13088839190121,
133.533099100579));
#224562=CARTESIAN_POINT('Ctrl Pts',(-101.307367006353,-0.47760553709043,
136.596072139193));
#224563=CARTESIAN_POINT('Ctrl Pts',(-101.585814630166,4.61457347397855,
134.33674523027));
#224564=CARTESIAN_POINT('Ctrl Pts',(-101.864262253979,5.46618489690847,
128.831329428852));
#224565=CARTESIAN_POINT('Ctrl Pts',(-102.142709877791,1.29463943755703,
125.139032901931));
#224566=CARTESIAN_POINT('Ctrl Pts',(-102.421157501604,-4.06661641825637,
126.652895779031));
#224567=CARTESIAN_POINT('Ctrl Pts',(-102.699605125417,-5.69085045094906,
131.981752032413));
#224568=CARTESIAN_POINT('Ctrl Pts',(-102.97805274923,-2.08547093271925,
136.228643094318));
#224569=CARTESIAN_POINT('Ctrl Pts',(-103.256500373043,3.43635449176034,
135.490883551018));
#224570=CARTESIAN_POINT('Ctrl Pts',(-103.534947996856,5.80033801356182,
130.446438381249));
#224571=CARTESIAN_POINT('Ctrl Pts',(-103.813395620669,2.83409426316523,
125.730906261181));
#224572=CARTESIAN_POINT('Ctrl Pts',(-104.091843244482,-2.73654366187847,
125.677630842606));
#224573=CARTESIAN_POINT('Ctrl Pts',(-104.370290868295,-5.79243164924577,
130.335569632546));
#224574=CARTESIAN_POINT('Ctrl Pts',(-104.648738492108,-3.52535792697413,
135.424304436005));
#224575=CARTESIAN_POINT('Ctrl Pts',(-104.92718611592,1.98134750687769,136.267536567122));
#224576=CARTESIAN_POINT('Ctrl Pts',(-105.205633739733,5.66729137611554,
132.090376891579));
#224577=CARTESIAN_POINT('Ctrl Pts',(-105.484081363546,4.14527133327901,
126.731431085605));
#224578=CARTESIAN_POINT('Ctrl Pts',(-105.762528987359,-1.18605055707886,
125.115308545834));
#224579=CARTESIAN_POINT('Ctrl Pts',(-106.040976611172,-5.42744992727162,
128.72714693434));
#224580=CARTESIAN_POINT('Ctrl Pts',(-106.319424234985,-4.68128795997122,
134.247843220201));
#224581=CARTESIAN_POINT('Ctrl Pts',(-106.597871858798,0.366748948912009,
136.604147217717));
#224582=CARTESIAN_POINT('Ctrl Pts',(-106.876319482611,5.07776149042729,
133.630730665021));
#224583=CARTESIAN_POINT('Ctrl Pts',(-107.154767106424,5.12255928467941,
128.060018114567));
#224584=CARTESIAN_POINT('Ctrl Pts',(-107.433214730236,0.45997534724462,
125.011222255784));
#224585=CARTESIAN_POINT('Ctrl Pts',(-107.711662354049,-4.62530346326349,
127.286037540936));
#224586=CARTESIAN_POINT('Ctrl Pts',(-107.990109977862,-5.46015434966779,
132.794019853873));
#224587=CARTESIAN_POINT('Ctrl Pts',(-108.268557601675,-1.2773901320969,
136.473602528901));
#224588=CARTESIAN_POINT('Ctrl Pts',(-108.547005225488,4.07923321289408,
134.943428845277));
#224589=CARTESIAN_POINT('Ctrl Pts',(-108.825452849301,5.6872405168564,129.609653665109));
#224590=CARTESIAN_POINT('Ctrl Pts',(-109.103900473114,2.06895162297316,
125.373755809571));
#224591=CARTESIAN_POINT('Ctrl Pts',(-109.382348096927,-3.45060273851677,
126.128318472786));
#224592=CARTESIAN_POINT('Ctrl Pts',(-109.66079572074,-5.79922175462486,
131.179935429694));
#224593=CARTESIAN_POINT('Ctrl Pts',(-109.939243344552,-2.81863928596571,
135.886417482107));
#224594=CARTESIAN_POINT('Ctrl Pts',(-110.217690968365,2.7521349883118,135.922737548286));
#224595=CARTESIAN_POINT('Ctrl Pts',(-110.496138592178,5.79383165759959,
131.255519261747));
#224596=CARTESIAN_POINT('Ctrl Pts',(-110.774586215991,3.51128007796473,
126.17370822153));
#224597=CARTESIAN_POINT('Ctrl Pts',(-111.053033839804,-1.99796635775128,
125.347240513325));
#224598=CARTESIAN_POINT('Ctrl Pts',(-111.331481463617,-5.67117931677705,
129.535599585778));
#224599=CARTESIAN_POINT('Ctrl Pts',(-111.60992908743,-4.13285553619637,
134.889888064022));
#224600=CARTESIAN_POINT('Ctrl Pts',(-111.888376711243,1.20336058093108,
136.489776408084));
#224601=CARTESIAN_POINT('Ctrl Pts',(-112.166824335056,5.43374711161577,
132.865045388662));
#224602=CARTESIAN_POINT('Ctrl Pts',(-112.445271958868,4.67078550002918,
127.34664573465));
#224603=CARTESIAN_POINT('Ctrl Pts',(-112.723719582681,-0.384399805526852,
125.005717139274));
#224604=CARTESIAN_POINT('Ctrl Pts',(-113.002167206494,-5.08634046877848,
127.993458620965));
#224605=CARTESIAN_POINT('Ctrl Pts',(-113.280614830307,-5.11418272276831,
133.564281717336));
#224606=CARTESIAN_POINT('Ctrl Pts',(-113.55906245412,-0.442340896249408,
136.598872152659));
#224607=CARTESIAN_POINT('Ctrl Pts',(-113.837510077933,4.63599060436829,
134.308589564856));
#224608=CARTESIAN_POINT('Ctrl Pts',(-114.115957701746,5.45407322030374,
128.798091765594));
#224609=CARTESIAN_POINT('Ctrl Pts',(-114.394405325558,1.26012899306928,
125.131257029612));
#224610=CARTESIAN_POINT('Ctrl Pts',(-114.672852949372,-4.09181221807183,
126.677727344441));
#224611=CARTESIAN_POINT('Ctrl Pts',(-114.951300573184,-5.68357789694507,
132.016372040028));
#224612=CARTESIAN_POINT('Ctrl Pts',(-115.229748196997,-2.05241314674147,
136.241237448422));
#224613=CARTESIAN_POINT('Ctrl Pts',(-115.50819582081,3.46481901936097,135.469878655457));
#224614=CARTESIAN_POINT('Ctrl Pts',(-115.786643444623,5.79805177248978,
130.411136708898));
#224615=CARTESIAN_POINT('Ctrl Pts',(-116.065091068436,2.80315819727665,
125.713748324348));
#224616=CARTESIAN_POINT('Ctrl Pts',(-116.343538692249,-2.76770081934284,
125.694383947029));
#224617=CARTESIAN_POINT('Ctrl Pts',(-116.621986316062,-5.79517799268792,
130.370838493694));
#224618=CARTESIAN_POINT('Ctrl Pts',(-116.900433939875,-3.49716970093708,
135.445678693465));
#224619=CARTESIAN_POINT('Ctrl Pts',(-117.178881563688,2.0145666997373,136.255374322477));
#224620=CARTESIAN_POINT('Ctrl Pts',(-117.4573291875,5.67501472040751,132.055854653499));
#224621=CARTESIAN_POINT('Ctrl Pts',(-117.735776811314,4.12040145290537,
126.706273104381));
#224622=CARTESIAN_POINT('Ctrl Pts',(-118.014224435126,-1.22065945701595,
125.122633777175));
#224623=CARTESIAN_POINT('Ctrl Pts',(-118.29267205894,-5.43999395846872,
128.760223848501));
#224624=CARTESIAN_POINT('Ctrl Pts',(-118.571119682752,-4.6602397705682,
134.276275748964));
#224625=CARTESIAN_POINT('Ctrl Pts',(-118.849567306565,0.402047101114997,
136.601807256156));
#224626=CARTESIAN_POINT('Ctrl Pts',(-119.128014930377,5.09487232796628,
133.599768523497));
#224627=CARTESIAN_POINT('Ctrl Pts',(-119.406462554191,5.10575878376697,
128.028886488555));
#224628=CARTESIAN_POINT('Ctrl Pts',(-119.684910178003,0.424702347469154,
125.008529588725));
#224629=CARTESIAN_POINT('Ctrl Pts',(-119.963357801817,-4.64663479828973,
127.314258262312));
#224630=CARTESIAN_POINT('Ctrl Pts',(-120.241805425629,-5.44794156515001,
132.827220499399));
#224631=CARTESIAN_POINT('Ctrl Pts',(-120.520253049442,-1.24285618037906,
136.48127332728));
#224632=CARTESIAN_POINT('Ctrl Pts',(-120.798700673255,4.10435331726091,
134.918520707537));
#224633=CARTESIAN_POINT('Ctrl Pts',(-121.077148297068,5.67986262514396,
129.575055953004));
#224634=CARTESIAN_POINT('Ctrl Pts',(-121.355595920881,2.03585565723516,
125.361262130332));
#224635=CARTESIAN_POINT('Ctrl Pts',(-121.634043544694,-3.47900320259493,
126.149409907283));
#224636=CARTESIAN_POINT('Ctrl Pts',(-121.912491168507,-5.79682807799514,
131.215229979999));
#224637=CARTESIAN_POINT('Ctrl Pts',(-122.19093879232,-2.78765114051323,
135.903481180724));
#224638=CARTESIAN_POINT('Ctrl Pts',(-122.469386416133,2.78324101077128,
135.905889689793));
#224639=CARTESIAN_POINT('Ctrl Pts',(-122.747834039945,5.79647064203949,
131.220242205036));
#224640=CARTESIAN_POINT('Ctrl Pts',(-123.026281663758,3.48302692660634,
126.152419858339));
#224641=CARTESIAN_POINT('Ctrl Pts',(-123.304729287571,-2.03114837905279,
125.359503809431));
#224642=CARTESIAN_POINT('Ctrl Pts',(-123.583176911384,-5.67879755147744,
129.570145171156));
#224643=CARTESIAN_POINT('Ctrl Pts',(-123.861624535197,-4.10790919877744,
134.914970233354));
#224644=CARTESIAN_POINT('Ctrl Pts',(-124.14007215901,1.23794702507767,136.482345873087));
#224645=CARTESIAN_POINT('Ctrl Pts',(-124.418519782823,5.44619040996103,
132.831930447996));
#224646=CARTESIAN_POINT('Ctrl Pts',(-124.696967406636,4.64965086928273,
127.318277401031));
#224647=CARTESIAN_POINT('Ctrl Pts',(-124.975415030448,-0.419690672193134,
125.00816452543));
#224648=CARTESIAN_POINT('Ctrl Pts',(-125.253862654262,-5.10335698895296,
128.024472698579));
#224649=CARTESIAN_POINT('Ctrl Pts',(-125.532310278074,-5.09728754571388,
133.595362064203));
#224650=CARTESIAN_POINT('Ctrl Pts',(-125.810757901887,-0.407059864303788,
136.601457448367));
#224651=CARTESIAN_POINT('Ctrl Pts',(-126.0892055257,4.65723594642128,134.280304048949));
#224652=CARTESIAN_POINT('Ctrl Pts',(-126.367653149513,5.44175944101008,
128.764928445366));
#224653=CARTESIAN_POINT('Ctrl Pts',(-126.646100773326,1.22557185403828,
125.123691376234));
#224654=CARTESIAN_POINT('Ctrl Pts',(-126.924548397139,-4.11685639428078,
126.702711823764));
#224655=CARTESIAN_POINT('Ctrl Pts',(-127.202996020952,-5.67609473587197,
132.050947136115));
#224656=CARTESIAN_POINT('Ctrl Pts',(-127.481443644765,-2.01927930784003,
136.253630337055));
#224657=CARTESIAN_POINT('Ctrl Pts',(-127.759891268577,3.4931551568182,135.44870087741));
#224658=CARTESIAN_POINT('Ctrl Pts',(-128.038338892391,5.79555068247735,
130.375849607603));
#224659=CARTESIAN_POINT('Ctrl Pts',(-128.316786516203,2.77211825933019,
125.696779022025));
#224660=CARTESIAN_POINT('Ctrl Pts',(-128.595234140016,-2.7987554186355,
125.711326403516));
#224661=CARTESIAN_POINT('Ctrl Pts',(-128.873681763829,-5.79770959367839,
130.406123419165));
#224662=CARTESIAN_POINT('Ctrl Pts',(-129.152129387642,-3.46885188599067,
135.466880965177));
#224663=CARTESIAN_POINT('Ctrl Pts',(-129.430577011455,2.04771124208698,
136.243010088514));
#224664=CARTESIAN_POINT('Ctrl Pts',(-129.709024635268,5.68252777494204,
132.021286040849));
#224665=CARTESIAN_POINT('Ctrl Pts',(-129.98747225908,4.09537888954061,126.681266979298));
#224666=CARTESIAN_POINT('Ctrl Pts',(-130.265919882893,-1.25522312496795,
125.130169546993));
#224667=CARTESIAN_POINT('Ctrl Pts',(-130.544367506706,-5.45233640868912,
128.793376508901));
#224668=CARTESIAN_POINT('Ctrl Pts',(-130.822815130519,-4.63901889426667,
134.304579624636));
#224669=CARTESIAN_POINT('Ctrl Pts',(-131.101262754332,0.437330355314798,
136.599252468079));
#224670=CARTESIAN_POINT('Ctrl Pts',(-131.379710378145,5.11179437313754,
133.568702797104));
#224671=CARTESIAN_POINT('Ctrl Pts',(-131.658158001958,5.08876908708517,
127.997857708758));
#224672=CARTESIAN_POINT('Ctrl Pts',(-131.936605625771,0.389413610192037,
125.006051688315));
#224673=CARTESIAN_POINT('Ctrl Pts',(-132.215053249584,-4.66779395055513,
127.342608310716));
#224674=CARTESIAN_POINT('Ctrl Pts',(-132.493500873397,-5.43552690515385,
132.860346187109));
#224675=CARTESIAN_POINT('Ctrl Pts',(-132.77194849721,-1.20827617416795,
136.488733765571));
#224676=CARTESIAN_POINT('Ctrl Pts',(-133.050396121022,4.12932133330617,
134.893460118082));
#224677=CARTESIAN_POINT('Ctrl Pts',(-133.328843744835,5.67227426403318,
129.540503793235));
#224678=CARTESIAN_POINT('Ctrl Pts',(-133.607291368648,2.00268425211708,
125.348970147109));
#224679=CARTESIAN_POINT('Ctrl Pts',(-133.885738992461,-3.50727475093002,
126.170673832692));
#224680=CARTESIAN_POINT('Ctrl Pts',(-134.164186616274,-5.79421959776922,
131.25050930539));
#224681=CARTESIAN_POINT('Ctrl Pts',(-134.442634240087,-2.75655969762259,
135.920355929551));
#224682=CARTESIAN_POINT('Ctrl Pts',(-134.7210818639,2.81424389921159,135.888852792264));
#224683=CARTESIAN_POINT('Ctrl Pts',(-134.999529487713,5.79889483612785,
131.18494973768));
#224684=CARTESIAN_POINT('Ctrl Pts',(-135.277977111526,3.45464471040472,
126.131303874523));
#224685=CARTESIAN_POINT('Ctrl Pts',(-135.556424735338,-2.06425513540386,
125.371968866708));
#224686=CARTESIAN_POINT('Ctrl Pts',(-135.834872359151,-5.68620535624619,
129.604736490841));
#224687=CARTESIAN_POINT('Ctrl Pts',(-136.113319982964,-4.08281064127246,
134.939900082537));
#224688=CARTESIAN_POINT('Ctrl Pts',(-136.391767606777,1.27248759664198,
136.474704938258));
#224689=CARTESIAN_POINT('Ctrl Pts',(-136.67021523059,5.45843189771781,132.798740374984));
#224690=CARTESIAN_POINT('Ctrl Pts',(-136.948662854403,4.62834394401342,
127.290038245509));
#224691=CARTESIAN_POINT('Ctrl Pts',(-137.227110478216,-0.454965987067202,
125.010826691762));
#224692=CARTESIAN_POINT('Ctrl Pts',(-137.505558102029,-5.12018440235748,
128.055589785961));
#224693=CARTESIAN_POINT('Ctrl Pts',(-137.784005725841,-5.0802034867949,
133.626338989485));
#224694=CARTESIAN_POINT('Ctrl Pts',(-138.062453349655,-0.371763748605222,
136.603827930521));
#224695=CARTESIAN_POINT('Ctrl Pts',(-138.340900973467,4.67830871288359,
134.251889730681));
#224696=CARTESIAN_POINT('Ctrl Pts',(-138.61934859728,5.42924401531914,128.731840697047));
#224697=CARTESIAN_POINT('Ctrl Pts',(-138.897796221093,1.19096930099152,
125.116336222143));
#224698=CARTESIAN_POINT('Ctrl Pts',(-139.176243844906,-4.14174801886209,
126.727848291193));
#224699=CARTESIAN_POINT('Ctrl Pts',(-139.454691468719,-5.66840124502105,
132.085476039479));
#224700=CARTESIAN_POINT('Ctrl Pts',(-139.733139092532,-1.98607064380098,
136.265821300996));
#224701=CARTESIAN_POINT('Ctrl Pts',(-140.011586716345,3.52136185412693,
135.427351001626));
#224702=CARTESIAN_POINT('Ctrl Pts',(-140.290034340158,5.79283483620279,
130.340578384942));
#224703=CARTESIAN_POINT('Ctrl Pts',(-140.56848196397,2.7409755995222,125.679998983016));
#224704=CARTESIAN_POINT('Ctrl Pts',(-140.846929587784,-2.82970630901691,
125.72845758426));
#224705=CARTESIAN_POINT('Ctrl Pts',(-141.125377211596,-5.80002635840773,
130.441423101462));
#224706=CARTESIAN_POINT('Ctrl Pts',(-141.403824835409,-3.44040553146196,
135.487910465481));
#224707=CARTESIAN_POINT('Ctrl Pts',(-141.682272459222,2.08077990574355,
136.230444323395));
#224708=CARTESIAN_POINT('Ctrl Pts',(-141.960720083035,5.68983026132012,
131.986672334579));
#224709=CARTESIAN_POINT('Ctrl Pts',(-142.239167706848,4.07020457040501,
126.656413636965));
#224710=CARTESIAN_POINT('Ctrl Pts',(-142.517615330661,-1.289740280165,125.137915576048));
#224711=CARTESIAN_POINT('Ctrl Pts',(-142.796062954474,-5.46447682057862,
128.826603687055));
#224712=CARTESIAN_POINT('Ctrl Pts',(-143.074510578287,-4.61762611741445,
134.332753798405));
#224713=CARTESIAN_POINT('Ctrl Pts',(-143.352958202099,0.472597404077474,
136.596482948152));
#224714=CARTESIAN_POINT('Ctrl Pts',(-143.631405825913,5.12852699888841,
133.537534636997));
#224715=CARTESIAN_POINT('Ctrl Pts',(-143.909853449725,5.07159082419343,
127.966932924958));
#224716=CARTESIAN_POINT('Ctrl Pts',(-144.188301073538,0.354110443050382,
125.003788646376));
#224717=CARTESIAN_POINT('Ctrl Pts',(-144.466748697351,-4.6887801359991,
127.371086635623));
#224718=CARTESIAN_POINT('Ctrl Pts',(-144.745196321164,-5.4229108297093,
132.893395689516));
#224719=CARTESIAN_POINT('Ctrl Pts',(-145.023643944977,-1.17365139483885,
136.495983567324));
#224720=CARTESIAN_POINT('Ctrl Pts',(-145.30209156879,4.15413633583088,134.868248005541));
#224721=CARTESIAN_POINT('Ctrl Pts',(-145.580539192603,5.66447571471356,
129.505998466145));
#224722=CARTESIAN_POINT('Ctrl Pts',(-145.858986816416,1.96943863679757,
125.336880315387));
#224723=CARTESIAN_POINT('Ctrl Pts',(-146.137434440228,-3.53541633590941,
126.192109461069));
#224724=CARTESIAN_POINT('Ctrl Pts',(-146.415882064041,-5.79139641060527,
131.285772098575));
#224725=CARTESIAN_POINT('Ctrl Pts',(-146.694329687854,-2.72536610939861,
135.937041103293));
#224726=CARTESIAN_POINT('Ctrl Pts',(-146.972777311667,2.84514250480927,
135.871627487008));
#224727=CARTESIAN_POINT('Ctrl Pts',(-147.25122493548,5.80110415003576,131.149643167454));
#224728=CARTESIAN_POINT('Ctrl Pts',(-147.529672559293,3.42613448107249,
126.110361052543));
#224729=CARTESIAN_POINT('Ctrl Pts',(-147.808120183106,-2.09728540002206,
125.38463522326));
#224730=CARTESIAN_POINT('Ctrl Pts',(-148.086567806919,-5.69340245658434,
129.639372263039));
#224731=CARTESIAN_POINT('Ctrl Pts',(-148.365015430732,-4.05756079371773,
134.964676687782));
#224732=CARTESIAN_POINT('Ctrl Pts',(-148.643463054544,1.30698101571045,
136.466853886735));
#224733=CARTESIAN_POINT('Ctrl Pts',(-148.921910678358,5.47047112127328,
132.765476399497));
#224734=CARTESIAN_POINT('Ctrl Pts',(-149.20035830217,4.60686551375719,127.261929314495));
#224735=CARTESIAN_POINT('Ctrl Pts',(-149.478805925983,-0.49022444300932,
125.013703539625));
#224736=CARTESIAN_POINT('Ctrl Pts',(-149.757253549796,-5.13682208544599,
128.086808730058));
#224737=CARTESIAN_POINT('Ctrl Pts',(-150.035701173609,-5.06293117906749,
133.657211345319));
#224738=CARTESIAN_POINT('Ctrl Pts',(-150.314148797422,-0.336453857064764,
136.605983511281));
#224739=CARTESIAN_POINT('Ctrl Pts',(-150.592596421235,4.69920812289605,
134.223347662954));
#224740=CARTESIAN_POINT('Ctrl Pts',(-150.871044045047,5.41652740699458,
128.698829746717));
#224741=CARTESIAN_POINT('Ctrl Pts',(-151.14949166886,1.15632261613933,125.109191839888));
#224742=CARTESIAN_POINT('Ctrl Pts',(-151.427939292673,-4.1664861694474,
126.753135815284));
#224743=CARTESIAN_POINT('Ctrl Pts',(-151.706386916486,-5.66049770947745,
132.119957470642));
#224744=CARTESIAN_POINT('Ctrl Pts',(-151.984834540299,-1.95278838518384,
136.277809888502));
#224745=CARTESIAN_POINT('Ctrl Pts',(-152.263282164112,3.54943806607717,
135.405829819234));
#224746=CARTESIAN_POINT('Ctrl Pts',(-152.541729787925,5.78990433430307,
130.3053243479));
#224747=CARTESIAN_POINT('Ctrl Pts',(-152.820177411738,2.70973137185537,
125.663408829112));
#224748=CARTESIAN_POINT('Ctrl Pts',(-153.09862503555,-2.86055234359039,
125.745776854456));
#224749=CARTESIAN_POINT('Ctrl Pts',(-153.377072659364,-5.80212820102742,
130.476736232542));
#224750=CARTESIAN_POINT('Ctrl Pts',(-153.655520283176,-3.41183169144105,
135.508766415124));
#224751=CARTESIAN_POINT('Ctrl Pts',(-153.933967906989,2.1137714653355,136.21767749275));
#224752=CARTESIAN_POINT('Ctrl Pts',(-154.212415530802,5.69692190894542,
131.952014817313));
#224753=CARTESIAN_POINT('Ctrl Pts',(-154.490863154615,4.04487942834225,
126.631713998332));
#224754=CARTESIAN_POINT('Ctrl Pts',(-154.769310778428,-1.32420964356211,
125.145871577308));
#224755=CARTESIAN_POINT('Ctrl Pts',(-155.047758402241,-5.47641474427016,
128.859904151722));
#224756=CARTESIAN_POINT('Ctrl Pts',(-155.326206026054,-4.59606223272787,
134.360797226267));
#224757=CARTESIAN_POINT('Ctrl Pts',(-155.604653649866,0.507846940569522,
136.593498799002));
#224758=CARTESIAN_POINT('Ctrl Pts',(-155.88310127368,5.14506958518534,133.50626519812));
#224759=CARTESIAN_POINT('Ctrl Pts',(-156.161548897493,5.05422463163864,
127.936113283085));
#224760=CARTESIAN_POINT('Ctrl Pts',(-156.439996521305,0.318794154216047,
125.001740546765));
#224761=CARTESIAN_POINT('Ctrl Pts',(-156.718444145118,-4.70959257697085,
127.399692181761));
#224762=CARTESIAN_POINT('Ctrl Pts',(-156.996891768931,-5.41009380630968,
132.926367781962));
#224763=CARTESIAN_POINT('Ctrl Pts',(-157.275339392744,-1.1389831254257,
136.503022463895));
#224764=CARTESIAN_POINT('Ctrl Pts',(-157.553787016557,4.17879740530553,
134.84288530416));
#224765=CARTESIAN_POINT('Ctrl Pts',(-157.83223464037,5.65646726616335,129.471541250343));
#224766=CARTESIAN_POINT('Ctrl Pts',(-158.110682264183,1.93612004320555,
125.324993083158));
#224767=CARTESIAN_POINT('Ctrl Pts',(-158.389129887996,-3.56342691473634,
126.213715998108));
#224768=CARTESIAN_POINT('Ctrl Pts',(-158.667577511808,-5.78835862111754,
131.321017052882));
#224769=CARTESIAN_POINT('Ctrl Pts',(-158.946025135621,-2.69407153173119,
135.95353608367));
#224770=CARTESIAN_POINT('Ctrl Pts',(-159.224472759434,2.87593568260513,
135.854214412314));
#224771=CARTESIAN_POINT('Ctrl Pts',(-159.502920383247,5.80309850189603,
131.114323802656));
#224772=CARTESIAN_POINT('Ctrl Pts',(-159.78136800706,3.39749729506709,126.089592168444));
#224773=CARTESIAN_POINT('Ctrl Pts',(-160.059815630873,-2.13023794895846,
125.39750240973));
#224774=CARTESIAN_POINT('Ctrl Pts',(-160.338263254686,-5.70038858580074,
129.674051204309));
#224775=CARTESIAN_POINT('Ctrl Pts',(-160.616710878499,-4.03216059175559,
134.989299130986));
#224776=CARTESIAN_POINT('Ctrl Pts',(-160.895158502312,1.34142600411673,
136.458793009441));
#224777=CARTESIAN_POINT('Ctrl Pts',(-161.173606126125,5.48230763450959,
132.732139754142));
#224778=CARTESIAN_POINT('Ctrl Pts',(-161.452053749937,4.58521637440516,
127.233951649575));
#224779=CARTESIAN_POINT('Ctrl Pts',(-161.730501373751,-0.525464733504406,
125.016794962416));
#224780=CARTESIAN_POINT('Ctrl Pts',(-162.008948997563,-5.15326942170307,
128.118128374039));
#224781=CARTESIAN_POINT('Ctrl Pts',(-162.287396621376,-5.04547126256333,
133.687977987722));
#224782=CARTESIAN_POINT('Ctrl Pts',(-162.565844245189,-0.301131498102361,
136.607924110772));
#224783=CARTESIAN_POINT('Ctrl Pts',(-162.844291869002,4.71993340202341,
134.194678903404));
#224784=CARTESIAN_POINT('Ctrl Pts',(-163.122739492814,5.40361008725504,
128.665896817606));
#224785=CARTESIAN_POINT('Ctrl Pts',(-163.401187116628,1.12163308332736,
125.102258494207));
#224786=CARTESIAN_POINT('Ctrl Pts',(-163.67963474044,-4.19106992935549,
126.778573459));
#224787=CARTESIAN_POINT('Ctrl Pts',(-163.958082364253,-5.65238442210956,
132.154390151878));
#224788=CARTESIAN_POINT('Ctrl Pts',(-164.236529988066,-1.91943376527495,
136.289595655332));
#224789=CARTESIAN_POINT('Ctrl Pts',(-164.514977611879,3.57738275229458,
135.384138127707));
#224790=CARTESIAN_POINT('Ctrl Pts',(-164.793425235692,5.78675928536899,
130.270088802833));
#224791=CARTESIAN_POINT('Ctrl Pts',(-165.071872859505,2.67838673409632,
125.647009175068));
#224792=CARTESIAN_POINT('Ctrl Pts',(-165.350320483318,-2.89129237934434,
125.763283572333));
#224793=CARTESIAN_POINT('Ctrl Pts',(-165.628768107131,-5.80401504365309,
130.512061503863));
#224794=CARTESIAN_POINT('Ctrl Pts',(-165.907215730944,-3.38313142474212,
135.52944804128));
#224795=CARTESIAN_POINT('Ctrl Pts',(-166.185663354757,2.14668469834846,
136.204710069657));
#224796=CARTESIAN_POINT('Ctrl Pts',(-166.464110978569,5.70380245503433,
131.917314773299));
#224797=CARTESIAN_POINT('Ctrl Pts',(-166.742558602383,4.01940440178476,
126.607168978656));
#224798=CARTESIAN_POINT('Ctrl Pts',(-167.021006226195,-1.3586299378839,
125.15403725596));
#224799=CARTESIAN_POINT('Ctrl Pts',(-167.299453850008,-5.48814973739939,
128.893276668938));
#224800=CARTESIAN_POINT('Ctrl Pts',(-167.577901473821,-4.57432803926507,
134.388708869063));
#224801=CARTESIAN_POINT('Ctrl Pts',(-167.856349097634,0.543077658606429,
136.590300131209));
#224802=CARTESIAN_POINT('Ctrl Pts',(-168.134796721447,5.16142151903669,
133.474895639175));
#224803=CARTESIAN_POINT('Ctrl Pts',(-168.413244345259,5.03667115293141,
127.905399925171));
#224804=CARTESIAN_POINT('Ctrl Pts',(-168.691691969073,0.283466052347084,
124.999907465374));
#224805=CARTESIAN_POINT('Ctrl Pts',(-168.970139592885,-4.7302305022577,
127.42842388914));
#224806=CARTESIAN_POINT('Ctrl Pts',(-169.248587216698,-5.39707630989451,
132.959261242652));
#224807=CARTESIAN_POINT('Ctrl Pts',(-169.527034840511,-1.10427265057399,
136.509850194457));
#224808=CARTESIAN_POINT('Ctrl Pts',(-169.805482464324,4.20330362790601,
134.81737295376));
#224809=CARTESIAN_POINT('Ctrl Pts',(-170.083930088137,5.6482492151383,129.437133422652));
#224810=CARTESIAN_POINT('Ctrl Pts',(-170.36237771195,1.90272970597286,125.313308890908));
#224811=CARTESIAN_POINT('Ctrl Pts',(-170.640825335763,-3.59130544946847,
126.235492643171));
#224812=CARTESIAN_POINT('Ctrl Pts',(-170.919272959575,-5.78510634187241,
131.356242862295));
#224813=CARTESIAN_POINT('Ctrl Pts',(-171.197720583389,-2.66267712425244,
135.969840259458));
#224814=CARTESIAN_POINT('Ctrl Pts',(-171.476168207202,2.90662229154664,
135.836614213432));
#224815=CARTESIAN_POINT('Ctrl Pts',(-171.754615831014,5.80487781780722,
131.07899295206));
#224816=CARTESIAN_POINT('Ctrl Pts',(-172.033063454828,3.36873421355001,
126.068997991823));
#224817=CARTESIAN_POINT('Ctrl Pts',(-172.31151107864,-2.16311156114431,
125.410569949319));
#224818=CARTESIAN_POINT('Ctrl Pts',(-172.589958702453,-5.70716348502144,
129.70877202961));
#224819=CARTESIAN_POINT('Ctrl Pts',(-172.868406326266,-4.00661097660031,
135.013766499754));
#224820=CARTESIAN_POINT('Ctrl Pts',(-173.146853950079,1.3758212854888,136.450522605077));
#224821=CARTESIAN_POINT('Ctrl Pts',(-173.425301573892,5.49394099882038,
132.698731674224));
#224822=CARTESIAN_POINT('Ctrl Pts',(-173.703749197705,4.56339732817417,
127.206106287473));
#224823=CARTESIAN_POINT('Ctrl Pts',(-173.982196821517,-0.560685552710569,
125.02010084558));
#224824=CARTESIAN_POINT('Ctrl Pts',(-174.260644445331,-5.1695258016666,
128.149547557344));
#224825=CARTESIAN_POINT('Ctrl Pts',(-174.539092069143,-5.02782438426607,
133.718637776622));
#224826=CARTESIAN_POINT('Ctrl Pts',(-174.817539692956,-0.265797980601551,
136.609649657082));
#224827=CARTESIAN_POINT('Ctrl Pts',(-175.095987316769,4.74048378228282,
134.165884514362));
#224828=CARTESIAN_POINT('Ctrl Pts',(-175.374434940582,5.39049253475655,
128.633043130058));
#224829=CARTESIAN_POINT('Ctrl Pts',(-175.652882564395,1.08690198798901,
125.095536442018));
#224830=CARTESIAN_POINT('Ctrl Pts',(-175.931330188208,-4.21549838762608,
126.80416027974));
#224831=CARTESIAN_POINT('Ctrl Pts',(-176.209777812021,-5.64406168355824,
132.188772807274));
#224832=CARTESIAN_POINT('Ctrl Pts',(-176.488225435833,-1.886008020042,136.301178164761));
#224833=CARTESIAN_POINT('Ctrl Pts',(-176.766673059646,3.60519487727851,
135.362276730843));
#224834=CARTESIAN_POINT('Ctrl Pts',(-177.045120683459,5.78339980594152,
130.234873055403));
#224835=CARTESIAN_POINT('Ctrl Pts',(-177.323568307272,2.64694284773159,
125.630800628577));
#224836=CARTESIAN_POINT('Ctrl Pts',(-177.602015931085,-2.92192527719638,
125.780977089175));
#224837=CARTESIAN_POINT('Ctrl Pts',(-177.880463554898,-5.80568681636668,
130.547397606436));
#224838=CARTESIAN_POINT('Ctrl Pts',(-178.158911178711,-3.35430579486411,
135.549954577584));
#224839=CARTESIAN_POINT('Ctrl Pts',(-178.437358802524,2.17951838517049,
136.191542534628));
#224840=CARTESIAN_POINT('Ctrl Pts',(-178.715806426336,5.71047164462571,
131.88257348836));
#224841=CARTESIAN_POINT('Ctrl Pts',(-178.99425405015,3.99378043471903,126.582779487459));
#224842=CARTESIAN_POINT('Ctrl Pts',(-179.272701673962,-1.39299988767372,
125.162412309422));
#224843=CARTESIAN_POINT('Ctrl Pts',(-179.551149297775,-5.49968136512185,
128.926720002072));
#224844=CARTESIAN_POINT('Ctrl Pts',(-179.829596921588,-4.55242434239454,
134.416487692516));
#224845=CARTESIAN_POINT('Ctrl Pts',(-180.108044545401,0.578288252700551,
136.5868870633));
#224846=CARTESIAN_POINT('Ctrl Pts',(-180.386492169214,5.17758219451528,
133.443427122574));
#224847=CARTESIAN_POINT('Ctrl Pts',(-180.664939793027,5.01893103852278,
127.874793989312));
#224848=CARTESIAN_POINT('Ctrl Pts',(-180.94338741684,0.248127446539293,
124.998289470128));
#224849=CARTESIAN_POINT('Ctrl Pts',(-181.221835040653,-4.75069314711374,
127.457280693096));
#224850=CARTESIAN_POINT('Ctrl Pts',(-181.500282664465,-5.38385882283189,
132.992074852706));
#224851=CARTESIAN_POINT('Ctrl Pts',(-181.778730288279,-1.06952125649312,
136.516466506004));
#224852=CARTESIAN_POINT('Ctrl Pts',(-182.057177912091,4.22765409554481,
134.791711899713));
#224853=CARTESIAN_POINT('Ctrl Pts',(-182.335625535904,5.63982186616143,
129.402776258069));
#224854=CARTESIAN_POINT('Ctrl Pts',(-182.614073159717,1.86926886239121,
125.301828171599));
#224855=CARTESIAN_POINT('Ctrl Pts',(-182.89252078353,-3.61905090705647,
126.257438589318));
#224856=CARTESIAN_POINT('Ctrl Pts',(-183.170968407343,-5.78163969338434,
131.391448221508));
#224857=CARTESIAN_POINT('Ctrl Pts',(-183.449416031155,-2.63118405029363,
135.985953026497));
#224858=CARTESIAN_POINT('Ctrl Pts',(-183.727863654969,2.93720119453022,
135.818827542541));
#224859=CARTESIAN_POINT('Ctrl Pts',(-184.006311278781,5.80644203183612,
131.04365192486));
#224860=CARTESIAN_POINT('Ctrl Pts',(-184.284758902595,3.33984630234777,
126.048579285806));
#224861=CARTESIAN_POINT('Ctrl Pts',(-184.563206526407,-2.19590501843575,
125.423837357804));
#224862=CARTESIAN_POINT('Ctrl Pts',(-184.84165415022,-5.71372690320071,
129.743533452349));
#224863=CARTESIAN_POINT('Ctrl Pts',(-185.120101774033,-3.98091289500146,
135.03807788744));
#224864=CARTESIAN_POINT('Ctrl Pts',(-185.398549397846,1.41016558529749,
136.442042980103));
#224865=CARTESIAN_POINT('Ctrl Pts',(-185.676997021659,5.50537078312707,
132.665253397689));
#224866=CARTESIAN_POINT('Ctrl Pts',(-185.955444645472,4.54140918357699,
127.178394260007));
#224867=CARTESIAN_POINT('Ctrl Pts',(-186.233892269285,-0.595885595507362,
125.023621066618));
#224868=CARTESIAN_POINT('Ctrl Pts',(-186.512339893098,-5.18559062295048,
128.181065115723));
#224869=CARTESIAN_POINT('Ctrl Pts',(-186.79078751691,-5.00999119808726,
133.749189575911));
#224870=CARTESIAN_POINT('Ctrl Pts',(-187.069235140724,-0.230454613858838,
136.611160086272));
#224871=CARTESIAN_POINT('Ctrl Pts',(-187.347682764536,4.76085850217237,
134.136965562817));
#224872=CARTESIAN_POINT('Ctrl Pts',(-187.626130388349,5.37717523557474,
128.600269901479));
#224873=CARTESIAN_POINT('Ctrl Pts',(-187.904578012162,1.05213061709833,
125.089025932407));
#224874=CARTESIAN_POINT('Ctrl Pts',(-188.183025635975,-4.23977063905356,
126.829895329374));
#224875=CARTESIAN_POINT('Ctrl Pts',(-188.461473259788,-5.63552980222562,
132.223104162766));
#224876=CARTESIAN_POINT('Ctrl Pts',(-188.739920883601,-1.85251238808831,
136.312556987595));
#224877=CARTESIAN_POINT('Ctrl Pts',(-189.018368507414,3.63287341044046,
135.340246438718));
#224878=CARTESIAN_POINT('Ctrl Pts',(-189.296816131227,5.77982602050738,
130.199678410544));
#224879=CARTESIAN_POINT('Ctrl Pts',(-189.575263755039,2.61540087792624,
125.614783790254));
#224880=CARTESIAN_POINT('Ctrl Pts',(-189.853711378852,-2.95244990203274,
125.798856749341));
#224881=CARTESIAN_POINT('Ctrl Pts',(-190.132159002665,-5.80714345722022,
130.582743230867));
#224882=CARTESIAN_POINT('Ctrl Pts',(-190.410606626478,-3.32535586995153,
135.570285264159));
#224883=CARTESIAN_POINT('Ctrl Pts',(-190.689054250291,2.21227130913674,
136.178175375592));
#224884=CARTESIAN_POINT('Ctrl Pts',(-190.967501874104,5.7169292305904,131.847792249846));
#224885=CARTESIAN_POINT('Ctrl Pts',(-191.245949497917,3.96800847665057,
126.558546428502));
#224886=CARTESIAN_POINT('Ctrl Pts',(-191.52439712173,-1.4273182193404,125.170996427354));
#224887=CARTESIAN_POINT('Ctrl Pts',(-191.802844745543,-5.51100920012879,
128.960232911869));
#224888=CARTESIAN_POINT('Ctrl Pts',(-192.081292369355,-4.53035195376586,
134.444132667273));
#224889=CARTESIAN_POINT('Ctrl Pts',(-192.359739993168,0.613477418111232,
136.583259721745));
#224890=CARTESIAN_POINT('Ctrl Pts',(-192.638187616981,5.19355101278185,
133.411860814392));
#224891=CARTESIAN_POINT('Ctrl Pts',(-192.916635240794,5.00100494577841,
127.844296609621));
#224892=CARTESIAN_POINT('Ctrl Pts',(-193.195082864607,0.21277964627773,
124.996886620986));
#224893=CARTESIAN_POINT('Ctrl Pts',(-193.47353048842,-4.77097975328813,
127.486261524329));
#224894=CARTESIAN_POINT('Ctrl Pts',(-193.751978112233,-5.3704418349007,
133.024807396204));
#224895=CARTESIAN_POINT('Ctrl Pts',(-194.030425736046,-1.03473023090876,
136.522871153366));
#224896=CARTESIAN_POINT('Ctrl Pts',(-194.308873359859,4.25184790590635,
134.765903092897));
#224897=CARTESIAN_POINT('Ctrl Pts',(-194.587320983671,5.63118553151129,
129.368471029708));
#224898=CARTESIAN_POINT('Ctrl Pts',(-194.865768607484,1.83573875236439,
125.290551350653));
#224899=CARTESIAN_POINT('Ctrl Pts',(-195.144216231297,-3.64666225938173,
126.279553023333));
#224900=CARTESIAN_POINT('Ctrl Pts',(-195.42266385511,-5.77795880411129,
131.426631825972));
#224901=CARTESIAN_POINT('Ctrl Pts',(-195.701111478923,-2.59959347684268,
136.001873787725));
#224902=CARTESIAN_POINT('Ctrl Pts',(-195.979559102736,2.96767125844341,
135.800855058734));
#224903=CARTESIAN_POINT('Ctrl Pts',(-196.258006726549,5.80779108602021,
131.008302030633));
#224904=CARTESIAN_POINT('Ctrl Pts',(-196.536454350362,3.31083463191258,
126.028336807015));
#224905=CARTESIAN_POINT('Ctrl Pts',(-196.814901974175,-2.22861710565919,
125.437304143558));
#224906=CARTESIAN_POINT('Ctrl Pts',(-197.093349597988,-5.72007859712835,
129.778334184429));
#224907=CARTESIAN_POINT('Ctrl Pts',(-197.3717972218,-3.95506729921131,135.062232393175));
#224908=CARTESIAN_POINT('Ctrl Pts',(-197.650244845613,1.44445763090186,
136.433354448736));
#224909=CARTESIAN_POINT('Ctrl Pts',(-197.928692469426,5.51659656389443,
132.631706165088));
#224910=CARTESIAN_POINT('Ctrl Pts',(-198.207140093239,4.51925275539276,
127.150816594059));
#224911=CARTESIAN_POINT('Ctrl Pts',(-198.485587717052,-0.631063557543924,
125.027355495085));
#224912=CARTESIAN_POINT('Ctrl Pts',(-198.764035340865,-5.2014632902668,
128.212679881281));
#224913=CARTESIAN_POINT('Ctrl Pts',(-199.042482964678,-4.99197236484219,
133.779632253479));
#224914=CARTESIAN_POINT('Ctrl Pts',(-199.320930588491,-0.19510270753564,
136.612455342372));
#224915=CARTESIAN_POINT('Ctrl Pts',(-199.599378212304,4.7810568066993,134.10792312037));
#224916=CARTESIAN_POINT('Ctrl Pts',(-199.877825836116,5.36365868318719,
128.56757834629));
#224917=CARTESIAN_POINT('Ctrl Pts',(-200.156273459929,1.01732025912016,
125.082727206624));
#224918=CARTESIAN_POINT('Ctrl Pts',(-200.434721083742,-4.26388578422093,
126.855777654281));
#224919=CARTESIAN_POINT('Ctrl Pts',(-200.713168707555,-5.62678909426374,
132.257382946195));
#224920=CARTESIAN_POINT('Ctrl Pts',(-200.991616331368,-1.8189481106068,
136.323731702186));
#224921=CARTESIAN_POINT('Ctrl Pts',(-201.270063955181,3.66041732614217,
135.318048067677));
#224922=CARTESIAN_POINT('Ctrl Pts',(-201.548511578994,5.77603806149454,
130.164506172408));
#224923=CARTESIAN_POINT('Ctrl Pts',(-201.826959202806,2.58376199347953,
125.59895925361));
#224924=CARTESIAN_POINT('Ctrl Pts',(-202.10540682662,-2.9828651227522,125.816921890294));
#224925=CARTESIAN_POINT('Ctrl Pts',(-202.383854450432,-5.80838491223743,
130.618097067413));
#224926=CARTESIAN_POINT('Ctrl Pts',(-202.662302074245,-3.29628272275406,
135.590439347642));
#224927=CARTESIAN_POINT('Ctrl Pts',(-202.940749698058,2.24494225657654,
136.164609087875));
#224928=CARTESIAN_POINT('Ctrl Pts',(-203.219197321871,5.72317497363993,
131.812972346589));
#224929=CARTESIAN_POINT('Ctrl Pts',(-203.497644945684,3.94208948256877,
126.534470699752));
#224930=CARTESIAN_POINT('Ctrl Pts',(-203.776092569497,-1.46158366120557,
125.179789291667));
#224931=CARTESIAN_POINT('Ctrl Pts',(-204.05454019331,-5.52213282266317,
128.993814156497));
#224932=CARTESIAN_POINT('Ctrl Pts',(-204.332987817123,-4.5081116912795,
134.471642768938));
#224933=CARTESIAN_POINT('Ctrl Pts',(-204.611435440935,0.648643850890564,
136.579418240959));
#224934=CARTESIAN_POINT('Ctrl Pts',(-204.889883064748,5.20932738210573,
133.380197884332));
#224935=CARTESIAN_POINT('Ctrl Pts',(-205.168330688562,4.98289353895661,
127.813908916192));
#224936=CARTESIAN_POINT('Ctrl Pts',(-205.446778312374,0.177423961388546,
124.995698969927));
#224937=CARTESIAN_POINT('Ctrl Pts',(-205.725225936187,-4.79108956905296,
127.515365308944));
#224938=CARTESIAN_POINT('Ctrl Pts',(-206.00367356,-5.35682584327266,133.057457660231));
#224939=CARTESIAN_POINT('Ctrl Pts',(-206.282121183813,-0.999900863015179,
136.529063899218));
#224940=CARTESIAN_POINT('Ctrl Pts',(-206.560568807626,4.27588416248015,
134.739947489669));
#224941=CARTESIAN_POINT('Ctrl Pts',(-206.839016431439,5.62234053121038,
129.334219008764));
#224942=CARTESIAN_POINT('Ctrl Pts',(-207.117464055252,1.80214061836306,
125.279478845937));
#224943=CARTESIAN_POINT('Ctrl Pts',(-207.395911679064,-3.67413848329639,
126.301835125757));
#224944=CARTESIAN_POINT('Ctrl Pts',(-207.674359302878,-5.77406381044983,
131.461792371951));
#224945=CARTESIAN_POINT('Ctrl Pts',(-207.95280692669,-2.56790657449899,
136.01760195319));
#224946=CARTESIAN_POINT('Ctrl Pts',(-208.231254550503,2.99803135420673,
135.782697427989));
#224947=CARTESIAN_POINT('Ctrl Pts',(-208.509702174316,5.8089249303698,130.972944579282));
#224948=CARTESIAN_POINT('Ctrl Pts',(-208.788149798129,3.28170027728254,
126.008271305542));
#224949=CARTESIAN_POINT('Ctrl Pts',(-209.066597421942,-2.2612466106562,
125.450969807563));
#224950=CARTESIAN_POINT('Ctrl Pts',(-209.345045045754,-5.72621833144002,
129.813172936296));
#224951=CARTESIAN_POINT('Ctrl Pts',(-209.623492669568,-3.92907514694791,
135.086229121905));
#224952=CARTESIAN_POINT('Ctrl Pts',(-209.90194029338,1.4786961515975,136.424457332932));
#224953=CARTESIAN_POINT('Ctrl Pts',(-210.180387917194,5.52761792514773,
132.598091219525));
#224954=CARTESIAN_POINT('Ctrl Pts',(-210.458835541006,4.49692886463537,
127.123374311529));
#224955=CARTESIAN_POINT('Ctrl Pts',(-210.73728316482,-0.666218135288655,
125.031303992602));
#224956=CARTESIAN_POINT('Ctrl Pts',(-211.015730788632,-5.21714321544808,
128.244390682522));
#224957=CARTESIAN_POINT('Ctrl Pts',(-211.294178412445,-4.97376855222533,
133.809964681263));
#224958=CARTESIAN_POINT('Ctrl Pts',(-211.572626036258,-0.159743571609885,
136.613535377387));
#224959=CARTESIAN_POINT('Ctrl Pts',(-211.851073660071,4.80107794740803,
134.0787582632));
#224960=CARTESIAN_POINT('Ctrl Pts',(-212.129521283884,5.34994337845465,
128.534969675892));
#224961=CARTESIAN_POINT('Ctrl Pts',(-212.407968907697,0.982472203965689,
125.076640498072));
#224962=CARTESIAN_POINT('Ctrl Pts',(-212.686416531509,-4.28784292953254,
126.881806295382));
#224963=CARTESIAN_POINT('Ctrl Pts',(-212.964864155322,-5.61783988356258,
132.291607887347));
#224964=CARTESIAN_POINT('Ctrl Pts',(-213.243311779135,-1.78531643133465,
136.334701894451));
#224965=CARTESIAN_POINT('Ctrl Pts',(-213.521759402948,3.68782560373359,
135.295682440288));
#224966=CARTESIAN_POINT('Ctrl Pts',(-213.800207026761,5.77203606926717,
130.129357644311));
#224967=CARTESIAN_POINT('Ctrl Pts',(-214.078654650574,2.55202736678199,
125.583327605028));
#224968=CARTESIAN_POINT('Ctrl Pts',(-214.357102274386,-3.0131698123076,
125.835171842623));
#224969=CARTESIAN_POINT('Ctrl Pts',(-214.6355498982,-5.80941113541564,130.653457806023));
#224970=CARTESIAN_POINT('Ctrl Pts',(-214.913997522012,-3.26708743058812,
135.610416081219));
#224971=CARTESIAN_POINT('Ctrl Pts',(-215.192445145826,2.27753001685547,
136.15084417418));
#224972=CARTESIAN_POINT('Ctrl Pts',(-215.470892769638,5.72920864233609,
131.778115068854));
#224973=CARTESIAN_POINT('Ctrl Pts',(-215.749340393451,3.9160244129115,126.510553193344));
#224974=CARTESIAN_POINT('Ctrl Pts',(-216.027788017264,-1.49579494355069,
125.18879057654));
#224975=CARTESIAN_POINT('Ctrl Pts',(-216.306235641077,-5.53305182053502,
129.02746249159));
#224976=CARTESIAN_POINT('Ctrl Pts',(-216.58468326489,-4.48570437905656,
134.499016978113));
#224977=CARTESIAN_POINT('Ctrl Pts',(-216.863130888703,0.683786247933482,
136.57536276329));
#224978=CARTESIAN_POINT('Ctrl Pts',(-217.141578512516,5.2249107178877,133.348439505674));
#224979=CARTESIAN_POINT('Ctrl Pts',(-217.420026136328,4.96459748918233,
127.78363203505));
#224980=CARTESIAN_POINT('Ctrl Pts',(-217.698473760142,0.142061701988793,
124.994726560962));
#224981=CARTESIAN_POINT('Ctrl Pts',(-217.976921383954,-4.81102184923216,
127.544590968491));
#224982=CARTESIAN_POINT('Ctrl Pts',(-218.255369007768,-5.34301135249269,
133.090024434919));
#224983=CARTESIAN_POINT('Ctrl Pts',(-218.53381663158,-0.965034443427401,
136.535044514085));
#224984=CARTESIAN_POINT('Ctrl Pts',(-218.812264255394,4.29976197459382,
134.713846051821));
#224985=CARTESIAN_POINT('Ctrl Pts',(-219.090711879206,5.61328719301349,
129.300021464458));
#224986=CARTESIAN_POINT('Ctrl Pts',(-219.369159503019,1.76847570537835,
125.268611067748));
#224987=CARTESIAN_POINT('Ctrl Pts',(-219.647607126831,-3.70147856065836,
126.324284070919));
#224988=CARTESIAN_POINT('Ctrl Pts',(-219.926054750645,-5.76995485673049,
131.496928556552));
#224989=CARTESIAN_POINT('Ctrl Pts',(-220.204502374457,-2.5361245174328,
136.033136940081));
#224990=CARTESIAN_POINT('Ctrl Pts',(-220.48294999827,3.02828035681523,135.764355323142));
#224991=CARTESIAN_POINT('Ctrl Pts',(-220.761397622083,5.80984352286985,
130.937580880991));
#224992=CARTESIAN_POINT('Ctrl Pts',(-221.039845245896,3.25244431804234,
125.988383524923));
#224993=CARTESIAN_POINT('Ctrl Pts',(-221.318292869709,-2.29379232432851,
125.464833843433));
#224994=CARTESIAN_POINT('Ctrl Pts',(-221.596740493522,-5.73214587862558,
129.848048416986));
#224995=CARTESIAN_POINT('Ctrl Pts',(-221.875188117335,-3.90293740136003,
135.110067184424));
#224996=CARTESIAN_POINT('Ctrl Pts',(-222.153635741148,1.51287987866345,
136.415351962378));
#224997=CARTESIAN_POINT('Ctrl Pts',(-222.432083364961,5.53843445848603,
132.564409806615));
#224998=CARTESIAN_POINT('Ctrl Pts',(-222.710530988774,4.47443833852516,
127.0960684293));
#224999=CARTESIAN_POINT('Ctrl Pts',(-222.988978612586,-0.701348026075381,
125.035466412855));
#225000=CARTESIAN_POINT('Ctrl Pts',(-223.267426236399,-5.23262981746888,
128.27619634439));
#225001=CARTESIAN_POINT('Ctrl Pts',(-223.545873860212,-4.95538043478568,
133.840185735283));
#225002=CARTESIAN_POINT('Ctrl Pts',(-223.824321484025,-0.124378516327312,
136.614400151295));
#225003=CARTESIAN_POINT('Ctrl Pts',(-224.102769107838,4.82092118240782,
134.049472072021));
#225004=CARTESIAN_POINT('Ctrl Pts',(-224.381216731651,5.33602982960279,
128.502445098609));
#225005=CARTESIAN_POINT('Ctrl Pts',(-224.659664355464,0.947587742942381,
125.070766032295));
#225006=CARTESIAN_POINT('Ctrl Pts',(-224.938111979277,-4.31164118724753,
126.907980288176));
#225007=CARTESIAN_POINT('Ctrl Pts',(-225.216559603089,-5.60868250173869,
132.325777718005));
#225008=CARTESIAN_POINT('Ctrl Pts',(-225.495007226903,-1.75161859650508,
136.345467157888));
#225009=CARTESIAN_POINT('Ctrl Pts',(-225.773454850715,3.71509722759125,
135.273150385318));
#225010=CARTESIAN_POINT('Ctrl Pts',(-226.051902474528,5.7678201921206,130.0942341287));
#225011=CARTESIAN_POINT('Ctrl Pts',(-226.330350098341,2.52019817377184,
125.567889423742));
#225012=CARTESIAN_POINT('Ctrl Pts',(-226.608797722154,-3.04336284774751,
125.853605930069));
#225013=CARTESIAN_POINT('Ctrl Pts',(-226.887245345967,-5.81022208872781,
130.688824136393));
#225014=CARTESIAN_POINT('Ctrl Pts',(-227.16569296978,-3.23777107529596,
135.630214724643));
#225015=CARTESIAN_POINT('Ctrl Pts',(-227.444140593593,2.31003338242206,
136.13688114457));
#225016=CARTESIAN_POINT('Ctrl Pts',(-227.722588217406,5.73503001309909,
131.74322170829));
#225017=CARTESIAN_POINT('Ctrl Pts',(-228.001035841218,3.88981423352964,
126.486794795549));
#225018=CARTESIAN_POINT('Ctrl Pts',(-228.279483465031,-1.52995079866356,
125.197999948425));
#225019=CARTESIAN_POINT('Ctrl Pts',(-228.557931088844,-5.54376578913698,
129.061176670297));
#225020=CARTESIAN_POINT('Ctrl Pts',(-228.836378712657,-4.46313084740822,
134.526254280438));
#225021=CARTESIAN_POINT('Ctrl Pts',(-229.11482633647,0.718903307025501,
136.571093439014));
#225022=CARTESIAN_POINT('Ctrl Pts',(-229.393273960283,5.24030044268158,
133.316586855238));
#225023=CARTESIAN_POINT('Ctrl Pts',(-229.671721584096,4.94611747442232,
127.753467088116));
#225024=CARTESIAN_POINT('Ctrl Pts',(-229.950169207909,0.106694178440453,
124.993969430123));
#225025=CARTESIAN_POINT('Ctrl Pts',(-230.228616831722,-4.83077585522751,
127.57393742));
#225026=CARTESIAN_POINT('Ctrl Pts',(-230.507064455534,-5.32899887446215,
133.122506513493));
#225027=CARTESIAN_POINT('Ctrl Pts',(-230.785512079348,-0.930132264133436,
136.540812776352));
#225028=CARTESIAN_POINT('Ctrl Pts',(-231.06395970316,4.3234804574463,134.687599746553));
#225029=CARTESIAN_POINT('Ctrl Pts',(-231.342407326973,5.60402585239536,
129.265879663993));
#225030=CARTESIAN_POINT('Ctrl Pts',(-231.620854950786,1.73474526087603,
125.257948418793));
#225031=CARTESIAN_POINT('Ctrl Pts',(-231.899302574599,-3.72868147837107,
126.346899026965));
#225032=CARTESIAN_POINT('Ctrl Pts',(-232.177750198412,-5.76563209521201,
131.532039077795));
#225033=CARTESIAN_POINT('Ctrl Pts',(-232.456197822225,-2.50424848333998,
136.048478172742));
#225034=CARTESIAN_POINT('Ctrl Pts',(-232.734645446038,3.05841714538193,
135.745829423867));
#225035=CARTESIAN_POINT('Ctrl Pts',(-233.01309306985,5.81054682948159,130.902212246173));
#225036=CARTESIAN_POINT('Ctrl Pts',(-233.291540693664,3.22306783828139,
125.968674202107));
#225037=CARTESIAN_POINT('Ctrl Pts',(-233.569988317476,-2.32625304068266,
125.478895737432));
#225038=CARTESIAN_POINT('Ctrl Pts',(-233.84843594129,-5.73786101903762,
129.882959334177));
#225039=CARTESIAN_POINT('Ctrl Pts',(-234.126883565102,-3.87665503099142,
135.133745697402));
#225040=CARTESIAN_POINT('Ctrl Pts',(-234.405331188915,1.54700754540913,
136.406038674476));
#225041=CARTESIAN_POINT('Ctrl Pts',(-234.683778812728,5.54904576309872,
132.530663174436));
#225042=CARTESIAN_POINT('Ctrl Pts',(-234.962226436541,4.45178201045685,
127.0688999592));
#225043=CARTESIAN_POINT('Ctrl Pts',(-235.240674060353,-0.736451928153096,
125.039842601604));
#225044=CARTESIAN_POINT('Ctrl Pts',(-235.519121684167,-5.24792252246713,
128.308095688315));
#225045=CARTESIAN_POINT('Ctrl Pts',(-235.797569307979,-4.93680869390195,
133.870294295687));
#225046=CARTESIAN_POINT('Ctrl Pts',(-236.076016931792,-0.0890088521534987,
136.61504963205));
#225047=CARTESIAN_POINT('Ctrl Pts',(-236.354464555605,4.8405857764003,134.020065632043));
#225048=CARTESIAN_POINT('Ctrl Pts',(-236.632912179418,5.32191855220324,
128.470005819654));
#225049=CARTESIAN_POINT('Ctrl Pts',(-236.911359803231,0.912668168706789,
125.065104026974));
#225050=CARTESIAN_POINT('Ctrl Pts',(-237.189807427044,-4.33527967551271,
126.934298662776));
#225051=CARTESIAN_POINT('Ctrl Pts',(-237.468255050857,-5.59931728812211,
132.359891171993));
#225052=CARTESIAN_POINT('Ctrl Pts',(-237.74670267467,-1.71785585480426,
136.356027093583));
#225053=CARTESIAN_POINT('Ctrl Pts',(-238.025150298482,3.7422311871549,135.250452737698));
#225054=CARTESIAN_POINT('Ctrl Pts',(-238.303597922296,5.76339058627568,
130.059136927086));
#225055=CARTESIAN_POINT('Ctrl Pts',(-238.582045546108,2.48827559389159,
125.552645281824));
#225056=CARTESIAN_POINT('Ctrl Pts',(-238.860493169922,-3.07344311025789,
125.87222346955));
#225057=CARTESIAN_POINT('Ctrl Pts',(-239.138940793734,-5.81081774212379,
130.724194748009));
#225058=CARTESIAN_POINT('Ctrl Pts',(-239.417388417547,-3.20833474320591,
135.649834544268));
#225059=CARTESIAN_POINT('Ctrl Pts',(-239.69583604136,2.34245114885216,136.12272051645));
#225060=CARTESIAN_POINT('Ctrl Pts',(-239.974283665173,5.7406388702159,131.708293557882));
#225061=CARTESIAN_POINT('Ctrl Pts',(-240.252731288985,3.86345991565072,
126.463196386742));
#225062=CARTESIAN_POINT('Ctrl Pts',(-240.531178912799,-1.56404996088748,
125.207417066067));
#225063=CARTESIAN_POINT('Ctrl Pts',(-240.809626536611,-5.5542743314588,
129.094955443325));
#225064=CARTESIAN_POINT('Ctrl Pts',(-241.088074160425,-4.44039193280503,
134.553353666625));
#225065=CARTESIAN_POINT('Ctrl Pts',(-241.366521784237,0.753993726891117,
136.566610426332));
#225066=CARTESIAN_POINT('Ctrl Pts',(-241.64496940805,5.25549598621542,133.284641113335));
#225067=CARTESIAN_POINT('Ctrl Pts',(-241.923417031863,4.92745417946037,
127.723415193164));
#225068=CARTESIAN_POINT('Ctrl Pts',(-242.201864655676,0.071322701300089,
124.993427605467));
#225069=CARTESIAN_POINT('Ctrl Pts',(-242.480312279489,-4.85035085504701,
127.603403576029));
#225070=CARTESIAN_POINT('Ctrl Pts',(-242.758759903302,-5.31478892841856,
133.154902692318));
#225071=CARTESIAN_POINT('Ctrl Pts',(-243.037207527115,-0.895195618446729,
136.546368472274));
#225072=CARTESIAN_POINT('Ctrl Pts',(-243.315655150928,4.34703873214009,
134.661209546432));
#225073=CARTESIAN_POINT('Ctrl Pts',(-243.59410277474,5.59455685253872,129.231794872506));
#225074=CARTESIAN_POINT('Ctrl Pts',(-243.872550398553,1.7009505347501,125.247491294183));
#225075=CARTESIAN_POINT('Ctrl Pts',(-244.150998022366,-3.75574622842035,
126.36967915589));
#225076=CARTESIAN_POINT('Ctrl Pts',(-244.429445646179,-5.76109568607594,
131.567122634643));
#225077=CARTESIAN_POINT('Ctrl Pts',(-244.707893269992,-2.47227965339868,
136.063625082699));
#225078=CARTESIAN_POINT('Ctrl Pts',(-244.986340893805,3.08844060317656,
135.727120416648));
#225079=CARTESIAN_POINT('Ctrl Pts',(-245.264788517618,5.81103482414375,
130.866839985428));
#225080=CARTESIAN_POINT('Ctrl Pts',(-245.543236141431,3.1935719265564,125.949144067427));
#225081=CARTESIAN_POINT('Ctrl Pts',(-245.821683765243,-2.35862755687492,
125.49315496849));
#225082=CARTESIAN_POINT('Ctrl Pts',(-246.100131389057,-5.74336354089951,
129.917904394232));
#225083=CARTESIAN_POINT('Ctrl Pts',(-246.378579012869,-3.85022900974501,
135.157263783424));
#225084=CARTESIAN_POINT('Ctrl Pts',(-246.657026636682,1.58107788722132,
136.396517814333));
#225085=CARTESIAN_POINT('Ctrl Pts',(-246.935474260495,5.55945144577998,
132.496852573479));
#225086=CARTESIAN_POINT('Ctrl Pts',(-247.213921884308,4.42896071996899,
127.04186990797));
#225087=CARTESIAN_POINT('Ctrl Pts',(-247.492369508121,-0.77152854073377,
125.044432396689));
#225088=CARTESIAN_POINT('Ctrl Pts',(-247.770817131934,-5.26302076376676,
128.340087532256));
#225089=CARTESIAN_POINT('Ctrl Pts',(-248.049264755747,-4.91805401775627,
133.90028924679));
#225090=CARTESIAN_POINT('Ctrl Pts',(-248.32771237956,-0.0536358897235281,
136.615483795589));
#225091=CARTESIAN_POINT('Ctrl Pts',(-248.606160003372,4.86007100070672,
133.990540032933));
#225092=CARTESIAN_POINT('Ctrl Pts',(-248.884607627186,5.30761006915461,
128.437653041073));
#225093=CARTESIAN_POINT('Ctrl Pts',(-249.163055250998,0.877714775216597,
125.059654691916));
#225094=CARTESIAN_POINT('Ctrl Pts',(-249.441502874812,-4.35875751839529,
126.960760443945));
#225095=CARTESIAN_POINT('Ctrl Pts',(-249.719950498624,-5.58974458974414,
132.393946985223));
#225096=CARTESIAN_POINT('Ctrl Pts',(-249.998398122437,-1.68402945732324,
136.366381310236));
#225097=CARTESIAN_POINT('Ctrl Pts',(-250.27684574625,3.76922647696617,135.227590338499));
#225098=CARTESIAN_POINT('Ctrl Pts',(-250.555293370063,5.75874741587205,
130.024067340013));
#225099=CARTESIAN_POINT('Ctrl Pts',(-250.833740993876,2.45626081004631,
125.537595744144));
#225100=CARTESIAN_POINT('Ctrl Pts',(-251.112188617689,-3.10340948520656,
125.891023771197));
#225101=CARTESIAN_POINT('Ctrl Pts',(-251.390636241501,-5.81119807352532,
130.759568330183));
#225102=CARTESIAN_POINT('Ctrl Pts',(-251.669083865314,-3.17877952510356,
135.669274813107));
#225103=CARTESIAN_POINT('Ctrl Pts',(-251.947531489127,2.37478211491517,
136.10836281449));
#225104=CARTESIAN_POINT('Ctrl Pts',(-252.22597911294,5.74603500580729,131.673331912019));
#225105=CARTESIAN_POINT('Ctrl Pts',(-252.504426736753,3.83696243592119,
126.439758841162));
#225106=CARTESIAN_POINT('Ctrl Pts',(-252.782874360566,-1.59809116681098,
125.217041580908));
#225107=CARTESIAN_POINT('Ctrl Pts',(-253.061321984379,-5.5645770578269,
129.128797558239));
#225108=CARTESIAN_POINT('Ctrl Pts',(-253.339769608192,-4.41748847836656,
134.580314133917));
#225109=CARTESIAN_POINT('Ctrl Pts',(-253.618217232004,0.789056208225191,
136.561913888683));
#225110=CARTESIAN_POINT('Ctrl Pts',(-253.896664855818,5.27049678355612,
133.252603468789));
#225111=CARTESIAN_POINT('Ctrl Pts',(-254.17511247963,4.90860829937749,127.693477454216));
#225112=CARTESIAN_POINT('Ctrl Pts',(-254.453560103444,0.0359485746511809,
124.993101125124));
#225113=CARTESIAN_POINT('Ctrl Pts',(-254.732007727256,-4.86974611083267,
127.632988310607));
#225114=CARTESIAN_POINT('Ctrl Pts',(-255.010455351069,-5.30038206451776,
133.187211835313));
#225115=CARTESIAN_POINT('Ctrl Pts',(-255.288902974882,-0.860225756393269,
136.55171127444));
#225116=CARTESIAN_POINT('Ctrl Pts',(-255.567350598695,4.37043584157037,
134.634676658854));
#225117=CARTESIAN_POINT('Ctrl Pts',(-255.845798222508,5.58488070320316,
129.197767919676));
#225118=CARTESIAN_POINT('Ctrl Pts',(-256.12424584632,1.66709247927321,125.23724089965));
#225119=CARTESIAN_POINT('Ctrl Pts',(-256.402693470134,-3.78267124144458,
126.39262206856));
#225120=CARTESIAN_POINT('Ctrl Pts',(-256.681141093946,-5.75634686702621,
131.602180844355));
#225121=CARTESIAN_POINT('Ctrl Pts',(-256.95958871776,-2.44021719259262,
136.078571600242));
#225122=CARTESIAN_POINT('Ctrl Pts',(-257.238036341572,3.118345804191,135.708239395799));
#225123=CARTESIAN_POINT('Ctrl Pts',(-257.516483965385,5.81131468939531,
130.8314457702));
#225124=CARTESIAN_POINT('Ctrl Pts',(-257.794931589198,3.16394407961038,
125.929830927563));
#225125=CARTESIAN_POINT('Ctrl Pts',(-258.073379213011,-2.39088900078744,
125.507540987923));
#225126=CARTESIAN_POINT('Ctrl Pts',(-258.351826836824,-5.74870171518396,
129.953014515613));
#225127=CARTESIAN_POINT('Ctrl Pts',(-258.630274460636,-3.82356878618261,
135.180370918811));
#225128=CARTESIAN_POINT('Ctrl Pts',(-258.908722084449,1.61491681105698,
136.387261181902));
#225129=CARTESIAN_POINT('Ctrl Pts',(-259.187169708263,5.56997747689423,
132.462088635074));
#225130=CARTESIAN_POINT('Ctrl Pts',(-259.465617332075,4.40535894966821,
127.016664495574));
#225131=CARTESIAN_POINT('Ctrl Pts',(-259.744064955888,-0.805411631290512,
125.046024618449));
#225132=CARTESIAN_POINT('Ctrl Pts',(-260.022512579701,-5.28013240410161,
128.378470706602));
#225133=CARTESIAN_POINT('Ctrl Pts',(-260.254552266212,-4.95911089365773,
132.993351965875));
#225134=CARTESIAN_POINT('Ctrl Pts',(-260.440213228287,-2.45877638613931,
135.28779596926));
#225135=CARTESIAN_POINT('Ctrl Pts',(-260.53305831576,-0.833059752290926,
135.715219187214));
#225136=CARTESIAN_POINT('Ctrl Pts',(-260.579495465929,-0.013892627260139,
135.717527172907));
#225137=CARTESIAN_POINT('',(177.785583446829,-5.06713383344665,133.858953737923));
#225138=CARTESIAN_POINT('',(177.476367722506,-5.12057379406247,130.804360617566));
#225139=CARTESIAN_POINT('Ctrl Pts',(177.783358963677,-5.06757454116058,
133.84805929277));
#225140=CARTESIAN_POINT('Ctrl Pts',(177.741301979325,-5.0865756231635,133.64169093706));
#225141=CARTESIAN_POINT('Ctrl Pts',(177.703514081134,-5.10373431764903,
133.434432378098));
#225142=CARTESIAN_POINT('Ctrl Pts',(177.627192311405,-5.13661944562339,
132.960177896229));
#225143=CARTESIAN_POINT('Ctrl Pts',(177.591437451862,-5.1506006863121,132.693106637366));
#225144=CARTESIAN_POINT('Ctrl Pts',(177.518755771383,-5.17068200829881,
132.013332647003));
#225145=CARTESIAN_POINT('Ctrl Pts',(177.491556503003,-5.1685893640333,131.600259531465));
#225146=CARTESIAN_POINT('Ctrl Pts',(177.477967247678,-5.13994992058266,
131.059495215027));
#225147=CARTESIAN_POINT('Ctrl Pts',(177.476367722506,-5.13129070204266,
130.931828234693));
#225148=CARTESIAN_POINT('Ctrl Pts',(177.476367722506,-5.12057379406246,
130.804360617566));
#225149=CARTESIAN_POINT('',(177.936624807795,-5.91674751037323,130.798932819469));
#225150=CARTESIAN_POINT('Ctrl Pts',(177.785647847033,-5.06709630945435,
133.859269053708));
#225151=CARTESIAN_POINT('Ctrl Pts',(177.79294899737,-5.14728668343649,133.72625938859));
#225152=CARTESIAN_POINT('Ctrl Pts',(177.800250147706,-5.22230291617104,
133.589979284485));
#225153=CARTESIAN_POINT('Ctrl Pts',(177.807551298043,-5.29186881662205,
133.450878138793));
#225154=CARTESIAN_POINT('Ctrl Pts',(177.814849277387,-5.36140450361573,
133.311837406702));
#225155=CARTESIAN_POINT('Ctrl Pts',(177.82214725673,-5.42549439663099,133.169978413749));
#225156=CARTESIAN_POINT('Ctrl Pts',(177.829445236074,-5.48390773829624,
133.025776040299));
#225157=CARTESIAN_POINT('Ctrl Pts',(177.836741578552,-5.5423079784222,132.881606010025));
#225158=CARTESIAN_POINT('Ctrl Pts',(177.844037921031,-5.59503405761397,
132.735094001483));
#225159=CARTESIAN_POINT('Ctrl Pts',(177.851334263509,-5.64190307126974,
132.586735521142));
#225160=CARTESIAN_POINT('Ctrl Pts',(177.858632982365,-5.68878734989527,
132.438328721292));
#225161=CARTESIAN_POINT('Ctrl Pts',(177.86593170122,-5.72981062989802,132.288074613004));
#225162=CARTESIAN_POINT('Ctrl Pts',(177.873230420075,-5.76483961792187,
132.136484764235));
#225163=CARTESIAN_POINT('Ctrl Pts',(177.880530161697,-5.79987351453996,
131.984873673257));
#225164=CARTESIAN_POINT('Ctrl Pts',(177.887829903318,-5.82891136813785,
131.831926845543));
#225165=CARTESIAN_POINT('Ctrl Pts',(177.895129644939,-5.85187103627661,
131.678166052023));
#225166=CARTESIAN_POINT('Ctrl Pts',(177.902435936344,-5.87485130526188,
131.524267294728));
#225167=CARTESIAN_POINT('Ctrl Pts',(177.909742227748,-5.89174244466227,
131.369553494223));
#225168=CARTESIAN_POINT('Ctrl Pts',(177.917048519153,-5.90251416797608,
131.21455210863));
#225169=CARTESIAN_POINT('Ctrl Pts',(177.9235739487,-5.91213466046586,131.076116537779));
#225170=CARTESIAN_POINT('Ctrl Pts',(177.930099378248,-5.9168745824033,130.937451810787));
#225171=CARTESIAN_POINT('Ctrl Pts',(177.936624807795,-5.91674751037323,
130.798932819469));
#225172=CARTESIAN_POINT('',(178.183682610571,-3.73058779372404,126.219102738339));
#225173=CARTESIAN_POINT('Ctrl Pts',(177.936624807795,-5.91746116842021,
130.798932164786));
#225174=CARTESIAN_POINT('Ctrl Pts',(177.957120624423,-5.9215064818599,130.363799294495));
#225175=CARTESIAN_POINT('Ctrl Pts',(178.039473225349,-5.74509580593375,
128.618678131439));
#225176=CARTESIAN_POINT('Ctrl Pts',(178.121825826274,-4.74534417957617,
127.058332616678));
#225177=CARTESIAN_POINT('Ctrl Pts',(178.183682610571,-3.73058779372456,
126.219102738339));
#225178=CARTESIAN_POINT('Ctrl Pts',(177.476367722506,-5.12057379406248,
130.804360617566));
#225179=CARTESIAN_POINT('Ctrl Pts',(177.476367722506,-5.10013257136415,
130.561231353665));
#225180=CARTESIAN_POINT('Ctrl Pts',(177.482192124778,-5.07221048657026,
130.318826954245));
#225181=CARTESIAN_POINT('Ctrl Pts',(177.495566578132,-5.02964518562034,
130.038571223779));
#225182=CARTESIAN_POINT('Ctrl Pts',(177.497588701151,-5.0234574971161,129.999383302672));
#225183=CARTESIAN_POINT('Ctrl Pts',(177.499824837013,-5.01684285690672,
129.959067960444));
#225184=CARTESIAN_POINT('Ctrl Pts',(177.499890045632,-5.01665015058729,
129.957894766361));
#225185=CARTESIAN_POINT('Ctrl Pts',(177.499971960186,-5.01640830578995,
129.956424078135));
#225186=CARTESIAN_POINT('Ctrl Pts',(177.499988541006,-5.01635936437147,
129.956126544398));
#225187=CARTESIAN_POINT('Ctrl Pts',(177.500014499698,-5.01628276091504,
129.95566097563));
#225188=CARTESIAN_POINT('Ctrl Pts',(177.500023871669,-5.01625510823518,
129.955492939538));
#225189=CARTESIAN_POINT('Ctrl Pts',(177.500041185287,-5.0162040301161,129.955182604992));
#225190=CARTESIAN_POINT('Ctrl Pts',(177.500049126247,-5.01618060563769,
129.955040304703));
#225191=CARTESIAN_POINT('Ctrl Pts',(177.500066566138,-5.01612916686506,
129.954727864379));
#225192=CARTESIAN_POINT('Ctrl Pts',(177.500076065797,-5.01610115158613,
129.95455772672));
#225193=CARTESIAN_POINT('Ctrl Pts',(177.500102731179,-5.01602252400973,
129.954080297032));
#225194=CARTESIAN_POINT('Ctrl Pts',(177.500119903333,-5.01597190148107,
129.953773005773));
#225195=CARTESIAN_POINT('Ctrl Pts',(177.500219182879,-5.01567930376682,
129.951997389358));
#225196=CARTESIAN_POINT('Ctrl Pts',(177.500301490531,-5.01543701294836,
129.950529128138));
#225197=CARTESIAN_POINT('Ctrl Pts',(177.500536651928,-5.01474557825448,
129.946344990489));
#225198=CARTESIAN_POINT('Ctrl Pts',(177.500690012856,-5.01429563401943,
129.94362927491));
#225199=CARTESIAN_POINT('Ctrl Pts',(177.501483934731,-5.01197134589284,
129.929637033759));
#225200=CARTESIAN_POINT('Ctrl Pts',(177.502136129423,-5.0100786087708,129.918364247601));
#225201=CARTESIAN_POINT('Ctrl Pts',(177.507494427648,-4.99465822545836,
129.82749951209));
#225202=CARTESIAN_POINT('Ctrl Pts',(177.512808699789,-4.98015314808467,
129.748006760148));
#225203=CARTESIAN_POINT('Ctrl Pts',(177.536252366813,-4.91867001249372,
129.434266685906));
#225204=CARTESIAN_POINT('Ctrl Pts',(177.559035115434,-4.86392156822592,
129.202282649367));
#225205=CARTESIAN_POINT('Ctrl Pts',(177.641117942126,-4.68015889981346,
128.524160057609));
#225206=CARTESIAN_POINT('Ctrl Pts',(177.714428393931,-4.53033676743336,
128.085641009048));
#225207=CARTESIAN_POINT('Ctrl Pts',(177.860352889966,-4.2591342270638,127.393966784111));
#225208=CARTESIAN_POINT('Ctrl Pts',(177.922457124534,-4.14884818442793,
127.134214134108));
#225209=CARTESIAN_POINT('Ctrl Pts',(178.050554224604,-3.93347667359594,
126.653734659887));
#225210=CARTESIAN_POINT('Ctrl Pts',(178.114950700917,-3.82966817966767,
126.432690898171));
#225211=CARTESIAN_POINT('Ctrl Pts',(178.184070351179,-3.72422348156493,
126.213846503759));
#225212=CARTESIAN_POINT('Origin',(210.,0.,130.804360617566));
#225213=CARTESIAN_POINT('',(178.655995448006,0.643991232007665,124.924876168436));
#225214=CARTESIAN_POINT('Ctrl Pts',(178.656596669642,0.650137269913459,
124.923437892962));
#225215=CARTESIAN_POINT('Ctrl Pts',(178.631192637209,1.19960075686107,124.98418119942));
#225216=CARTESIAN_POINT('Ctrl Pts',(178.571783995707,1.75472463999775,125.12573841184));
#225217=CARTESIAN_POINT('Ctrl Pts',(178.487391008075,2.2825507450488,125.345610175187));
#225218=CARTESIAN_POINT('Ctrl Pts',(178.486208584818,2.28991117210278,125.34869374146));
#225219=CARTESIAN_POINT('Ctrl Pts',(178.485021693585,2.29726490846875,125.351792002425));
#225220=CARTESIAN_POINT('',(179.938376004444,-5.92191450869858,130.805748116515));
#225221=CARTESIAN_POINT('Ctrl Pts',(179.938375192211,-5.91674983355068,
130.805764069745));
#225222=CARTESIAN_POINT('Ctrl Pts',(179.934802337543,-5.91673193815412,
130.881208453364));
#225223=CARTESIAN_POINT('Ctrl Pts',(179.931229482876,-5.91527111751309,
130.956633994371));
#225224=CARTESIAN_POINT('Ctrl Pts',(179.927656628208,-5.91236916926149,
131.032003690964));
#225225=CARTESIAN_POINT('Ctrl Pts',(179.920233361803,-5.90633983502618,
131.18859817597));
#225226=CARTESIAN_POINT('Ctrl Pts',(179.912810095397,-5.89407576518302,
131.345189745836));
#225227=CARTESIAN_POINT('Ctrl Pts',(179.905386828992,-5.87556700792397,
131.501241452354));
#225228=CARTESIAN_POINT('Ctrl Pts',(179.897972336271,-5.85708012647892,
131.657108718716));
#225229=CARTESIAN_POINT('Ctrl Pts',(179.89055784355,-5.83236329248394,131.81243702474));
#225230=CARTESIAN_POINT('Ctrl Pts',(179.883143350829,-5.80145853932096,
131.966689907845));
#225231=CARTESIAN_POINT('Ctrl Pts',(179.875736004475,-5.77058357332259,
132.120794116214));
#225232=CARTESIAN_POINT('Ctrl Pts',(179.868328658121,-5.73353263444466,
132.27382460163));
#225233=CARTESIAN_POINT('Ctrl Pts',(179.860921311767,-5.69039947340868,
132.425250618624));
#225234=CARTESIAN_POINT('Ctrl Pts',(179.853519490092,-5.64729848271151,
132.576563696382));
#225235=CARTESIAN_POINT('Ctrl Pts',(179.846117668417,-5.59812440416739,
132.726274330983));
#225236=CARTESIAN_POINT('Ctrl Pts',(179.838715846741,-5.54302190257774,
132.873862671212));
#225237=CARTESIAN_POINT('Ctrl Pts',(179.83131793243,-5.48794848916994,133.021373100704));
#225238=CARTESIAN_POINT('Ctrl Pts',(179.823920018118,-5.42695301563993,
133.166763118208));
#225239=CARTESIAN_POINT('Ctrl Pts',(179.816522103807,-5.3602297308131,133.309528834554));
#225240=CARTESIAN_POINT('Ctrl Pts',(179.809125418895,-5.2935175341856,133.452270825829));
#225241=CARTESIAN_POINT('Ctrl Pts',(179.801728733983,-5.22107957331895,
133.592389043643));
#225242=CARTESIAN_POINT('Ctrl Pts',(179.79433204907,-5.1431579462292,133.729400258774));
#225243=CARTESIAN_POINT('Ctrl Pts',(179.786935692135,-5.06523977426604,
133.866405398685));
#225244=CARTESIAN_POINT('Ctrl Pts',(179.779539335199,-4.98183860409271,
134.000303485351));
#225245=CARTESIAN_POINT('Ctrl Pts',(179.772142978264,-4.89324200758084,
134.13063679638));
#225246=CARTESIAN_POINT('Ctrl Pts',(179.764745488927,-4.80463184670375,
134.260990061772));
#225247=CARTESIAN_POINT('Ctrl Pts',(179.757347999591,-4.71082488554907,
134.387777156069));
#225248=CARTESIAN_POINT('Ctrl Pts',(179.749950510254,-4.61215135748797,
134.510570328055));
#225249=CARTESIAN_POINT('Ctrl Pts',(179.742550427739,-4.51344323957483,
134.633406544996));
#225250=CARTESIAN_POINT('Ctrl Pts',(179.735150345224,-4.4098653918718,134.752245761303));
#225251=CARTESIAN_POINT('Ctrl Pts',(179.727750262709,-4.30178744852212,
134.866694344654));
#225252=CARTESIAN_POINT('Ctrl Pts',(179.720342043042,-4.19359066236287,
134.981268775988));
#225253=CARTESIAN_POINT('Ctrl Pts',(179.712933823376,-4.08088415489833,
135.091442661055));
#225254=CARTESIAN_POINT('Ctrl Pts',(179.70552560371,-3.96407396764172,135.19685969458));
#225255=CARTESIAN_POINT('Ctrl Pts',(179.698112824407,-3.84719188566385,
135.30234161053));
#225256=CARTESIAN_POINT('Ctrl Pts',(179.690700045105,-3.72620137726176,
135.403060602727));
#225257=CARTESIAN_POINT('Ctrl Pts',(179.683287265803,-3.60154006095042,
135.49870186548));
#225258=CARTESIAN_POINT('Ctrl Pts',(179.675863894774,-3.47670062270434,
135.594479784955));
#225259=CARTESIAN_POINT('Ctrl Pts',(179.668440523746,-3.34818020526591,
135.685165269879));
#225260=CARTESIAN_POINT('Ctrl Pts',(179.661017152717,-3.21644446134536,
135.77048743729));
#225261=CARTESIAN_POINT('Ctrl Pts',(179.657081103276,-3.14659500896289,
135.815727297728));
#225262=CARTESIAN_POINT('Ctrl Pts',(179.653145053835,-3.07584201855703,
135.859460108231));
#225263=CARTESIAN_POINT('Ctrl Pts',(179.649209004394,-3.00425738879533,
135.901650888324));
#225264=CARTESIAN_POINT('Ctrl Pts',(179.641785737989,-2.86925101114459,
135.981221382851));
#225265=CARTESIAN_POINT('Ctrl Pts',(179.634362471584,-2.73087705919654,
136.05554484203));
#225266=CARTESIAN_POINT('Ctrl Pts',(179.626939205178,-2.58958190348824,
136.124322659501));
#225267=CARTESIAN_POINT('Ctrl Pts',(179.619524712457,-2.44845374692,136.193019187303));
#225268=CARTESIAN_POINT('Ctrl Pts',(179.612110219736,-2.30441159141906,
136.256182958357));
#225269=CARTESIAN_POINT('Ctrl Pts',(179.604695727015,-2.15792949821889,
136.313559365407));
#225270=CARTESIAN_POINT('Ctrl Pts',(179.597288380661,-2.01158858997503,
136.370880470916));
#225271=CARTESIAN_POINT('Ctrl Pts',(179.589881034308,-1.86281277106264,
136.422425182046));
#225272=CARTESIAN_POINT('Ctrl Pts',(179.582473687954,-1.71209924723198,
136.467985493044));
#225273=CARTESIAN_POINT('Ctrl Pts',(179.575071866278,-1.5614981312336,136.513511823442));
#225274=CARTESIAN_POINT('Ctrl Pts',(179.567670044603,-1.40896254372182,
136.553062533368));
#225275=CARTESIAN_POINT('Ctrl Pts',(179.560268222928,-1.25500804510559,
136.586478341136));
#225276=CARTESIAN_POINT('Ctrl Pts',(179.552870308616,-1.10113481787052,
136.619876508959));
#225277=CARTESIAN_POINT('Ctrl Pts',(179.545472394305,-0.945844535144645,
136.647146145406));
#225278=CARTESIAN_POINT('Ctrl Pts',(179.538074479993,-0.789666129390942,
136.668178313112));
#225279=CARTESIAN_POINT('Ctrl Pts',(179.530677795081,-0.633513677655301,
136.689206985652));
#225280=CARTESIAN_POINT('Ctrl Pts',(179.523281110169,-0.476473765410261,
136.704000196932));
#225281=CARTESIAN_POINT('Ctrl Pts',(179.515884425257,-0.319083806977362,
136.712500433669));
#225282=CARTESIAN_POINT('Ctrl Pts',(179.508488068321,-0.161700827380124,
136.721000293498));
#225283=CARTESIAN_POINT('Ctrl Pts',(179.501091711386,-0.0039682052111765,
136.723207713473));
#225284=CARTESIAN_POINT('Ctrl Pts',(179.493695354451,0.153573525095219,
136.71911722582));
#225285=CARTESIAN_POINT('Ctrl Pts',(179.486297865114,0.311139375442765,
136.715026111904));
#225286=CARTESIAN_POINT('Ctrl Pts',(179.478900375777,0.468513902538733,
136.704635180148));
#225287=CARTESIAN_POINT('Ctrl Pts',(179.471502886441,0.625158727965406,
136.687991055259));
#225288=CARTESIAN_POINT('Ctrl Pts',(179.464102803926,0.781858464992578,
136.671341095798));
#225289=CARTESIAN_POINT('Ctrl Pts',(179.456702721411,0.937827620086148,
136.648433618271));
#225290=CARTESIAN_POINT('Ctrl Pts',(179.449302638896,1.09253522294258,136.619366838468));
#225291=CARTESIAN_POINT('Ctrl Pts',(179.44189441923,1.24741294271294,136.590268096752));
#225292=CARTESIAN_POINT('Ctrl Pts',(179.434486199563,1.40102597280012,136.554996596033));
#225293=CARTESIAN_POINT('Ctrl Pts',(179.427077979897,1.55285506812971,136.513701358832));
#225294=CARTESIAN_POINT('Ctrl Pts',(179.419665200595,1.70477761173422,136.472380705102));
#225295=CARTESIAN_POINT('Ctrl Pts',(179.412252421292,1.85491367752859,136.425029039235));
#225296=CARTESIAN_POINT('Ctrl Pts',(179.40483964199,2.0027618670726,136.371844381916));
#225297=CARTESIAN_POINT('Ctrl Pts',(179.397416270962,2.15082130904315,136.318583731865));
#225298=CARTESIAN_POINT('Ctrl Pts',(179.389992899933,2.29658600076753,136.259473584504));
#225299=CARTESIAN_POINT('Ctrl Pts',(179.382569528904,2.43957634407283,136.194759287789));
#225300=CARTESIAN_POINT('Ctrl Pts',(179.378633479463,2.51539325509978,136.160446214872));
#225301=CARTESIAN_POINT('Ctrl Pts',(179.374697430023,2.59043062670582,136.124558372525));
#225302=CARTESIAN_POINT('Ctrl Pts',(179.370761380582,2.66462016584161,136.087137343332));
#225303=CARTESIAN_POINT('Ctrl Pts',(179.363338114176,2.80453932127499,136.016562450144));
#225304=CARTESIAN_POINT('Ctrl Pts',(179.355914847771,2.94186425343108,135.940318170553));
#225305=CARTESIAN_POINT('Ctrl Pts',(179.348491581365,3.07610246214482,135.858618644704));
#225306=CARTESIAN_POINT('Ctrl Pts',(179.341077088644,3.21018201244378,135.777015680909));
#225307=CARTESIAN_POINT('Ctrl Pts',(179.333662595923,3.3411817853958,135.689970497116));
#225308=CARTESIAN_POINT('Ctrl Pts',(179.326248103202,3.46863133103027,135.597744313025));
#225309=CARTESIAN_POINT('Ctrl Pts',(179.318840756849,3.59595803599425,135.505607020003));
#225310=CARTESIAN_POINT('Ctrl Pts',(179.311433410495,3.71974102546335,135.408298885418));
#225311=CARTESIAN_POINT('Ctrl Pts',(179.304026064141,3.83953654645319,135.306125790357));
#225312=CARTESIAN_POINT('Ctrl Pts',(179.296624242466,3.95924271942392,135.204028899845));
#225313=CARTESIAN_POINT('Ctrl Pts',(179.28922242079,4.07496706275787,135.097074514833));
#225314=CARTESIAN_POINT('Ctrl Pts',(179.281820599115,4.18629689526787,134.985610295255));
#225315=CARTESIAN_POINT('Ctrl Pts',(179.274422684804,4.29756795762586,134.87420491677));
#225316=CARTESIAN_POINT('Ctrl Pts',(179.267024770492,4.40444886607418,134.758294708461));
#225317=CARTESIAN_POINT('Ctrl Pts',(179.259626856181,4.50656206760595,134.638265792882));
#225318=CARTESIAN_POINT('Ctrl Pts',(179.252230171269,4.6086582997761,134.518256823932));
#225319=CARTESIAN_POINT('Ctrl Pts',(179.244833486356,4.70598815587262,134.394130790199));
#225320=CARTESIAN_POINT('Ctrl Pts',(179.237436801444,4.79821276277581,134.266308746241));
#225321=CARTESIAN_POINT('Ctrl Pts',(179.230040444509,4.89043328034328,134.138492370046));
#225322=CARTESIAN_POINT('Ctrl Pts',(179.222644087573,4.97754878040159,134.006980612211));
#225323=CARTESIAN_POINT('Ctrl Pts',(179.215247730638,5.05926249069234,133.872225284199));
#225324=CARTESIAN_POINT('Ctrl Pts',(179.207850241301,5.14098871156078,133.737449324802));
#225325=CARTESIAN_POINT('Ctrl Pts',(179.200452751965,5.21731130237002,133.599429125651));
#225326=CARTESIAN_POINT('Ctrl Pts',(179.193055262628,5.28797848312044,133.45864284155));
#225327=CARTESIAN_POINT('Ctrl Pts',(179.185655180113,5.3586704361415,133.317807205035));
#225328=CARTESIAN_POINT('Ctrl Pts',(179.178255097598,5.42370286461153,133.174203886429));
#225329=CARTESIAN_POINT('Ctrl Pts',(179.170855015083,5.4828713978363,133.028332694119));
#225330=CARTESIAN_POINT('Ctrl Pts',(179.163446795416,5.54210499294605,132.882301101438));
#225331=CARTESIAN_POINT('Ctrl Pts',(179.15603857575,5.59546167541947,132.733997000985));
#225332=CARTESIAN_POINT('Ctrl Pts',(179.148630356084,5.64278615747782,132.583937798662));
#225333=CARTESIAN_POINT('Ctrl Pts',(179.141217576781,5.69013976696525,132.433786237403));
#225334=CARTESIAN_POINT('Ctrl Pts',(179.133804797479,5.73145368024142,132.281877781146));
#225335=CARTESIAN_POINT('Ctrl Pts',(179.126392018177,5.76662347961273,132.128741305616));
#225336=CARTESIAN_POINT('Ctrl Pts',(179.118968647149,5.80184353124267,131.975386021508));
#225337=CARTESIAN_POINT('Ctrl Pts',(179.11154527612,5.83090186655938,131.820799579596));
#225338=CARTESIAN_POINT('Ctrl Pts',(179.104121905091,5.85374566921849,131.665518095967));
#225339=CARTESIAN_POINT('Ctrl Pts',(179.10018585565,5.86585800151788,131.583184127419));
#225340=CARTESIAN_POINT('Ctrl Pts',(179.096249806209,5.87622407559727,131.50065480612));
#225341=CARTESIAN_POINT('Ctrl Pts',(179.092313756769,5.88484196200156,131.41801006535));
#225342=CARTESIAN_POINT('Ctrl Pts',(179.084890490363,5.90109502680501,131.262144663512));
#225343=CARTESIAN_POINT('Ctrl Pts',(179.077467223958,5.91117603521354,131.105397413357));
#225344=CARTESIAN_POINT('Ctrl Pts',(179.070043957552,5.91499894102585,130.948298417199));
#225345=CARTESIAN_POINT('Ctrl Pts',(179.062629464831,5.91881732848096,130.791385099008));
#225346=CARTESIAN_POINT('Ctrl Pts',(179.05521497211,5.91639232723587,130.63412123188));
#225347=CARTESIAN_POINT('Ctrl Pts',(179.047800479389,5.90768941912305,130.477043814329));
#225348=CARTESIAN_POINT('Ctrl Pts',(179.040393133036,5.89899489920073,130.320117793906));
#225349=CARTESIAN_POINT('Ctrl Pts',(179.032985786682,5.88403453903981,130.163378235523));
#225350=CARTESIAN_POINT('Ctrl Pts',(179.025578440328,5.8628258257359,130.007363817331));
#225351=CARTESIAN_POINT('Ctrl Pts',(179.018176618653,5.84163293069053,129.851465760579));
#225352=CARTESIAN_POINT('Ctrl Pts',(179.010774796977,5.81420101177123,129.696292135444));
#225353=CARTESIAN_POINT('Ctrl Pts',(179.003372975302,5.78059950086301,129.542378060982));
#225354=CARTESIAN_POINT('Ctrl Pts',(178.99597506099,5.74701572793086,129.388545236562));
#225355=CARTESIAN_POINT('Ctrl Pts',(178.988577146679,5.70726892866063,129.235971002404));
#225356=CARTESIAN_POINT('Ctrl Pts',(178.981179232368,5.66147988227038,129.08518171322));
#225357=CARTESIAN_POINT('Ctrl Pts',(178.973782547456,5.61569844518896,128.93441748248));
#225358=CARTESIAN_POINT('Ctrl Pts',(178.966385862543,5.56387686221214,128.785437964842));
#225359=CARTESIAN_POINT('Ctrl Pts',(178.958989177631,5.5061862092642,128.638755854132));
#225360=CARTESIAN_POINT('Ctrl Pts',(178.951592820696,5.44849811438028,128.49208024746));
#225361=CARTESIAN_POINT('Ctrl Pts',(178.94419646376,5.38494160360329,128.347702192559));
#225362=CARTESIAN_POINT('Ctrl Pts',(178.936800106825,5.31573638605803,128.206115587466));
#225363=CARTESIAN_POINT('Ctrl Pts',(178.929402617488,5.24652057301731,128.064507305103));
#225364=CARTESIAN_POINT('Ctrl Pts',(178.922005128152,5.17165449515218,127.925691658915));
#225365=CARTESIAN_POINT('Ctrl Pts',(178.914607638815,5.09140434440064,127.790138932899));
#225366=CARTESIAN_POINT('Ctrl Pts',(178.9072075563,5.01112606208312,127.654538689084));
#225367=CARTESIAN_POINT('Ctrl Pts',(178.899807473785,4.9254601391764,127.522203963786));
#225368=CARTESIAN_POINT('Ctrl Pts',(178.89240739127,4.8347166112795,127.393576858499));
#225369=CARTESIAN_POINT('Ctrl Pts',(178.884999171604,4.743873301545,127.264808314486));
#225370=CARTESIAN_POINT('Ctrl Pts',(178.877590951937,4.64794145183068,127.139755837558));
#225371=CARTESIAN_POINT('Ctrl Pts',(178.870182732271,4.54727243353588,127.018829746248));
#225372=CARTESIAN_POINT('Ctrl Pts',(178.862769952969,4.44654145513995,126.897829226946));
#225373=CARTESIAN_POINT('Ctrl Pts',(178.855357173667,4.34106774789423,126.780960430458));
#225374=CARTESIAN_POINT('Ctrl Pts',(178.847944394365,4.23123982961107,126.668597076596));
#225375=CARTESIAN_POINT('Ctrl Pts',(178.840521023336,4.12125498404791,126.556073172705));
#225376=CARTESIAN_POINT('Ctrl Pts',(178.833097652307,4.00690377237975,126.448067824391));
#225377=CARTESIAN_POINT('Ctrl Pts',(178.825674281278,3.88860869573101,126.344915251381));
#225378=CARTESIAN_POINT('Ctrl Pts',(178.821738231838,3.82588580763872,126.290221282058));
#225379=CARTESIAN_POINT('Ctrl Pts',(178.817802182397,3.76205466852198,126.236890896299));
#225380=CARTESIAN_POINT('Ctrl Pts',(178.813866132956,3.69718148559496,126.184968923298));
#225381=CARTESIAN_POINT('Ctrl Pts',(178.806443476583,3.57484274165308,126.087053749827));
#225382=CARTESIAN_POINT('Ctrl Pts',(178.79902082021,3.448426597239,125.993853866056));
#225383=CARTESIAN_POINT('Ctrl Pts',(178.791598163837,3.31833243238178,125.905728111376));
#225384=CARTESIAN_POINT('Ctrl Pts',(178.784183856821,3.18838460363009,125.817701484737));
#225385=CARTESIAN_POINT('Ctrl Pts',(178.776769549805,3.05476729371877,125.734737835851));
#225386=CARTESIAN_POINT('Ctrl Pts',(178.769355242789,2.91791360112221,125.657156446476));
#225387=CARTESIAN_POINT('Ctrl Pts',(178.76194781101,2.78118681203899,125.579646997804));
#225388=CARTESIAN_POINT('Ctrl Pts',(178.754540379231,2.641229936335,125.507510057233));
#225389=CARTESIAN_POINT('Ctrl Pts',(178.747132947452,2.49850564450236,125.44102209507));
#225390=CARTESIAN_POINT('Ctrl Pts',(178.739588257635,2.35313670375903,125.373302125976));
#225391=CARTESIAN_POINT('Ctrl Pts',(178.732043567817,2.20489709196751,125.311442779602));
#225392=CARTESIAN_POINT('Ctrl Pts',(178.724498878,2.05430357548496,125.255688039169));
#225393=CARTESIAN_POINT('Ctrl Pts',(178.717100998755,1.90664042737168,125.201018218802));
#225394=CARTESIAN_POINT('Ctrl Pts',(178.70970311951,1.7567145097062,125.152217743023));
#225395=CARTESIAN_POINT('Ctrl Pts',(178.702305240265,1.60503429277867,125.109468565779));
#225396=CARTESIAN_POINT('Ctrl Pts',(178.694687145161,1.44883894547903,125.065446855357));
#225397=CARTESIAN_POINT('Ctrl Pts',(178.687069050057,1.29078361105623,125.027842463903));
#225398=CARTESIAN_POINT('Ctrl Pts',(178.679450954953,1.13144104857084,124.996799019433));
#225399=CARTESIAN_POINT('Ctrl Pts',(178.67183285985,0.972098486085417,124.965755574963));
#225400=CARTESIAN_POINT('Ctrl Pts',(178.664214764746,0.811469119563494,
124.94127316358));
#225401=CARTESIAN_POINT('Ctrl Pts',(178.656596669642,0.650137269913457,
124.923437892962));
#225402=CARTESIAN_POINT('',(181.688375192211,-5.9116597264178,130.809147953816));
#225403=CARTESIAN_POINT('Ctrl Pts',(181.688375192211,-5.9116597264178,130.809147953816));
#225404=CARTESIAN_POINT('Ctrl Pts',(181.658364251836,-5.91648848400863,
131.447879361033));
#225405=CARTESIAN_POINT('Ctrl Pts',(181.535537436858,-5.52634643860716,
134.05629721562));
#225406=CARTESIAN_POINT('Ctrl Pts',(181.31989474727,-1.71655817300176,137.588974723689));
#225407=CARTESIAN_POINT('Ctrl Pts',(181.041447123461,4.78024637596874,135.91579927174));
#225408=CARTESIAN_POINT('Ctrl Pts',(180.762999499646,6.88423803344246,129.54546140426));
#225409=CARTESIAN_POINT('Ctrl Pts',(180.484551875834,2.66195125190711,124.331990413167));
#225410=CARTESIAN_POINT('Ctrl Pts',(180.209677598402,-3.92096128402385,
125.056887831312));
#225411=CARTESIAN_POINT('Ctrl Pts',(180.027619195576,-5.92009025890988,
128.918301208267));
#225412=CARTESIAN_POINT('Ctrl Pts',(179.938376667353,-5.92612969673344,
130.805735096168));
#225413=CARTESIAN_POINT('',(183.438375192211,-5.90878783959383,130.801050019915));
#225414=CARTESIAN_POINT('Ctrl Pts',(183.438375192211,-5.90878783959383,
130.801050019915));
#225415=CARTESIAN_POINT('Ctrl Pts',(183.381926166128,-5.90269714734493,
132.003937776489));
#225416=CARTESIAN_POINT('Ctrl Pts',(183.232661265441,-4.96014564476939,
135.193432897632));
#225417=CARTESIAN_POINT('Ctrl Pts',(182.99058049015,0.258615936756311,137.79797758789));
#225418=CARTESIAN_POINT('Ctrl Pts',(182.712132866336,6.02371625752071,134.36700050664));
#225419=CARTESIAN_POINT('Ctrl Pts',(182.433685242524,6.2533156125226,127.662131411966));
#225420=CARTESIAN_POINT('Ctrl Pts',(182.155237618711,0.736423411067356,
123.844817450807));
#225421=CARTESIAN_POINT('Ctrl Pts',(181.906800935273,-4.78965977321783,
126.145110250613));
#225422=CARTESIAN_POINT('Ctrl Pts',(181.75118012644,-5.90155441818334,129.472452618097));
#225423=CARTESIAN_POINT('Ctrl Pts',(181.688375192211,-5.9116597264178,130.809147953816));
#225424=CARTESIAN_POINT('',(185.188375192211,-5.92379981193959,130.800775453898));
#225425=CARTESIAN_POINT('Ctrl Pts',(185.188375192211,-5.92379981193959,
130.800775453898));
#225426=CARTESIAN_POINT('Ctrl Pts',(185.105488080421,-5.9112852874943,132.555621405934));
#225427=CARTESIAN_POINT('Ctrl Pts',(184.929785094025,-4.15424292220225,
136.29728126716));
#225428=CARTESIAN_POINT('Ctrl Pts',(184.661266233027,2.21295931186131,137.443665672644));
#225429=CARTESIAN_POINT('Ctrl Pts',(184.382818609213,6.78199394032505,132.531241830544));
#225430=CARTESIAN_POINT('Ctrl Pts',(184.104370985402,5.11870745645332,126.031898516554));
#225431=CARTESIAN_POINT('Ctrl Pts',(183.825923361588,-1.24842111713792,
123.918214725658));
#225432=CARTESIAN_POINT('Ctrl Pts',(183.603924763859,-5.41009564609318,
127.278197857111));
#225433=CARTESIAN_POINT('Ctrl Pts',(183.474742040733,-5.91271172097454,
130.026098884935));
#225434=CARTESIAN_POINT('Ctrl Pts',(183.438375192211,-5.90878783959383,
130.801050019915));
#225435=CARTESIAN_POINT('',(186.938375192211,-5.91753456722523,130.809401790279));
#225436=CARTESIAN_POINT('Ctrl Pts',(186.938375192211,-5.9200304115163,130.809403916499));
#225437=CARTESIAN_POINT('Ctrl Pts',(186.921865869317,-5.92320279675294,
131.159511089235));
#225438=CARTESIAN_POINT('Ctrl Pts',(186.812540671824,-5.73530460751272,
133.474529816069));
#225439=CARTESIAN_POINT('Ctrl Pts',(186.610399599713,-2.68163859043372,
137.268598778454));
#225440=CARTESIAN_POINT('Ctrl Pts',(186.331951975907,3.98905548069682,136.554577735401));
#225441=CARTESIAN_POINT('Ctrl Pts',(186.05350435209,6.99400244126163,130.556388074787));
#225442=CARTESIAN_POINT('Ctrl Pts',(185.775056728279,3.57180283432081,124.78607306685));
#225443=CARTESIAN_POINT('Ctrl Pts',(185.496609104465,-3.13270908509169,
124.546270308331));
#225444=CARTESIAN_POINT('Ctrl Pts',(185.301048592443,-5.81959460894973,
128.416832856216));
#225445=CARTESIAN_POINT('Ctrl Pts',(185.198303955025,-5.92529888389735,
130.590568476525));
#225446=CARTESIAN_POINT('Ctrl Pts',(185.188375192211,-5.92379981193959,
130.800775453898));
#225447=CARTESIAN_POINT('',(188.688375158851,-5.91280930184219,130.805575254198));
#225448=CARTESIAN_POINT('Ctrl Pts',(188.688375135582,-5.9167498750567,130.805576560215));
#225449=CARTESIAN_POINT('Ctrl Pts',(188.680495520896,-5.916715288546,130.97387375165));
#225450=CARTESIAN_POINT('Ctrl Pts',(188.67261590621,-5.90949584186738,131.141986835927));
#225451=CARTESIAN_POINT('Ctrl Pts',(188.664736291524,-5.89516395080611,
131.309308689764));
#225452=CARTESIAN_POINT('Ctrl Pts',(188.656841930411,-5.88080523810475,
131.476943680682));
#225453=CARTESIAN_POINT('Ctrl Pts',(188.648947569298,-5.85930751799326,
131.643784192002));
#225454=CARTESIAN_POINT('Ctrl Pts',(188.641053208185,-5.83079446595158,
131.809231981636));
#225455=CARTESIAN_POINT('Ctrl Pts',(188.633135901846,-5.80219853976692,
131.975160650825));
#225456=CARTESIAN_POINT('Ctrl Pts',(188.625218595508,-5.76654654061531,
132.139688210389));
#225457=CARTESIAN_POINT('Ctrl Pts',(188.617301289169,-5.72401296888253,
132.30222779945));
#225458=CARTESIAN_POINT('Ctrl Pts',(188.609371641021,-5.68141309414261,
132.465020761625));
#225459=CARTESIAN_POINT('Ctrl Pts',(188.601441992874,-5.63191030844115,
132.625819284766));
#225460=CARTESIAN_POINT('Ctrl Pts',(188.593512344726,-5.5757279961427,132.784054501865));
#225461=CARTESIAN_POINT('Ctrl Pts',(188.585563505692,-5.51940971458834,
132.94267267089));
#225462=CARTESIAN_POINT('Ctrl Pts',(188.577614666658,-5.45637968482179,
133.098714854591));
#225463=CARTESIAN_POINT('Ctrl Pts',(188.569665827625,-5.38690907388433,
133.251632811704));
#225464=CARTESIAN_POINT('Ctrl Pts',(188.566288207219,-5.35738962430293,
133.316610704718));
#225465=CARTESIAN_POINT('Ctrl Pts',(188.562910586813,-5.32670783786975,
133.381024824207));
#225466=CARTESIAN_POINT('Ctrl Pts',(188.559532966408,-5.29488692684622,
133.444834626984));
#225467=CARTESIAN_POINT('Ctrl Pts',(188.552109700002,-5.22495156661437,
133.585074532128));
#225468=CARTESIAN_POINT('Ctrl Pts',(188.544686433597,-5.14933503520301,
133.722746124474));
#225469=CARTESIAN_POINT('Ctrl Pts',(188.537263167192,-5.06824922202705,
133.857355931339));
#225470=CARTESIAN_POINT('Ctrl Pts',(188.529848674471,-4.98725924554844,
133.991806640591));
#225471=CARTESIAN_POINT('Ctrl Pts',(188.52243418175,-4.90081304514209,134.123202450914));
#225472=CARTESIAN_POINT('Ctrl Pts',(188.515019689029,-4.80916968995939,
134.251071724647));
#225473=CARTESIAN_POINT('Ctrl Pts',(188.507612342675,-4.71761466409284,
134.37881775316));
#225474=CARTESIAN_POINT('Ctrl Pts',(188.500204996321,-4.62087267180682,
134.503043710459));
#225475=CARTESIAN_POINT('Ctrl Pts',(188.492797649967,-4.51924756505893,
134.623304451692));
#225476=CARTESIAN_POINT('Ctrl Pts',(188.485395828292,-4.41769825414966,
134.743475497927));
#225477=CARTESIAN_POINT('Ctrl Pts',(188.477994006617,-4.31127332042061,
134.859686932794));
#225478=CARTESIAN_POINT('Ctrl Pts',(188.470592184941,-4.2003185360947,134.971524492174));
#225479=CARTESIAN_POINT('Ctrl Pts',(188.46319427063,-4.08942232393587,135.083303013377));
#225480=CARTESIAN_POINT('Ctrl Pts',(188.455796356319,-3.97400128576268,
135.190711993113));
#225481=CARTESIAN_POINT('Ctrl Pts',(188.448398442007,-3.85443981639646,
135.293372119476));
#225482=CARTESIAN_POINT('Ctrl Pts',(188.441001757095,-3.73489821597734,
135.396015185588));
#225483=CARTESIAN_POINT('Ctrl Pts',(188.433605072183,-3.61121783291183,
135.493910721659));
#225484=CARTESIAN_POINT('Ctrl Pts',(188.426208387271,-3.483818170251,135.586717935786));
#225485=CARTESIAN_POINT('Ctrl Pts',(188.418812030335,-3.35642415662479,
135.679521034743));
#225486=CARTESIAN_POINT('Ctrl Pts',(188.4114156734,-3.22531149304034,135.767236040568));
#225487=CARTESIAN_POINT('Ctrl Pts',(188.404019316464,-3.09093063134526,
135.849564121362));
#225488=CARTESIAN_POINT('Ctrl Pts',(188.396621827128,-2.95652919559707,
135.931904806795));
#225489=CARTESIAN_POINT('Ctrl Pts',(188.389224337791,-2.81885888376706,
136.00885672998));
#225490=CARTESIAN_POINT('Ctrl Pts',(188.381826848455,-2.67839669617966,
136.080165930539));
#225491=CARTESIAN_POINT('Ctrl Pts',(188.37442676594,-2.53788526979019,136.151500128428));
#225492=CARTESIAN_POINT('Ctrl Pts',(188.367026683425,-2.39458035173523,
136.217187496532));
#225493=CARTESIAN_POINT('Ctrl Pts',(188.35962660091,-2.24898081214349,136.277021384424));
#225494=CARTESIAN_POINT('Ctrl Pts',(188.352218381243,-2.10322117088992,
136.336921065828));
#225495=CARTESIAN_POINT('Ctrl Pts',(188.344810161577,-1.95516221465031,
136.390954270921));
#225496=CARTESIAN_POINT('Ctrl Pts',(188.33740194191,-1.80532063496924,136.43896335134));
#225497=CARTESIAN_POINT('Ctrl Pts',(188.329989162608,-1.65538683029596,
136.487001980547));
#225498=CARTESIAN_POINT('Ctrl Pts',(188.322576383306,-1.50366857485122,
136.529008997548));
#225499=CARTESIAN_POINT('Ctrl Pts',(188.315163604004,-1.35069426213214,
136.564877571169));
#225500=CARTESIAN_POINT('Ctrl Pts',(188.307740232975,-1.19750137254131,
136.600797395489));
#225501=CARTESIAN_POINT('Ctrl Pts',(188.300316861946,-1.04304920681346,
136.630561188534));
#225502=CARTESIAN_POINT('Ctrl Pts',(188.292893490918,-0.887873634317857,
136.654113686883));
#225503=CARTESIAN_POINT('Ctrl Pts',(188.288957441477,-0.805595822389184,
136.666601786643));
#225504=CARTESIAN_POINT('Ctrl Pts',(188.285021392036,-0.72311468724722,
136.67734453826));
#225505=CARTESIAN_POINT('Ctrl Pts',(188.281085342595,-0.640510152529407,
136.686339647366));
#225506=CARTESIAN_POINT('Ctrl Pts',(188.273662076189,-0.484720578059533,
136.703304142411));
#225507=CARTESIAN_POINT('Ctrl Pts',(188.266238809784,-0.328020986091857,
136.714100671442));
#225508=CARTESIAN_POINT('Ctrl Pts',(188.258815543378,-0.170941080575582,
136.718640768985));
#225509=CARTESIAN_POINT('Ctrl Pts',(188.251401050657,-0.014046830462841,
136.72317550051));
#225510=CARTESIAN_POINT('Ctrl Pts',(188.243986557936,0.143226468969914,
136.721468508825));
#225511=CARTESIAN_POINT('Ctrl Pts',(188.236572065215,0.300341982397618,
136.713482824469));
#225512=CARTESIAN_POINT('Ctrl Pts',(188.229164718861,0.457306061978129,
136.705504837015));
#225513=CARTESIAN_POINT('Ctrl Pts',(188.221757372508,0.61411228800125,136.691260223337));
#225514=CARTESIAN_POINT('Ctrl Pts',(188.214350026154,0.770221908090596,
136.670764011026));
#225515=CARTESIAN_POINT('Ctrl Pts',(188.206948204478,0.926215095735712,
136.650283085563));
#225516=CARTESIAN_POINT('Ctrl Pts',(188.199546382803,1.08151234342266,136.623559893873));
#225517=CARTESIAN_POINT('Ctrl Pts',(188.192144561128,1.23557822068304,136.590661424046));
#225518=CARTESIAN_POINT('Ctrl Pts',(188.184746646816,1.38956276776613,136.557780321065));
#225519=CARTESIAN_POINT('Ctrl Pts',(188.177348732505,1.54231687484672,136.518730509913));
#225520=CARTESIAN_POINT('Ctrl Pts',(188.169950818194,1.69331364128615,136.473630365491));
#225521=CARTESIAN_POINT('Ctrl Pts',(188.162554133281,1.84428531480222,136.428537715894));
#225522=CARTESIAN_POINT('Ctrl Pts',(188.155157448369,1.99349986995265,136.377396835288));
#225523=CARTESIAN_POINT('Ctrl Pts',(188.147760763457,2.14044383721241,136.320376457123));
#225524=CARTESIAN_POINT('Ctrl Pts',(188.140364406522,2.28738128882264,136.263358607301));
#225525=CARTESIAN_POINT('Ctrl Pts',(188.132968049586,2.43204800471394,136.20046191333));
#225526=CARTESIAN_POINT('Ctrl Pts',(188.125571692651,2.57394908891939,136.131903827166));
#225527=CARTESIAN_POINT('Ctrl Pts',(188.118174203314,2.71587189854313,136.063335244583));
#225528=CARTESIAN_POINT('Ctrl Pts',(188.110776713978,2.85502789723953,135.989103706352));
#225529=CARTESIAN_POINT('Ctrl Pts',(188.103379224641,2.99094559062203,135.909473254564));
#225530=CARTESIAN_POINT('Ctrl Pts',(188.095979142126,3.12691092974114,135.829814888445));
#225531=CARTESIAN_POINT('Ctrl Pts',(188.088579059611,3.25963538151613,135.744754029243));
#225532=CARTESIAN_POINT('Ctrl Pts',(188.081178977096,3.38867543359986,135.65459869092));
#225533=CARTESIAN_POINT('Ctrl Pts',(188.07377075743,3.51785737848661,135.564344217535));
#225534=CARTESIAN_POINT('Ctrl Pts',(188.066362537763,3.64334652662018,135.46898429159));
#225535=CARTESIAN_POINT('Ctrl Pts',(188.058954318097,3.76473095956622,135.368868407524));
#225536=CARTESIAN_POINT('Ctrl Pts',(188.051541538795,3.88619010260547,135.268690903801));
#225537=CARTESIAN_POINT('Ctrl Pts',(188.044128759492,4.0035392187013,135.163751857378));
#225538=CARTESIAN_POINT('Ctrl Pts',(188.03671598019,4.11640281816916,135.054438075809));
#225539=CARTESIAN_POINT('Ctrl Pts',(188.029292609162,4.22942768244064,134.944968101584));
#225540=CARTESIAN_POINT('Ctrl Pts',(188.021869238133,4.33795397276301,134.831111177405));
#225541=CARTESIAN_POINT('Ctrl Pts',(188.014445867104,4.44164554397361,134.713288274123));
#225542=CARTESIAN_POINT('Ctrl Pts',(188.010509817663,4.49662530307466,134.650815743681));
#225543=CARTESIAN_POINT('Ctrl Pts',(188.006573768223,4.55024655251569,134.587228748358));
#225544=CARTESIAN_POINT('Ctrl Pts',(188.002637718782,4.60246416130131,134.522593290011));
#225545=CARTESIAN_POINT('Ctrl Pts',(187.995214452376,4.70094494181516,134.400692832772));
#225546=CARTESIAN_POINT('Ctrl Pts',(187.987791185971,4.79472832452141,134.274692815747));
#225547=CARTESIAN_POINT('Ctrl Pts',(187.980367919565,4.88345356298841,134.144991076123));
#225548=CARTESIAN_POINT('Ctrl Pts',(187.972953426844,4.9720739355918,134.015442633183));
#225549=CARTESIAN_POINT('Ctrl Pts',(187.965538934123,5.05564785509995,133.882201481457));
#225550=CARTESIAN_POINT('Ctrl Pts',(187.958124441402,5.13385404545199,133.745699292812));
#225551=CARTESIAN_POINT('Ctrl Pts',(187.950717095049,5.21198485773338,133.609328670115));
#225552=CARTESIAN_POINT('Ctrl Pts',(187.943309748695,5.28475805618814,133.469703589541));
#225553=CARTESIAN_POINT('Ctrl Pts',(187.935902402341,5.3518950751355,133.327285441504));
#225554=CARTESIAN_POINT('Ctrl Pts',(187.928500580666,5.41898202076117,133.184973514294));
#225555=CARTESIAN_POINT('Ctrl Pts',(187.92109875899,5.48044099847369,133.03987300371));
#225556=CARTESIAN_POINT('Ctrl Pts',(187.913696937315,5.53603895400241,132.892470591267));
#225557=CARTESIAN_POINT('Ctrl Pts',(187.906299023003,5.59160755980321,132.74514599141));
#225558=CARTESIAN_POINT('Ctrl Pts',(187.898901108692,5.64132117383657,132.595522258129));
#225559=CARTESIAN_POINT('Ctrl Pts',(187.891503194381,5.68499458559291,132.44410667238));
#225560=CARTESIAN_POINT('Ctrl Pts',(187.884106509468,5.72866073962051,132.292716249155));
#225561=CARTESIAN_POINT('Ctrl Pts',(187.876709824556,5.76628858020843,132.139534922778));
#225562=CARTESIAN_POINT('Ctrl Pts',(187.869313139644,5.79774252476681,131.985085894254));
#225563=CARTESIAN_POINT('Ctrl Pts',(187.861916782709,5.82919507462433,131.830643714162));
#225564=CARTESIAN_POINT('Ctrl Pts',(187.854520425773,5.85447419827982,131.67493430948));
#225565=CARTESIAN_POINT('Ctrl Pts',(187.847124068838,5.87349534086361,131.518491588294));
#225566=CARTESIAN_POINT('Ctrl Pts',(187.839726579501,5.8925193956329,131.362024915329));
#225567=CARTESIAN_POINT('Ctrl Pts',(187.832329090164,5.90528351654167,131.204825072902));
#225568=CARTESIAN_POINT('Ctrl Pts',(187.824931600828,5.91175499544869,131.047431463797));
#225569=CARTESIAN_POINT('Ctrl Pts',(187.817531518313,5.9182287429226,130.889982680606));
#225570=CARTESIAN_POINT('Ctrl Pts',(187.810131435798,5.91840544118585,130.73234036825));
#225571=CARTESIAN_POINT('Ctrl Pts',(187.802731353283,5.91230450185313,130.575044155298));
#225572=CARTESIAN_POINT('Ctrl Pts',(187.795323133616,5.90619685391042,130.417574978989));
#225573=CARTESIAN_POINT('Ctrl Pts',(187.78791491395,5.89379779728831,130.260453035358));
#225574=CARTESIAN_POINT('Ctrl Pts',(187.780506694283,5.87517871958054,130.10421379333));
#225575=CARTESIAN_POINT('Ctrl Pts',(187.773093914981,5.8565481821411,129.947878388655));
#225576=CARTESIAN_POINT('Ctrl Pts',(187.765681135679,5.83169005401839,129.792427135914));
#225577=CARTESIAN_POINT('Ctrl Pts',(187.758268356377,5.80072680601682,129.638385024143));
#225578=CARTESIAN_POINT('Ctrl Pts',(187.750844985348,5.76971931627449,129.484122809779));
#225579=CARTESIAN_POINT('Ctrl Pts',(187.74342161432,5.73258937218858,129.331274119478));
#225580=CARTESIAN_POINT('Ctrl Pts',(187.735998243291,5.68950945378594,129.180349306712));
#225581=CARTESIAN_POINT('Ctrl Pts',(187.73206219385,5.66666744736085,129.100325349594));
#225582=CARTESIAN_POINT('Ctrl Pts',(187.728126144409,5.64215350241321,129.020841949638));
#225583=CARTESIAN_POINT('Ctrl Pts',(187.724190094969,5.61599875376964,128.941972752443));
#225584=CARTESIAN_POINT('Ctrl Pts',(187.716766828563,5.56667171408872,128.793227907954));
#225585=CARTESIAN_POINT('Ctrl Pts',(187.709343562158,5.51135654039937,128.646219205077));
#225586=CARTESIAN_POINT('Ctrl Pts',(187.701920295752,5.45019295213473,128.501465190717));
#225587=CARTESIAN_POINT('Ctrl Pts',(187.694505803031,5.38910165415207,128.356882263581));
#225588=CARTESIAN_POINT('Ctrl Pts',(187.68709131031,5.32217584452053,128.214549061059));
#225589=CARTESIAN_POINT('Ctrl Pts',(187.679676817589,5.24960504344817,128.074969210988));
#225590=CARTESIAN_POINT('Ctrl Pts',(187.672269471236,5.17710418884611,127.935523893231));
#225591=CARTESIAN_POINT('Ctrl Pts',(187.664862124882,5.09896934552089,127.798826973745));
#225592=CARTESIAN_POINT('Ctrl Pts',(187.657454778528,5.01543812273929,127.665362210514));
#225593=CARTESIAN_POINT('Ctrl Pts',(187.650052956853,4.9319692006951,127.53199699034));
#225594=CARTESIAN_POINT('Ctrl Pts',(187.642651135177,4.84311211035346,127.401859441534));
#225595=CARTESIAN_POINT('Ctrl Pts',(187.635249313502,4.74915033913089,127.275408702502));
#225596=CARTESIAN_POINT('Ctrl Pts',(187.62785139919,4.65523816959588,127.149024715831));
#225597=CARTESIAN_POINT('Ctrl Pts',(187.620453484879,4.55622690793055,127.026323961781));
#225598=CARTESIAN_POINT('Ctrl Pts',(187.613055570568,4.45244323316465,126.907736460947));
#225599=CARTESIAN_POINT('Ctrl Pts',(187.605658885656,4.34867680536279,126.789168667204));
#225600=CARTESIAN_POINT('Ctrl Pts',(187.598262200743,4.24013978411027,126.674713050673));
#225601=CARTESIAN_POINT('Ctrl Pts',(187.590865515831,4.12719906752894,126.56476648375));
#225602=CARTESIAN_POINT('Ctrl Pts',(187.583469158896,4.01426335885729,126.454824791973));
#225603=CARTESIAN_POINT('Ctrl Pts',(187.57607280196,3.89692461059156,126.349392012655));
#225604=CARTESIAN_POINT('Ctrl Pts',(187.568676445025,3.77558631075384,126.248827874566));
#225605=CARTESIAN_POINT('Ctrl Pts',(187.561278955688,3.65422943371256,126.14824833985));
#225606=CARTESIAN_POINT('Ctrl Pts',(187.553881466352,3.52887207328063,126.05253916878));
#225607=CARTESIAN_POINT('Ctrl Pts',(187.546483977015,3.39995036474609,125.962019440019));
#225608=CARTESIAN_POINT('Ctrl Pts',(187.5390838945,3.27098346290651,125.871467979709));
#225609=CARTESIAN_POINT('Ctrl Pts',(187.531683811985,3.13845003058641,125.786109797999));
#225610=CARTESIAN_POINT('Ctrl Pts',(187.52428372947,3.00281456503668,125.706220245773));
#225611=CARTESIAN_POINT('Ctrl Pts',(187.516875509804,2.86702995434889,125.626242846772));
#225612=CARTESIAN_POINT('Ctrl Pts',(187.509467290137,2.72813682027947,125.551746275818));
#225613=CARTESIAN_POINT('Ctrl Pts',(187.502059070471,2.58662425473907,125.482959906541));
#225614=CARTESIAN_POINT('Ctrl Pts',(187.494646291169,2.44502459057584,125.414131200402));
#225615=CARTESIAN_POINT('Ctrl Pts',(187.487233511867,2.3008026235927,125.351019848396));
#225616=CARTESIAN_POINT('Ctrl Pts',(187.479820732564,2.15446624039682,125.293806581764));
#225617=CARTESIAN_POINT('Ctrl Pts',(187.472397361536,2.00792076491405,125.236511566134));
#225618=CARTESIAN_POINT('Ctrl Pts',(187.464973990507,1.85925519113648,125.185131589024));
#225619=CARTESIAN_POINT('Ctrl Pts',(187.457550619478,1.7089921235619,125.139797396619));
#225620=CARTESIAN_POINT('Ctrl Pts',(187.453614570037,1.62931903962022,125.115760120027));
#225621=CARTESIAN_POINT('Ctrl Pts',(187.449678520597,1.54919701811686,125.093421677015));
#225622=CARTESIAN_POINT('Ctrl Pts',(187.445742471156,1.46870484831581,125.072795680218));
#225623=CARTESIAN_POINT('Ctrl Pts',(187.43831920475,1.31689912814708,125.033895693975));
#225624=CARTESIAN_POINT('Ctrl Pts',(187.430895938345,1.1633173403862,125.000972121415));
#225625=CARTESIAN_POINT('Ctrl Pts',(187.423472671939,1.00847127499773,124.97418769989));
#225626=CARTESIAN_POINT('Ctrl Pts',(187.416058179218,0.853808224799215,
124.947434935327));
#225627=CARTESIAN_POINT('Ctrl Pts',(187.408643686497,0.697884235571734,
124.926806941762));
#225628=CARTESIAN_POINT('Ctrl Pts',(187.401229193776,0.541225463979645,
124.912416493625));
#225629=CARTESIAN_POINT('Ctrl Pts',(187.393821847423,0.384717686009742,
124.898039915544));
#225630=CARTESIAN_POINT('Ctrl Pts',(187.386414501069,0.227476904821062,
124.889888948137));
#225631=CARTESIAN_POINT('Ctrl Pts',(187.379007154715,0.0700385533196246,
124.888025167006));
#225632=CARTESIAN_POINT('Ctrl Pts',(187.37160533304,-0.0872823747195095,
124.886162775954));
#225633=CARTESIAN_POINT('Ctrl Pts',(187.364203511364,-0.244800208001704,
124.890578238706));
#225634=CARTESIAN_POINT('Ctrl Pts',(187.356801689689,-0.401975428509942,
124.901281224794));
#225635=CARTESIAN_POINT('Ctrl Pts',(187.349403775377,-0.559067677442723,
124.911978560858));
#225636=CARTESIAN_POINT('Ctrl Pts',(187.342005861066,-0.715817302305466,
124.928956784745));
#225637=CARTESIAN_POINT('Ctrl Pts',(187.334607946755,-0.871685936598251,
124.952173488771));
#225638=CARTESIAN_POINT('Ctrl Pts',(187.327211261842,-1.02752866835165,
124.975386334601));
#225639=CARTESIAN_POINT('Ctrl Pts',(187.31981457693,-1.18249033124199,125.00483554804));
#225640=CARTESIAN_POINT('Ctrl Pts',(187.312417892018,-1.33603870788574,
125.040426966531));
#225641=CARTESIAN_POINT('Ctrl Pts',(187.305021535083,-1.48958027603362,
125.076016806862));
#225642=CARTESIAN_POINT('Ctrl Pts',(187.297625178147,-1.64170831888113,
125.117748226424));
#225643=CARTESIAN_POINT('Ctrl Pts',(187.290228821212,-1.79190209129523,
125.165476201504));
#225644=CARTESIAN_POINT('Ctrl Pts',(187.282831331875,-1.94211885875933,
125.213211483858));
#225645=CARTESIAN_POINT('Ctrl Pts',(187.275433842538,-2.09040041034268,
125.266945036705));
#225646=CARTESIAN_POINT('Ctrl Pts',(187.268036353202,-2.2362425543513,125.326482396885));
#225647=CARTESIAN_POINT('Ctrl Pts',(187.260636270687,-2.38213582309748,
125.386040627795));
#225648=CARTESIAN_POINT('Ctrl Pts',(187.253236188172,-2.52558763631716,
125.451406575745));
#225649=CARTESIAN_POINT('Ctrl Pts',(187.245836105657,-2.66611526140484,
125.522338279919));
#225650=CARTESIAN_POINT('Ctrl Pts',(187.23842788599,-2.80679741106287,125.593347980794));
#225651=CARTESIAN_POINT('Ctrl Pts',(187.231019666324,-2.94454861767688,
125.669935491864));
#225652=CARTESIAN_POINT('Ctrl Pts',(187.223611446657,-3.07891153659171,
125.751813308303));
#225653=CARTESIAN_POINT('Ctrl Pts',(187.216198667355,-3.2133571536413,125.833741519172));
#225654=CARTESIAN_POINT('Ctrl Pts',(187.208785888053,-3.34441001746257,
125.920966317233));
#225655=CARTESIAN_POINT('Ctrl Pts',(187.201373108751,-3.47164354862595,
126.013158092752));
#225656=CARTESIAN_POINT('Ctrl Pts',(187.193949737723,-3.59905887702523,
126.105481596203));
#225657=CARTESIAN_POINT('Ctrl Pts',(187.186526366694,-3.72264368091018,
126.202786021196));
#225658=CARTESIAN_POINT('Ctrl Pts',(187.179102995665,-3.84200547931489,
126.304702357274));
#225659=CARTESIAN_POINT('Ctrl Pts',(187.175166946224,-3.90529396887533,
126.358740844111));
#225660=CARTESIAN_POINT('Ctrl Pts',(187.171230896784,-3.96739584334917,
126.414075295879));
#225661=CARTESIAN_POINT('Ctrl Pts',(187.167294847343,-4.02825706251959,
126.470646782902));
#225662=CARTESIAN_POINT('Ctrl Pts',(187.159982110724,-4.14133035410826,
126.57575023523));
#225663=CARTESIAN_POINT('Ctrl Pts',(187.152669374104,-4.25048290247324,
126.685464074864));
#225664=CARTESIAN_POINT('Ctrl Pts',(187.145356637485,-4.355306958856,126.799459637936));
#225665=CARTESIAN_POINT('Ctrl Pts',(187.138052644169,-4.4600056848014,126.913318904872));
#225666=CARTESIAN_POINT('Ctrl Pts',(187.130748650852,-4.56038595696257,
127.03144942948));
#225667=CARTESIAN_POINT('Ctrl Pts',(187.123444657536,-4.65607377997443,
127.153482980896));
#225668=CARTESIAN_POINT('Ctrl Pts',(187.11614769061,-4.75166955197894,127.275399136901));
#225669=CARTESIAN_POINT('Ctrl Pts',(187.108850723683,-4.84258162128955,
127.401210547057));
#225670=CARTESIAN_POINT('Ctrl Pts',(187.101553756756,-4.92847369766666,
127.530513099139));
#225671=CARTESIAN_POINT('Ctrl Pts',(187.094262461591,-5.01429901214382,
127.659715147376));
#225672=CARTESIAN_POINT('Ctrl Pts',(187.086971166426,-5.09511188989882,
127.792402615212));
#225673=CARTESIAN_POINT('Ctrl Pts',(187.079679871261,-5.1706173282255,127.92813965812));
#225674=CARTESIAN_POINT('Ctrl Pts',(187.072391625532,-5.24609118793796,
128.063819931771));
#225675=CARTESIAN_POINT('Ctrl Pts',(187.065103379803,-5.31626183691263,
128.202546907271));
#225676=CARTESIAN_POINT('Ctrl Pts',(187.057815134074,-5.38087854125002,
128.343857277431));
#225677=CARTESIAN_POINT('Ctrl Pts',(187.050528398168,-5.44548185967987,
128.48513837393));
#225678=CARTESIAN_POINT('Ctrl Pts',(187.043241662262,-5.50453336306754,
128.629001449778));
#225679=CARTESIAN_POINT('Ctrl Pts',(187.035954926356,-5.55782922554555,
128.774960493842));
#225680=CARTESIAN_POINT('Ctrl Pts',(187.028668162023,-5.61112529593695,
128.920920107308));
#225681=CARTESIAN_POINT('Ctrl Pts',(187.021381397691,-5.65866555016246,
129.068975342758));
#225682=CARTESIAN_POINT('Ctrl Pts',(187.014094633358,-5.7002951840503,129.218622500097));
#225683=CARTESIAN_POINT('Ctrl Pts',(187.006803471584,-5.74194994073617,
129.368359967031));
#225684=CARTESIAN_POINT('Ctrl Pts',(186.999512309809,-5.77768684994215,
129.519690902912));
#225685=CARTESIAN_POINT('Ctrl Pts',(186.992221148034,-5.80740158088912,
129.672098527418));
#225686=CARTESIAN_POINT('Ctrl Pts',(186.984927500083,-5.8371264441105,129.824558120621));
#225687=CARTESIAN_POINT('Ctrl Pts',(186.977633852133,-5.86082497829701,
129.97809475339));
#225688=CARTESIAN_POINT('Ctrl Pts',(186.970340204182,-5.87844452383703,
130.132184641597));
#225689=CARTESIAN_POINT('Ctrl Pts',(186.963039152689,-5.89608195439748,
130.286430941374));
#225690=CARTESIAN_POINT('Ctrl Pts',(186.955738101197,-5.90762804625571,
130.441231234208));
#225691=CARTESIAN_POINT('Ctrl Pts',(186.948437049704,-5.91308220639865,
130.596059434488));
#225692=CARTESIAN_POINT('Ctrl Pts',(186.945083097206,-5.91558773509581,
130.66718431692));
#225693=CARTESIAN_POINT('Ctrl Pts',(186.941729144709,-5.91680841145624,
130.738315114615));
#225694=CARTESIAN_POINT('Ctrl Pts',(186.938375192211,-5.91674785298769,
130.809401120074));
#225695=CARTESIAN_POINT('',(190.438375193894,-5.91568182138061,130.798900870218));
#225696=CARTESIAN_POINT('Ctrl Pts',(190.438375192211,-5.91556591356672,
130.798901012961));
#225697=CARTESIAN_POINT('Ctrl Pts',(190.368989697902,-5.90218450277572,
132.273183331429));
#225698=CARTESIAN_POINT('Ctrl Pts',(190.206788328991,-4.59798200865986,
135.740709904657));
#225699=CARTESIAN_POINT('Ctrl Pts',(189.951771085471,1.22745627517318,137.694274377758));
#225700=CARTESIAN_POINT('Ctrl Pts',(189.673323461659,6.46014967796433,133.495833572777));
#225701=CARTESIAN_POINT('Ctrl Pts',(189.394875837845,5.75628112256356,126.824060607722));
#225702=CARTESIAN_POINT('Ctrl Pts',(189.116428214034,-0.237328574507486,
123.809988903246));
#225703=CARTESIAN_POINT('Ctrl Pts',(188.880927998822,-5.12203658652489,
126.696922428952));
#225704=CARTESIAN_POINT('Ctrl Pts',(188.738243658214,-5.90521979014647,
129.742180863919));
#225705=CARTESIAN_POINT('Ctrl Pts',(188.688375192211,-5.90715995150835,
130.805573381844));
#225706=CARTESIAN_POINT('',(192.188375873533,-5.92197168067619,130.805533319426));
#225707=CARTESIAN_POINT('Ctrl Pts',(192.188375192211,-5.91674988112158,
130.805546681526));
#225708=CARTESIAN_POINT('Ctrl Pts',(192.185367486799,-5.91673715075054,
130.869052886841));
#225709=CARTESIAN_POINT('Ctrl Pts',(192.182359781387,-5.91570200665032,
130.932547687523));
#225710=CARTESIAN_POINT('Ctrl Pts',(192.179352075975,-5.91364535475517,
130.996009204001));
#225711=CARTESIAN_POINT('Ctrl Pts',(192.17192880957,-5.90856936730653,131.152637489943));
#225712=CARTESIAN_POINT('Ctrl Pts',(192.164505543164,-5.89725874201999,
131.309300813403));
#225713=CARTESIAN_POINT('Ctrl Pts',(192.157082276759,-5.87970025871574,
131.465462296703));
#225714=CARTESIAN_POINT('Ctrl Pts',(192.149667784038,-5.86216252808058,
131.621439210099));
#225715=CARTESIAN_POINT('Ctrl Pts',(192.142253291317,-5.83839167951754,
131.776915096634));
#225716=CARTESIAN_POINT('Ctrl Pts',(192.134838798596,-5.80842648002977,
131.931353247794));
#225717=CARTESIAN_POINT('Ctrl Pts',(192.127431452242,-5.77849016212943,
132.08564254565));
#225718=CARTESIAN_POINT('Ctrl Pts',(192.120024105888,-5.74237144971965,
132.238895735347));
#225719=CARTESIAN_POINT('Ctrl Pts',(192.112616759534,-5.70016086098663,
132.390581510562));
#225720=CARTESIAN_POINT('Ctrl Pts',(192.105214937859,-5.65798175450327,
132.542154152802));
#225721=CARTESIAN_POINT('Ctrl Pts',(192.097813116184,-5.60971991816693,
132.692161350184));
#225722=CARTESIAN_POINT('Ctrl Pts',(192.090411294508,-5.55551684961682,
132.84008238051));
#225723=CARTESIAN_POINT('Ctrl Pts',(192.083013380197,-5.5013423944446,132.987925324475));
#225724=CARTESIAN_POINT('Ctrl Pts',(192.075615465886,-5.44123308132258,
133.133683944999));
#225725=CARTESIAN_POINT('Ctrl Pts',(192.068217551574,-5.37538008816079,
133.2768531798));
#225726=CARTESIAN_POINT('Ctrl Pts',(192.060820866662,-5.30953803857184,
133.419998622472));
#225727=CARTESIAN_POINT('Ctrl Pts',(192.05342418175,-5.23795435917514,133.560555194648));
#225728=CARTESIAN_POINT('Ctrl Pts',(192.046027496837,-5.16086820194777,
133.69803820234));
#225729=CARTESIAN_POINT('Ctrl Pts',(192.038631139902,-5.08378546280139,
133.835515113891));
#225730=CARTESIAN_POINT('Ctrl Pts',(192.031234782967,-5.00120091351712,
133.969918406331));
#225731=CARTESIAN_POINT('Ctrl Pts',(192.023838426031,-4.91339933435241,
134.100788615215));
#225732=CARTESIAN_POINT('Ctrl Pts',(192.016440936695,-4.82558431254177,
134.231678860662));
#225733=CARTESIAN_POINT('Ctrl Pts',(192.009043447358,-4.73255087844258,
134.359034635486));
#225734=CARTESIAN_POINT('Ctrl Pts',(192.001645958021,-4.63462665546448,
134.482426186171));
#225735=CARTESIAN_POINT('Ctrl Pts',(191.994245875506,-4.53666810530159,
134.605860991573));
#225736=CARTESIAN_POINT('Ctrl Pts',(191.986845792991,-4.43381558469625,
134.725328513823));
#225737=CARTESIAN_POINT('Ctrl Pts',(191.979445710476,-4.32643632479157,
134.840432877824));
#225738=CARTESIAN_POINT('Ctrl Pts',(191.97203749081,-4.21893899035197,134.955663810906));
#225739=CARTESIAN_POINT('Ctrl Pts',(191.964629271143,-4.10690523078763,
135.066521731207));
#225740=CARTESIAN_POINT('Ctrl Pts',(191.957221051477,-3.99073891115741,
135.172647868363));
#225741=CARTESIAN_POINT('Ctrl Pts',(191.949808272175,-3.8745010930958,135.278839324385));
#225742=CARTESIAN_POINT('Ctrl Pts',(191.942395492873,-3.75412593146085,
135.380292954059));
#225743=CARTESIAN_POINT('Ctrl Pts',(191.934982713571,-3.63004912034786,
135.476691293616));
#225744=CARTESIAN_POINT('Ctrl Pts',(191.927559342542,-3.50579502246853,
135.573227371642));
#225745=CARTESIAN_POINT('Ctrl Pts',(191.920135971513,-3.37782901450236,
135.664693516634));
#225746=CARTESIAN_POINT('Ctrl Pts',(191.912712600484,-3.24661509159063,
135.750816016087));
#225747=CARTESIAN_POINT('Ctrl Pts',(191.908776551044,-3.17704232122627,
135.796480231779));
#225748=CARTESIAN_POINT('Ctrl Pts',(191.904840501603,-3.10655685573822,
135.84064292555));
#225749=CARTESIAN_POINT('Ctrl Pts',(191.900904452162,-3.03523037952588,
135.883268679906));
#225750=CARTESIAN_POINT('Ctrl Pts',(191.893481185756,-2.90071087141565,
135.963659522316));
#225751=CARTESIAN_POINT('Ctrl Pts',(191.886057919351,-2.76279191120802,
136.038823925974));
#225752=CARTESIAN_POINT('Ctrl Pts',(191.878634652946,-2.62191804346816,
136.108460572868));
#225753=CARTESIAN_POINT('Ctrl Pts',(191.871220160225,-2.48121067694097,
136.178014915029));
#225754=CARTESIAN_POINT('Ctrl Pts',(191.863805667504,-2.33755568601003,
136.242054341289));
#225755=CARTESIAN_POINT('Ctrl Pts',(191.856391174783,-2.19142557325891,
136.300321363365));
#225756=CARTESIAN_POINT('Ctrl Pts',(191.848983828429,-2.04543630621208,
136.358532225492));
#225757=CARTESIAN_POINT('Ctrl Pts',(191.841576482075,-1.89697701105787,
136.410981622255));
#225758=CARTESIAN_POINT('Ctrl Pts',(191.834169135721,-1.74654361814439,
136.457458525122));
#225759=CARTESIAN_POINT('Ctrl Pts',(191.826767314046,-1.59622242413098,
136.503900763762));
#225760=CARTESIAN_POINT('Ctrl Pts',(191.819365492371,-1.44393041914754,
136.544379268321));
#225761=CARTESIAN_POINT('Ctrl Pts',(191.811963670695,-1.29018218445807,
136.578731621702));
#225762=CARTESIAN_POINT('Ctrl Pts',(191.804565756384,-1.1365151122651,136.613065840743));
#225763=CARTESIAN_POINT('Ctrl Pts',(191.797167842073,-0.981393704726121,
136.641280267975));
#225764=CARTESIAN_POINT('Ctrl Pts',(191.789769927761,-0.825346221371544,
136.663262748287));
#225765=CARTESIAN_POINT('Ctrl Pts',(191.782373242849,-0.669324670277544,
136.68524157551));
#225766=CARTESIAN_POINT('Ctrl Pts',(191.774976557937,-0.512377718094195,
136.700990459225));
#225767=CARTESIAN_POINT('Ctrl Pts',(191.767579873025,-0.355042419086338,
136.710448615822));
#225768=CARTESIAN_POINT('Ctrl Pts',(191.760183516089,-0.19771409649043,
136.719906353036));
#225769=CARTESIAN_POINT('Ctrl Pts',(191.752787159154,-0.0399978339334864,
136.723073895353));
#225770=CARTESIAN_POINT('Ctrl Pts',(191.745390802218,0.117565877448984,
136.719942484716));
#225771=CARTESIAN_POINT('Ctrl Pts',(191.737993312882,0.275153712237935,
136.716810594653));
#225772=CARTESIAN_POINT('Ctrl Pts',(191.730595823545,0.432588576099383,
136.707377838831));
#225773=CARTESIAN_POINT('Ctrl Pts',(191.723198334209,0.589331816772684,
136.691687563833));
#225774=CARTESIAN_POINT('Ctrl Pts',(191.715798251694,0.746130003545964,
136.675991788633));
#225775=CARTESIAN_POINT('Ctrl Pts',(191.708398169179,0.902235713210191,
136.654034164045));
#225776=CARTESIAN_POINT('Ctrl Pts',(191.700998086664,1.0571173874321,136.625909671872));
#225777=CARTESIAN_POINT('Ctrl Pts',(191.693589866998,1.21216936997707,136.597754253928));
#225778=CARTESIAN_POINT('Ctrl Pts',(191.686181647331,1.36599426160672,136.563418492823));
#225779=CARTESIAN_POINT('Ctrl Pts',(191.678773427665,1.51807191972469,136.523048247525));
#225780=CARTESIAN_POINT('Ctrl Pts',(191.671360648363,1.67024317910383,136.482653155014));
#225781=CARTESIAN_POINT('Ctrl Pts',(191.663947869061,1.82066470625482,136.43621628731));
#225782=CARTESIAN_POINT('Ctrl Pts',(191.656535089759,1.96883390661907,136.383932609274));
#225783=CARTESIAN_POINT('Ctrl Pts',(191.64911171873,2.11721481808522,136.331574225866));
#225784=CARTESIAN_POINT('Ctrl Pts',(191.641688347701,2.26333662937201,136.273352484731));
#225785=CARTESIAN_POINT('Ctrl Pts',(191.634264976672,2.40671825768975,136.209509809827));
#225786=CARTESIAN_POINT('Ctrl Pts',(191.630328927231,2.48274263741927,136.175658891709));
#225787=CARTESIAN_POINT('Ctrl Pts',(191.626392877791,2.55799707823944,136.140228488059));
#225788=CARTESIAN_POINT('Ctrl Pts',(191.62245682835,2.63241303524121,136.103259764973));
#225789=CARTESIAN_POINT('Ctrl Pts',(191.615033561944,2.77275920770318,136.033537906988));
#225790=CARTESIAN_POINT('Ctrl Pts',(191.607610295539,2.91054571611699,135.958130975866));
#225791=CARTESIAN_POINT('Ctrl Pts',(191.600187029134,3.04527876591065,135.877250109798));
#225792=CARTESIAN_POINT('Ctrl Pts',(191.592772536413,3.17985257242841,135.796464838196));
#225793=CARTESIAN_POINT('Ctrl Pts',(191.585358043692,3.31137978699819,135.710218699948));
#225794=CARTESIAN_POINT('Ctrl Pts',(191.577943550971,3.43938837824726,135.618770046154));
#225795=CARTESIAN_POINT('Ctrl Pts',(191.570536204617,3.56727358999668,135.527409534016));
#225796=CARTESIAN_POINT('Ctrl Pts',(191.563128858263,3.69164662828833,135.430856704515));
#225797=CARTESIAN_POINT('Ctrl Pts',(191.555721511909,3.81206188637452,135.329414731823));
#225798=CARTESIAN_POINT('Ctrl Pts',(191.548319690234,3.93238733421826,135.228048418381));
#225799=CARTESIAN_POINT('Ctrl Pts',(191.540917868558,4.04876059514704,135.121800461911));
#225800=CARTESIAN_POINT('Ctrl Pts',(191.533516046883,4.16076687931502,135.011016003796));
#225801=CARTESIAN_POINT('Ctrl Pts',(191.526118132572,4.27271403623751,134.900290027933));
#225802=CARTESIAN_POINT('Ctrl Pts',(191.51872021826,4.38029854276746,134.785032581598));
#225803=CARTESIAN_POINT('Ctrl Pts',(191.511322303949,4.48314050245561,134.665627481918));
#225804=CARTESIAN_POINT('Ctrl Pts',(191.503925619037,4.58596537167568,134.546242225199));
#225805=CARTESIAN_POINT('Ctrl Pts',(191.496528934124,4.68404901487392,134.422710965694));
#225806=CARTESIAN_POINT('Ctrl Pts',(191.489132249212,4.77705000213056,134.295452687341));
#225807=CARTESIAN_POINT('Ctrl Pts',(191.481735892277,4.87004686562598,134.168200051753));
#225808=CARTESIAN_POINT('Ctrl Pts',(191.474339535341,4.95796130103329,134.037221027301));
#225809=CARTESIAN_POINT('Ctrl Pts',(191.466943178406,5.04049379128799,133.902965610541));
#225810=CARTESIAN_POINT('Ctrl Pts',(191.459545689069,5.12303891747765,133.768689638933));
#225811=CARTESIAN_POINT('Ctrl Pts',(191.452148199733,5.20020026233308,133.63113659425));
#225812=CARTESIAN_POINT('Ctrl Pts',(191.444750710396,5.27172313985551,133.490783089779));
#225813=CARTESIAN_POINT('Ctrl Pts',(191.437350627881,5.34327108961184,133.350380384605));
#225814=CARTESIAN_POINT('Ctrl Pts',(191.429950545366,5.40917646734144,133.207175597486));
#225815=CARTESIAN_POINT('Ctrl Pts',(191.422550462851,5.4692318636611,133.061667283488));
#225816=CARTESIAN_POINT('Ctrl Pts',(191.415142243184,5.52935329706284,132.915998968139));
#225817=CARTESIAN_POINT('Ctrl Pts',(191.407734023518,5.58361176011364,132.768022412689));
#225818=CARTESIAN_POINT('Ctrl Pts',(191.400325803851,5.63184881831531,132.618254068169));
#225819=CARTESIAN_POINT('Ctrl Pts',(191.392913024549,5.68011556562145,132.468393543732));
#225820=CARTESIAN_POINT('Ctrl Pts',(191.385500245247,5.72235342333643,132.316739391503));
#225821=CARTESIAN_POINT('Ctrl Pts',(191.378087465945,5.75845475628461,132.163819841788));
#225822=CARTESIAN_POINT('Ctrl Pts',(191.370664094916,5.79460767251027,132.01068179345));
#225823=CARTESIAN_POINT('Ctrl Pts',(191.363240723888,5.82460648099202,131.856275102001));
#225824=CARTESIAN_POINT('Ctrl Pts',(191.355817352859,5.84839510287327,131.701135552089));
#225825=CARTESIAN_POINT('Ctrl Pts',(191.351881303418,5.86100840099461,131.618876840204));
#225826=CARTESIAN_POINT('Ctrl Pts',(191.347945253977,5.87187666241779,131.536412149219));
#225827=CARTESIAN_POINT('Ctrl Pts',(191.344009204537,5.88099747114688,131.453821399187));
#225828=CARTESIAN_POINT('Ctrl Pts',(191.336585938131,5.89819903175955,131.298057822193));
#225829=CARTESIAN_POINT('Ctrl Pts',(191.329162671726,5.90923401839223,131.14137484216));
#225830=CARTESIAN_POINT('Ctrl Pts',(191.32173940532,5.91401315955457,130.984302027795));
#225831=CARTESIAN_POINT('Ctrl Pts',(191.314324912599,5.91878665216895,130.827414860453));
#225832=CARTESIAN_POINT('Ctrl Pts',(191.306910419878,5.91731900564953,130.67013914539));
#225833=CARTESIAN_POINT('Ctrl Pts',(191.299495927157,5.90957243360595,130.513011661047));
#225834=CARTESIAN_POINT('Ctrl Pts',(191.292088580803,5.90183332800017,130.35603562209));
#225835=CARTESIAN_POINT('Ctrl Pts',(191.28468123445,5.88782736319993,130.199207899769));
#225836=CARTESIAN_POINT('Ctrl Pts',(191.277273888096,5.86756874689005,130.043067268706));
#225837=CARTESIAN_POINT('Ctrl Pts',(191.269872066421,5.84732524022051,129.887043093216));
#225838=CARTESIAN_POINT('Ctrl Pts',(191.262470244745,5.82083841545084,129.731705357212));
#225839=CARTESIAN_POINT('Ctrl Pts',(191.25506842307,5.78817444575804,129.577589592487));
#225840=CARTESIAN_POINT('Ctrl Pts',(191.247670508758,5.7555277191206,129.423555184274));
#225841=CARTESIAN_POINT('Ctrl Pts',(191.240272594447,5.71671041893551,129.270741826916));
#225842=CARTESIAN_POINT('Ctrl Pts',(191.232874680136,5.67184011811256,129.119676600586));
#225843=CARTESIAN_POINT('Ctrl Pts',(191.225477995223,5.6269772739196,128.968636478556));
#225844=CARTESIAN_POINT('Ctrl Pts',(191.218081310311,5.57606353168593,128.819344268479));
#225845=CARTESIAN_POINT('Ctrl Pts',(191.210684625399,5.51926684325338,128.672313696069));
#225846=CARTESIAN_POINT('Ctrl Pts',(191.203288268464,5.46247267324549,128.525289643149));
#225847=CARTESIAN_POINT('Ctrl Pts',(191.195891911528,5.39979621022294,128.380527376718));
#225848=CARTESIAN_POINT('Ctrl Pts',(191.188495554593,5.33145415274227,128.238522123095));
#225849=CARTESIAN_POINT('Ctrl Pts',(191.181098065256,5.26310163191814,128.096495128106));
#225850=CARTESIAN_POINT('Ctrl Pts',(191.17370057592,5.18908195138688,127.957226322785));
#225851=CARTESIAN_POINT('Ctrl Pts',(191.166303086583,5.10965843540239,127.821187602801));
#225852=CARTESIAN_POINT('Ctrl Pts',(191.158903004068,5.03020707762741,127.685101194655));
#225853=CARTESIAN_POINT('Ctrl Pts',(191.151502921553,4.94534830094565,127.552247448424));
#225854=CARTESIAN_POINT('Ctrl Pts',(191.144102839038,4.8553894440146,127.423070344689));
#225855=CARTESIAN_POINT('Ctrl Pts',(191.136694619372,4.7653316680724,127.293751197449));
#225856=CARTESIAN_POINT('Ctrl Pts',(191.129286399705,4.67016282567414,127.168117073055));
#225857=CARTESIAN_POINT('Ctrl Pts',(191.121878180039,4.5702317839837,127.046580421338));
#225858=CARTESIAN_POINT('Ctrl Pts',(191.114465400737,4.47023923640445,126.924968965839));
#225859=CARTESIAN_POINT('Ctrl Pts',(191.107052621435,4.3654788968777,126.807460286267));
#225860=CARTESIAN_POINT('Ctrl Pts',(191.099639842133,4.25633700107888,126.694430460526));
#225861=CARTESIAN_POINT('Ctrl Pts',(191.092216471104,4.14703915822113,126.58123913247));
#225862=CARTESIAN_POINT('Ctrl Pts',(191.084793100075,4.03334752442669,126.472539696962));
#225863=CARTESIAN_POINT('Ctrl Pts',(191.077369729046,3.91568255850171,126.368668939423));
#225864=CARTESIAN_POINT('Ctrl Pts',(191.073433679605,3.85329377023497,126.31359417143));
#225865=CARTESIAN_POINT('Ctrl Pts',(191.069497630165,3.78978845095696,126.259876215498));
#225866=CARTESIAN_POINT('Ctrl Pts',(191.065561580724,3.72523253376711,126.207560303014));
#225867=CARTESIAN_POINT('Ctrl Pts',(191.058138314318,3.60348208867042,126.108894124795));
#225868=CARTESIAN_POINT('Ctrl Pts',(191.050715047913,3.47762493989561,126.014919100111));
#225869=CARTESIAN_POINT('Ctrl Pts',(191.043291781507,3.34805837517246,125.925996580418));
#225870=CARTESIAN_POINT('Ctrl Pts',(191.035877288786,3.2186449473689,125.837179159759));
#225871=CARTESIAN_POINT('Ctrl Pts',(191.028462796065,3.08553113521307,125.753402566677));
#225872=CARTESIAN_POINT('Ctrl Pts',(191.021048303344,2.94914812114376,125.674988733792));
#225873=CARTESIAN_POINT('Ctrl Pts',(191.013640956991,2.81289655815807,125.596650479111));
#225874=CARTESIAN_POINT('Ctrl Pts',(191.006233610637,2.67338238768785,125.523664879322));
#225875=CARTESIAN_POINT('Ctrl Pts',(190.998826264283,2.53106657568212,125.456311201941));
#225876=CARTESIAN_POINT('Ctrl Pts',(190.991424442608,2.38885690817838,125.389007759474));
#225877=CARTESIAN_POINT('Ctrl Pts',(190.984022620932,2.24385009572029,125.327328034653));
#225878=CARTESIAN_POINT('Ctrl Pts',(190.976620799257,2.09653246459078,125.271505822127));
#225879=CARTESIAN_POINT('Ctrl Pts',(190.969222884945,1.94929260129213,125.215713077712));
#225880=CARTESIAN_POINT('Ctrl Pts',(190.961824970634,1.79974469693171,125.165771819394));
#225881=CARTESIAN_POINT('Ctrl Pts',(190.954427056323,1.64839575001803,125.121868029465));
#225882=CARTESIAN_POINT('Ctrl Pts',(190.94703037141,1.49707195455342,125.077971535549));
#225883=CARTESIAN_POINT('Ctrl Pts',(190.939633686498,1.34394806872582,125.040110622631));
#225884=CARTESIAN_POINT('Ctrl Pts',(190.932237001586,1.18954708660089,125.008421669366));
#225885=CARTESIAN_POINT('Ctrl Pts',(190.924840644651,1.03515295077734,124.976734121223));
#225886=CARTESIAN_POINT('Ctrl Pts',(190.917444287715,0.879482196927022,
124.951218063633));
#225887=CARTESIAN_POINT('Ctrl Pts',(190.91004793078,0.723068603840397,124.931958863885));
#225888=CARTESIAN_POINT('Ctrl Pts',(190.902650441443,0.566631063433394,
124.912696715504));
#225889=CARTESIAN_POINT('Ctrl Pts',(190.895252952107,0.409450827861063,
124.899693377976));
#225890=CARTESIAN_POINT('Ctrl Pts',(190.88785546277,0.252067249504715,124.892982380283));
#225891=CARTESIAN_POINT('Ctrl Pts',(190.880455380255,0.0946285005788653,
124.88626903006));
#225892=CARTESIAN_POINT('Ctrl Pts',(190.87305529774,-0.0630133603256108,
124.885852427237));
#225893=CARTESIAN_POINT('Ctrl Pts',(190.865655215225,-0.220318675722416,
124.891713981445));
#225894=CARTESIAN_POINT('Ctrl Pts',(190.858246995558,-0.377796964484852,
124.897581981035));
#225895=CARTESIAN_POINT('Ctrl Pts',(190.850838775892,-0.534937595424837,
124.909741910448));
#225896=CARTESIAN_POINT('Ctrl Pts',(190.843430556225,-0.691204991596928,
124.928123197065));
#225897=CARTESIAN_POINT('Ctrl Pts',(190.836017776923,-0.84756856774404,
124.946515797058));
#225898=CARTESIAN_POINT('Ctrl Pts',(190.828604997621,-1.00305747031484,
124.971137326051));
#225899=CARTESIAN_POINT('Ctrl Pts',(190.821192218319,-1.15714652449987,
125.001866112326));
#225900=CARTESIAN_POINT('Ctrl Pts',(190.81376884729,-1.31145574835155,125.032638805332));
#225901=CARTESIAN_POINT('Ctrl Pts',(190.806345476262,-1.46436076711051,
125.069536096735));
#225902=CARTESIAN_POINT('Ctrl Pts',(190.798922105233,-1.61535096541017,
125.112386283379));
#225903=CARTESIAN_POINT('Ctrl Pts',(190.794986055792,-1.69540959150786,
125.135106480513));
#225904=CARTESIAN_POINT('Ctrl Pts',(190.791050006351,-1.77493020547604,
125.15949943687));
#225905=CARTESIAN_POINT('Ctrl Pts',(190.787113956911,-1.85383911441731,
125.185534129735));
#225906=CARTESIAN_POINT('Ctrl Pts',(190.779690690505,-2.0026588540193,125.234634747963));
#225907=CARTESIAN_POINT('Ctrl Pts',(190.7722674241,-2.14975156694095,125.289726135378));
#225908=CARTESIAN_POINT('Ctrl Pts',(190.764844157694,-2.29459849424747,
125.350669361848));
#225909=CARTESIAN_POINT('Ctrl Pts',(190.757429664973,-2.4392742245148,125.411540558485));
#225910=CARTESIAN_POINT('Ctrl Pts',(190.750015172252,-2.58170911190695,
125.478249683713));
#225911=CARTESIAN_POINT('Ctrl Pts',(190.742600679531,-2.72139924075281,
125.550607983978));
#225912=CARTESIAN_POINT('Ctrl Pts',(190.735193333178,-2.86095473099336,
125.62289654259));
#225913=CARTESIAN_POINT('Ctrl Pts',(190.727785986824,-2.99777040011747,
125.700823265995));
#225914=CARTESIAN_POINT('Ctrl Pts',(190.72037864047,-3.13136212909958,125.784151281399));
#225915=CARTESIAN_POINT('Ctrl Pts',(190.712976818795,-3.26485422033005,
125.867417147625));
#225916=CARTESIAN_POINT('Ctrl Pts',(190.705574997119,-3.39512684380415,
125.956076087876));
#225917=CARTESIAN_POINT('Ctrl Pts',(190.698173175444,-3.5217204302287,126.049845313793));
#225918=CARTESIAN_POINT('Ctrl Pts',(190.690775261132,-3.6482471888842,126.143565039666));
#225919=CARTESIAN_POINT('Ctrl Pts',(190.683377346821,-3.77109847913389,
126.242389457018));
#225920=CARTESIAN_POINT('Ctrl Pts',(190.67597943251,-3.88984378373164,126.345992541614));
#225921=CARTESIAN_POINT('Ctrl Pts',(190.668582747597,-4.0085693550141,126.449578409258));
#225922=CARTESIAN_POINT('Ctrl Pts',(190.661186062685,-4.12319001387754,
126.557941122862));
#225923=CARTESIAN_POINT('Ctrl Pts',(190.653789377773,-4.23330833002912,
126.670714388701));
#225924=CARTESIAN_POINT('Ctrl Pts',(190.646393020838,-4.34342176341914,
126.783482654056));
#225925=CARTESIAN_POINT('Ctrl Pts',(190.638996663902,-4.44903299024769,
126.900660815703));
#225926=CARTESIAN_POINT('Ctrl Pts',(190.631600306967,-4.54978166812228,
127.021845933534));
#225927=CARTESIAN_POINT('Ctrl Pts',(190.62420281763,-4.65054577087687,127.143049605116));
#225928=CARTESIAN_POINT('Ctrl Pts',(190.616805328294,-4.7464456036807,127.268261167321));
#225929=CARTESIAN_POINT('Ctrl Pts',(190.609407838957,-4.83716142451464,
127.397044970948));
#225930=CARTESIAN_POINT('Ctrl Pts',(190.602007756442,-4.92790904563891,
127.525873919538));
#225931=CARTESIAN_POINT('Ctrl Pts',(190.594607673927,-5.01346882182785,
127.658277297765));
#225932=CARTESIAN_POINT('Ctrl Pts',(190.587207591412,-5.09356469563254,
127.793791027952));
#225933=CARTESIAN_POINT('Ctrl Pts',(190.579799371746,-5.17374864308446,
127.929453769417));
#225934=CARTESIAN_POINT('Ctrl Pts',(190.572391152079,-5.24845649947873,
128.068233371551));
#225935=CARTESIAN_POINT('Ctrl Pts',(190.564982932413,-5.31745814713684,
128.209641092078));
#225936=CARTESIAN_POINT('Ctrl Pts',(190.557570153111,-5.38650226415769,
128.351135846697));
#225937=CARTESIAN_POINT('Ctrl Pts',(190.550157373809,-5.44983302436487,
128.495261601939));
#225938=CARTESIAN_POINT('Ctrl Pts',(190.542744594507,-5.50726892380859,
128.641510746828));
#225939=CARTESIAN_POINT('Ctrl Pts',(190.535321223478,-5.56478689035895,
128.787968859353));
#225940=CARTESIAN_POINT('Ctrl Pts',(190.527897852449,-5.61639305166817,
128.9365560694));
#225941=CARTESIAN_POINT('Ctrl Pts',(190.52047448142,-5.66195586638615,129.086749972048));
#225942=CARTESIAN_POINT('Ctrl Pts',(190.516538431979,-5.68611436401442,
129.166386383086));
#225943=CARTESIAN_POINT('Ctrl Pts',(190.512602382539,-5.70857471323609,
129.246474316501));
#225944=CARTESIAN_POINT('Ctrl Pts',(190.508666333098,-5.72932318152839,
129.326935003837));
#225945=CARTESIAN_POINT('Ctrl Pts',(190.498971765574,-5.78042706879116,
129.525111266141));
#225946=CARTESIAN_POINT('Ctrl Pts',(190.48927719805,-5.82126881850071,129.726034303134));
#225947=CARTESIAN_POINT('Ctrl Pts',(190.479582630525,-5.85160626396125,
129.928783839625));
#225948=CARTESIAN_POINT('Ctrl Pts',(190.470087632604,-5.88131919141924,
130.127359631965));
#225949=CARTESIAN_POINT('Ctrl Pts',(190.460592634683,-5.90095589270113,
130.327687736164));
#225950=CARTESIAN_POINT('Ctrl Pts',(190.451097636761,-5.91033348368092,
130.528881627115));
#225951=CARTESIAN_POINT('Ctrl Pts',(190.446856827631,-5.91452185462971,
130.618742088053));
#225952=CARTESIAN_POINT('Ctrl Pts',(190.4426160185,-5.9166642962425,130.708774942494));
#225953=CARTESIAN_POINT('Ctrl Pts',(190.438375209369,-5.91674747976679,
130.798899557834));
#225954=CARTESIAN_POINT('',(193.938375192211,-5.91196518873725,130.809243212275));
#225955=CARTESIAN_POINT('Ctrl Pts',(193.938375192211,-5.91196518873725,
130.809243212275));
#225956=CARTESIAN_POINT('Ctrl Pts',(193.908929401091,-5.91681433885312,
131.435864751108));
#225957=CARTESIAN_POINT('Ctrl Pts',(193.78666773537,-5.53611148477146,134.031915457605));
#225958=CARTESIAN_POINT('Ctrl Pts',(193.571590195038,-1.75782624092181,
137.578399843691));
#225959=CARTESIAN_POINT('Ctrl Pts',(193.293142571227,4.74904303118782,135.944803285106));
#225960=CARTESIAN_POINT('Ctrl Pts',(193.014694947413,6.89177376128537,129.587391039638));
#225961=CARTESIAN_POINT('Ctrl Pts',(192.736247323601,2.70130108662762,124.348314384016));
#225962=CARTESIAN_POINT('Ctrl Pts',(192.46080781812,-3.8994475031143,125.034534503354));
#225963=CARTESIAN_POINT('Ctrl Pts',(192.278184187244,-5.92103596021112,
128.906232297951));
#225964=CARTESIAN_POINT('Ctrl Pts',(192.188376430972,-5.92624401559878,
130.805522386918));
#225965=CARTESIAN_POINT('',(195.688375192211,-5.90858988324653,130.801212225252));
#225966=CARTESIAN_POINT('Ctrl Pts',(195.688375192211,-5.90858988324653,
130.801212225252));
#225967=CARTESIAN_POINT('Ctrl Pts',(195.632491315384,-5.90286694115081,
131.992156895353));
#225968=CARTESIAN_POINT('Ctrl Pts',(195.483791563953,-4.97462506172764,
135.169312250667));
#225969=CARTESIAN_POINT('Ctrl Pts',(195.242275937916,0.216039013678407,
137.799422280975));
#225970=CARTESIAN_POINT('Ctrl Pts',(194.963828314104,6.00191785180767,134.403602569768));
#225971=CARTESIAN_POINT('Ctrl Pts',(194.685380690291,6.27232739411319,127.70025533723));
#225972=CARTESIAN_POINT('Ctrl Pts',(194.406933066478,0.778774481457,123.849429213348));
#225973=CARTESIAN_POINT('Ctrl Pts',(194.157931233786,-4.77381132895269,
126.121196694781));
#225974=CARTESIAN_POINT('Ctrl Pts',(194.001745275696,-5.90152936629919,
129.46069533092));
#225975=CARTESIAN_POINT('Ctrl Pts',(193.938375192211,-5.91196518873725,
130.809243212275));
#225976=CARTESIAN_POINT('',(197.438375192211,-5.92351700154912,130.800613675003));
#225977=CARTESIAN_POINT('Ctrl Pts',(197.438375192211,-5.92351700154912,
130.800613675003));
#225978=CARTESIAN_POINT('Ctrl Pts',(197.356053229677,-5.91065473800382,
132.543712972427));
#225979=CARTESIAN_POINT('Ctrl Pts',(197.180915392537,-4.17421686252449,
136.274385756281));
#225980=CARTESIAN_POINT('Ctrl Pts',(196.912961680794,2.17250297652081,137.457013573142));
#225981=CARTESIAN_POINT('Ctrl Pts',(196.634514056981,6.77135626959459,132.57249375751));
#225982=CARTESIAN_POINT('Ctrl Pts',(196.356066433169,5.14766395005485,126.063145964373));
#225983=CARTESIAN_POINT('Ctrl Pts',(196.077618809355,-1.20648006222068,
123.910742816309));
#225984=CARTESIAN_POINT('Ctrl Pts',(195.85505506237,-5.39917704206329,127.253819372125));
#225985=CARTESIAN_POINT('Ctrl Pts',(195.725307189988,-5.91237200604756,
130.014152192806));
#225986=CARTESIAN_POINT('Ctrl Pts',(195.688375192211,-5.90858988324653,
130.801212225252));
#225987=CARTESIAN_POINT('',(199.188375192211,-5.92038509218979,130.80931765918));
#225988=CARTESIAN_POINT('Ctrl Pts',(199.188375192211,-5.92038509218979,
130.80931765918));
#225989=CARTESIAN_POINT('Ctrl Pts',(199.172431018573,-5.92341887942187,
131.147387550494));
#225990=CARTESIAN_POINT('Ctrl Pts',(199.06367097033,-5.7429796640639,133.450227209526));
#225991=CARTESIAN_POINT('Ctrl Pts',(198.862095047485,-2.72093855833704,
137.252155115847));
#225992=CARTESIAN_POINT('Ctrl Pts',(198.583647423671,3.9539783690358,136.578753710139));
#225993=CARTESIAN_POINT('Ctrl Pts',(198.305199799859,6.99538233784591,130.598967147137));
#225994=CARTESIAN_POINT('Ctrl Pts',(198.026752176046,3.60837168160217,124.807927149431));
#225995=CARTESIAN_POINT('Ctrl Pts',(197.748304552233,-3.09455627127803,
124.527316566881));
#225996=CARTESIAN_POINT('Ctrl Pts',(197.552178890954,-5.81278598755467,
128.392589611084));
#225997=CARTESIAN_POINT('Ctrl Pts',(197.448869104281,-5.92515660607875,
130.578413788211));
#225998=CARTESIAN_POINT('Ctrl Pts',(197.438375192211,-5.92351700154912,
130.800613675003));
#225999=CARTESIAN_POINT('',(200.938375192211,-5.90723919874194,130.805767413591));
#226000=CARTESIAN_POINT('Ctrl Pts',(200.938375192211,-5.90723919874194,
130.805767413591));
#226001=CARTESIAN_POINT('Ctrl Pts',(200.895992932866,-5.90915334356233,
131.70949422463));
#226002=CARTESIAN_POINT('Ctrl Pts',(200.760794798915,-5.28885804543136,
134.58986393661));
#226003=CARTESIAN_POINT('Ctrl Pts',(200.532780790362,-0.799939293036777,
137.756889485374));
#226004=CARTESIAN_POINT('Ctrl Pts',(200.254333166548,5.41697271486199,135.235383878266));
#226005=CARTESIAN_POINT('Ctrl Pts',(199.975885542736,6.65595143161651,128.641984362081));
#226006=CARTESIAN_POINT('Ctrl Pts',(199.697437918923,1.77843594402775,124.035702986741));
#226007=CARTESIAN_POINT('Ctrl Pts',(199.434934468748,-4.36050283967217,
125.557080494142));
#226008=CARTESIAN_POINT('Ctrl Pts',(199.265246893177,-5.90575828303711,
129.179380091958));
#226009=CARTESIAN_POINT('Ctrl Pts',(199.188375192211,-5.92038509218979,
130.80931765918));
#226010=CARTESIAN_POINT('',(202.688375192211,-5.91520709160217,130.79891930971));
#226011=CARTESIAN_POINT('Ctrl Pts',(202.688375192211,-5.91520709160217,
130.79891930971));
#226012=CARTESIAN_POINT('Ctrl Pts',(202.619554847158,-5.90204591476485,
132.26141930917));
#226013=CARTESIAN_POINT('Ctrl Pts',(202.457918627501,-4.61506249001968,
135.717037067151));
#226014=CARTESIAN_POINT('Ctrl Pts',(202.203466533238,1.18549267223545,137.701618597998));
#226015=CARTESIAN_POINT('Ctrl Pts',(201.925018909427,6.44364622673833,133.535108470905));
#226016=CARTESIAN_POINT('Ctrl Pts',(201.646571285612,5.78040368780743,126.859174470383));
#226017=CARTESIAN_POINT('Ctrl Pts',(201.368123661802,-0.194747451439191,
123.808673806412));
#226018=CARTESIAN_POINT('Ctrl Pts',(201.132058297333,-5.10870273655874,
126.672675766875));
#226019=CARTESIAN_POINT('Ctrl Pts',(200.98880880747,-5.90496142391559,129.730359660658));
#226020=CARTESIAN_POINT('Ctrl Pts',(200.938375192211,-5.90723919874194,
130.805767413591));
#226021=CARTESIAN_POINT('',(204.438375192211,-5.92105141345348,130.805327648265));
#226022=CARTESIAN_POINT('Ctrl Pts',(204.438375192211,-5.92634035306676,
130.805328512059));
#226023=CARTESIAN_POINT('Ctrl Pts',(204.435932636055,-5.9264572190019,130.856982408026));
#226024=CARTESIAN_POINT('Ctrl Pts',(204.433490079899,-5.92584057372106,
130.908633442257));
#226025=CARTESIAN_POINT('Ctrl Pts',(204.338231649138,-5.87285210044721,
132.922235594029));
#226026=CARTESIAN_POINT('Ctrl Pts',(204.152599899928,-3.62660601729001,
136.789783698913));
#226027=CARTESIAN_POINT('Ctrl Pts',(203.874152276118,3.07543675800755,137.09079434209));
#226028=CARTESIAN_POINT('Ctrl Pts',(203.595704652303,6.95130345427144,131.614879558226));
#226029=CARTESIAN_POINT('Ctrl Pts',(203.317257028491,4.43926183532277,125.394137434058));
#226030=CARTESIAN_POINT('Ctrl Pts',(203.038809404678,-2.1522445239837,124.145126127266));
#226031=CARTESIAN_POINT('Ctrl Pts',(202.829182125918,-5.62563427618384,
127.811846704057));
#226032=CARTESIAN_POINT('Ctrl Pts',(202.712370721762,-5.91979598762536,
130.288990713325));
#226033=CARTESIAN_POINT('Ctrl Pts',(202.688375192211,-5.91520709160217,
130.79891930971));
#226034=CARTESIAN_POINT('',(206.188375157422,-5.91500286463066,130.809335122326));
#226035=CARTESIAN_POINT('Ctrl Pts',(206.188375135149,-5.91674790721062,
130.80933706396));
#226036=CARTESIAN_POINT('Ctrl Pts',(206.179566065341,-5.91659014051484,
130.996913839284));
#226037=CARTESIAN_POINT('Ctrl Pts',(206.170756995534,-5.90750858188079,
131.184105581818));
#226038=CARTESIAN_POINT('Ctrl Pts',(206.161947925727,-5.88963571160845,
131.370153642484));
#226039=CARTESIAN_POINT('Ctrl Pts',(206.153074186251,-5.87163163195439,
131.557567530276));
#226040=CARTESIAN_POINT('Ctrl Pts',(206.144200446775,-5.84470678641371,
131.74382085212));
#226041=CARTESIAN_POINT('Ctrl Pts',(206.135326707299,-5.80904529038186,
131.928159254686));
#226042=CARTESIAN_POINT('Ctrl Pts',(206.126381804847,-5.77309780689119,
132.113975959543));
#226043=CARTESIAN_POINT('Ctrl Pts',(206.117436902394,-5.72827303913071,
132.297846882214));
#226044=CARTESIAN_POINT('Ctrl Pts',(206.108491999942,-5.67480770886274,
132.479021189124));
#226045=CARTESIAN_POINT('Ctrl Pts',(206.106239088835,-5.66134164402378,
132.524652721779));
#226046=CARTESIAN_POINT('Ctrl Pts',(206.103986177728,-5.64732768966758,
132.570113299786));
#226047=CARTESIAN_POINT('Ctrl Pts',(206.101733266621,-5.63277009911369,
132.615391145478));
#226048=CARTESIAN_POINT('Ctrl Pts',(206.094310026419,-5.58480349665586,
132.764579599188));
#226049=CARTESIAN_POINT('Ctrl Pts',(206.086886786216,-5.53083319938669,
132.91208669215));
#226050=CARTESIAN_POINT('Ctrl Pts',(206.079463546014,-5.47099418136574,
133.057392625763));
#226051=CARTESIAN_POINT('Ctrl Pts',(206.072049079851,-5.41122589119732,
133.202526812296));
#226052=CARTESIAN_POINT('Ctrl Pts',(206.064634613687,-5.34560282846522,
133.345464676374));
#226053=CARTESIAN_POINT('Ctrl Pts',(206.057220147523,-5.274309902267,133.485700882685));
#226054=CARTESIAN_POINT('Ctrl Pts',(206.049812828053,-5.20308569425869,
133.625801917405));
#226055=CARTESIAN_POINT('Ctrl Pts',(206.042405508582,-5.12620267075052,
133.763206148049));
#226056=CARTESIAN_POINT('Ctrl Pts',(206.034998189112,-5.04389400946855,
133.897427668851));
#226057=CARTESIAN_POINT('Ctrl Pts',(206.027596394619,-4.96164674063805,
134.031549076396));
#226058=CARTESIAN_POINT('Ctrl Pts',(206.020194600126,-4.87398208622341,
134.162492184038));
#226059=CARTESIAN_POINT('Ctrl Pts',(206.012792805633,-4.78117932515222,
134.289795285328));
#226060=CARTESIAN_POINT('Ctrl Pts',(206.005394918777,-4.68842555753051,
134.417031179371));
#226061=CARTESIAN_POINT('Ctrl Pts',(205.99799703192,-4.59053930480269,134.540630593273));
#226062=CARTESIAN_POINT('Ctrl Pts',(205.990599145064,-4.48784330175735,
134.660160542533));
#226063=CARTESIAN_POINT('Ctrl Pts',(205.983202487927,-4.38516436944237,
134.779670622824));
#226064=CARTESIAN_POINT('Ctrl Pts',(205.975805830791,-4.27767751662466,
134.895112298157));
#226065=CARTESIAN_POINT('Ctrl Pts',(205.968409173654,-4.16574599834706,
135.0060853634));
#226066=CARTESIAN_POINT('Ctrl Pts',(205.961012844691,-4.05381944622384,
135.117053505014));
#226067=CARTESIAN_POINT('Ctrl Pts',(205.953616515728,-3.93744888583708,
135.223553167924));
#226068=CARTESIAN_POINT('Ctrl Pts',(205.946220186765,-3.81703449993298,
135.325220954805));
#226069=CARTESIAN_POINT('Ctrl Pts',(205.938822725573,-3.69660168102824,
135.426904304962));
#226070=CARTESIAN_POINT('Ctrl Pts',(205.931425264382,-3.5721240892894,135.523754065483));
#226071=CARTESIAN_POINT('Ctrl Pts',(205.924027803191,-3.44403492469912,
135.61544718922));
#226072=CARTESIAN_POINT('Ctrl Pts',(205.916627748971,-3.31590086107405,
135.707172454105));
#226073=CARTESIAN_POINT('Ctrl Pts',(205.909227694752,-3.18415300742791,
135.793737266225));
#226074=CARTESIAN_POINT('Ctrl Pts',(205.901827640532,-3.04925332393586,
135.874862045331));
#226075=CARTESIAN_POINT('Ctrl Pts',(205.894419449247,-2.9142053053851,135.956076028864));
#226076=CARTESIAN_POINT('Ctrl Pts',(205.887011257962,-2.77599885578924,
136.031837840764));
#226077=CARTESIAN_POINT('Ctrl Pts',(205.879603066678,-2.63512094888712,
136.10191365149));
#226078=CARTESIAN_POINT('Ctrl Pts',(205.872190315849,-2.49415633539396,
136.172032592006));
#226079=CARTESIAN_POINT('Ctrl Pts',(205.864777565021,-2.35051732811826,
136.236458405575));
#226080=CARTESIAN_POINT('Ctrl Pts',(205.857364814192,-2.20471013894131,
136.295005731371));
#226081=CARTESIAN_POINT('Ctrl Pts',(205.849941471535,-2.05869461081846,
136.353636713455));
#226082=CARTESIAN_POINT('Ctrl Pts',(205.842518128878,-1.91050506407407,
136.406372307113));
#226083=CARTESIAN_POINT('Ctrl Pts',(205.835094786222,-1.76066288435223,
136.453077000087));
#226084=CARTESIAN_POINT('Ctrl Pts',(205.831158405083,-1.68120596618447,
136.477843130523));
#226085=CARTESIAN_POINT('Ctrl Pts',(205.827222023945,-1.60128453480154,
136.500914311524));
#226086=CARTESIAN_POINT('Ctrl Pts',(205.823285642806,-1.5209772722179,136.52227620805));
#226087=CARTESIAN_POINT('Ctrl Pts',(205.815862363887,-1.36953278846232,
136.562560751281));
#226088=CARTESIAN_POINT('Ctrl Pts',(205.808439084968,-1.21625774237482,
136.596885322964));
#226089=CARTESIAN_POINT('Ctrl Pts',(205.801015806049,-1.06166241873887,
136.625082520486));
#226090=CARTESIAN_POINT('Ctrl Pts',(205.793601300696,-0.907249811172222,
136.653246391767));
#226091=CARTESIAN_POINT('Ctrl Pts',(205.786186795344,-0.751520395763363,
136.675297237676));
#226092=CARTESIAN_POINT('Ctrl Pts',(205.778772289991,-0.594999279427515,
136.691117485314));
#226093=CARTESIAN_POINT('Ctrl Pts',(205.771364930901,-0.438629021562489,
136.706922485052));
#226094=CARTESIAN_POINT('Ctrl Pts',(205.76395757181,-0.281468950781068,
136.716508804378));
#226095=CARTESIAN_POINT('Ctrl Pts',(205.75655021272,-0.124053917183144,
136.719809982418));
#226096=CARTESIAN_POINT('Ctrl Pts',(205.749148378216,0.0332437125062621,
136.723108698361));
#226097=CARTESIAN_POINT('Ctrl Pts',(205.741746543712,0.190795554774945,
136.720131598888));
#226098=CARTESIAN_POINT('Ctrl Pts',(205.734344709207,0.348062200778197,
136.710864089747));
#226099=CARTESIAN_POINT('Ctrl Pts',(205.726946781988,0.505245828778614,
136.701601472745));
#226100=CARTESIAN_POINT('Ctrl Pts',(205.719548854768,0.662144188633564,
136.686055081083));
#226101=CARTESIAN_POINT('Ctrl Pts',(205.712150927548,0.818218547581937,
136.664262406068));
#226102=CARTESIAN_POINT('Ctrl Pts',(205.704754229649,0.97426697149117,136.642473352365));
#226103=CARTESIAN_POINT('Ctrl Pts',(205.697357531751,1.12949129690173,136.614440126908));
#226104=CARTESIAN_POINT('Ctrl Pts',(205.689960833853,1.28335846744775,136.580252029853));
#226105=CARTESIAN_POINT('Ctrl Pts',(205.682564463884,1.43721881635304,136.546065448514));
#226106=CARTESIAN_POINT('Ctrl Pts',(205.675168093915,1.5897217656208,136.505724619111));
#226107=CARTESIAN_POINT('Ctrl Pts',(205.667771723946,1.74034526633639,136.459369805573));
#226108=CARTESIAN_POINT('Ctrl Pts',(205.66037422154,1.89099182858503,136.413007894781));
#226109=CARTESIAN_POINT('Ctrl Pts',(205.652976719135,2.03975801251326,136.360630276258));
#226110=CARTESIAN_POINT('Ctrl Pts',(205.645579216729,2.18613787059475,136.30242680244));
#226111=CARTESIAN_POINT('Ctrl Pts',(205.63817912112,2.3325690423081,136.244202925325));
#226112=CARTESIAN_POINT('Ctrl Pts',(205.630779025511,2.47661187598612,136.180149264629));
#226113=CARTESIAN_POINT('Ctrl Pts',(205.623378929902,2.61778144864533,136.110503364386));
#226114=CARTESIAN_POINT('Ctrl Pts',(205.61597069717,2.75910625094721,136.040780881718));
#226115=CARTESIAN_POINT('Ctrl Pts',(205.608562464438,2.89755114766472,135.965454044387));
#226116=CARTESIAN_POINT('Ctrl Pts',(205.601154231705,3.03265618688166,135.884806170337));
#226117=CARTESIAN_POINT('Ctrl Pts',(205.593741439334,3.16784438091394,135.804108658914));
#226118=CARTESIAN_POINT('Ctrl Pts',(205.586328646963,3.29968830944655,135.718083788424));
#226119=CARTESIAN_POINT('Ctrl Pts',(205.578915854592,3.4277584000582,135.627057260869));
#226120=CARTESIAN_POINT('Ctrl Pts',(205.571492470601,3.55601148104427,135.535900671891));
#226121=CARTESIAN_POINT('Ctrl Pts',(205.56406908661,3.68047966012121,135.439728380284));
#226122=CARTESIAN_POINT('Ctrl Pts',(205.55664570262,3.80076710215312,135.338905798473));
#226123=CARTESIAN_POINT('Ctrl Pts',(205.552709808078,3.86454376885181,135.285449443535));
#226124=CARTESIAN_POINT('Ctrl Pts',(205.548773913536,3.92714579463605,135.230686447014));
#226125=CARTESIAN_POINT('Ctrl Pts',(205.544838018994,3.98851860995265,135.174675235595));
#226126=CARTESIAN_POINT('Ctrl Pts',(205.537414752403,4.10427038243128,135.069035678946));
#226127=CARTESIAN_POINT('Ctrl Pts',(205.529991485813,4.21599734533866,134.958634520244));
#226128=CARTESIAN_POINT('Ctrl Pts',(205.522568219222,4.32328283706097,134.843810589193));
#226129=CARTESIAN_POINT('Ctrl Pts',(205.515153726284,4.43044152670348,134.729122369998));
#226130=CARTESIAN_POINT('Ctrl Pts',(205.507739233346,4.53316894181514,134.610022053583));
#226131=CARTESIAN_POINT('Ctrl Pts',(205.500324740408,4.63108233208609,134.486887874212));
#226132=CARTESIAN_POINT('Ctrl Pts',(205.492917393806,4.7289013501625,134.363872375674));
#226133=CARTESIAN_POINT('Ctrl Pts',(205.485510047204,4.82191534978399,134.236831044588));
#226134=CARTESIAN_POINT('Ctrl Pts',(205.478102700602,4.90977931610782,134.106177939833));
#226135=CARTESIAN_POINT('Ctrl Pts',(205.470700878647,4.99757775054161,133.975622280541));
#226136=CARTESIAN_POINT('Ctrl Pts',(205.463299056693,5.08023359234056,133.841460519697));
#226137=CARTESIAN_POINT('Ctrl Pts',(205.455897234738,5.15744299933014,133.704138586853));
#226138=CARTESIAN_POINT('Ctrl Pts',(205.448499320116,5.23461164839757,133.566889144614));
#226139=CARTESIAN_POINT('Ctrl Pts',(205.441101405494,5.30633940608169,133.426483177278));
#226140=CARTESIAN_POINT('Ctrl Pts',(205.433703490873,5.37236661664779,133.283394199192));
#226141=CARTESIAN_POINT('Ctrl Pts',(205.426306805605,5.4383828550952,133.140328999019));
#226142=CARTESIAN_POINT('Ctrl Pts',(205.418910120337,5.49870027026613,132.994582011598));
#226143=CARTESIAN_POINT('Ctrl Pts',(205.411513435069,5.55310586287155,132.846649979591));
#226144=CARTESIAN_POINT('Ctrl Pts',(205.40411707775,5.60750904328352,132.698724506482));
#226145=CARTESIAN_POINT('Ctrl Pts',(205.396720720431,5.6560007934494,132.548614531768));
#226146=CARTESIAN_POINT('Ctrl Pts',(205.389324363111,5.6984169411165,132.396835084456));
#226147=CARTESIAN_POINT('Ctrl Pts',(205.381926873363,5.74083958296442,132.245032398749));
#226148=CARTESIAN_POINT('Ctrl Pts',(205.374529383615,5.77718466965693,132.091560091043));
#226149=CARTESIAN_POINT('Ctrl Pts',(205.367131893866,5.80733845234025,131.936946447634));
#226150=CARTESIAN_POINT('Ctrl Pts',(205.359731810911,5.83750280549823,131.782278604073));
#226151=CARTESIAN_POINT('Ctrl Pts',(205.352331727957,5.8614714620337,131.626468994384));
#226152=CARTESIAN_POINT('Ctrl Pts',(205.344931645002,5.87918216165979,131.470053994821));
#226153=CARTESIAN_POINT('Ctrl Pts',(205.337523424855,5.89691233611661,131.313467000041));
#226154=CARTESIAN_POINT('Ctrl Pts',(205.330115204709,5.90837076922905,131.156273657112));
#226155=CARTESIAN_POINT('Ctrl Pts',(205.322706984562,5.91354720906745,130.999014075358));
#226156=CARTESIAN_POINT('Ctrl Pts',(205.315294204756,5.91872683493454,130.84165770246));
#226157=CARTESIAN_POINT('Ctrl Pts',(205.30788142495,5.91761676570394,130.684235381923));
#226158=CARTESIAN_POINT('Ctrl Pts',(205.300468645144,5.91025882921648,130.527284573548));
#226159=CARTESIAN_POINT('Ctrl Pts',(205.293045273578,5.90289037933228,130.370109505815));
#226160=CARTESIAN_POINT('Ctrl Pts',(205.285621902013,5.88925626469626,130.213407666724));
#226161=CARTESIAN_POINT('Ctrl Pts',(205.278198530447,5.86944995847761,130.057709596387));
#226162=CARTESIAN_POINT('Ctrl Pts',(205.274262485358,5.85894819204549,129.975154840818));
#226163=CARTESIAN_POINT('Ctrl Pts',(205.270326440269,5.84671205599,129.892882092421));
#226164=CARTESIAN_POINT('Ctrl Pts',(205.266390395181,5.8327612125786,129.810968852179));
#226165=CARTESIAN_POINT('Ctrl Pts',(205.258967132391,5.80645034102074,129.656482941948));
#226166=CARTESIAN_POINT('Ctrl Pts',(205.251543869601,5.77395789796265,129.502809451314));
#226167=CARTESIAN_POINT('Ctrl Pts',(205.244120606812,5.73534373383937,129.350482074768));
#226168=CARTESIAN_POINT('Ctrl Pts',(205.236706117758,5.69677520874019,129.198334737669));
#226169=CARTESIAN_POINT('Ctrl Pts',(205.229291628704,5.65209945553443,129.047530706073));
#226170=CARTESIAN_POINT('Ctrl Pts',(205.22187713965,5.60142780672731,128.898596443141));
#226171=CARTESIAN_POINT('Ctrl Pts',(205.214469797011,5.55080499751139,128.749805729682));
#226172=CARTESIAN_POINT('Ctrl Pts',(205.207062454371,5.49419791719723,128.602881548161));
#226173=CARTESIAN_POINT('Ctrl Pts',(205.199655111732,5.43176843551374,128.458337977979));
#226174=CARTESIAN_POINT('Ctrl Pts',(205.192253293815,5.36938551648445,128.313902214751));
#226175=CARTESIAN_POINT('Ctrl Pts',(205.184851475898,5.30118899017215,128.171843868699));
#226176=CARTESIAN_POINT('Ctrl Pts',(205.17744965798,5.22738979486144,128.03265960644));
#226177=CARTESIAN_POINT('Ctrl Pts',(205.170051747467,5.15362955798969,127.893548819258));
#226178=CARTESIAN_POINT('Ctrl Pts',(205.162653836954,5.07427271682429,127.757309423218));
#226179=CARTESIAN_POINT('Ctrl Pts',(205.155255926441,4.98957730139766,127.624415819951));
#226180=CARTESIAN_POINT('Ctrl Pts',(205.147859245375,4.90489596136757,127.491544302061));
#226181=CARTESIAN_POINT('Ctrl Pts',(205.140462564308,4.81487800835612,127.362017787878));
#226182=CARTESIAN_POINT('Ctrl Pts',(205.133065883242,4.7198262340098,127.236283981162));
#226183=CARTESIAN_POINT('Ctrl Pts',(205.125669530182,4.62477867473806,127.110555750117));
#226184=CARTESIAN_POINT('Ctrl Pts',(205.118273177122,4.52469796309431,126.988620189907));
#226185=CARTESIAN_POINT('Ctrl Pts',(205.110876824062,4.41992866778351,126.870893808985));
#226186=CARTESIAN_POINT('Ctrl Pts',(205.103479338627,4.31514333238748,126.753149404261));
#226187=CARTESIAN_POINT('Ctrl Pts',(205.096081853192,4.20566823223877,126.639615740833));
#226188=CARTESIAN_POINT('Ctrl Pts',(205.088684367756,4.0918863448901,126.53067407045));
#226189=CARTESIAN_POINT('Ctrl Pts',(205.081284289166,3.97806457180816,126.42169421105));
#226190=CARTESIAN_POINT('Ctrl Pts',(205.073884210575,3.85993327514114,126.317309807603));
#226191=CARTESIAN_POINT('Ctrl Pts',(205.066484131984,3.73791006961344,126.217863165917));
#226192=CARTESIAN_POINT('Ctrl Pts',(205.059075916258,3.61575268720724,126.118307172572));
#226193=CARTESIAN_POINT('Ctrl Pts',(205.051667700531,3.48969513894966,126.02370002017));
#226194=CARTESIAN_POINT('Ctrl Pts',(205.044259484804,3.36018629211852,125.93434227625));
#226195=CARTESIAN_POINT('Ctrl Pts',(205.036846709456,3.23059773496496,125.844929534275));
#226196=CARTESIAN_POINT('Ctrl Pts',(205.029433934108,3.09755396123104,125.76077283788));
#226197=CARTESIAN_POINT('Ctrl Pts',(205.02202115876,2.9615297594948,125.682127506302));
#226198=CARTESIAN_POINT('Ctrl Pts',(205.014597791674,2.82531119969063,125.603369802408));
#226199=CARTESIAN_POINT('Ctrl Pts',(205.007174424588,2.68610403603951,125.530139364625));
#226200=CARTESIAN_POINT('Ctrl Pts',(204.999751057502,2.5444051509773,125.462644321264));
#226201=CARTESIAN_POINT('Ctrl Pts',(204.995814962124,2.46927208532876,125.42685639307));
#226202=CARTESIAN_POINT('Ctrl Pts',(204.991878866746,2.39343879236606,125.39268011218));
#226203=CARTESIAN_POINT('Ctrl Pts',(204.987942771368,2.31698110677334,125.360140828344));
#226204=CARTESIAN_POINT('Ctrl Pts',(204.980519502944,2.17278594159917,125.298773454077));
#226205=CARTESIAN_POINT('Ctrl Pts',(204.97309623452,2.02593299682858,125.243045954815));
#226206=CARTESIAN_POINT('Ctrl Pts',(204.965672966097,1.87690363642786,125.193196451186));
#226207=CARTESIAN_POINT('Ctrl Pts',(204.958258471337,1.7280504158966,125.143405865378));
#226208=CARTESIAN_POINT('Ctrl Pts',(204.950843976577,1.57702625054469,125.099479563857));
#226209=CARTESIAN_POINT('Ctrl Pts',(204.943429481818,1.42433424764934,125.061608445177));
#226210=CARTESIAN_POINT('Ctrl Pts',(204.936022133407,1.27178941463677,125.023773828004));
#226211=CARTESIAN_POINT('Ctrl Pts',(204.928614784996,1.11758030422428,124.991982864216));
#226212=CARTESIAN_POINT('Ctrl Pts',(204.921207436585,0.962226921405626,
124.966377240215));
#226213=CARTESIAN_POINT('Ctrl Pts',(204.913805612837,0.80698940662729,124.940790713794));
#226214=CARTESIAN_POINT('Ctrl Pts',(204.906403789088,0.650609685497499,
124.921380402016));
#226215=CARTESIAN_POINT('Ctrl Pts',(204.899001965339,0.493619635819424,
124.908237296465));
#226216=CARTESIAN_POINT('Ctrl Pts',(204.89160404894,0.336712459641496,124.89510112903));
#226217=CARTESIAN_POINT('Ctrl Pts',(204.884206132541,0.179195967619653,
124.888225610057));
#226218=CARTESIAN_POINT('Ctrl Pts',(204.876808216143,0.0216087595666902,
124.887650076733));
#226219=CARTESIAN_POINT('Ctrl Pts',(204.869411529128,-0.135952260670864,
124.88707463905));
#226220=CARTESIAN_POINT('Ctrl Pts',(204.862014842114,-0.293583600686453,
124.89279711053));
#226221=CARTESIAN_POINT('Ctrl Pts',(204.854618155099,-0.450744927651624,
124.90480473829));
#226222=CARTESIAN_POINT('Ctrl Pts',(204.847221796053,-0.607899286109743,
124.916811833635));
#226223=CARTESIAN_POINT('Ctrl Pts',(204.839825437006,-0.764583300742472,
124.935103502707));
#226224=CARTESIAN_POINT('Ctrl Pts',(204.83242907796,-0.920260302747,124.95961498258));
#226225=CARTESIAN_POINT('Ctrl Pts',(204.825031586505,-1.07596113944049,
124.984130215246));
#226226=CARTESIAN_POINT('Ctrl Pts',(204.81763409505,-1.23065428774014,125.014867096753));
#226227=CARTESIAN_POINT('Ctrl Pts',(204.810236603595,-1.38381198042967,
125.051709492622));
#226228=CARTESIAN_POINT('Ctrl Pts',(204.802836518957,-1.53702336240519,
125.088564803558));
#226229=CARTESIAN_POINT('Ctrl Pts',(204.795436434318,-1.68869785439576,
125.131529802889));
#226230=CARTESIAN_POINT('Ctrl Pts',(204.78803634968,-1.83832173330245,125.180438163676));
#226231=CARTESIAN_POINT('Ctrl Pts',(204.780628127893,-1.98811013894526,
125.229400304201));
#226232=CARTESIAN_POINT('Ctrl Pts',(204.773219906105,-2.13584307336326,
125.284318741618));
#226233=CARTESIAN_POINT('Ctrl Pts',(204.765811684318,-2.2810250362999,125.344978294787));
#226234=CARTESIAN_POINT('Ctrl Pts',(204.758398902893,-2.42629635631982,
125.405675182902));
#226235=CARTESIAN_POINT('Ctrl Pts',(204.750986121469,-2.56901323864276,
125.47212007064));
#226236=CARTESIAN_POINT('Ctrl Pts',(204.743573340044,-2.70870424060689,
125.544051510734));
#226237=CARTESIAN_POINT('Ctrl Pts',(204.736149966909,-2.84859483927297,
125.616085729662));
#226238=CARTESIAN_POINT('Ctrl Pts',(204.728726593773,-2.98545059862428,
125.693621974519));
#226239=CARTESIAN_POINT('Ctrl Pts',(204.721303220637,-3.11882783680492,
125.77635470201));
#226240=CARTESIAN_POINT('Ctrl Pts',(204.717367196277,-3.18954717814477,
125.820221287307));
#226241=CARTESIAN_POINT('Ctrl Pts',(204.713431171916,-3.25928911964002,
125.865548075032));
#226242=CARTESIAN_POINT('Ctrl Pts',(204.709495147555,-3.3279913467505,125.912284968268));
#226243=CARTESIAN_POINT('Ctrl Pts',(204.702104411593,-3.45699461857756,
126.000043580996));
#226244=CARTESIAN_POINT('Ctrl Pts',(204.694713675631,-3.58272775527118,
126.093046915379));
#226245=CARTESIAN_POINT('Ctrl Pts',(204.68732293967,-3.70473253445668,126.191022627494));
#226246=CARTESIAN_POINT('Ctrl Pts',(204.679940958213,-3.82659279604236,
126.288882285019));
#226247=CARTESIAN_POINT('Ctrl Pts',(204.672558976756,-3.94473319850045,
126.391702364622));
#226248=CARTESIAN_POINT('Ctrl Pts',(204.665176995299,-4.05872330506565,
126.499166580659));
#226249=CARTESIAN_POINT('Ctrl Pts',(204.657802110667,-4.17260382482097,
126.60652748369));
#226250=CARTESIAN_POINT('Ctrl Pts',(204.650427226035,-4.28234171832161,
126.71852337928));
#226251=CARTESIAN_POINT('Ctrl Pts',(204.643052341403,-4.38753867962024,
126.83479705247));
#226252=CARTESIAN_POINT('Ctrl Pts',(204.635682901836,-4.49265797131831,
126.950984877841));
#226253=CARTESIAN_POINT('Ctrl Pts',(204.628313462269,-4.59324275370197,
127.071443914587));
#226254=CARTESIAN_POINT('Ctrl Pts',(204.620944022703,-4.68893086223868,
127.195779465417));
#226255=CARTESIAN_POINT('Ctrl Pts',(204.613336988099,-4.78770401129907,
127.324123667047));
#226256=CARTESIAN_POINT('Ctrl Pts',(204.605729953495,-4.88125914129115,
127.45659826124));
#226257=CARTESIAN_POINT('Ctrl Pts',(204.598122918891,-4.96924186267879,
127.592730833064));
#226258=CARTESIAN_POINT('Ctrl Pts',(204.590758398115,-5.05441967681546,
127.724523470504));
#226259=CARTESIAN_POINT('Ctrl Pts',(204.583393877339,-5.13437472757324,
127.859744080796));
#226260=CARTESIAN_POINT('Ctrl Pts',(204.576029356562,-5.20882895299715,
127.997933796692));
#226261=CARTESIAN_POINT('Ctrl Pts',(204.568664962593,-5.283281896423,128.136121133155));
#226262=CARTESIAN_POINT('Ctrl Pts',(204.561300568623,-5.35223402382612,
128.277277141798));
#226263=CARTESIAN_POINT('Ctrl Pts',(204.553936174654,-5.41545310427121,
128.420918099287));
#226264=CARTESIAN_POINT('Ctrl Pts',(204.54657042013,-5.47868386429348,128.564585594107));
#226265=CARTESIAN_POINT('Ctrl Pts',(204.539204665606,-5.53617931718692,
128.710738606591));
#226266=CARTESIAN_POINT('Ctrl Pts',(204.531838911082,-5.58775535548524,
128.858873365039));
#226267=CARTESIAN_POINT('Ctrl Pts',(204.524470308052,-5.63935133941324,
129.007065410574));
#226268=CARTESIAN_POINT('Ctrl Pts',(204.517101705023,-5.68502322819046,
129.157240371933));
#226269=CARTESIAN_POINT('Ctrl Pts',(204.509733101994,-5.7246368129675,129.308879450143));
#226270=CARTESIAN_POINT('Ctrl Pts',(204.502356410778,-5.76429387980796,
129.460684975799));
#226271=CARTESIAN_POINT('Ctrl Pts',(204.494979719562,-5.79787927133109,
129.613957462062));
#226272=CARTESIAN_POINT('Ctrl Pts',(204.487603028346,-5.82530980176946,
129.768167452221));
#226273=CARTESIAN_POINT('Ctrl Pts',(204.480221494494,-5.85275833974991,
129.922478677858));
#226274=CARTESIAN_POINT('Ctrl Pts',(204.472839960642,-5.87404391676752,
130.077728261269));
#226275=CARTESIAN_POINT('Ctrl Pts',(204.465458426791,-5.88913528604936,
130.233382382334));
#226276=CARTESIAN_POINT('Ctrl Pts',(204.458067024258,-5.90424683161207,
130.389244603885));
#226277=CARTESIAN_POINT('Ctrl Pts',(204.450675621726,-5.91314761819259,
130.545512068223));
#226278=CARTESIAN_POINT('Ctrl Pts',(204.443284219194,-5.91585846087386,
130.701651156428));
#226279=CARTESIAN_POINT('Ctrl Pts',(204.441647876866,-5.91645859956244,
130.736217938293));
#226280=CARTESIAN_POINT('Ctrl Pts',(204.440011534539,-5.91675556357633,
130.770778450004));
#226281=CARTESIAN_POINT('Ctrl Pts',(204.438375192211,-5.91674992108927,
130.805326945742));
#226282=CARTESIAN_POINT('',(207.300060471638,3.90699806772732,135.242283170684));
#226283=CARTESIAN_POINT('Ctrl Pts',(207.300060471638,3.90699806772668,135.242283170685));
#226284=CARTESIAN_POINT('Ctrl Pts',(207.271881568382,4.36049763724443,134.850189658193));
#226285=CARTESIAN_POINT('Ctrl Pts',(207.150886790522,6.05211717572361,132.884390582407));
#226286=CARTESIAN_POINT('Ctrl Pts',(206.937076138059,6.29112482667552,127.7385118325));
#226287=CARTESIAN_POINT('Ctrl Pts',(206.658628514245,0.821087121814331,
123.854289400871));
#226288=CARTESIAN_POINT('Ctrl Pts',(206.409061532297,-4.75784521223805,
126.09730669271));
#226289=CARTESIAN_POINT('Ctrl Pts',(206.252310424952,-5.90151704252715,
129.448939722285));
#226290=CARTESIAN_POINT('Ctrl Pts',(206.188375192211,-5.91227720962736,
130.809332089608));
#226291=CARTESIAN_POINT('Ctrl Pts',(207.097092794244,3.07160564976241,135.861352736884));
#226292=CARTESIAN_POINT('Ctrl Pts',(207.16165438619,3.37382896112027,135.677782976688));
#226293=CARTESIAN_POINT('Ctrl Pts',(207.23109396594,3.65610320797724,135.468837830569));
#226294=CARTESIAN_POINT('Ctrl Pts',(207.299797282174,3.91217312619061,135.243147838555));
#226295=CARTESIAN_POINT('Origin',(210.,0.,130.804360617566));
#226296=CARTESIAN_POINT('',(207.956496781212,-5.9049774143355,130.419651541055));
#226297=CARTESIAN_POINT('Ctrl Pts',(207.794825763995,-5.47599840541864,
128.563518805578));
#226298=CARTESIAN_POINT('Ctrl Pts',(207.883706865838,-5.72070422757077,
129.161512240337));
#226299=CARTESIAN_POINT('Ctrl Pts',(207.940449287037,-5.86515699931026,
129.80416200646));
#226300=CARTESIAN_POINT('Ctrl Pts',(207.955834607772,-5.90485866211524,
130.429427632964));
#226301=CARTESIAN_POINT('',(207.851560096186,-5.62714347058183,132.623000814592));
#226302=CARTESIAN_POINT('Ctrl Pts',(207.851491355655,-5.63013302498849,
132.623572722691));
#226303=CARTESIAN_POINT('Ctrl Pts',(207.832959583949,-5.58032197094584,
132.77772894207));
#226304=CARTESIAN_POINT('Ctrl Pts',(207.812258447827,-5.52411769153045,
132.929986067143));
#226305=CARTESIAN_POINT('Ctrl Pts',(207.709562033561,-5.24073952453561,
133.610284849743));
#226306=CARTESIAN_POINT('Ctrl Pts',(207.605087833971,-4.94084622400808,
134.106396899339));
#226307=CARTESIAN_POINT('Ctrl Pts',(207.49642148088,-4.59106392006869,134.53666053107));
#226308=CARTESIAN_POINT('',(207.938375235231,-5.91423241434992,130.80143089854));
#226309=CARTESIAN_POINT('Ctrl Pts',(207.938375192211,-5.90834445110727,
130.801434732496));
#226310=CARTESIAN_POINT('Ctrl Pts',(207.909436826869,-5.90555594570905,
131.418178106961));
#226311=CARTESIAN_POINT('Ctrl Pts',(207.880498461528,-5.81083010793395,
132.035697025576));
#226312=CARTESIAN_POINT('Ctrl Pts',(207.851560096186,-5.62714347058182,
132.623000814592));
#226313=CARTESIAN_POINT('Ctrl Pts',(207.956549707745,-5.9038746591298,130.414239390529));
#226314=CARTESIAN_POINT('Ctrl Pts',(207.95049155637,-5.91238172765814,130.542980568468));
#226315=CARTESIAN_POINT('Ctrl Pts',(207.944433404995,-5.91668521597131,
130.672132721857));
#226316=CARTESIAN_POINT('Ctrl Pts',(207.938375253621,-5.91674927385308,
130.801429259683));
#226317=CARTESIAN_POINT('Ctrl Pts',(210.579426101437,-2.14555810197798,
126.384433368448));
#226318=CARTESIAN_POINT('Ctrl Pts',(210.533016425084,-2.88204635455982,
126.741945114569));
#226319=CARTESIAN_POINT('Ctrl Pts',(210.440198811428,-4.16073755837059,
127.832228156677));
#226320=CARTESIAN_POINT('Ctrl Pts',(210.254565323169,-5.41774734084591,
130.983824311839));
#226321=CARTESIAN_POINT('Ctrl Pts',(210.022525636658,-3.70466367662459,
135.280954889074));
#226322=CARTESIAN_POINT('Ctrl Pts',(209.744078012845,1.77278938863763,136.341871604603));
#226323=CARTESIAN_POINT('Ctrl Pts',(209.465630389032,5.61248518735455,132.305536381355));
#226324=CARTESIAN_POINT('Ctrl Pts',(209.187182765219,4.2990952821384,126.894094626803));
#226325=CARTESIAN_POINT('Ctrl Pts',(208.908735141406,-0.967335548355457,
125.073681250508));
#226326=CARTESIAN_POINT('Ctrl Pts',(208.630287517594,-5.34357155608916,
128.520706403956));
#226327=CARTESIAN_POINT('Ctrl Pts',(208.351839893781,-4.80999390579215,
134.065650134797));
#226328=CARTESIAN_POINT('Ctrl Pts',(208.073392269968,0.144086686833323,
136.613971320579));
#226329=CARTESIAN_POINT('Ctrl Pts',(207.794944646155,4.96557142732685,133.823362329787));
#226330=CARTESIAN_POINT('Ctrl Pts',(207.516497022342,5.22403776314189,128.258534510045));
#226331=CARTESIAN_POINT('Ctrl Pts',(207.238049398529,0.681816090004523,
125.033145533949));
#226332=CARTESIAN_POINT('Ctrl Pts',(206.959601774716,-4.48693345015888,
127.111248278652));
#226333=CARTESIAN_POINT('Ctrl Pts',(206.681154150904,-5.53242507739068,
132.583126545744));
#226334=CARTESIAN_POINT('Ctrl Pts',(206.40270652709,-1.49388053201802,136.420413394932));
#226335=CARTESIAN_POINT('Ctrl Pts',(206.124258903278,3.91746311099657,135.0968180907));
#226336=CARTESIAN_POINT('Ctrl Pts',(205.845811279465,5.72885172159717,129.828666190814));
#226337=CARTESIAN_POINT('Ctrl Pts',(205.567363655652,2.27570431130586,125.457128678938));
#226338=CARTESIAN_POINT('Ctrl Pts',(205.288916031839,-3.26870357308214,
125.999436687584));
#226339=CARTESIAN_POINT('Ctrl Pts',(205.010468408026,-5.80933288384994,
130.9572347388));
#226340=CARTESIAN_POINT('Ctrl Pts',(204.732020784213,-3.01146890392974,
135.774549108008));
#226341=CARTESIAN_POINT('Ctrl Pts',(204.4535731604,2.5537877891123,136.024502973214));
#226342=CARTESIAN_POINT('Ctrl Pts',(204.175125536587,5.77223831170541,131.477401078575));
#226343=CARTESIAN_POINT('Ctrl Pts',(203.896677912775,3.6862837897924,126.311807855303));
#226344=CARTESIAN_POINT('Ctrl Pts',(203.618230288961,-1.78718543642468,
125.274651160291));
#226345=CARTESIAN_POINT('Ctrl Pts',(203.339782665149,-5.61831856260093,
129.319027308227));
#226346=CARTESIAN_POINT('Ctrl Pts',(203.061335041336,-4.28649139606962,
134.728352208566));
#226347=CARTESIAN_POINT('Ctrl Pts',(202.782887417523,0.984411954691954,
136.531720532469));
#226348=CARTESIAN_POINT('Ctrl Pts',(202.50443979371,5.3506888113544,133.071924892697));
#226349=CARTESIAN_POINT('Ctrl Pts',(202.225992169897,4.79994404549834,127.528348460205));
#226350=CARTESIAN_POINT('Ctrl Pts',(201.947544546084,-0.161714807569177,
124.995267158526));
#226351=CARTESIAN_POINT('Ctrl Pts',(201.669096922271,-4.97476565284641,
127.800458955558));
#226352=CARTESIAN_POINT('Ctrl Pts',(201.390649298458,-5.21624989388704,
133.366089631302));
#226353=CARTESIAN_POINT('Ctrl Pts',(201.112201674645,-0.664255310463968,
136.577616490799));
#226354=CARTESIAN_POINT('Ctrl Pts',(200.833754050833,4.49815745262305,134.483803242045));
#226355=CARTESIAN_POINT('Ctrl Pts',(200.55530642702,5.52698326394509,129.008761972148));
#226356=CARTESIAN_POINT('Ctrl Pts',(200.276858803207,1.47678146385132,125.183788137525));
#226357=CARTESIAN_POINT('Ctrl Pts',(199.998411179394,-3.93051035674001,
126.523845831826));
#226358=CARTESIAN_POINT('Ctrl Pts',(199.719963555581,-5.7258551755912,131.79748749945));
#226359=CARTESIAN_POINT('Ctrl Pts',(199.441515931768,-2.25941881165118,
136.158494079568));
#226360=CARTESIAN_POINT('Ctrl Pts',(199.163068307955,3.28331306145151,135.599313572066));
#226361=CARTESIAN_POINT('Ctrl Pts',(198.884620684142,5.80884062984016,130.633805545853));
#226362=CARTESIAN_POINT('Ctrl Pts',(198.606173060329,2.99632743704681,125.825029298466));
#226363=CARTESIAN_POINT('Ctrl Pts',(198.327725436517,-2.56966429165962,
125.592015279473));
#226364=CARTESIAN_POINT('Ctrl Pts',(198.049277812704,-5.77426007141042,
130.148891988961));
#226365=CARTESIAN_POINT('Ctrl Pts',(197.770830188891,-3.6725929338218,135.308112346714));
#226366=CARTESIAN_POINT('Ctrl Pts',(197.492382565078,1.80400769380988,136.328604885883));
#226367=CARTESIAN_POINT('Ctrl Pts',(197.213934941265,5.62281338150559,132.272586816804));
#226368=CARTESIAN_POINT('Ctrl Pts',(196.935487317452,4.27452826130232,126.867340597462));
#226369=CARTESIAN_POINT('Ctrl Pts',(196.657039693639,-1.00183950872307,
125.080023442474));
#226370=CARTESIAN_POINT('Ctrl Pts',(196.378592069827,-5.35756571281285,
128.553092501978));
#226371=CARTESIAN_POINT('Ctrl Pts',(196.100144446013,-4.78995075846325,
134.094966979145));
#226372=CARTESIAN_POINT('Ctrl Pts',(195.821696822201,0.179394940810534,
136.612934965078));
#226373=CARTESIAN_POINT('Ctrl Pts',(195.543249198387,4.98388545340951,133.79310689028));
#226374=CARTESIAN_POINT('Ctrl Pts',(195.264801574575,5.20842871066526,128.22676699923));
#226375=CARTESIAN_POINT('Ctrl Pts',(194.986353950762,0.64668042870769,125.029109720981));
#226376=CARTESIAN_POINT('Ctrl Pts',(194.70790632695,-4.50933557513701,127.138625880003));
#226377=CARTESIAN_POINT('Ctrl Pts',(194.429458703136,-5.52149247872048,
132.616773181746));
#226378=CARTESIAN_POINT('Ctrl Pts',(194.151011079324,-1.4596675342632,136.429401878284));
#226379=CARTESIAN_POINT('Ctrl Pts',(193.87256345551,3.9435205654586,135.072892454764));
#226380=CARTESIAN_POINT('Ctrl Pts',(193.594115831698,5.72280591721378,129.793810802232));
#226381=CARTESIAN_POINT('Ctrl Pts',(193.315668207884,2.24311220566103,125.443375061888));
#226382=CARTESIAN_POINT('Ctrl Pts',(193.037220584072,-3.29789204077089,
126.019423148508));
#226383=CARTESIAN_POINT('Ctrl Pts',(192.758772960259,-5.80829461271728,
130.992595012001));
#226384=CARTESIAN_POINT('Ctrl Pts',(192.480325336446,-2.98115818654302,
135.792788662769));
#226385=CARTESIAN_POINT('Ctrl Pts',(192.201877712633,2.58551697539033,136.008860638253));
#226386=CARTESIAN_POINT('Ctrl Pts',(191.92343008882,5.77622834646622,131.442251348686));
#226387=CARTESIAN_POINT('Ctrl Pts',(191.644982465007,3.658868051582,126.289451639914));
#226388=CARTESIAN_POINT('Ctrl Pts',(191.366534841194,-1.82081323706467,
125.285632716038));
#226389=CARTESIAN_POINT('Ctrl Pts',(191.088087217381,-5.6272561125207,129.35325512882));
#226390=CARTESIAN_POINT('Ctrl Pts',(190.809639593569,-4.26252552731426,
134.754372595315));
#226391=CARTESIAN_POINT('Ctrl Pts',(190.531191969755,1.01925778154541,136.525622023071));
#226392=CARTESIAN_POINT('Ctrl Pts',(190.252744345943,5.36439298267566,133.039311718326));
#226393=CARTESIAN_POINT('Ctrl Pts',(189.974296722129,4.77991309789331,127.499190535413));
#226394=CARTESIAN_POINT('Ctrl Pts',(189.695849098317,-0.197073412116412,
124.996359191464));
#226395=CARTESIAN_POINT('Ctrl Pts',(189.417401474504,-4.99295908396257,
127.830797421458));
#226396=CARTESIAN_POINT('Ctrl Pts',(189.138953850692,-5.20055927725872,
133.397794962038));
#226397=CARTESIAN_POINT('Ctrl Pts',(188.860506226878,-0.629099556198964,
136.581553036358));
#226398=CARTESIAN_POINT('Ctrl Pts',(188.582058603065,4.52047192378579,134.456353509349));
#226399=CARTESIAN_POINT('Ctrl Pts',(188.303610979253,5.51595054314194,128.975150924561));
#226400=CARTESIAN_POINT('Ctrl Pts',(188.02516335544,1.44254008251539,125.174902685784));
#226401=CARTESIAN_POINT('Ctrl Pts',(187.746715731627,-3.95649424194195,
126.547851272005));
#226402=CARTESIAN_POINT('Ctrl Pts',(187.468268107814,-5.71970364354381,
131.832324004755));
#226403=CARTESIAN_POINT('Ctrl Pts',(187.189820484001,-2.22678481978599,
136.172148603481));
#226404=CARTESIAN_POINT('Ctrl Pts',(186.911372860188,3.312440468869,135.579238274173));
#226405=CARTESIAN_POINT('Ctrl Pts',(186.632925236375,5.80769478834652,130.598448644184));
#226406=CARTESIAN_POINT('Ctrl Pts',(186.354477612562,2.96596131899707,125.806882058373));
#226407=CARTESIAN_POINT('Ctrl Pts',(186.076029988749,-2.60134570724499,
125.607754128061));
#226408=CARTESIAN_POINT('Ctrl Pts',(185.797582364937,-5.7781431113317,130.184053693262));
#226409=CARTESIAN_POINT('Ctrl Pts',(185.519134741124,-3.64510927408837,
135.33038501822));
#226410=CARTESIAN_POINT('Ctrl Pts',(185.240687117311,1.83760191255446,136.317521027561));
#226411=CARTESIAN_POINT('Ctrl Pts',(184.962239493498,5.63164671340385,132.238331952975));
#226412=CARTESIAN_POINT('Ctrl Pts',(184.683791869685,4.25048330587202,126.841393274542));
#226413=CARTESIAN_POINT('Ctrl Pts',(184.405344245872,-1.03666661210287,
125.086227982629));
#226414=CARTESIAN_POINT('Ctrl Pts',(184.126896622059,-5.37117055753467,
128.585747235914));
#226415=CARTESIAN_POINT('Ctrl Pts',(183.848448998247,-4.7698311568614,134.124063801647));
#226416=CARTESIAN_POINT('Ctrl Pts',(183.570001374433,0.214750057761129,
136.611735317726));
#226417=CARTESIAN_POINT('Ctrl Pts',(183.291553750621,5.00198646042476,133.762713190383));
#226418=CARTESIAN_POINT('Ctrl Pts',(183.013106126807,5.19264166658148,128.195109572179));
#226419=CARTESIAN_POINT('Ctrl Pts',(182.734658502995,0.611512855797894,
125.025280195685));
#226420=CARTESIAN_POINT('Ctrl Pts',(182.456210879182,-4.53156639540017,
127.166143403126));
#226421=CARTESIAN_POINT('Ctrl Pts',(182.177763255369,-5.5103575085511,132.650350493844));
#226422=CARTESIAN_POINT('Ctrl Pts',(181.899315631556,-1.42539926727337,
136.438183069882));
#226423=CARTESIAN_POINT('Ctrl Pts',(181.620868007743,3.96943126600311,135.048808039769));
#226424=CARTESIAN_POINT('Ctrl Pts',(181.34242038393,5.71654838332065,129.758993181434));
#226425=CARTESIAN_POINT('Ctrl Pts',(181.063972760118,2.21043680528058,125.429819927867));
#226426=CARTESIAN_POINT('Ctrl Pts',(180.785525136304,-3.32695821097111,
126.039587007222));
#226427=CARTESIAN_POINT('Ctrl Pts',(180.507077512492,-5.80704116228462,
131.027948262352));
#226428=CARTESIAN_POINT('Ctrl Pts',(180.228629888679,-2.95073697519064,
135.810843394787));
#226429=CARTESIAN_POINT('Ctrl Pts',(179.950182264866,2.61715034058839,135.993025435236));
#226430=CARTESIAN_POINT('Ctrl Pts',(179.671734641053,5.78000434826875,131.407077988614));
#226431=CARTESIAN_POINT('Ctrl Pts',(179.39328701724,3.63131672880039,126.26726272238));
#226432=CARTESIAN_POINT('Ctrl Pts',(179.114839393428,-1.8543735647511,125.296818772266));
#226433=CARTESIAN_POINT('Ctrl Pts',(178.836391769614,-5.63598514348121,
129.387536719606));
#226434=CARTESIAN_POINT('Ctrl Pts',(178.557944145802,-4.23840170853308,
134.780246613475));
#226435=CARTESIAN_POINT('Ctrl Pts',(178.279496521988,1.05406583912245,136.519311509933));
#226436=CARTESIAN_POINT('Ctrl Pts',(178.001048898175,5.3778983746034,133.006615727177));
#226437=CARTESIAN_POINT('Ctrl Pts',(177.722601274363,4.75970502876524,127.470155084831));
#226438=CARTESIAN_POINT('Ctrl Pts',(177.44415365055,-0.232424713990654,
124.997666442073));
#226439=CARTESIAN_POINT('Ctrl Pts',(177.165706026737,-5.01096749916768,
127.861246073811));
#226440=CARTESIAN_POINT('Ctrl Pts',(176.887258402924,-5.18467595198119,
133.429404192122));
#226441=CARTESIAN_POINT('Ctrl Pts',(176.608810779111,-0.593920490425269,
136.585275505922));
#226442=CARTESIAN_POINT('Ctrl Pts',(176.330363155298,4.54261888720253,134.428768450716));
#226443=CARTESIAN_POINT('Ctrl Pts',(176.051915531486,5.50471342676105,128.941607659011));
#226444=CARTESIAN_POINT('Ctrl Pts',(175.773467907672,1.40824524732727,125.166225835676));
#226445=CARTESIAN_POINT('Ctrl Pts',(175.49502028386,-3.98233151779528,126.572014438702));
#226446=CARTESIAN_POINT('Ctrl Pts',(175.216572660047,-5.7133401657742,131.867122418498));
#226447=CARTESIAN_POINT('Ctrl Pts',(174.938125036234,-2.19406831359054,
136.185604222037));
#226448=CARTESIAN_POINT('Ctrl Pts',(174.659677412421,3.34144513258691,135.558986041432));
#226449=CARTESIAN_POINT('Ctrl Pts',(174.381229788608,5.80633374058666,130.563099372659));
#226450=CARTESIAN_POINT('Ctrl Pts',(174.102782164795,2.93548529615992,125.788920001687));
#226451=CARTESIAN_POINT('Ctrl Pts',(173.824334540982,-2.63293072900865,
125.623685538813));
#226452=CARTESIAN_POINT('Ctrl Pts',(173.54588691717,-5.7818120400351,130.219238383264));
#226453=CARTESIAN_POINT('Ctrl Pts',(173.267439293356,-3.61749054349026,
135.352489976228));
#226454=CARTESIAN_POINT('Ctrl Pts',(172.988991669544,1.87112803828436,136.306232877052));
#226455=CARTESIAN_POINT('Ctrl Pts',(172.71054404573,5.64027136256211,132.204023952811));
#226456=CARTESIAN_POINT('Ctrl Pts',(172.432096421918,4.22628084721974,126.815592800833));
#226457=CARTESIAN_POINT('Ctrl Pts',(172.153648798105,-1.07145530142008,
125.092644410292));
#226458=CARTESIAN_POINT('Ctrl Pts',(171.875201174292,-5.38457637155629,
128.618484181386));
#226459=CARTESIAN_POINT('Ctrl Pts',(171.596753550479,-4.74953480741189,
134.153037611328));
#226460=CARTESIAN_POINT('Ctrl Pts',(171.318305926666,0.25009721706947,136.610320475968));
#226461=CARTESIAN_POINT('Ctrl Pts',(171.039858302853,5.01990211699227,133.732209867644));
#226462=CARTESIAN_POINT('Ctrl Pts',(170.76141067904,5.1766622072511,128.163548831885));
#226463=CARTESIAN_POINT('Ctrl Pts',(170.482963055228,0.576322623054293,
125.021664816339));
#226464=CARTESIAN_POINT('Ctrl Pts',(170.204515431414,-4.55362929680409,
127.193795741725));
#226465=CARTESIAN_POINT('Ctrl Pts',(169.926067807602,-5.4990183500578,132.683859402108));
#226466=CARTESIAN_POINT('Ctrl Pts',(169.647620183788,-1.39107818158956,
136.446755498118));
#226467=CARTESIAN_POINT('Ctrl Pts',(169.369172559976,3.99519487781229,135.024566345214));
#226468=CARTESIAN_POINT('Ctrl Pts',(169.090724936163,5.71007902062496,129.724214297113));
#226469=CARTESIAN_POINT('Ctrl Pts',(168.81227731235,2.17767949635139,125.416463949427));
#226470=CARTESIAN_POINT('Ctrl Pts',(168.533829688537,-3.35590109951139,
126.059927426375));
#226471=CARTESIAN_POINT('Ctrl Pts',(168.255382064725,-5.80557252980615,
131.063293227581));
#226472=CARTESIAN_POINT('Ctrl Pts',(167.976934440911,-2.92020642319446,
135.828712609743));
#226473=CARTESIAN_POINT('Ctrl Pts',(167.698486817099,2.64868672631821,135.976997964335));
#226474=CARTESIAN_POINT('Ctrl Pts',(167.420039193286,5.78356616988455,131.371882294628));
#226475=CARTESIAN_POINT('Ctrl Pts',(167.141591569473,3.60363084624196,126.245241928676));
#226476=CARTESIAN_POINT('Ctrl Pts',(166.86314394566,-1.88786517794308,125.308208912483));
#226477=CARTESIAN_POINT('Ctrl Pts',(166.584696321847,-5.64450533093961,
129.421870811324));
#226478=CARTESIAN_POINT('Ctrl Pts',(166.306248698034,-4.21412083421794,
134.805973303719));
#226479=CARTESIAN_POINT('Ctrl Pts',(166.027801074221,1.08883483790225,136.512789227187));
#226480=CARTESIAN_POINT('Ctrl Pts',(165.749353450409,5.3912044865292,132.973838130654));
#226481=CARTESIAN_POINT('Ctrl Pts',(165.470905826595,4.73932058701693,127.441243184462));
#226482=CARTESIAN_POINT('Ctrl Pts',(165.192458202783,-0.267767403281747,
124.999188861871));
#226483=CARTESIAN_POINT('Ctrl Pts',(164.914010578969,-5.02879023112935,
127.891803784357));
#226484=CARTESIAN_POINT('Ctrl Pts',(164.635562955157,-5.16860050662956,
133.46091615025));
#226485=CARTESIAN_POINT('Ctrl Pts',(164.357115331344,-0.55871941670932,
136.588783761558));
#226486=CARTESIAN_POINT('Ctrl Pts',(164.078667707531,4.56459752220588,134.401049088318));
#226487=CARTESIAN_POINT('Ctrl Pts',(163.800220083718,5.49327233119978,128.908133418456));
#226488=CARTESIAN_POINT('Ctrl Pts',(163.521772459905,1.37389822909362,125.157757908727));
#226489=CARTESIAN_POINT('Ctrl Pts',(163.243324836092,-4.00802122688977,
126.596334436543));
#226490=CARTESIAN_POINT('Ctrl Pts',(162.964877212279,-5.70676497808368,
131.901881451211));
#226491=CARTESIAN_POINT('Ctrl Pts',(162.686429588467,-2.16127050538683,
136.198860436632));
#226492=CARTESIAN_POINT('Ctrl Pts',(162.407981964654,3.37032597782655,135.538557624299));
#226493=CARTESIAN_POINT('Ctrl Pts',(162.129534340841,5.80475753699479,130.527759041158));
#226494=CARTESIAN_POINT('Ctrl Pts',(161.851086717028,2.90490049783562,125.771143793998));
#226495=CARTESIAN_POINT('Ctrl Pts',(161.572639093215,-2.66441818655578,
125.639808921385));
#226496=CARTESIAN_POINT('Ctrl Pts',(161.294191469402,-5.7852667215671,130.254444755185));
#226497=CARTESIAN_POINT('Ctrl Pts',(161.015743845589,-3.58973776544978,
135.37442640163));
#226498=CARTESIAN_POINT('Ctrl Pts',(160.737296221776,1.90458482867669,136.294740852644));
#226499=CARTESIAN_POINT('Ctrl Pts',(160.458848597964,5.64868700939082,132.169664087608));
#226500=CARTESIAN_POINT('Ctrl Pts',(160.18040097415,4.20192178217643,126.789940132385));
#226501=CARTESIAN_POINT('Ctrl Pts',(159.901953350338,-1.10620428756715,
125.099272487699));
#226502=CARTESIAN_POINT('Ctrl Pts',(159.623505726525,-5.39778265812024,
128.651302125312));
#226503=CARTESIAN_POINT('Ctrl Pts',(159.345058102712,-4.72906246220349,
134.18188733455));
#226504=CARTESIAN_POINT('Ctrl Pts',(159.066610478899,0.285435108933367,
136.608690492233));
#226505=CARTESIAN_POINT('Ctrl Pts',(158.788162855086,5.03763175924073,133.701598052375));
#226506=CARTESIAN_POINT('Ctrl Pts',(158.509715231273,5.16049092479898,128.132085947844));
#226507=CARTESIAN_POINT('Ctrl Pts',(158.23126760746,0.541111034464008,125.018263716911));
#226508=CARTESIAN_POINT('Ctrl Pts',(157.952819983648,-4.57552346179978,
127.221581871133));
#226509=CARTESIAN_POINT('Ctrl Pts',(157.674372359834,-5.48747542341729,
132.717298664853));
#226510=CARTESIAN_POINT('Ctrl Pts',(157.395924736022,-1.35670554899215,
136.455118845335));
#226511=CARTESIAN_POINT('Ctrl Pts',(157.117477112209,4.02081044620608,135.000168269382));
#226512=CARTESIAN_POINT('Ctrl Pts',(156.839029488396,5.70339806885126,129.68947543801));
#226513=CARTESIAN_POINT('Ctrl Pts',(156.560581864583,2.1448414927076,125.403307621479));
#226514=CARTESIAN_POINT('Ctrl Pts',(156.28213424077,-3.38471963390224,126.080443652244));
#226515=CARTESIAN_POINT('Ctrl Pts',(156.003686616957,-5.8038887697026,131.098628597966));
#226516=CARTESIAN_POINT('Ctrl Pts',(155.725238993144,-2.88956766187541,
135.846395645489));
#226517=CARTESIAN_POINT('Ctrl Pts',(155.446791369331,2.68012496398725,135.960778819456));
#226518=CARTESIAN_POINT('Ctrl Pts',(155.168343745519,5.78691367932904,131.336665570917));
#226519=CARTESIAN_POINT('Ctrl Pts',(154.889896121706,3.57581142981733,126.223390074792));
#226520=CARTESIAN_POINT('Ctrl Pts',(154.611448497893,-1.92128683559663,
125.319802714623));
#226521=CARTESIAN_POINT('Ctrl Pts',(154.33300087408,-5.65281635917722,129.456256131708));
#226522=CARTESIAN_POINT('Ctrl Pts',(154.054553250267,-4.18968380410554,
134.831551712731));
#226523=CARTESIAN_POINT('Ctrl Pts',(153.776105626454,1.12356348950664,136.50605541652));
#226524=CARTESIAN_POINT('Ctrl Pts',(153.497658002641,5.40431082539012,132.940980143345));
#226525=CARTESIAN_POINT('Ctrl Pts',(153.219210378828,4.71876052800142,127.412455905645));
#226526=CARTESIAN_POINT('Ctrl Pts',(152.940762755016,-0.303100170353132,
125.000926394444));
#226527=CARTESIAN_POINT('Ctrl Pts',(152.662315131202,-5.04642661941966,
127.922469420767));
#226528=CARTESIAN_POINT('Ctrl Pts',(152.38386750739,-5.15233353688545,133.492329668737));
#226529=CARTESIAN_POINT('Ctrl Pts',(152.105419883576,-0.523497639439988,
136.592077673268));
#226530=CARTESIAN_POINT('Ctrl Pts',(151.826972259764,4.58640701436939,134.373196449306));
#226531=CARTESIAN_POINT('Ctrl Pts',(151.548524635951,5.48162768041213,128.874729443297));
#226532=CARTESIAN_POINT('Ctrl Pts',(151.270077012138,1.33950030055583,125.149499218718));
#226533=CARTESIAN_POINT('Ctrl Pts',(150.991629388325,-4.03356241728369,
126.620810364342));
#226534=CARTESIAN_POINT('Ctrl Pts',(150.713181764512,-5.69997832411825,
131.936599814887));
#226535=CARTESIAN_POINT('Ctrl Pts',(150.434734140699,-2.1283926105098,136.211916756054));
#226536=CARTESIAN_POINT('Ctrl Pts',(150.156286516886,3.39908193439765,135.517953779753));
#226537=CARTESIAN_POINT('Ctrl Pts',(149.877838893074,5.8029662359777,130.49242895923));
#226538=CARTESIAN_POINT('Ctrl Pts',(149.599391269261,2.87420805735513,125.753554094008));
#226539=CARTESIAN_POINT('Ctrl Pts',(149.320943645448,-2.69580691310719,
125.65612367832));
#226540=CARTESIAN_POINT('Ctrl Pts',(149.042496021635,-5.7885070279132,130.289671504441));
#226541=CARTESIAN_POINT('Ctrl Pts',(148.764048397822,-3.56185196835627,
135.396193481562));
#226542=CARTESIAN_POINT('Ctrl Pts',(148.485600774009,1.93797104397778,136.283045380177));
#226543=CARTESIAN_POINT('Ctrl Pts',(148.207153150196,5.6568933420451,132.135253630582));
#226544=CARTESIAN_POINT('Ctrl Pts',(147.928705526383,4.17740701337624,126.764436219762));
#226545=CARTESIAN_POINT('Ctrl Pts',(147.65025790257,-1.14091228290746,125.106111969245));
#226546=CARTESIAN_POINT('Ctrl Pts',(147.371810278758,-5.41078892786276,
128.684199851613));
#226547=CARTESIAN_POINT('Ctrl Pts',(147.093362654945,-4.70841487984645,
134.210611902278));
#226548=CARTESIAN_POINT('Ctrl Pts',(146.814915031132,0.320762423894332,
136.60684542692));
#226549=CARTESIAN_POINT('Ctrl Pts',(146.536467407319,5.05517473019176,133.670878878906));
#226550=CARTESIAN_POINT('Ctrl Pts',(146.258019783506,5.14412841845787,128.100722085923));
#226551=CARTESIAN_POINT('Ctrl Pts',(145.979572159693,0.505879394805349,
125.015077023433));
#226552=CARTESIAN_POINT('Ctrl Pts',(145.70112453588,-4.59724807909095,127.249500761725));
#226553=CARTESIAN_POINT('Ctrl Pts',(145.422676912067,-5.47572915635697,
132.750667042976));
#226554=CARTESIAN_POINT('Ctrl Pts',(145.144229288255,-1.32228264317164,
136.463272801628));
#226555=CARTESIAN_POINT('Ctrl Pts',(144.865781664442,4.0462770219901,134.975614716357));
#226556=CARTESIAN_POINT('Ctrl Pts',(144.587334040629,5.69650577556471,129.654777891387));
#226557=CARTESIAN_POINT('Ctrl Pts',(144.308886416816,2.11192401117359,125.390351431538));
#226558=CARTESIAN_POINT('Ctrl Pts',(144.030438793003,-3.41341274626234,
126.101134924595));
#226559=CARTESIAN_POINT('Ctrl Pts',(143.75199116919,-5.80198994436631,131.133953064144));
#226560=CARTESIAN_POINT('Ctrl Pts',(143.473543545377,-2.85882182656403,
135.863891846773));
#226561=CARTESIAN_POINT('Ctrl Pts',(143.195095921564,2.71146388864014,135.944368601604));
#226562=CARTESIAN_POINT('Ctrl Pts',(142.916648297751,5.790046752559,131.301429122451));
#226563=CARTESIAN_POINT('Ctrl Pts',(142.638200673938,3.54785951038517,126.201707970457));
#226564=CARTESIAN_POINT('Ctrl Pts',(142.359753050125,-1.95463729925998,
125.331599749072));
#226565=CARTESIAN_POINT('Ctrl Pts',(142.081305426313,-5.66091792022584,
129.490691406602));
#226566=CARTESIAN_POINT('Ctrl Pts',(141.8028578025,-4.16509152371897,134.856980892698));
#226567=CARTESIAN_POINT('Ctrl Pts',(141.524410178687,1.15825050705268,136.499110327454));
#226568=CARTESIAN_POINT('Ctrl Pts',(141.245962554874,5.41721690552589,132.908042982814));
#226569=CARTESIAN_POINT('Ctrl Pts',(140.967514931061,4.69802561357932,127.383794315106));
#226570=CARTESIAN_POINT('Ctrl Pts',(140.689067307248,-0.338421705936203,
125.002878975406));
#226571=CARTESIAN_POINT('Ctrl Pts',(140.410619683435,-5.06387601051571,
127.953241846716));
#226572=CARTESIAN_POINT('Ctrl Pts',(140.132172059623,-5.13587564552739,
133.523643583541));
#226573=CARTESIAN_POINT('Ctrl Pts',(139.85372443581,-0.48825646377323,136.595157118993));
#226574=CARTESIAN_POINT('Ctrl Pts',(139.575276811997,4.60804655553434,134.34521156577));
#226575=CARTESIAN_POINT('Ctrl Pts',(139.296829188184,5.46977990589493,128.841396971331));
#226576=CARTESIAN_POINT('Ctrl Pts',(139.018381564371,1.30505273634171,125.141450071677));
#226577=CARTESIAN_POINT('Ctrl Pts',(138.739933940558,-4.05895414253892,
126.645441315135));
#226578=CARTESIAN_POINT('Ctrl Pts',(138.461486316745,-5.69298045535984,
131.971276223022));
#226579=CARTESIAN_POINT('Ctrl Pts',(138.183038692932,-2.09543584726193,
136.224772696493));
#226580=CARTESIAN_POINT('Ctrl Pts',(137.904591069119,3.42771193673771,135.49717527128));
#226581=CARTESIAN_POINT('Ctrl Pts',(137.626143445306,5.80095990391266,130.457110436044));
#226582=CARTESIAN_POINT('Ctrl Pts',(137.347695821494,2.84340911203807,125.736151553513));
#226583=CARTESIAN_POINT('Ctrl Pts',(137.069248197681,-2.727095745542,125.672629205068));
#226584=CARTESIAN_POINT('Ctrl Pts',(136.790800573868,-5.7915328390027,130.324917325691));
#226585=CARTESIAN_POINT('Ctrl Pts',(136.512352950055,-3.53383418552815,
135.417790409441));
#226586=CARTESIAN_POINT('Ctrl Pts',(136.233905326242,1.97128544704926,136.271146893031));
#226587=CARTESIAN_POINT('Ctrl Pts',(135.955457702429,5.66489005643625,132.100793856825));
#226588=CARTESIAN_POINT('Ctrl Pts',(135.677010078616,4.15273744922295,126.739082008025));
#226589=CARTESIAN_POINT('Ctrl Pts',(135.398562454803,-1.17557800132362,
125.113162601491));
#226590=CARTESIAN_POINT('Ctrl Pts',(135.12011483099,-5.42359469883174,128.717176141249));
#226591=CARTESIAN_POINT('Ctrl Pts',(134.841667207177,-4.68759282544451,
134.239210250113));
#226592=CARTESIAN_POINT('Ctrl Pts',(134.563219583365,0.356077852885664,
136.604785348398));
#226593=CARTESIAN_POINT('Ctrl Pts',(134.284771959552,5.0725303797842,133.640053485549));
#226594=CARTESIAN_POINT('Ctrl Pts',(134.006324335739,5.12757529454644,128.069458408322));
#226595=CARTESIAN_POINT('Ctrl Pts',(133.727876711926,0.470629009599695,
125.012104853988));
#226596=CARTESIAN_POINT('Ctrl Pts',(133.449429088113,-4.61880234366392,
127.277551378957));
#226597=CARTESIAN_POINT('Ctrl Pts',(133.1709814643,-5.46377998413907,132.783963299997));
#226598=CARTESIAN_POINT('Ctrl Pts',(132.892533840487,-1.28781073968153,
136.47121706485));
#226599=CARTESIAN_POINT('Ctrl Pts',(132.614086216674,4.07159366149105,134.950906595976));
#226600=CARTESIAN_POINT('Ctrl Pts',(132.335638592862,5.68940239616175,129.620122942976));
#226601=CARTESIAN_POINT('Ctrl Pts',(132.057190969048,2.07892827151876,125.377595859696));
#226602=CARTESIAN_POINT('Ctrl Pts',(131.778743345236,-3.44197937335791,
126.122000476702));
#226603=CARTESIAN_POINT('Ctrl Pts',(131.500295721423,-5.79987612415893,
131.169265317152));
#226604=CARTESIAN_POINT('Ctrl Pts',(131.22184809761,-2.82797005655853,135.881200565267));
#226605=CARTESIAN_POINT('Ctrl Pts',(130.943400473797,2.74270233900145,135.927767918864));
#226606=CARTESIAN_POINT('Ctrl Pts',(130.664952849984,5.79296527347731,131.26617425493));
#226607=CARTESIAN_POINT('Ctrl Pts',(130.386505226171,3.51977612371406,126.180196419108));
#226608=CARTESIAN_POINT('Ctrl Pts',(130.108057602358,-1.98791533311939,
125.343599578688));
#226609=CARTESIAN_POINT('Ctrl Pts',(129.829609978546,-5.66880971387908,
129.52517535999));
#226610=CARTESIAN_POINT('Ctrl Pts',(129.551162354732,-4.14034490433441,
134.882259901329));
#226611=CARTESIAN_POINT('Ctrl Pts',(129.27271473092,1.19289460520041,136.491954217345));
#226612=CARTESIAN_POINT('Ctrl Pts',(128.994267107107,5.42992224869717,132.875027869557));
#226613=CARTESIAN_POINT('Ctrl Pts',(128.715819483294,4.67711661209022,127.355259474909));
#226614=CARTESIAN_POINT('Ctrl Pts',(128.437371859481,-0.373730701178542,
125.005046532403));
#226615=CARTESIAN_POINT('Ctrl Pts',(128.158924235668,-5.0811377578241,127.984119921918));
#226616=CARTESIAN_POINT('Ctrl Pts',(127.880476611855,-5.11922744240848,
133.554856734316));
#226617=CARTESIAN_POINT('Ctrl Pts',(127.602028988042,-0.452997195583419,
136.598021984625));
#226618=CARTESIAN_POINT('Ctrl Pts',(127.323581364229,4.62951534383955,134.3170954747));
#226619=CARTESIAN_POINT('Ctrl Pts',(127.045133740417,5.45772944667181,128.808137237705));
#226620=CARTESIAN_POINT('Ctrl Pts',(126.766686116604,1.2705568129186,125.133610765869));
#226621=CARTESIAN_POINT('Ctrl Pts',(126.488238492791,-4.08419546175569,
126.67022637621));
#226622=CARTESIAN_POINT('Ctrl Pts',(126.209790868978,-5.68577163111709,
132.005909390672));
#226623=CARTESIAN_POINT('Ctrl Pts',(125.931343245165,-2.06240143686808,
136.237427781569));
#226624=CARTESIAN_POINT('Ctrl Pts',(125.652895621352,3.45621492395137,135.476222868834));
#226625=CARTESIAN_POINT('Ctrl Pts',(125.374447997539,5.79873861514512,130.421804780342));
#226626=CARTESIAN_POINT('Ctrl Pts',(125.096000373726,2.8125048031507,125.718936817367));
#226627=CARTESIAN_POINT('Ctrl Pts',(124.817552749914,-2.75828352444112,
125.68932489001));
#226628=CARTESIAN_POINT('Ctrl Pts',(124.5391051261,-5.79434404271298,130.36018091289));
#226629=CARTESIAN_POINT('Ctrl Pts',(124.260657502288,-3.50568545517477,
135.439216384981));
#226630=CARTESIAN_POINT('Ctrl Pts',(123.982209878475,2.00452680341345,136.25904583211));
#226631=CARTESIAN_POINT('Ctrl Pts',(123.703762254662,5.67267685624313,132.066286043259));
#226632=CARTESIAN_POINT('Ctrl Pts',(123.425314630849,4.12791400385628,126.71387843668));
#226633=CARTESIAN_POINT('Ctrl Pts',(123.146867007036,-1.21020015826455,
125.120424123171));
#226634=CARTESIAN_POINT('Ctrl Pts',(122.868419383223,-5.43619949650465,
128.750229772276));
#226635=CARTESIAN_POINT('Ctrl Pts',(122.58997175941,-4.66659707056658,134.267681318331));
#226636=CARTESIAN_POINT('Ctrl Pts',(122.311524135597,0.391380087281262,
136.602510333005));
#226637=CARTESIAN_POINT('Ctrl Pts',(122.033076511785,5.08969806489794,133.609123014551));
#226638=CARTESIAN_POINT('Ctrl Pts',(121.754628887972,5.11083216644683,128.038296073528));
#226639=CARTESIAN_POINT('Ctrl Pts',(121.476181264159,0.435361185062875,
125.00934731871));
#226640=CARTESIAN_POINT('Ctrl Pts',(121.197733640346,-4.64018545681751,
127.305732683402));
#226641=CARTESIAN_POINT('Ctrl Pts',(120.919286016533,-5.45162834954452,
132.817186202114));
#226642=CARTESIAN_POINT('Ctrl Pts',(120.64083839272,-1.25329111589093,136.478951340622));
#226643=CARTESIAN_POINT('Ctrl Pts',(120.362390768907,4.09675942659154,134.92604482381));
#226644=CARTESIAN_POINT('Ctrl Pts',(120.083943145094,5.68208819386074,129.585511876926));
#226645=CARTESIAN_POINT('Ctrl Pts',(119.805495521281,2.04585549641223,125.36504137862));
#226646=CARTESIAN_POINT('Ctrl Pts',(119.527047897469,-3.47041845664194,
126.143039535386));
#226647=CARTESIAN_POINT('Ctrl Pts',(119.248600273655,-5.79754738740892,
131.204564048482));
#226648=CARTESIAN_POINT('Ctrl Pts',(118.970152649843,-2.7970134950826,135.898321159589));
#226649=CARTESIAN_POINT('Ctrl Pts',(118.69170502603,2.77383915751901,135.910977386384));
#226650=CARTESIAN_POINT('Ctrl Pts',(118.413257402217,5.795669133937,131.230902274733));
#226651=CARTESIAN_POINT('Ctrl Pts',(118.134809778404,3.49156231044436,126.158856217863));
#226652=CARTESIAN_POINT('Ctrl Pts',(117.856362154591,-2.02111970404504,
125.355801758813));
#226653=CARTESIAN_POINT('Ctrl Pts',(117.577914530778,-5.67649144770371,
129.559706714059));
#226654=CARTESIAN_POINT('Ctrl Pts',(117.299466906965,-4.11544486294674,
134.907387801903));
#226655=CARTESIAN_POINT('Ctrl Pts',(117.021019283153,1.22749450019975,136.484587351363));
#226656=CARTESIAN_POINT('Ctrl Pts',(116.74257165934,5.44242638410263,132.841936026965));
#226657=CARTESIAN_POINT('Ctrl Pts',(116.464124035527,4.65603429832517,127.326852442422));
#226658=CARTESIAN_POINT('Ctrl Pts',(116.185676411714,-0.409025847692317,
125.007428985116));
#226659=CARTESIAN_POINT('Ctrl Pts',(115.907228787901,-5.09821122170419,
128.015102502178));
#226660=CARTESIAN_POINT('Ctrl Pts',(115.628781164088,-5.10238954443416,
133.585967964446));
#226661=CARTESIAN_POINT('Ctrl Pts',(115.350333540275,-0.417721141415912,
136.600672164005));
#226662=CARTESIAN_POINT('Ctrl Pts',(115.071885916462,4.65081258375125,134.288849217947));
#226663=CARTESIAN_POINT('Ctrl Pts',(114.793438292649,5.44547674927697,128.77495147487));
#226664=CARTESIAN_POINT('Ctrl Pts',(114.514990668836,1.23601380854556,125.125981591782));
#226665=CARTESIAN_POINT('Ctrl Pts',(114.236543045024,-4.10928543960769,
126.695164629152));
#226666=CARTESIAN_POINT('Ctrl Pts',(113.958095421211,-5.67835211851559,
132.040498034489));
#226667=CARTESIAN_POINT('Ctrl Pts',(113.679647797398,-2.02929060343055,
136.249881542344));
#226668=CARTESIAN_POINT('Ctrl Pts',(113.401200173585,3.48458983985001,135.455097348814));
#226669=CARTESIAN_POINT('Ctrl Pts',(113.122752549772,5.79630245198571,130.386513300387));
#226670=CARTESIAN_POINT('Ctrl Pts',(112.844304925959,2.78149627586357,125.701910523471));
#226671=CARTESIAN_POINT('Ctrl Pts',(112.565857302146,-2.78936909412988,
125.706210114483));
#226672=CARTESIAN_POINT('Ctrl Pts',(112.287409678333,-5.7969405348739,130.395460959329));
#226673=CARTESIAN_POINT('Ctrl Pts',(112.008962054521,-3.47740682035766,
135.460470614237));
#226674=CARTESIAN_POINT('Ctrl Pts',(111.730514430707,2.03769388129978,136.246742645822));
#226675=CARTESIAN_POINT('Ctrl Pts',(111.452066806895,5.68025345292297,132.031731468582));
#226676=CARTESIAN_POINT('Ctrl Pts',(111.173619183082,4.10293759711819,126.688826439658));
#226677=CARTESIAN_POINT('Ctrl Pts',(110.895171559269,-1.24477747079359,
125.127896265209));
#226678=CARTESIAN_POINT('Ctrl Pts',(110.616723935456,-5.44860285380605,
128.783359519875));
#226679=CARTESIAN_POINT('Ctrl Pts',(110.338276311643,-4.64542839321807,
134.296024051927));
#226680=CARTESIAN_POINT('Ctrl Pts',(110.05982868783,0.426667818943798,136.600020465042));
#226681=CARTESIAN_POINT('Ctrl Pts',(109.781381064017,5.10667714937814,133.57808861205));
#226682=CARTESIAN_POINT('Ctrl Pts',(109.502933440204,5.0938996545818,128.007236236273));
#226683=CARTESIAN_POINT('Ctrl Pts',(109.224485816392,0.400077228057368,
125.006804519781));
#226684=CARTESIAN_POINT('Ctrl Pts',(108.946038192578,-4.66139662619255,
127.334043630792));
#226685=CARTESIAN_POINT('Ctrl Pts',(108.667590568766,-5.43927470285667,
132.850334518237));
#226686=CARTESIAN_POINT('Ctrl Pts',(108.389142944953,-1.21872505093712,
136.486475342347));
#226687=CARTESIAN_POINT('Ctrl Pts',(108.11069532114,4.1217733847649,134.901030321119));
#226688=CARTESIAN_POINT('Ctrl Pts',(107.832247697327,5.67456343969215,129.550945975765));
#226689=CARTESIAN_POINT('Ctrl Pts',(107.553800073514,2.01270691137792,125.352688453517));
#226690=CARTESIAN_POINT('Ctrl Pts',(107.275352449701,-3.49872894229381,
126.164251321038));
#226691=CARTESIAN_POINT('Ctrl Pts',(106.996904825888,-5.7950038204084,131.239847950126));
#226692=CARTESIAN_POINT('Ctrl Pts',(106.718457202076,-2.76595328924301,
135.91525299533));
#226693=CARTESIAN_POINT('Ctrl Pts',(106.440009578262,2.80487319040651,135.893997626342));
#226694=CARTESIAN_POINT('Ctrl Pts',(106.16156195445,5.7981582337456,131.195614488879));
#226695=CARTESIAN_POINT('Ctrl Pts',(105.883114330637,3.46321911604922,126.137688157493));
#226696=CARTESIAN_POINT('Ctrl Pts',(105.604666706824,-2.05424918163679,
125.36820583729));
#226697=CARTESIAN_POINT('Ctrl Pts',(105.326219083011,-5.68396283705021,
129.594284189235));
#226698=CARTESIAN_POINT('Ctrl Pts',(105.047771459198,-4.09039232223623,
134.932363663296));
#226699=CARTESIAN_POINT('Ctrl Pts',(104.769323835385,1.26204890993897,136.47701000249));
#226700=CARTESIAN_POINT('Ctrl Pts',(104.490876211572,5.45472884839698,132.808768681268));
#226701=CARTESIAN_POINT('Ctrl Pts',(104.21242858776,4.63477945349693,127.29857427028));
#226702=CARTESIAN_POINT('Ctrl Pts',(103.933980963947,-0.444305837602887,
125.010026245263));
#226703=CARTESIAN_POINT('Ctrl Pts',(103.655533340134,-5.1150957694926,128.046188439421));
#226704=CARTESIAN_POINT('Ctrl Pts',(103.377085716321,-5.08536257553889,
133.616976121092));
#226705=CARTESIAN_POINT('Ctrl Pts',(103.098638092508,-0.38242960843803,
136.603107558928));
#226706=CARTESIAN_POINT('Ctrl Pts',(102.820190468695,4.6719374860923,134.260473842188));
#226707=CARTESIAN_POINT('Ctrl Pts',(102.541742844882,5.4330222677386,128.741840912539));
#226708=CARTESIAN_POINT('Ctrl Pts',(102.263295221069,1.2014250032263,125.118562832119));
#226709=CARTESIAN_POINT('Ctrl Pts',(101.984847597256,-4.13422314637653,
126.720255149861));
#226710=CARTESIAN_POINT('Ctrl Pts',(101.706399973443,-5.67072219248816,
132.07504087278));
#226711=CARTESIAN_POINT('Ctrl Pts',(101.427952349631,-1.99610457388343,
136.262133517338));
#226712=CARTESIAN_POINT('Ctrl Pts',(101.149504725818,3.51283563299066,135.433799494034));
#226713=CARTESIAN_POINT('Ctrl Pts',(100.871057102005,5.7936515047074,130.351237303918));
#226714=CARTESIAN_POINT('Ctrl Pts',(100.592609478192,2.75038467920892,125.685073302739));
#226715=CARTESIAN_POINT('Ctrl Pts',(100.314161854379,-2.82035130272114,
125.723284252797));
#226716=CARTESIAN_POINT('Ctrl Pts',(100.035714230566,-5.79932221927147,
130.430756157697));
#226717=CARTESIAN_POINT('Ctrl Pts',(99.7572666067534,-3.44899932895201,
135.481552309624));
#226718=CARTESIAN_POINT('Ctrl Pts',(99.4788189829407,2.07078545168999,136.234237790066));
#226719=CARTESIAN_POINT('Ctrl Pts',(99.2003713591278,5.6876195657222,131.997131413226));
#226720=CARTESIAN_POINT('Ctrl Pts',(98.9219237353147,4.07780915451857,126.663926945268));
#226721=CARTESIAN_POINT('Ctrl Pts',(98.6434761115021,-1.27930865763567,
125.13557875072));
#226722=CARTESIAN_POINT('Ctrl Pts',(98.3650284876889,-5.460804311125,128.816564156414));
#226723=CARTESIAN_POINT('Ctrl Pts',(98.0865808638763,-4.62408757781209,
134.324237400649));
#226724=CARTESIAN_POINT('Ctrl Pts',(97.8081332400632,0.461939740273397,
136.597315836771));
#226725=CARTESIAN_POINT('Ctrl Pts',(97.5296856162504,5.12346700405862,133.546951428038));
#226726=CARTESIAN_POINT('Ctrl Pts',(97.2512379924375,5.07677838639178,127.97628004749));
#226727=CARTESIAN_POINT('Ctrl Pts',(96.9727903686245,0.364778446043045,
125.004476551425));
#226728=CARTESIAN_POINT('Ctrl Pts',(96.6943427448119,-4.68243506580139,
127.362483172053));
#226729=CARTESIAN_POINT('Ctrl Pts',(96.4158951209985,-5.42671950184442,
132.883407020047));
#226730=CARTESIAN_POINT('Ctrl Pts',(96.1374474971861,-1.18411382567837,
136.493788791223));
#226731=CARTESIAN_POINT('Ctrl Pts',(95.8589998733729,4.14663460910971,134.875864014826));
#226732=CARTESIAN_POINT('Ctrl Pts',(95.5805522495601,5.66682841248846,129.516426520346));
#226733=CARTESIAN_POINT('Ctrl Pts',(95.3021046257473,1.97948374474885,125.340537542131));
#226734=CARTESIAN_POINT('Ctrl Pts',(95.0236570019342,-3.52690978125809,
126.185635047646));
#226735=CARTESIAN_POINT('Ctrl Pts',(94.7452093781216,-5.79224551741027,
131.275115714627));
#226736=CARTESIAN_POINT('Ctrl Pts',(94.4667617543085,-2.73479058998699,
135.931995445075));
#226737=CARTESIAN_POINT('Ctrl Pts',(94.1883141304955,2.8358032876865,135.876829267928));
#226738=CARTESIAN_POINT('Ctrl Pts',(93.909866506683,5.80043248066857,131.160312204968));
#226739=CARTESIAN_POINT('Ctrl Pts',(93.6314188828698,3.43474759079615,126.116693022386));
#226740=CARTESIAN_POINT('Ctrl Pts',(93.352971259057,-2.08730253826965,125.380811354481));
#226741=CARTESIAN_POINT('Ctrl Pts',(93.0745236352441,-5.69122360506351,
129.628906504239));
#226742=CARTESIAN_POINT('Ctrl Pts',(92.7960760114314,-4.06518821053398,
134.957186560018));
#226743=CARTESIAN_POINT('Ctrl Pts',(92.5176283876181,1.29655655399172,136.469222451509));
#226744=CARTESIAN_POINT('Ctrl Pts',(92.2391807638055,5.46682918570788,132.775527061492));
#226745=CARTESIAN_POINT('Ctrl Pts',(91.9607331399925,4.61335286521161,127.270426006341));
#226746=CARTESIAN_POINT('Ctrl Pts',(91.6822855161797,-0.479569363597252,
125.012838216602));
#226747=CARTESIAN_POINT('Ctrl Pts',(91.4038378923669,-5.13179077552621,
128.077376581749));
#226748=CARTESIAN_POINT('Ctrl Pts',(91.1253902685539,-5.06814716666323,
133.647880055237));
#226749=CARTESIAN_POINT('Ctrl Pts',(90.846942644741,-0.347123904390365,
136.605328079151));
#226750=CARTESIAN_POINT('Ctrl Pts',(90.5684950209282,4.69288926807169,134.231970398883));
#226751=CARTESIAN_POINT('Ctrl Pts',(90.2900473971151,5.42036646356212,128.708806777632));
#226752=CARTESIAN_POINT('Ctrl Pts',(90.0115997733025,1.16679167866171,125.111354761782));
#226753=CARTESIAN_POINT('Ctrl Pts',(89.7331521494893,-4.15900765798632,
126.7454970086));
#226754=CARTESIAN_POINT('Ctrl Pts',(89.4547045256766,-5.66288213576447,
132.109536625546));
#226755=CARTESIAN_POINT('Ctrl Pts',(89.1762569018636,-1.96284457794726,
136.274183252551));
#226756=CARTESIAN_POINT('Ctrl Pts',(88.8978092780507,3.5409512567151,135.412330093694));
#226757=CARTESIAN_POINT('Ctrl Pts',(88.619361654238,5.79078587154194,130.3159780981));
#226758=CARTESIAN_POINT('Ctrl Pts',(88.3409140304249,2.71917116603865,125.668425779081));
#226759=CARTESIAN_POINT('Ctrl Pts',(88.0624664066122,-2.85122900215762,
125.740546672265));
#226760=CARTESIAN_POINT('Ctrl Pts',(87.7840187827991,-5.80148900765152,
130.466065200115));
#226761=CARTESIAN_POINT('Ctrl Pts',(87.5055711589863,-3.42046403360785,
135.502460689953));
#226762=CARTESIAN_POINT('Ctrl Pts',(87.2271235351733,2.10380028836375,136.221531728214));
#226763=CARTESIAN_POINT('Ctrl Pts',(86.9486759113605,5.69477492168681,131.962487159311));
#226764=CARTESIAN_POINT('Ctrl Pts',(86.6702282875477,4.05252960720113,126.63918087617));
#226765=CARTESIAN_POINT('Ctrl Pts',(86.3917806637346,-1.31379243922498,
125.14347129503));
#226766=CARTESIAN_POINT('Ctrl Pts',(86.113333039922,-5.47280341633199,128.849842451481));
#226767=CARTESIAN_POINT('Ctrl Pts',(85.8348854161089,-4.6025754151404,134.352320319043));
#226768=CARTESIAN_POINT('Ctrl Pts',(85.5564377922961,0.497194544256039,
136.594396548415));
#226769=CARTESIAN_POINT('Ctrl Pts',(85.2779901684829,5.1400670067851,133.515712616316));
#226770=CARTESIAN_POINT('Ctrl Pts',(84.9995425446705,5.05946899631168,127.945428654274));
#226771=CARTESIAN_POINT('Ctrl Pts',(84.7210949208572,0.329466147029263,
125.002363499906));
#226772=CARTESIAN_POINT('Ctrl Pts',(84.4426472970446,-4.70329999605691,
127.391050253351));
#226773=CARTESIAN_POINT('Ctrl Pts',(84.1641996732315,-5.41396321174535,
132.916402482027));
#226774=CARTESIAN_POINT('Ctrl Pts',(83.8857520494189,-1.14945872264635,
136.500891416245));
#226775=CARTESIAN_POINT('Ctrl Pts',(83.6073044256056,4.17134217838416,134.850546837477));
#226776=CARTESIAN_POINT('Ctrl Pts',(83.328856801793,5.65888339887398,129.481954789796));
#226777=CARTESIAN_POINT('Ctrl Pts',(83.05040917798,1.94618722762166,125.328589094719));
#226778=CARTESIAN_POINT('Ctrl Pts',(82.7719615541671,-3.5549599292834,126.207189922827));
#226779=CARTESIAN_POINT('Ctrl Pts',(82.4935139303543,-5.78927258062435,
131.310366035126));
#226780=CARTESIAN_POINT('Ctrl Pts',(82.2150663065413,-2.70352655206008,
135.948547888425));
#226781=CARTESIAN_POINT('Ctrl Pts',(81.9366186827285,2.86662830323276,135.859472947324));
#226782=CARTESIAN_POINT('Ctrl Pts',(81.6581710589156,5.80249179043285,131.124996731141));
#226783=CARTESIAN_POINT('Ctrl Pts',(81.3797234351026,3.40614878970799,126.095871590527));
#226784=CARTESIAN_POINT('Ctrl Pts',(81.1012758112897,-2.12027854913937,
125.393617843285));
#226785=CARTESIAN_POINT('Ctrl Pts',(80.822828187477,-5.6982734826932,129.663572376127));
#226786=CARTESIAN_POINT('Ctrl Pts',(80.5443805636639,-4.03983346178761,
134.981855572247));
#226787=CARTESIAN_POINT('Ctrl Pts',(80.2659329398512,1.33101615366455,136.461224986989));
#226788=CARTESIAN_POINT('Ctrl Pts',(79.9874853160382,5.47872694765296,132.742212399419));
#226789=CARTESIAN_POINT('Ctrl Pts',(79.7090376922254,4.59175532743923,127.242408693648));
#226790=CARTESIAN_POINT('Ctrl Pts',(79.4305900684125,-0.514815118972584,
125.015864794932));
#226791=CARTESIAN_POINT('Ctrl Pts',(79.1521424445996,-5.1482956211654,128.108665773475));
#226792=CARTESIAN_POINT('Ctrl Pts',(78.8736948207867,-5.05074395573051,
133.678678621723));
#226793=CARTESIAN_POINT('Ctrl Pts',(78.5952471969738,-0.31180533753877,
136.607333642391));
#226794=CARTESIAN_POINT('Ctrl Pts',(78.3167995731609,4.71366715331346,134.203339944237));
#226795=CARTESIAN_POINT('Ctrl Pts',(78.0383519493481,5.407509805713,128.675850294243));
#226796=CARTESIAN_POINT('Ctrl Pts',(77.7599043255351,1.1321151182024,125.104357647873));
#226797=CARTESIAN_POINT('Ctrl Pts',(77.4814567017223,-4.18363805603787,
126.770889270024));
#226798=CARTESIAN_POINT('Ctrl Pts',(77.2030090779094,-5.65483223886072,
132.143984014535));
#226799=CARTESIAN_POINT('Ctrl Pts',(76.9245614540965,-1.92951184808342,
136.286030301474));
#226800=CARTESIAN_POINT('Ctrl Pts',(76.6461138302835,3.56893566918854,135.390689943351));
#226801=CARTESIAN_POINT('Ctrl Pts',(76.3676662064707,5.78770565867644,130.280736989476));
#226802=CARTESIAN_POINT('Ctrl Pts',(76.0892185826578,2.68785689298084,125.651968569378));
#226803=CARTESIAN_POINT('Ctrl Pts',(75.8107709588449,-2.8820010482549,125.75799673322));
#226804=CARTESIAN_POINT('Ctrl Pts',(75.532323335032,-5.8034408197229,130.501386778194));
#226805=CARTESIAN_POINT('Ctrl Pts',(75.2538757112192,-3.39180199171105,
135.523194980456));
#226806=CARTESIAN_POINT('Ctrl Pts',(74.9754280874062,2.13673716794415,136.208624931095));
#226807=CARTESIAN_POINT('Ctrl Pts',(74.6969804635933,5.70171925567246,131.92779999059));
#226808=CARTESIAN_POINT('Ctrl Pts',(74.4185328397805,4.02709989190878,126.61458914934));
#226809=CARTESIAN_POINT('Ctrl Pts',(74.1400852159675,-1.34822753775231,
125.151573605674));
#226810=CARTESIAN_POINT('Ctrl Pts',(73.8616375921548,-5.48459972479585,
128.883193171938));
#226811=CARTESIAN_POINT('Ctrl Pts',(73.5831899683417,-4.58089270234404,
134.380271766487));
#226812=CARTESIAN_POINT('Ctrl Pts',(73.3047423445289,0.532430924512096,
136.591262708148));
#226813=CARTESIAN_POINT('Ctrl Pts',(73.026294720716,5.15647654243839,133.484373334449));
#226814=CARTESIAN_POINT('Ctrl Pts',(72.7478470969032,5.04197212574731,127.914683199832));
#226815=CARTESIAN_POINT('Ctrl Pts',(72.46939947309,0.294141639526237,125.000465443524));
#226816=CARTESIAN_POINT('Ctrl Pts',(72.1909518492774,-4.72399064380143,
127.419743816117));
#226817=CARTESIAN_POINT('Ctrl Pts',(71.9125042254643,-5.40100630524849,
132.949319681519));
#226818=CARTESIAN_POINT('Ctrl Pts',(71.6340566016516,-1.11476102599866,
136.507782954223));
#226819=CARTESIAN_POINT('Ctrl Pts',(71.3556089778387,4.19589517704018,134.82507972721));
#226820=CARTESIAN_POINT('Ctrl Pts',(71.0771613540258,5.65072869325411,129.447532061481));
#226821=CARTESIAN_POINT('Ctrl Pts',(70.7987137302128,1.91281859381102,125.316843554035));
#226822=CARTESIAN_POINT('Ctrl Pts',(70.5202661064001,-3.58287834696108,
126.22891514786));
#226823=CARTESIAN_POINT('Ctrl Pts',(70.241818482587,-5.78608512021397,131.345597605407));
#226824=CARTESIAN_POINT('Ctrl Pts',(69.9633708587742,-2.67216233396265,
135.964909712024));
#226825=CARTESIAN_POINT('Ctrl Pts',(69.6849232349613,2.89734709481291,135.841929307673));
#226826=CARTESIAN_POINT('Ctrl Pts',(69.4064756111484,5.80433608672999,131.089669376025));
#226827=CARTESIAN_POINT('Ctrl Pts',(69.1280279873355,3.37742377252397,126.07522463346));
#226828=CARTESIAN_POINT('Ctrl Pts',(68.8495803635227,-2.15317599230747,
125.406624829152));
#226829=CARTESIAN_POINT('Ctrl Pts',(68.5711327397097,-5.70511220870344,
129.698280520343));
#226830=CARTESIAN_POINT('Ctrl Pts',(68.2926851158969,-4.01432901552682,
135.006369785865));
#226831=CARTESIAN_POINT('Ctrl Pts',(68.014237492084,1.36542643204398,136.45301790528));
#226832=CARTESIAN_POINT('Ctrl Pts',(67.735789868271,5.49042169335597,132.708825929535));
#226833=CARTESIAN_POINT('Ctrl Pts',(67.4573422444582,4.56998764048497,127.214523370394));
#226834=CARTESIAN_POINT('Ctrl Pts',(67.1788946206453,-0.550041797684044,
125.019105868103));
#226835=CARTESIAN_POINT('Ctrl Pts',(66.9004469968323,-5.164609694817,128.140054855163));
#226836=CARTESIAN_POINT('Ctrl Pts',(66.6219993730196,-5.03315358762317,
133.709370679297));
#226837=CARTESIAN_POINT('Ctrl Pts',(66.3435517492066,-0.2764752166261,136.609124174332));
#226838=CARTESIAN_POINT('Ctrl Pts',(66.0651041253938,4.73427037188528,134.174583539162));
#226839=CARTESIAN_POINT('Ctrl Pts',(65.7866565015808,5.39445277059944,128.642972683589));
#226840=CARTESIAN_POINT('Ctrl Pts',(65.508208877768,1.0973966068015,125.097571749668));
#226841=CARTESIAN_POINT('Ctrl Pts',(65.2297612539551,-4.20811342784249,
126.796430993211));
#226842=CARTESIAN_POINT('Ctrl Pts',(64.9513136301422,-5.64657280006891,
132.178381763287));
#226843=CARTESIAN_POINT('Ctrl Pts',(64.6728660063292,-1.89610761944867,
136.297674225111));
#226844=CARTESIAN_POINT('Ctrl Pts',(64.3944183825164,3.59678783343796,135.368879844889));
#226845=CARTESIAN_POINT('Ctrl Pts',(64.1159707587035,5.78441098024938,130.245515283918));
#226846=CARTESIAN_POINT('Ctrl Pts',(63.8375231348906,2.65644302039782,125.635702283457));
#226847=CARTESIAN_POINT('Ctrl Pts',(63.5590755110777,-2.91266630074331,
125.775633789045));
#226848=CARTESIAN_POINT('Ctrl Pts',(63.2806278872649,-5.80517758316048,
130.53671958308));
#226849=CARTESIAN_POINT('Ctrl Pts',(63.0021802634519,-3.36301426534433,
135.543754412816));
#226850=CARTESIAN_POINT('Ctrl Pts',(62.723732639639,2.16959486994269,136.195517876976));
#226851=CARTESIAN_POINT('Ctrl Pts',(62.4452850158262,5.70845231035428,131.893071192411));
#226852=CARTESIAN_POINT('Ctrl Pts',(62.1668373920132,4.00152095094907,126.590152676031));
#226853=CARTESIAN_POINT('Ctrl Pts',(61.8883897682004,-1.38261267721222,
125.159885382419));
#226854=CARTESIAN_POINT('Ctrl Pts',(61.6099421443874,-5.49619279939966,
128.916615081961));
#226855=CARTESIAN_POINT('Ctrl Pts',(61.3314945205747,-4.55904024288434,
134.408090707227));
#226856=CARTESIAN_POINT('Ctrl Pts',(61.0530468967616,0.567647575344072,
136.587914432096));
#226857=CARTESIAN_POINT('Ctrl Pts',(60.7745992729488,5.17269500295686,133.452934743723));
#226858=CARTESIAN_POINT('Ctrl Pts',(60.496151649136,5.02428842305186,127.884044823451));
#226859=CARTESIAN_POINT('Ctrl Pts',(60.2177040253229,0.258806232497024,
124.998782452612));
#226860=CARTESIAN_POINT('Ctrl Pts',(59.9392564015102,-4.74450624233532,
127.448562797104));
#226861=CARTESIAN_POINT('Ctrl Pts',(59.6608087776971,-5.38784926247686,
132.982157398764));
#226862=CARTESIAN_POINT('Ctrl Pts',(59.3823611538844,-1.08002202147149,
136.514463149789));
#226863=CARTESIAN_POINT('Ctrl Pts',(59.1039135300714,4.22029269525717,134.799463627718));
#226864=CARTESIAN_POINT('Ctrl Pts',(58.8254659062585,5.64236459780459,129.413159610949));
#226865=CARTESIAN_POINT('Ctrl Pts',(58.5470182824457,1.8793790798041,125.305301355313));
#226866=CARTESIAN_POINT('Ctrl Pts',(58.2685706586328,-3.61066399976409,
126.250809917708));
#226867=CARTESIAN_POINT('Ctrl Pts',(57.9901230348199,-5.78268325429153,
131.380809119953));
#226868=CARTESIAN_POINT('Ctrl Pts',(57.711675411007,-2.64069909790739,135.981080309579));
#226869=CARTESIAN_POINT('Ctrl Pts',(57.4332277871941,2.92795852413098,135.824198999061));
#226870=CARTESIAN_POINT('Ctrl Pts',(57.1547801633813,5.80596530121877,131.054331448687));
#226871=CARTESIAN_POINT('Ctrl Pts',(56.8763325395683,3.34857360366007,126.054752916266));
#226872=CARTESIAN_POINT('Ctrl Pts',(56.5978849157555,-2.18599364874745,
125.419831830104));
#226873=CARTESIAN_POINT('Ctrl Pts',(56.3194372919424,-5.71173952968275,
129.733029650764));
#226874=CARTESIAN_POINT('Ctrl Pts',(56.0409896681298,-3.98867581682796,
135.030728292487));
#226875=CARTESIAN_POINT('Ctrl Pts',(55.7625420443167,1.39978611404518,136.444601510497));
#226876=CARTESIAN_POINT('Ctrl Pts',(55.4840944205039,5.50191298946419,132.675368888989));
#226877=CARTESIAN_POINT('Ctrl Pts',(55.2056467966909,4.54805061095778,127.186771069878));
#226878=CARTESIAN_POINT('Ctrl Pts',(54.9271991728781,-0.585248094394635,
125.022561316018));
#226879=CARTESIAN_POINT('Ctrl Pts',(54.6487515490652,-5.18073239195715,
128.171542663682));
#226880=CARTESIAN_POINT('Ctrl Pts',(54.3703039252523,-5.01537671415865,
133.739955090657));
#226881=CARTESIAN_POINT('Ctrl Pts',(54.0918563014394,-0.241134850822232,
136.610699608625));
#226882=CARTESIAN_POINT('Ctrl Pts',(53.8134086776265,4.75469816032759,134.145702249237));
#226883=CARTESIAN_POINT('Ctrl Pts',(53.5349610538137,5.38119584205463,128.610175163959));
#226884=CARTESIAN_POINT('Ctrl Pts',(53.2565134300007,1.06263743096531,125.090997318624));
#226885=CARTESIAN_POINT('Ctrl Pts',(52.9780658061879,-4.23243286645675,
126.822121231705));
#226886=CARTESIAN_POINT('Ctrl Pts',(52.6996181823749,-5.63810412544538,
132.21272859718));
#226887=CARTESIAN_POINT('Ctrl Pts',(52.4211705585621,-1.86263312984859,
136.309114591992));
#226888=CARTESIAN_POINT('Ctrl Pts',(52.1427229347491,3.62450671739182,135.346900606486));
#226889=CARTESIAN_POINT('Ctrl Pts',(51.8642753109363,5.7809019583462,130.210314286579));
#226890=CARTESIAN_POINT('Ctrl Pts',(51.5858276871234,2.62493071234137,125.619627524071));
#226891=CARTESIAN_POINT('Ctrl Pts',(51.3073800633105,-2.94322362331098,
125.793457186192));
#226892=CARTESIAN_POINT('Ctrl Pts',(51.0289324394976,-5.80669923360788,
130.572062305503));
#226893=CARTESIAN_POINT('Ctrl Pts',(50.7504848156848,-3.33410192124705,
135.564138225197));
#226894=CARTESIAN_POINT('Ctrl Pts',(50.4720371918718,2.20237217680579,136.182211051539));
#226895=CARTESIAN_POINT('Ctrl Pts',(50.193589568059,5.71497383623647,131.858302051661));
#226896=CARTESIAN_POINT('Ctrl Pts',(49.915141944246,3.97579373215887,126.565872361749));
#226897=CARTESIAN_POINT('Ctrl Pts',(49.6366943204332,-1.41694658345112,
125.168406317271));
#226898=CARTESIAN_POINT('Ctrl Pts',(49.3582466966203,-5.50758221055828,
128.950106943089));
#226899=CARTESIAN_POINT('Ctrl Pts',(49.0797990728074,-4.53701884651156,
134.435776110423));
#226900=CARTESIAN_POINT('Ctrl Pts',(48.8013514489945,0.602843191786665,
136.584351844331));
#226901=CARTESIAN_POINT('Ctrl Pts',(48.5229038251815,5.18872178735999,133.421398009111));
#226902=CARTESIAN_POINT('Ctrl Pts',(48.2444562013688,5.006418543501,127.853514660444));
#226903=CARTESIAN_POINT('Ctrl Pts',(47.9660085775558,0.223461235307256,
124.997314589534));
#226904=CARTESIAN_POINT('Ctrl Pts',(47.6875609537429,-4.7648460314457,127.477506128414));
#226905=CARTESIAN_POINT('Ctrl Pts',(47.40911332993,-5.37449257096935,133.014914416948));
#226906=CARTESIAN_POINT('Ctrl Pts',(47.1306657061172,-1.04524299633083,
136.520931755405));
#226907=CARTESIAN_POINT('Ctrl Pts',(46.8522180823042,4.24453382897653,134.773699488214));
#226908=CARTESIAN_POINT('Ctrl Pts',(46.5737704584914,5.6337914224598,129.378838711881));
#226909=CARTESIAN_POINT('Ctrl Pts',(46.2953228346785,1.84586992471411,125.293962926255));
#226910=CARTESIAN_POINT('Ctrl Pts',(46.0168752108656,-3.63831585808481,
126.272873421051));
#226911=CARTESIAN_POINT('Ctrl Pts',(45.7384275870526,-5.77906710891461,
131.415999273987));
#226912=CARTESIAN_POINT('Ctrl Pts',(45.4599799632399,-2.60913800977569,
135.997059081882));
#226913=CARTESIAN_POINT('Ctrl Pts',(45.1815323394269,2.95846145686929,135.806282678493));
#226914=CARTESIAN_POINT('Ctrl Pts',(44.903084715614,5.80737937352832,131.018984258588));
#226915=CARTESIAN_POINT('Ctrl Pts',(44.6246370918012,3.31959935216964,126.034457197533));
#226916=CARTESIAN_POINT('Ctrl Pts',(44.3461894679882,-2.21873030238901,
125.43323835675));
#226917=CARTESIAN_POINT('Ctrl Pts',(44.0677418441753,-5.7181552000533,129.767818479747));
#226918=CARTESIAN_POINT('Ctrl Pts',(43.7892942203624,-3.96287481627985,
135.054930189501));
#226919=CARTESIAN_POINT('Ctrl Pts',(43.5108465965496,1.43409392645716,136.435976114513));
#226920=CARTESIAN_POINT('Ctrl Pts',(43.2323989727367,5.51320041016325,132.641842517543));
#226921=CARTESIAN_POINT('Ctrl Pts',(42.9539513489238,4.52594505174265,127.159152820475));
#226922=CARTESIAN_POINT('Ctrl Pts',(42.6755037251109,-0.620432704521861,
125.026231010632));
#226923=CARTESIAN_POINT('Ctrl Pts',(42.397056101298,-5.19666311515333,128.203128032237));
#226924=CARTESIAN_POINT('Ctrl Pts',(42.1186084774851,-4.99741399406557,
133.770430722483));
#226925=CARTESIAN_POINT('Ctrl Pts',(41.8401608536722,-0.205785549677785,
136.612059886891));
#226926=CARTESIAN_POINT('Ctrl Pts',(41.5617132298594,4.77494976168102,134.11669714467));
#226927=CARTESIAN_POINT('Ctrl Pts',(41.2832656060464,5.36773951131901,128.577458950676));
#226928=CARTESIAN_POINT('Ctrl Pts',(41.0048179822336,1.02783887870806,125.084634598359));
#226929=CARTESIAN_POINT('Ctrl Pts',(40.7263703584206,-4.25659547071474,
126.847959033542));
#226930=CARTESIAN_POINT('Ctrl Pts',(40.4479227346078,-5.62942652880005,
132.24702324348));
#226931=CARTESIAN_POINT('Ctrl Pts',(40.1694751107948,-1.82908961969292,
136.320350978189));
#226932=CARTESIAN_POINT('Ctrl Pts',(39.891027486982,3.65209129391637,135.324753042595));
#226933=CARTESIAN_POINT('Ctrl Pts',(39.6125798631691,5.77717872299504,130.175135301845));
#226934=CARTESIAN_POINT('Ctrl Pts',(39.3341322393562,2.59332113651206,125.603744886877));
#226935=CARTESIAN_POINT('Ctrl Pts',(39.0556846155433,-2.97367188364494,
125.811466264208));
#226936=CARTESIAN_POINT('Ctrl Pts',(38.7772369917304,-5.80800571467979,
130.607413635826));
#226937=CARTESIAN_POINT('Ctrl Pts',(38.4987893679175,-3.30506603077697,
135.584345662267));
#226938=CARTESIAN_POINT('Ctrl Pts',(38.2203417441046,2.23506787395795,136.16870494788));
#226939=CARTESIAN_POINT('Ctrl Pts',(37.9418941202917,5.72128359166147,131.823493856722));
#226940=CARTESIAN_POINT('Ctrl Pts',(37.6634464964789,3.94991918886983,126.541749106207));
#226941=CARTESIAN_POINT('Ctrl Pts',(37.3849988726659,-1.45122798421329,
125.177136094481));
#226942=CARTESIAN_POINT('Ctrl Pts',(37.1065512488531,-5.51876753623267,
128.983667514269));
#226943=CARTESIAN_POINT('Ctrl Pts',(36.8281036250402,-4.51482932923697,
134.463326950183));
#226944=CARTESIAN_POINT('Ctrl Pts',(36.5496560012273,0.6380164696531,136.580575076865));
#226945=CARTESIAN_POINT('Ctrl Pts',(36.2712083774144,5.20455630176915,133.389764299214));
#226946=CARTESIAN_POINT('Ctrl Pts',(35.9927607536015,4.9883631492699,127.82309384212));
#226947=CARTESIAN_POINT('Ctrl Pts',(35.7143131297886,0.188107957679239,
124.996061908681));
#226948=CARTESIAN_POINT('Ctrl Pts',(35.4358655059757,-4.78500925743413,
127.50657273754));
#226949=CARTESIAN_POINT('Ctrl Pts',(35.1574178821628,-5.36093672566315,
133.047589522248));
#226950=CARTESIAN_POINT('Ctrl Pts',(34.87897025835,-1.01042523932657,136.527188531377));
#226951=CARTESIAN_POINT('Ctrl Pts',(34.6005226345371,4.26861767993396,134.747788263399));
#226952=CARTESIAN_POINT('Ctrl Pts',(34.3220750107242,5.62500948490202,129.34457063605));
#226953=CARTESIAN_POINT('Ctrl Pts',(34.0436273869112,1.81229237023524,125.282828687009));
#226954=CARTESIAN_POINT('Ctrl Pts',(33.7651797630984,-3.66583289727342,
126.295104840318));
#226955=CARTESIAN_POINT('Ctrl Pts',(33.4867321392855,-5.77523681808073,
131.451166763527));
#226956=CARTESIAN_POINT('Ctrl Pts',(33.2082845154725,-2.57748023907555,
136.012845436834));
#226957=CARTESIAN_POINT('Ctrl Pts',(32.9298368916598,2.98885476273036,135.788181009863));
#226958=CARTESIAN_POINT('Ctrl Pts',(32.6513892678468,5.80857825125962,130.983629115531));
#226959=CARTESIAN_POINT('Ctrl Pts',(32.3729416440339,3.29050209170421,126.014338229324));
#226960=CARTESIAN_POINT('Ctrl Pts',(32.094494020221,-2.25138474016344,125.446843912307));
#226961=CARTESIAN_POINT('Ctrl Pts',(31.8160463964081,-5.72435898208005,
129.802645718181));
#226962=CARTESIAN_POINT('Ctrl Pts',(31.5375987725953,-3.93692696994811,
135.078974580096));
#226963=CARTESIAN_POINT('Ctrl Pts',(31.2591511487823,1.46834859799131,136.427142036947));
#226964=CARTESIAN_POINT('Ctrl Pts',(30.9807035249695,5.52428353719365,132.608248057529));
#226965=CARTESIAN_POINT('Ctrl Pts',(30.7022559011566,4.50367178196922,127.131669645585));
#226966=CARTESIAN_POINT('Ctrl Pts',(30.4238082773436,-0.655594324287056,
125.030114815962));
#226967=CARTESIAN_POINT('Ctrl Pts',(30.1453606535308,-5.21240127408669,
128.234809790423));
#226968=CARTESIAN_POINT('Ctrl Pts',(29.8669130297179,-4.97926609295916,
133.80079644549));
#226969=CARTESIAN_POINT('Ctrl Pts',(29.588465405905,-0.170428623074124,
136.613204958723));
#226970=CARTESIAN_POINT('Ctrl Pts',(29.3100177820921,4.79502442551506,134.087569300254));
#226971=CARTESIAN_POINT('Ctrl Pts',(29.0315701582792,5.35408427702179,128.544825256054));
#226972=CARTESIAN_POINT('Ctrl Pts',(28.7531225344664,0.99300223950345,125.078483824645));
#226973=CARTESIAN_POINT('Ctrl Pts',(28.4746749106534,-4.28060034526213,
126.873943441297));
#226974=CARTESIAN_POINT('Ctrl Pts',(28.1962272868406,-5.6205403316845,132.281264431386));
#226975=CARTESIAN_POINT('Ctrl Pts',(27.9177796630277,-1.79547833194873,
136.331382967337));
#226976=CARTESIAN_POINT('Ctrl Pts',(27.6393320392148,3.67954054085496,135.3024379739));
#226977=CARTESIAN_POINT('Ctrl Pts',(27.3608844154018,5.77324141216173,130.139979633288));
#226978=CARTESIAN_POINT('Ctrl Pts',(27.082436791589,2.56161546421434,125.58805496041));
#226979=CARTESIAN_POINT('Ctrl Pts',(26.8039891677761,-3.00400995347367,
125.82966035576));
#226980=CARTESIAN_POINT('Ctrl Pts',(26.5255415439632,-5.80909697796402,
130.642772264091));
#226981=CARTESIAN_POINT('Ctrl Pts',(26.2470939201503,-3.27590766986969,
135.604375975235));
#226982=CARTESIAN_POINT('Ctrl Pts',(25.9686462963375,2.2676807498481,136.155000066467));
#226983=CARTESIAN_POINT('Ctrl Pts',(25.6901986725246,5.727381342819,131.788647897428));
#226984=CARTESIAN_POINT('Ctrl Pts',(25.4117510487116,3.92389827987267,126.517783803302));
#226985=CARTESIAN_POINT('Ctrl Pts',(25.1333034248988,-1.48545560918882,
125.186074390566));
#226986=CARTESIAN_POINT('Ctrl Pts',(24.8548558010858,-5.5297483619465,129.017295551901));
#226987=CARTESIAN_POINT('Ctrl Pts',(24.576408177273,-4.49247251330123,134.490742205601));
#226988=CARTESIAN_POINT('Ctrl Pts',(24.2979605534601,0.673166105584617,
136.576584269648));
#226989=CARTESIAN_POINT('Ctrl Pts',(24.0195129296472,5.22019795943058,133.358034786234));
#226990=CARTESIAN_POINT('Ctrl Pts',(23.7410653058343,4.97012290940784,127.792783495733));
#226991=CARTESIAN_POINT('Ctrl Pts',(23.4626176820214,0.152747709641667,
124.995024456474));
#226992=CARTESIAN_POINT('Ctrl Pts',(23.1841700582085,-4.80499517314482,
127.53576154741));
#226993=CARTESIAN_POINT('Ctrl Pts',(22.9057224343956,-5.34718222887511,
133.080181503877));
#226994=CARTESIAN_POINT('Ctrl Pts',(22.6272748105827,-0.975570040643468,
136.533233245855));
#226995=CARTESIAN_POINT('Ctrl Pts',(22.3488271867698,4.29254335569345,134.721730913422));
#226996=CARTESIAN_POINT('Ctrl Pts',(22.070379562957,5.61601911054919,129.310356653276));
#226997=CARTESIAN_POINT('Ctrl Pts',(21.791931939144,1.77864766059611,125.27189905016));
#226998=CARTESIAN_POINT('Ctrl Pts',(21.5134843153312,-3.69321409767591,
126.317503351717));
#226999=CARTESIAN_POINT('Ctrl Pts',(21.2350366915183,-5.77119252372273,
131.486310285425));
#227000=CARTESIAN_POINT('Ctrl Pts',(20.9565890677054,-2.54572695889727,
136.028438789465));
#227001=CARTESIAN_POINT('Ctrl Pts',(20.6781414438925,3.01913731547902,135.769894663934));
#227002=CARTESIAN_POINT('Ctrl Pts',(20.3996938200796,5.80956188998761,130.948267329615));
#227003=CARTESIAN_POINT('Ctrl Pts',(20.1212461962667,3.26128290047392,125.994396757156));
#227004=CARTESIAN_POINT('Ctrl Pts',(19.8427985724538,-2.28395575204823,
125.460647992615));
#227005=CARTESIAN_POINT('Ctrl Pts',(19.5643509486409,-5.7303506458796,129.837510075529));
#227006=CARTESIAN_POINT('Ctrl Pts',(19.285903324828,-3.91083323933969,135.102860573299));
#227007=CARTESIAN_POINT('Ctrl Pts',(19.0074557010152,1.50254885932817,136.418099605148));
#227008=CARTESIAN_POINT('Ctrl Pts',(18.7290080772022,5.53516195986603,132.574586753804));
#227009=CARTESIAN_POINT('Ctrl Pts',(18.4505604533894,4.48123162698169,127.104322563612));
#227010=CARTESIAN_POINT('Ctrl Pts',(18.1721128295765,-0.690731650763477,
125.034212588094));
#227011=CARTESIAN_POINT('Ctrl Pts',(17.8936652057636,-5.22794628557398,
128.26658676426));
#227012=CARTESIAN_POINT('Ctrl Pts',(17.6152175819507,-4.96093368331654,
133.831051134467));
#227013=CARTESIAN_POINT('Ctrl Pts',(17.3367699581378,-0.135065381175154,
136.614134781694));
#227014=CARTESIAN_POINT('Ctrl Pts',(17.0583223343249,4.81492140795562,134.058319795333));
#227015=CARTESIAN_POINT('Ctrl Pts',(16.779874710512,5.34023064516271,128.512275289347));
#227016=CARTESIAN_POINT('Ctrl Pts',(16.5014270866992,0.958128804235671,
125.0725452254));
#227017=CARTESIAN_POINT('Ctrl Pts',(16.2229794628862,-4.30444660058956,
126.900073492105));
#227018=CARTESIAN_POINT('Ctrl Pts',(15.9445318390734,-5.61144586338,132.315450892077));
#227019=CARTESIAN_POINT('Ctrl Pts',(15.6660842152604,-1.76180051209467,
136.342210150638));
#227020=CARTESIAN_POINT('Ctrl Pts',(15.3876365914476,3.70685344106567,135.279956227294));
#227021=CARTESIAN_POINT('Ctrl Pts',(15.1091889676347,5.76909017174479,130.104848583611));
#227022=CARTESIAN_POINT('Ctrl Pts',(14.8307413438218,2.52981487031356,125.572558326068));
#227023=CARTESIAN_POINT('Ctrl Pts',(14.5522937200089,-3.03423670860886,
125.848038786661));
#227024=CARTESIAN_POINT('Ctrl Pts',(14.273846096196,-5.80997298302346,130.678136880072));
#227025=CARTESIAN_POINT('Ctrl Pts',(13.9953984723831,-3.24662791899898,
135.624228421867));
#227026=CARTESIAN_POINT('Ctrl Pts',(13.7169508485702,2.30020959599411,136.141096915141));
#227027=CARTESIAN_POINT('Ctrl Pts',(13.4385032247574,5.73326686375462,131.753765465006));
#227028=CARTESIAN_POINT('Ctrl Pts',(13.1600556009444,3.89773196938174,126.493977341077));
#227029=CARTESIAN_POINT('Ctrl Pts',(12.8816079771316,-1.51962819006047,
125.195220874312));
#227030=CARTESIAN_POINT('Ctrl Pts',(12.6031603533186,-5.54052428080121,
129.050989809886));
#227031=CARTESIAN_POINT('Ctrl Pts',(12.3247127295058,-4.46994922714442,
134.518020860792));
#227032=CARTESIAN_POINT('Ctrl Pts',(12.0462651056929,0.708290797098533,
136.572379570561));
#227033=CARTESIAN_POINT('Ctrl Pts',(11.76781748188,5.23564618073708,133.326210645918));
#227034=CARTESIAN_POINT('Ctrl Pts',(11.4893698580671,4.95169849981347,127.762584744442));
#227035=CARTESIAN_POINT('Ctrl Pts',(11.2109222342542,0.117381801481337,
124.994202271355));
#227036=CARTESIAN_POINT('Ctrl Pts',(10.9324746104413,-4.82480303799234,
127.565071476419));
#227037=CARTESIAN_POINT('Ctrl Pts',(10.6540269866284,-5.33322959028317,
133.112689154126));
#227038=CARTESIAN_POINT('Ctrl Pts',(10.3755793628155,-0.940678691853753,
136.539065674851));
#227039=CARTESIAN_POINT('Ctrl Pts',(10.0971317390026,4.31630996968034,134.695528403849));
#227040=CARTESIAN_POINT('Ctrl Pts',(9.81868411518972,5.60682063254294,129.276198031366));
#227041=CARTESIAN_POINT('Ctrl Pts',(9.54023649137686,1.74493704251384,125.261174420708));
#227042=CARTESIAN_POINT('Ctrl Pts',(9.26178886756394,-3.72045844467185,
126.340068125262));
#227043=CARTESIAN_POINT('Ctrl Pts',(8.98334124375105,-5.76693437570339,
131.52142853743));
#227044=CARTESIAN_POINT('Ctrl Pts',(8.70489361993813,-2.51387934587036,
136.043838561958));
#227045=CARTESIAN_POINT('Ctrl Pts',(8.42644599612531,3.0493079929842,135.751424318317));
#227046=CARTESIAN_POINT('Ctrl Pts',(8.14799837231237,5.81033025326331,130.912900211183));
#227047=CARTESIAN_POINT('Ctrl Pts',(7.86955074849947,3.23194286120641,125.974633519968));
#227048=CARTESIAN_POINT('Ctrl Pts',(7.59110312468663,-2.3164421311127,125.47465008616));
#227049=CARTESIAN_POINT('Ctrl Pts',(7.31265550087371,-5.73612996942864,
129.872410259879));
#227050=CARTESIAN_POINT('Ctrl Pts',(7.0342078770608,-3.88459459136738,135.126587284006));
#227051=CARTESIAN_POINT('Ctrl Pts',(6.75576025324794,1.53669344316449,136.408849154185));
#227052=CARTESIAN_POINT('Ctrl Pts',(6.47731262943506,5.54583527507644,132.540859853697));
#227053=CARTESIAN_POINT('Ctrl Pts',(6.19886500562214,4.45862541830825,127.077112587908));
#227054=CARTESIAN_POINT('Ctrl Pts',(5.92041738180924,-0.725843381924555,
125.038524175185));
#227055=CARTESIAN_POINT('Ctrl Pts',(5.64196975799638,-5.24329757358911,
128.29845777624));
#227056=CARTESIAN_POINT('Ctrl Pts',(5.36352213418349,-4.94241744445191,
133.861193668313));
#227057=CARTESIAN_POINT('Ctrl Pts',(5.08507451037056,-0.0996971343788212,
136.614849321347));
#227058=CARTESIAN_POINT('Ctrl Pts',(4.80662688655771,4.83463997171276,134.028949713759));
#227059=CARTESIAN_POINT('Ctrl Pts',(4.5281792627448,5.32617912909322,128.479810256704));
#227060=CARTESIAN_POINT('Ctrl Pts',(4.24973163893191,0.923219865152705,
125.066819020683));
#227061=CARTESIAN_POINT('Ctrl Pts',(3.97128401511898,-4.32813335306523,
126.926348217707));
#227062=CARTESIAN_POINT('Ctrl Pts',(3.69283639130614,-5.60214346088543,
132.349581358763));
#227063=CARTESIAN_POINT('Ctrl Pts',(3.41438876749324,-1.72805740807474,
136.352832126888));
#227064=CARTESIAN_POINT('Ctrl Pts',(3.13594114368033,3.73402898245891,135.257308635848));
#227065=CARTESIAN_POINT('Ctrl Pts',(2.85749351986744,5.76472515556999,130.06974345461));
#227066=CARTESIAN_POINT('Ctrl Pts',(2.5790458960546,2.49792053319242,125.557255558086));
#227067=CARTESIAN_POINT('Ctrl Pts',(2.30059827224166,-3.06435102898697,
125.866600875889));
#227068=CARTESIAN_POINT('Ctrl Pts',(2.02215064842876,-5.81063369739741,
130.713506173321));
#227069=CARTESIAN_POINT('Ctrl Pts',(1.74370302461591,-3.21722786313679,
135.643902266527));
#227070=CARTESIAN_POINT('Ctrl Pts',(1.46525540080302,2.33265320702766,136.12699600909));
#227071=CARTESIAN_POINT('Ctrl Pts',(1.18680777699008,5.73893993637821,131.718847852038));
#227072=CARTESIAN_POINT('Ctrl Pts',(0.908360153177235,3.87142122699929,
126.47033060169));
#227073=CARTESIAN_POINT('Ctrl Pts',(0.629912529364331,-1.55374446055069,
125.204575206795));
#227074=CARTESIAN_POINT('Ctrl Pts',(0.351464905551429,-5.55109489349118,
129.084749039672));
#227075=CARTESIAN_POINT('Ctrl Pts',(0.0730172817385382,-4.44726030537518,
134.545161904937));
#227076=CARTESIAN_POINT('Ctrl Pts',(-0.205430342074321,0.743389242636492,
136.56796113541));
#227077=CARTESIAN_POINT('Ctrl Pts',(-0.48387796588724,5.25090039324876,
133.294293057522));
#227078=CARTESIAN_POINT('Ctrl Pts',(-0.762325589700153,4.93309060321035,
127.732498707276));
#227079=CARTESIAN_POINT('Ctrl Pts',(-1.040773213513,0.0820115436953976,
124.993595383789));
#227080=CARTESIAN_POINT('Ctrl Pts',(-1.3192208373259,-4.84443211798899,
127.594501438479));
#227081=CARTESIAN_POINT('Ctrl Pts',(-1.5976684611388,-5.31907932690746,
133.145111268411));
#227082=CARTESIAN_POINT('Ctrl Pts',(-1.8761160849517,-0.905752485869179,
136.544685602242));
#227083=CARTESIAN_POINT('Ctrl Pts',(-2.15456370876455,4.33991664121397,
134.669181705622));
#227084=CARTESIAN_POINT('Ctrl Pts',(-2.43301133257747,5.59741439173625,
129.242096036083));
#227085=CARTESIAN_POINT('Ctrl Pts',(-2.71145895639038,1.71116176514775,
125.250655196059));
#227086=CARTESIAN_POINT('Ctrl Pts',(-2.98990658020324,-3.74756492871192,
126.362798324807));
#227087=CARTESIAN_POINT('Ctrl Pts',(-3.26835420401613,-5.76246253181,131.556520218218));
#227088=CARTESIAN_POINT('Ctrl Pts',(-3.54680182782904,-2.48193858011979,
136.059044183669));
#227089=CARTESIAN_POINT('Ctrl Pts',(-3.82524945164193,3.0793656772603,135.732770657435));
#227090=CARTESIAN_POINT('Ctrl Pts',(-4.1036970754548,5.81088331261472,130.877529070775));
#227091=CARTESIAN_POINT('Ctrl Pts',(-4.38214469926771,3.20248306110764,
125.955049250094));
#227092=CARTESIAN_POINT('Ctrl Pts',(-4.66059232308062,-2.34884267356213,
125.488849674089));
#227093=CARTESIAN_POINT('Ctrl Pts',(-4.93903994689347,-5.7416967385722,
129.907344977992));
#227094=CARTESIAN_POINT('Ctrl Pts',(-5.21748757070636,-3.85821199831392,
135.150153833014));
#227095=CARTESIAN_POINT('Ctrl Pts',(-5.49593519451928,1.57078108426016,
136.399391026839));
#227096=CARTESIAN_POINT('Ctrl Pts',(-5.77438281833216,5.55630308732125,
132.507068606974));
#227097=CARTESIAN_POINT('Ctrl Pts',(-6.05283044214503,4.43585399363028,
127.050040726751));
#227098=CARTESIAN_POINT('Ctrl Pts',(-6.33127806595794,-0.76092821669219,
125.043049417465));
#227099=CARTESIAN_POINT('Ctrl Pts',(-6.60972568977086,-5.25845456928442,
128.330421645371));
#227100=CARTESIAN_POINT('Ctrl Pts',(-6.88817331358369,-4.92371806249131,
133.891222930087));
#227101=CARTESIAN_POINT('Ctrl Pts',(-7.16662093739661,-0.0643251932685087,
136.615348551203));
#227102=CARTESIAN_POINT('Ctrl Pts',(-7.44506856120951,4.8541793861078,133.999460143849));
#227103=CARTESIAN_POINT('Ctrl Pts',(-7.72351618502242,5.3119302494974,128.44743136113));
#227104=CARTESIAN_POINT('Ctrl Pts',(-8.00196380883526,0.888276715818123,
125.06130542268));
#227105=CARTESIAN_POINT('Ctrl Pts',(-8.28041143264819,-4.35165972496785,
126.952766644486));
#227106=CARTESIAN_POINT('Ctrl Pts',(-8.55885905646108,-5.59263346890473,
132.383654566726));
#227107=CARTESIAN_POINT('Ctrl Pts',(-8.83730668027396,-1.69425027025207,
136.363248502487));
#227108=CARTESIAN_POINT('Ctrl Pts',(-9.11575430408684,3.76106615803527,
135.234496038775));
#227109=CARTESIAN_POINT('Ctrl Pts',(-9.39420192789976,5.7601465253845,130.034665547118));
#227110=CARTESIAN_POINT('Ctrl Pts',(-9.67264955171265,2.4659336347071,125.542147223509));
#227111=CARTESIAN_POINT('Ctrl Pts',(-9.95109717552551,-3.09435179871079,
125.885345935621));
#227112=CARTESIAN_POINT('Ctrl Pts',(-10.2295447993384,-5.81107909660284,
130.748878833214));
#227113=CARTESIAN_POINT('Ctrl Pts',(-10.5079924231513,-3.18770859171301,
135.663396780189));
#227114=CARTESIAN_POINT('Ctrl Pts',(-10.7864400469642,2.36501038073878,
136.112697870828));
#227115=CARTESIAN_POINT('Ctrl Pts',(-11.0648876707771,5.74440035047196,
131.683896352409));
#227116=CARTESIAN_POINT('Ctrl Pts',(-11.34333529459,3.84496702767957,126.446844461378));
#227117=CARTESIAN_POINT('Ctrl Pts',(-11.6217829184029,-1.58780315646856,
125.214137041385));
#227118=CARTESIAN_POINT('Ctrl Pts',(-11.9002305422157,-5.56145980831845,
129.118571990297));
#227119=CARTESIAN_POINT('Ctrl Pts',(-12.1786781660286,-4.42440658873985,
134.572164332316));
#227120=CARTESIAN_POINT('Ctrl Pts',(-12.4571257898416,0.778460141612691,
136.563329127923));
#227121=CARTESIAN_POINT('Ctrl Pts',(-12.7355734136544,5.26596003171537,
133.262283203764));
#227122=CARTESIAN_POINT('Ctrl Pts',(-13.0140210374673,4.91429990912079,
127.702526499083));
#227123=CARTESIAN_POINT('Ctrl Pts',(-13.2924686612802,0.0466382469415425,
124.993203816266));
#227124=CARTESIAN_POINT('Ctrl Pts',(-13.5709162850931,-4.86388168577195,
127.624050343051));
#227125=CARTESIAN_POINT('Ctrl Pts',(-13.849363908906,-5.30473196309121,
133.177446645321));
#227126=CARTESIAN_POINT('Ctrl Pts',(-14.1278115327188,-0.87079271689315,
136.550092819781));
#227127=CARTESIAN_POINT('Ctrl Pts',(-14.4062591565318,4.36336249554048,
134.642691795028));
#227128=CARTESIAN_POINT('Ctrl Pts',(-14.6847067803446,5.58780073668082,
129.20805193109));
#227129=CARTESIAN_POINT('Ctrl Pts',(-14.9631544041576,1.67732308005318,
125.240341766008));
#227130=CARTESIAN_POINT('Ctrl Pts',(-15.2416020279704,-3.77453254535539,
126.385693108075));
#227131=CARTESIAN_POINT('Ctrl Pts',(-15.5200496517834,-5.75777715774833,
131.591584027456));
#227132=CARTESIAN_POINT('Ctrl Pts',(-15.7984972755962,-2.44990584522241,
136.074055091149));
#227133=CARTESIAN_POINT('Ctrl Pts',(-16.0769448994091,3.1093092545088,135.713934372506));
#227134=CARTESIAN_POINT('Ctrl Pts',(-16.355392523222,5.81122104754806,130.842155219084));
#227135=CARTESIAN_POINT('Ctrl Pts',(-16.6338401470349,3.17290459182133,
125.935644673236));
#227136=CARTESIAN_POINT('Ctrl Pts',(-16.9122877708478,-2.38115617878252,
125.50324623023));
#227137=CARTESIAN_POINT('Ctrl Pts',(-17.1907353946607,-5.74705074703162,
129.94231293535));
#227138=CARTESIAN_POINT('Ctrl Pts',(-17.4691830184736,-3.83168643779603,
135.173559347056));
#227139=CARTESIAN_POINT('Ctrl Pts',(-17.7476306422864,1.6048105194851,136.389725573584));
#227140=CARTESIAN_POINT('Ctrl Pts',(-18.0260782660994,5.56656500871184,
132.473214265779));
#227141=CARTESIAN_POINT('Ctrl Pts',(-18.3045258899123,4.4129181967513,127.023107983299));
#227142=CARTESIAN_POINT('Ctrl Pts',(-18.5829735137251,-0.795984854984928,
125.047788147249));
#227143=CARTESIAN_POINT('Ctrl Pts',(-18.861421137538,-5.27341671101187,
128.362477187221));
#227144=CARTESIAN_POINT('Ctrl Pts',(-19.1398687613509,-4.90483623034722,
133.921137807042));
#227145=CARTESIAN_POINT('Ctrl Pts',(-19.4183163851638,-0.0289508685644962,
136.615632452765));
#227146=CARTESIAN_POINT('Ctrl Pts',(-19.6967640089767,4.87353892710056,
133.969852178351));
#227147=CARTESIAN_POINT('Ctrl Pts',(-19.9752116327896,5.29748453437273,
128.415139802436));
#227148=CARTESIAN_POINT('Ctrl Pts',(-20.2536592566025,0.853300651063172,
125.056004635698));
#227149=CARTESIAN_POINT('Ctrl Pts',(-20.5321068804154,-4.37502484451904,
126.979327793496));
#227150=CARTESIAN_POINT('Ctrl Pts',(-20.8105545042282,-5.58291623983416,
132.417669253371));
#227151=CARTESIAN_POINT('Ctrl Pts',(-21.0890021280412,-1.66038035136256,
136.37345889145));
#227152=CARTESIAN_POINT('Ctrl Pts',(-21.367449751854,3.78796396592178,135.211519281404));
#227153=CARTESIAN_POINT('Ctrl Pts',(-21.6458973756669,5.75535445085128,
129.999616160961));
#227154=CARTESIAN_POINT('Ctrl Pts',(-21.9243449994798,2.43385536014432,
125.527233882186));
#227155=CARTESIAN_POINT('Ctrl Pts',(-22.2027926232928,-3.12423790609075,
125.904273271251));
#227156=CARTESIAN_POINT('Ctrl Pts',(-22.4812402471056,-5.81130916413533,
130.784253549004));
#227157=CARTESIAN_POINT('Ctrl Pts',(-22.7596878709185,-3.15807119857507,
135.682711240481));
#227158=CARTESIAN_POINT('Ctrl Pts',(-23.0381354947314,2.39727991812053,
136.098203030175));
#227159=CARTESIAN_POINT('Ctrl Pts',(-23.3165831185443,5.74964790369824,
131.648912261261));
#227160=CARTESIAN_POINT('Ctrl Pts',(-23.5950307423572,3.81837035169266,
126.423519790431));
#227161=CARTESIAN_POINT('Ctrl Pts',(-23.8734783661701,-1.62180301575654,
125.223906023766));
#227162=CARTESIAN_POINT('Ctrl Pts',(-24.151925989983,-5.57161864120731,
129.15245740844));
#227163=CARTESIAN_POINT('Ctrl Pts',(-24.4303736137958,-4.4013889240913,
134.599027142342));
#227164=CARTESIAN_POINT('Ctrl Pts',(-24.7088212376087,0.813502194462058,
136.558483719739));
#227165=CARTESIAN_POINT('Ctrl Pts',(-24.9872688614217,5.28082453809644,
133.230182270781));
#227166=CARTESIAN_POINT('Ctrl Pts',(-25.2657164852345,4.89532711384086,
127.672669230493));
#227167=CARTESIAN_POINT('Ctrl Pts',(-25.5441641090475,0.0112632219902977,
124.993027583295));
#227168=CARTESIAN_POINT('Ctrl Pts',(-25.8226117328602,-4.88315102063038,
127.65371709519));
#227169=CARTESIAN_POINT('Ctrl Pts',(-26.1010593566733,-5.29018803048126,
133.209694086655));
#227170=CARTESIAN_POINT('Ctrl Pts',(-26.3795069804861,-0.835800680372761,
136.555287127099));
#227171=CARTESIAN_POINT('Ctrl Pts',(-26.6579546042989,4.38664666386508,
134.616059653661));
#227172=CARTESIAN_POINT('Ctrl Pts',(-26.9364022281119,5.57798002361419,
129.174066977901));
#227173=CARTESIAN_POINT('Ctrl Pts',(-27.2148498519247,1.64342224113504,
125.23023451272));
#227174=CARTESIAN_POINT('Ctrl Pts',(-27.4932974757377,-3.80136029530733,
126.408751626694));
#227175=CARTESIAN_POINT('Ctrl Pts',(-27.7717450995505,-5.75287842713667,
131.626618665841));
#227176=CARTESIAN_POINT('Ctrl Pts',(-28.0501927233634,-2.41778232816299,
136.088870728161));
#227177=CARTESIAN_POINT('Ctrl Pts',(-28.3286403471763,3.13913761515943,
135.694916161515));
#227178=CARTESIAN_POINT('Ctrl Pts',(-28.6070879709892,5.8113434455484,130.8067799669));
#227179=CARTESIAN_POINT('Ctrl Pts',(-28.8855355948021,3.14320854938853,
125.916420508438));
#227180=CARTESIAN_POINT('Ctrl Pts',(-29.163983218615,-2.41338144938502,
125.517839221114));
#227181=CARTESIAN_POINT('Ctrl Pts',(-29.4424308424279,-5.75219179641212,
129.977312836202));
#227182=CARTESIAN_POINT('Ctrl Pts',(-29.7208784662408,-3.80501889272807,
135.196802958832));
#227183=CARTESIAN_POINT('Ctrl Pts',(-29.9993260900537,1.6387804878663,136.379853152576));
#227184=CARTESIAN_POINT('Ctrl Pts',(-30.2777737138665,5.576620658989,132.439298084597));
#227185=CARTESIAN_POINT('Ctrl Pts',(-30.5562213376795,4.38981887756547,
126.996315355552));
#227186=CARTESIAN_POINT('Ctrl Pts',(-30.8346689614924,-0.831011997766135,
125.052740188944));
#227187=CARTESIAN_POINT('Ctrl Pts',(-31.1131165853052,-5.2881834443438,
128.394623213959));
#227188=CARTESIAN_POINT('Ctrl Pts',(-31.3915642091181,-4.88577264769286,
133.950937190672));
#227189=CARTESIAN_POINT('Ctrl Pts',(-31.670011832931,0.00642452892459172,
136.615701015511));
#227190=CARTESIAN_POINT('Ctrl Pts',(-31.9484594567439,4.89271787731614,
133.940126914399));
#227191=CARTESIAN_POINT('Ctrl Pts',(-32.2269070805568,5.28284251901049,
128.382936777197));
#227192=CARTESIAN_POINT('Ctrl Pts',(-32.5053547043697,0.818292966938792,
125.050916856162));
#227193=CARTESIAN_POINT('Ctrl Pts',(-32.7838023281826,-4.3982278459157,
127.006030680504));
#227194=CARTESIAN_POINT('Ctrl Pts',(-33.0622499519955,-5.57299213374921,
132.451624158271));
#227195=CARTESIAN_POINT('Ctrl Pts',(-33.3406975758084,-1.62644890646854,
136.383462915428));
#227196=CARTESIAN_POINT('Ctrl Pts',(-33.6191451996212,3.81472140941051,
135.188379215148));
#227197=CARTESIAN_POINT('Ctrl Pts',(-33.8975928234342,5.75034910954236,
129.964596594906));
#227198=CARTESIAN_POINT('Ctrl Pts',(-34.176040447247,2.40168689817613,125.512516086734));
#227199=CARTESIAN_POINT('Ctrl Pts',(-34.4544880710599,-3.15400824368619,
125.923382181419));
#227200=CARTESIAN_POINT('Ctrl Pts',(-34.7329356948729,-5.81132389146964,
130.81962900987));
#227201=CARTESIAN_POINT('Ctrl Pts',(-35.0113833186857,-3.1283167819475,
135.701844931696));
#227202=CARTESIAN_POINT('Ctrl Pts',(-35.2898309424986,2.42946062341331,
136.083512024245));
#227203=CARTESIAN_POINT('Ctrl Pts',(-35.5682785663115,5.75468240160701,
131.613896874941));
#227204=CARTESIAN_POINT('Ctrl Pts',(-35.8467261901244,3.79163218458816,
126.400357453152));
#227205=CARTESIAN_POINT('Ctrl Pts',(-36.1251738139373,-1.65574277853735,
125.233881791944));
#227206=CARTESIAN_POINT('Ctrl Pts',(-36.4036214377501,-5.58157101571846,
129.186404038463));
#227207=CARTESIAN_POINT('Ctrl Pts',(-36.6820690615631,-4.37820816435757,
134.625749339604));
#227208=CARTESIAN_POINT('Ctrl Pts',(-36.960516685376,0.848514102688449,
136.553425090409));
#227209=CARTESIAN_POINT('Ctrl Pts',(-37.2389643091888,5.29549336158222,
133.197991448084));
#227210=CARTESIAN_POINT('Ctrl Pts',(-37.5174119330018,4.87617292041449,
127.64292800788));
#227211=CARTESIAN_POINT('Ctrl Pts',(-37.7958595568146,-0.0241122203237842,
124.993066691407));
#227212=CARTESIAN_POINT('Ctrl Pts',(-38.0743071806275,-4.90223940853195,
127.683500595584));
#227213=CARTESIAN_POINT('Ctrl Pts',(-38.3527548044404,-5.27544806800837,
133.241852397473));
#227214=CARTESIAN_POINT('Ctrl Pts',(-38.6312024282533,-0.800777672950798,
136.560268331721));
#227215=CARTESIAN_POINT('Ctrl Pts',(-38.9096500520661,4.40976828338437,
134.589286268384));
#227216=CARTESIAN_POINT('Ctrl Pts',(-39.1880976758791,5.56795261644649,
129.140142435842));
#227217=CARTESIAN_POINT('Ctrl Pts',(-39.4665452996919,1.6094605046014,125.220333810727));
#227218=CARTESIAN_POINT('Ctrl Pts',(-39.7449929235049,-3.82804718445556,
126.43197302622));
#227219=CARTESIAN_POINT('Ctrl Pts',(-40.0234405473177,-5.74776652149929,
131.661622835152));
#227220=CARTESIAN_POINT('Ctrl Pts',(-40.3018881711306,-2.38556921929025,
136.103490545709));
#227221=CARTESIAN_POINT('Ctrl Pts',(-40.5803357949436,3.16884965391132,
135.675716729192));
#227222=CARTESIAN_POINT('Ctrl Pts',(-40.8587834187564,5.81125050208024,
130.771404625066));
#227223=CARTESIAN_POINT('Ctrl Pts',(-41.1372310425694,3.11339603420704,
125.897377468058));
#227224=CARTESIAN_POINT('Ctrl Pts',(-41.4156786663821,-2.4455172912504,
125.532628105994));
#227225=CARTESIAN_POINT('Ctrl Pts',(-41.6941262901951,-5.75711969621025,
130.012343383614));
#227226=CARTESIAN_POINT('Ctrl Pts',(-41.9725739140079,-3.77821035128576,
135.219883807042));
#227227=CARTESIAN_POINT('Ctrl Pts',(-42.2510215378209,1.67268973063362,
136.369774129642));
#227228=CARTESIAN_POINT('Ctrl Pts',(-42.5294691616338,5.58646966553678,
132.405321320208));
#227229=CARTESIAN_POINT('Ctrl Pts',(-42.8079167854466,4.366556892027,126.969663836325));
#227230=CARTESIAN_POINT('Ctrl Pts',(-43.0863644092596,-0.866008347092154,
125.057905359049));
#227231=CARTESIAN_POINT('Ctrl Pts',(-43.3648120330724,-5.3027542220935,
128.426858534403));
#227232=CARTESIAN_POINT('Ctrl Pts',(-43.6432596568854,-4.86652802093628,
133.98061997675));
#227233=CARTESIAN_POINT('Ctrl Pts',(-43.9217072806982,0.0417996883503892,
136.615554236903));
#227234=CARTESIAN_POINT('Ctrl Pts',(-44.2001549045111,4.9117155260715,133.910285453475));
#227235=CARTESIAN_POINT('Ctrl Pts',(-44.478602528324,5.26800474597596,128.350823478709));
#227236=CARTESIAN_POINT('Ctrl Pts',(-44.7570501521369,0.783254960667603,
125.046042272601));
#227237=CARTESIAN_POINT('Ctrl Pts',(-45.0354977759497,-4.42126786936209,
127.032874316024));
#227238=CARTESIAN_POINT('Ctrl Pts',(-45.3139453997627,-5.56286151839129,
132.485518023215));
#227239=CARTESIAN_POINT('Ctrl Pts',(-45.5923930235756,-1.59245719291215,
136.393260203719));
#227240=CARTESIAN_POINT('Ctrl Pts',(-45.8708406473885,3.84133749699455,
135.165076697471));
#227241=CARTESIAN_POINT('Ctrl Pts',(-46.1492882712014,5.74513068693249,
129.929608146614));
#227242=CARTESIAN_POINT('Ctrl Pts',(-46.4277358950142,2.3694294408167,125.497994382526));
#227243=CARTESIAN_POINT('Ctrl Pts',(-46.7061835188271,-3.18366170834627,
125.942671958037));
#227244=CARTESIAN_POINT('Ctrl Pts',(-46.98463114264,-5.81112327806003,130.85500390496));
#227245=CARTESIAN_POINT('Ctrl Pts',(-47.263078766453,-3.09844644439114,
135.720797144829));
#227246=CARTESIAN_POINT('Ctrl Pts',(-47.5415263902657,2.46155130414924,
136.068625397419));
#227247=CARTESIAN_POINT('Ctrl Pts',(-47.8199740140787,5.75950365764311,
131.578851490957));
#227248=CARTESIAN_POINT('Ctrl Pts',(-48.0984216378915,3.76475351715869,
126.377358307829));
#227249=CARTESIAN_POINT('Ctrl Pts',(-48.3768692617045,-1.6896211871606,
125.244063976264));
#227250=CARTESIAN_POINT('Ctrl Pts',(-48.6553168855173,-5.59131656306301,
129.220410622463));
#227251=CARTESIAN_POINT('Ctrl Pts',(-48.9337645093303,-4.35486516851022,
134.652329933902));
#227252=CARTESIAN_POINT('Ctrl Pts',(-49.2122121331431,0.883494568912716,
136.548153427379));
#227253=CARTESIAN_POINT('Ctrl Pts',(-49.4906597569561,5.3099659586141,133.165711928516));
#227254=CARTESIAN_POINT('Ctrl Pts',(-49.7691073807689,4.85683803860733,
127.613303933314));
#227255=CARTESIAN_POINT('Ctrl Pts',(-50.0475550045819,-0.0594867691506708,
124.993321139153));
#227256=CARTESIAN_POINT('Ctrl Pts',(-50.3260026283946,-4.92114614214944,
127.713399740592));
#227257=CARTESIAN_POINT('Ctrl Pts',(-50.6044502522077,-5.26051262186729,
133.273920386136));
#227258=CARTESIAN_POINT('Ctrl Pts',(-50.8828978760204,-0.765724992417492,
136.565036249065));
#227259=CARTESIAN_POINT('Ctrl Pts',(-51.1613454998334,4.4327264973184,134.562372631296));
#227260=CARTESIAN_POINT('Ctrl Pts',(-51.4397931236463,5.55771888674681,
129.106279562002));
#227261=CARTESIAN_POINT('Ctrl Pts',(-51.7182407474591,1.57543912891688,
125.210640026899));
#227262=CARTESIAN_POINT('Ctrl Pts',(-51.9966883712721,-3.85459222390762,
126.455356446176));
#227263=CARTESIAN_POINT('Ctrl Pts',(-52.2751359950849,-5.7424416302597,
131.696595238295));
#227264=CARTESIAN_POINT('Ctrl Pts',(-52.5535836188979,-2.35326771227282,
136.117914002047));
#227265=CARTESIAN_POINT('Ctrl Pts',(-52.8320312427106,3.19844426977395,
135.656336786975));
#227266=CARTESIAN_POINT('Ctrl Pts',(-53.1104788665238,5.81094222058764,
130.736030504428));
#227267=CARTESIAN_POINT('Ctrl Pts',(-53.3889264903363,3.08346815099054,
125.878516257743));
#227268=CARTESIAN_POINT('Ctrl Pts',(-53.6673741141495,-2.47756251357323,
125.547612336859));
#227269=CARTESIAN_POINT('Ctrl Pts',(-53.9458217379622,-5.76183426382087,
130.047403279515));
#227270=CARTESIAN_POINT('Ctrl Pts',(-54.2242693617753,-3.75126180686946,
135.242801036416));
#227271=CARTESIAN_POINT('Ctrl Pts',(-54.502716985588,1.70653699126786,136.359488878264));
#227272=CARTESIAN_POINT('Ctrl Pts',(-54.7811646094011,5.59611166339667,
132.371285231631));
#227273=CARTESIAN_POINT('Ctrl Pts',(-55.0596122332138,4.3431331021171,126.943154413196));
#227274=CARTESIAN_POINT('Ctrl Pts',(-55.3380598570268,-0.900972606160421,
125.063283466166));
#227275=CARTESIAN_POINT('Ctrl Pts',(-55.6165074808396,-5.31712850433539,
128.459181954061));
#227276=CARTESIAN_POINT('Ctrl Pts',(-55.8949551046525,-4.84710306319425,
134.01018506537));
#227277=CARTESIAN_POINT('Ctrl Pts',(-56.1734027284654,0.0771732988733811,
136.615192122377));
#227278=CARTESIAN_POINT('Ctrl Pts',(-56.4518503522783,4.93053116940174,
133.880328901363));
#227279=CARTESIAN_POINT('Ctrl Pts',(-56.7302979760911,5.25297176508825,
128.318801096944));
#227280=CARTESIAN_POINT('Ctrl Pts',(-57.0087455999042,0.748187930595796,
125.041381065643));
#227281=CARTESIAN_POINT('Ctrl Pts',(-57.2871932237169,-4.44414406110167,
127.059857705357));
#227282=CARTESIAN_POINT('Ctrl Pts',(-57.5656408475299,-5.55252476915405,
132.519349592253));
#227283=CARTESIAN_POINT('Ctrl Pts',(-57.8440884713427,-1.55840647026886,
136.402850393281));
#227284=CARTESIAN_POINT('Ctrl Pts',(-58.1225360951557,3.867811242405,135.141612591857));
#227285=CARTESIAN_POINT('Ctrl Pts',(-58.4009837189685,5.73969937639226,
129.894652112598));
#227286=CARTESIAN_POINT('Ctrl Pts',(-58.6794313427815,2.33708418337799,
125.483669307672));
#227287=CARTESIAN_POINT('Ctrl Pts',(-58.9578789665944,-3.21319720125095,
125.962141886319));
#227288=CARTESIAN_POINT('Ctrl Pts',(-59.2363265904072,-5.81070733134035,
130.890376923444));
#227289=CARTESIAN_POINT('Ctrl Pts',(-59.5147742142201,-3.06846129276222,
135.739567177598));
#227290=CARTESIAN_POINT('Ctrl Pts',(-59.793221838033,2.49355077119662,136.053543701326));
#227291=CARTESIAN_POINT('Ctrl Pts',(-60.071669461846,5.76411149315304,131.543777407928));
#227292=CARTESIAN_POINT('Ctrl Pts',(-60.3501170856587,3.73773534540316,
126.354523206705));
#227293=CARTESIAN_POINT('Ctrl Pts',(-60.6285647094717,-1.72343698624942,
125.254452199421));
#227294=CARTESIAN_POINT('Ctrl Pts',(-60.9070123332846,-5.6008549221161,
129.254475900312));
#227295=CARTESIAN_POINT('Ctrl Pts',(-61.1854599570975,-4.33136080153256,
134.678767940282));
#227296=CARTESIAN_POINT('Ctrl Pts',(-61.4639075809103,0.918442296920838,
136.542668925995));
#227297=CARTESIAN_POINT('Ctrl Pts',(-61.7423552047232,5.32424179290464,
133.133344908207));
#227298=CARTESIAN_POINT('Ctrl Pts',(-62.0208028285362,4.83732318488056,
127.583798104527));
#227299=CARTESIAN_POINT('Ctrl Pts',(-62.299250452349,-0.0948591136734494,
124.993790917104));
#227300=CARTESIAN_POINT('Ctrl Pts',(-62.5776980761619,-4.93987052088691,
127.743413422294));
#227301=CARTESIAN_POINT('Ctrl Pts',(-62.8561456999749,-5.24538224549645,
133.305896864355));
#227302=CARTESIAN_POINT('Ctrl Pts',(-63.1345933237877,-0.730643937663188,
136.569590702456));
#227303=CARTESIAN_POINT('Ctrl Pts',(-63.4130409476006,4.45552045494177,
134.53531973969));
#227304=CARTESIAN_POINT('Ctrl Pts',(-63.6914885714135,5.5472792137301,129.072479611178));
#227305=CARTESIAN_POINT('Ctrl Pts',(-63.9699361952264,1.54135937475606,
125.201153520444));
#227306=CARTESIAN_POINT('Ctrl Pts',(-64.2483838190392,-3.88099443002729,
126.478901020081));
#227307=CARTESIAN_POINT('Ctrl Pts',(-64.5268314428522,-5.73690395073373,
131.731534579357));
#227308=CARTESIAN_POINT('Ctrl Pts',(-64.805279066665,-2.32087900405488,
136.132140562712));
#227309=CARTESIAN_POINT('Ctrl Pts',(-65.083726690478,3.22792036610792,135.636777052998));
#227310=CARTESIAN_POINT('Ctrl Pts',(-65.3621743142908,5.81041861249411,
130.700658915789));
#227311=CARTESIAN_POINT('Ctrl Pts',(-65.6406219381037,3.05342600872776,
125.859837576403));
#227312=CARTESIAN_POINT('Ctrl Pts',(-65.9190695619166,-2.50951592890599,
125.562791358466));
#227313=CARTESIAN_POINT('Ctrl Pts',(-66.1975171857295,-5.76633532454392,
130.082491224748));
#227314=CARTESIAN_POINT('Ctrl Pts',(-66.4759648095424,-3.72417425806736,
135.26555379775));
#227315=CARTESIAN_POINT('Ctrl Pts',(-66.7544124333553,1.74032101554631,
136.348997779564));
#227316=CARTESIAN_POINT('Ctrl Pts',(-67.0328600571681,5.60554629528092,
132.337191080086));
#227317=CARTESIAN_POINT('Ctrl Pts',(-67.3113076809811,4.31954837581292,
126.916788068483));
#227318=CARTESIAN_POINT('Ctrl Pts',(-67.5897553047939,-0.935903479357421,
125.068874311009));
#227319=CARTESIAN_POINT('Ctrl Pts',(-67.8682029286069,-5.33130575842519,
128.491592275178));
#227320=CARTESIAN_POINT('Ctrl Pts',(-68.1466505524197,-4.82749849426569,
134.039631360986));
#227321=CARTESIAN_POINT('Ctrl Pts',(-68.4250981762326,0.112544049711387,
136.614614685353));
#227322=CARTESIAN_POINT('Ctrl Pts',(-68.7035458000455,4.94916411008632,
133.850258368115));
#227323=CARTESIAN_POINT('Ctrl Pts',(-68.9819934238584,5.23774413340002,
128.286870818499));
#227324=CARTESIAN_POINT('Ctrl Pts',(-69.2604410476712,0.713093176145084,
125.036933408012));
#227325=CARTESIAN_POINT('Ctrl Pts',(-69.5388886714842,-4.46685557344872,
127.086979848621));
#227326=CARTESIAN_POINT('Ctrl Pts',(-69.8173362952971,-5.54198226906957,
132.553117611744));
#227327=CARTESIAN_POINT('Ctrl Pts',(-70.09578391911,-1.52429800030071,136.412233128746));
#227328=CARTESIAN_POINT('Ctrl Pts',(-70.3742315429229,3.89414166464747,
135.117987767775));
#227329=CARTESIAN_POINT('Ctrl Pts',(-70.6526791667357,5.73405537918087,
129.859729788164));
#227330=CARTESIAN_POINT('Ctrl Pts',(-70.9311267905487,2.3046523244254,125.469541392991));
#227331=CARTESIAN_POINT('Ctrl Pts',(-71.2095744143614,-3.24261362795168,
125.981791244794));
#227332=CARTESIAN_POINT('Ctrl Pts',(-71.4880220381746,-5.81007606672361,
130.925746754563));
#227333=CARTESIAN_POINT('Ctrl Pts',(-71.7664696619872,-3.03836243817177,
135.758154334473));
#227334=CARTESIAN_POINT('Ctrl Pts',(-72.0449172858002,2.52545783880292,
136.038267494822));
#227335=CARTESIAN_POINT('Ctrl Pts',(-72.3233649096131,5.76850573739207,
131.508675925537));
#227336=CARTESIAN_POINT('Ctrl Pts',(-72.601812533426,3.71057867048956,126.331852995942));
#227337=CARTESIAN_POINT('Ctrl Pts',(-72.8802601572389,-1.75718892274731,
125.265046076474));
#227338=CARTESIAN_POINT('Ctrl Pts',(-73.1587077810518,-5.61018573943046,
129.28859860971));
#227339=CARTESIAN_POINT('Ctrl Pts',(-73.4371554048648,-4.30769593438731,
134.705062379074));
#227340=CARTESIAN_POINT('Ctrl Pts',(-73.7156030286775,0.953355991712339,
136.536971789486));
#227341=CARTESIAN_POINT('Ctrl Pts',(-73.9940506524905,5.33832033545752,
133.100891586529));
#227342=CARTESIAN_POINT('Ctrl Pts',(-74.2724982763033,4.81762908236426,
127.554411614868));
#227343=CARTESIAN_POINT('Ctrl Pts',(-74.5509459001162,-0.130227943157576,
124.994476007852));
#227344=CARTESIAN_POINT('Ctrl Pts',(-74.8293935239292,-4.95841185090586,
127.77354052852));
#227345=CARTESIAN_POINT('Ctrl Pts',(-75.107841147742,-5.23005749955717,
133.337780647228));
#227346=CARTESIAN_POINT('Ctrl Pts',(-75.3862887715549,-0.695535808628632,
136.573931523126));
#227347=CARTESIAN_POINT('Ctrl Pts',(-75.6647363953679,4.4781493116164,134.508128596022));
#227348=CARTESIAN_POINT('Ctrl Pts',(-75.9431840191806,5.53663398424198,
129.038743835842));
#227349=CARTESIAN_POINT('Ctrl Pts',(-76.2216316429937,1.50722250495638,
125.191874642891));
#227350=CARTESIAN_POINT('Ctrl Pts',(-76.5000792668064,-3.90725282447187,
126.502605875483));
#227351=CARTESIAN_POINT('Ctrl Pts',(-76.7785268906195,-5.73115368812196,
131.766439563647));
#227352=CARTESIAN_POINT('Ctrl Pts',(-77.0569745144322,-2.28840429481114,
136.146169700531));
#227353=CARTESIAN_POINT('Ctrl Pts',(-77.3354221382452,3.25727685066645,
135.617038252052));
#227354=CARTESIAN_POINT('Ctrl Pts',(-77.613869762058,5.80967969720196,130.665291169852));
#227355=CARTESIAN_POINT('Ctrl Pts',(-77.8923173858709,3.0232707206408,125.841342116181));
#227356=CARTESIAN_POINT('Ctrl Pts',(-78.1707650096839,-2.54137635320382,
125.57816460835));
#227357=CARTESIAN_POINT('Ctrl Pts',(-78.4492126334967,-5.77062271159095,
130.117605919119));
#227358=CARTESIAN_POINT('Ctrl Pts',(-78.7276602573096,-3.69694870861804,
135.288141247929));
#227359=CARTESIAN_POINT('Ctrl Pts',(-79.0061078811224,1.77404055158998,
136.338301222296));
#227360=CARTESIAN_POINT('Ctrl Pts',(-79.2845555049354,5.61477321158579,
132.303040128944));
#227361=CARTESIAN_POINT('Ctrl Pts',(-79.5630031287483,4.29580358705489,
126.8905657792));
#227362=CARTESIAN_POINT('Ctrl Pts',(-79.8414507525611,-0.970799672307275,
125.074677686406));
#227363=CARTESIAN_POINT('Ctrl Pts',(-80.1198983763742,-5.34528545901998,
128.524088296775));
#227364=CARTESIAN_POINT('Ctrl Pts',(-80.3983460001869,-4.80771504060458,
134.068957772455));
#227365=CARTESIAN_POINT('Ctrl Pts',(-80.6767936239998,0.147910630189091,
136.613821947228));
#227366=CARTESIAN_POINT('Ctrl Pts',(-80.9552412478128,4.96761365767528,
133.820074968005));
#227367=CARTESIAN_POINT('Ctrl Pts',(-81.2336888716256,5.22232241517632,
128.255033826564));
#227368=CARTESIAN_POINT('Ctrl Pts',(-81.5121364954386,0.6779719977639,125.032699464516));
#227369=CARTESIAN_POINT('Ctrl Pts',(-81.7905841192513,-4.48940156482041,
127.114239740797));
#227370=CARTESIAN_POINT('Ctrl Pts',(-82.0690317430644,-5.53123440879372,
132.586820830401));
#227371=CARTESIAN_POINT('Ctrl Pts',(-82.3474793668772,-1.490133046909,136.421408062431));
#227372=CARTESIAN_POINT('Ctrl Pts',(-82.62592699069,3.92032778803891,135.094203100652));
#227373=CARTESIAN_POINT('Ctrl Pts',(-82.9043746145031,5.72819890443852,
129.824842467372));
#227374=CARTESIAN_POINT('Ctrl Pts',(-83.1828222383158,2.27213506573304,
125.455611161998));
#227375=CARTESIAN_POINT('Ctrl Pts',(-83.4612698621288,-3.27190989841242,
126.001619305352));
#227376=CARTESIAN_POINT('Ctrl Pts',(-83.7397174859417,-5.80922950760163,
130.961112087674));
#227377=CARTESIAN_POINT('Ctrl Pts',(-84.0181651097544,-3.00815099594316,
135.776557926701));
#227378=CARTESIAN_POINT('Ctrl Pts',(-84.2966127335676,2.55727132464077,
136.022797343974));
#227379=CARTESIAN_POINT('Ctrl Pts',(-84.5750603573801,5.77268622752965,
131.473548344486));
#227380=CARTESIAN_POINT('Ctrl Pts',(-84.8535079811934,3.68328449871872,
126.309348515594));
#227381=CARTESIAN_POINT('Ctrl Pts',(-85.131955605006,-1.79087574596318,
125.275845214866));
#227382=CARTESIAN_POINT('Ctrl Pts',(-85.4104032288191,-5.61930866924928,
129.322777486226));
#227383=CARTESIAN_POINT('Ctrl Pts',(-85.6888508526319,-4.28387144398495,
134.731212275928));
#227384=CARTESIAN_POINT('Ctrl Pts',(-85.9672984764448,0.98823435954663,
136.531062228962));
#227385=CARTESIAN_POINT('Ctrl Pts',(-86.2457461002577,5.35220106458756,
133.068353166051));
#227386=CARTESIAN_POINT('Ctrl Pts',(-86.5241937240705,4.79775646083024,
127.525145553266));
#227387=CARTESIAN_POINT('Ctrl Pts',(-86.8026413478836,-0.165591946996939,
124.995376386011));
#227388=CARTESIAN_POINT('Ctrl Pts',(-87.0810889716963,-4.97676944515001,
127.803779942897));
#227389=CARTESIAN_POINT('Ctrl Pts',(-87.3595365955093,-5.21453895191432,
133.36957055329));
#227390=CARTESIAN_POINT('Ctrl Pts',(-87.6379842193221,-0.660401906259044,
136.578058550223));
#227391=CARTESIAN_POINT('Ctrl Pts',(-87.916431843135,4.50061222882128,134.480800207869));
#227392=CARTESIAN_POINT('Ctrl Pts',(-88.1948794669479,5.52578359274576,
129.005073486085));
#227393=CARTESIAN_POINT('Ctrl Pts',(-88.4733270907608,1.47302978447255,
125.182803738068));
#227394=CARTESIAN_POINT('Ctrl Pts',(-88.7517747145737,-3.93336643422502,
126.526470133988));
#227395=CARTESIAN_POINT('Ctrl Pts',(-89.0302223383866,-5.7251910555031,
131.801308897747));
#227396=CARTESIAN_POINT('Ctrl Pts',(-89.3086699621995,-2.25584478790559,
136.16000089565));
#227397=CARTESIAN_POINT('Ctrl Pts',(-89.5871175860123,3.28651263563227,
135.597121115567));
#227398=CARTESIAN_POINT('Ctrl Pts',(-89.8655652098253,5.80872550209253,
130.629928577187));
#227399=CARTESIAN_POINT('Ctrl Pts',(-90.1440128336381,2.99300340414587,
125.823030562435));
#227400=CARTESIAN_POINT('Ctrl Pts',(-90.4224604574511,-2.57314260586573,
125.593731516848));
#227401=CARTESIAN_POINT('Ctrl Pts',(-90.7009080812639,-5.77469626609129,
130.152746061436));
#227402=CARTESIAN_POINT('Ctrl Pts',(-90.9793557050769,-3.66958616737523,
135.310562549967));
#227403=CARTESIAN_POINT('Ctrl Pts',(-91.2578033288896,1.80769434990835,
136.327399602824));
#227404=CARTESIAN_POINT('Ctrl Pts',(-91.5362509527026,5.62379207040447,
132.268833643682));
#227405=CARTESIAN_POINT('Ctrl Pts',(-91.8146985765155,4.27189961571542,
126.864488517025));
#227406=CARTESIAN_POINT('Ctrl Pts',(-92.0931462003284,-1.00565989191805,
125.080693377311));
#227407=CARTESIAN_POINT('Ctrl Pts',(-92.3715938241412,-5.3590670880956,
128.556668814702));
#227408=CARTESIAN_POINT('Ctrl Pts',(-92.6500414479542,-4.78775343529548,
134.098163213075));
#227409=CARTESIAN_POINT('Ctrl Pts',(-92.928489071767,0.183271729783054,
136.612813937377));
#227410=CARTESIAN_POINT('Ctrl Pts',(-93.2069366955801,4.98587912851244,
133.789779819492));
#227411=CARTESIAN_POINT('Ctrl Pts',(-93.4853843193926,5.2067071818758,128.223291300872));
#227412=CARTESIAN_POINT('Ctrl Pts',(-93.7638319432059,0.642825696881324,
125.028679392048));
#227413=CARTESIAN_POINT('Ctrl Pts',(-94.0422795670186,-4.51178119976554,
127.14163637176));
#227414=CARTESIAN_POINT('Ctrl Pts',(-94.3207271908314,-5.52028158659305,
132.62045799934));
#227415=CARTESIAN_POINT('Ctrl Pts',(-94.5991748146444,-1.45591287608963,
136.430374854359));
#227416=CARTESIAN_POINT('Ctrl Pts',(-94.8776224384574,3.94636864224209,
135.07025947184));
#227417=CARTESIAN_POINT('Ctrl Pts',(-95.1560700622702,5.7221301691794,129.789991442987));
#227418=CARTESIAN_POINT('Ctrl Pts',(-95.4345176860831,2.23953361224044,
125.441879130882));
#227419=CARTESIAN_POINT('Ctrl Pts',(-95.7129653098959,-3.30108492704829,
126.021625333256));
#227420=CARTESIAN_POINT('Ctrl Pts',(-95.9914129337089,-5.80816768534362,
130.996471612301));
#227421=CARTESIAN_POINT('Ctrl Pts',(-96.2698605575217,-2.97782808557417,
135.794777272329));
#227422=CARTESIAN_POINT('Ctrl Pts',(-96.5483081813347,2.58899004984866,
136.007133822036));
#227423=CARTESIAN_POINT('Ctrl Pts',(-96.8267558051475,5.77665280865574,
131.438395966436));
#227424=CARTESIAN_POINT('Ctrl Pts',(-97.1052034289604,3.65585384148698,
126.287010599573));
#227425=CARTESIAN_POINT('Ctrl Pts',(-97.3836510527732,-1.82449620761995,
125.286849214428));
#227426=CARTESIAN_POINT('Ctrl Pts',(-97.6620986765863,-5.62822337351841,
129.35701126335));
#227427=CARTESIAN_POINT('Ctrl Pts',(-97.9405463003989,-4.25988821315111,
134.757216661848));
#227428=CARTESIAN_POINT('Ctrl Pts',(-98.2189939242121,1.02307610799351,
136.524940463405));
#227429=CARTESIAN_POINT('Ctrl Pts',(-98.4974415480248,5.36588346593846,
133.035730852497));
#227430=CARTESIAN_POINT('Ctrl Pts',(-98.7758891718378,4.77770605666655,
127.496001004183));
#227431=CARTESIAN_POINT('Ctrl Pts',(-99.0543367956506,-0.200949814765295,
124.996492018215));
#227432=CARTESIAN_POINT('Ctrl Pts',(-99.3327844194636,-4.99494262337204,
127.834130544897));
#227433=CARTESIAN_POINT('Ctrl Pts',(-99.6112320432764,-5.19882717761281,
133.401265404553));
#227434=CARTESIAN_POINT('Ctrl Pts',(-99.8896796670892,-0.625243532454567,
136.581971630822));
#227435=CARTESIAN_POINT('Ctrl Pts',(-100.168127290903,4.5229083741848,134.453335587896));
#227436=CARTESIAN_POINT('Ctrl Pts',(-100.446574914715,5.51472844130613,
128.971469809575));
#227437=CARTESIAN_POINT('Ctrl Pts',(-100.725022538528,1.43878248032906,
125.173941142103));
#227438=CARTESIAN_POINT('Ctrl Pts',(-101.003470162341,-3.95933429163924,
126.550492911299));
#227439=CARTESIAN_POINT('Ctrl Pts',(-101.281917786154,-5.71901627382367,
131.836141289563));
#227440=CARTESIAN_POINT('Ctrl Pts',(-101.560365409967,-2.22320168984167,
136.17363363555));
#227441=CARTESIAN_POINT('Ctrl Pts',(-101.83881303378,3.31562663766449,135.577026381578));
#227442=CARTESIAN_POINT('Ctrl Pts',(-102.117260657593,5.80755606252295,
130.594572448163));
#227443=CARTESIAN_POINT('Ctrl Pts',(-102.395708281405,2.96262518080941,
125.804903593708));
#227444=CARTESIAN_POINT('Ctrl Pts',(-102.674155905219,-2.60481350978186,
125.609491507123));
#227445=CARTESIAN_POINT('Ctrl Pts',(-102.952603529031,-5.77855583709781,
130.187910349571));
#227446=CARTESIAN_POINT('Ctrl Pts',(-103.231051152844,-3.64208764826766,
135.332816873036));
#227447=CARTESIAN_POINT('Ctrl Pts',(-103.509498776657,1.84128116344741,
136.316293325111));
#227448=CARTESIAN_POINT('Ctrl Pts',(-103.78794640047,5.63260253753978,132.234572891835));
#227449=CARTESIAN_POINT('Ctrl Pts',(-104.066394024283,4.24783734756473,
126.838557248259));
#227450=CARTESIAN_POINT('Ctrl Pts',(-104.344841648096,-1.04048284643121,
125.086921160811));
#227451=CARTESIAN_POINT('Ctrl Pts',(-104.623289271909,-5.3726501349701,
128.589332621676));
#227452=CARTESIAN_POINT('Ctrl Pts',(-104.901736895722,-4.76761441802147,
134.12724660063));
#227453=CARTESIAN_POINT('Ctrl Pts',(-105.180184519534,0.218626038175886,
136.611590693152));
#227454=CARTESIAN_POINT('Ctrl Pts',(-105.458632143348,5.00395984576562,
133.759374045173));
#227455=CARTESIAN_POINT('Ctrl Pts',(-105.73707976716,5.1908990121252,128.191644417652));
#227456=CARTESIAN_POINT('Ctrl Pts',(-106.015527390973,0.607655575856702,
125.024873339572));
#227457=CARTESIAN_POINT('Ctrl Pts',(-106.293975014786,-4.53399364899913,
127.169168726316));
#227458=CARTESIAN_POINT('Ctrl Pts',(-106.572422638599,-5.50912420832816,
132.654027872123));
#227459=CARTESIAN_POINT('Ctrl Pts',(-106.850870262412,-1.42163875588365,
136.43913317226));
#227460=CARTESIAN_POINT('Ctrl Pts',(-107.129317886225,3.97226326230387,
135.046157768576));
#227461=CARTESIAN_POINT('Ctrl Pts',(-107.407765510038,5.71584939828273,
129.755178006424));
#227462=CARTESIAN_POINT('Ctrl Pts',(-107.686213133851,2.20684917200607,
125.428345808491));
#227463=CARTESIAN_POINT('Ctrl Pts',(-107.964660757664,-3.3301376327682,
126.041808587174));
#227464=CARTESIAN_POINT('Ctrl Pts',(-108.243108381476,-5.80689063929651,
131.031824018185));
#227465=CARTESIAN_POINT('Ctrl Pts',(-108.521556005289,-2.94739483068967,
135.812811696231));
#227466=CARTESIAN_POINT('Ctrl Pts',(-108.800003629102,2.62061283907833,
135.991277509423));
#227467=CARTESIAN_POINT('Ctrl Pts',(-109.078451252915,5.7804053337882,131.403220093974));
#227468=CARTESIAN_POINT('Ctrl Pts',(-109.356898876728,3.62828771524594,
126.264840075618));
#227469=CARTESIAN_POINT('Ctrl Pts',(-109.635346500541,-1.85804906189805,
125.298057667405));
#227470=CARTESIAN_POINT('Ctrl Pts',(-109.913794124354,-5.636929521901,129.391298672536));
#227471=CARTESIAN_POINT('Ctrl Pts',(-110.192241748167,-4.2357471305931,
134.783074573235));
#227472=CARTESIAN_POINT('Ctrl Pts',(-110.470689371979,1.05787994597834,
136.518606719657));
#227473=CARTESIAN_POINT('Ctrl Pts',(-110.749136995792,5.37936703250445,
133.003025854698));
#227474=CARTESIAN_POINT('Ctrl Pts',(-111.027584619605,4.75747861284798,
127.466979047582));
#227475=CARTESIAN_POINT('Ctrl Pts',(-111.306032243418,-0.23630023626489,
124.997822863128));
#227476=CARTESIAN_POINT('Ctrl Pts',(-111.584479867231,-5.01293071215839,
127.864591209862));
#227477=CARTESIAN_POINT('Ctrl Pts',(-111.862927491044,-5.18292275885852,
133.432864026556));
#227478=CARTESIAN_POINT('Ctrl Pts',(-112.141375114857,-0.590061990020461,
136.585670619917));
#227479=CARTESIAN_POINT('Ctrl Pts',(-112.41982273867,4.54503692151536,134.425735753813));
#227480=CARTESIAN_POINT('Ctrl Pts',(-112.698270362483,5.50346893957634,
128.937934051507));
#227481=CARTESIAN_POINT('Ctrl Pts',(-112.976717986295,1.40448186157095,
125.165287183403));
#227482=CARTESIAN_POINT('Ctrl Pts',(-113.255165610108,-3.98515543446448,
126.574673317241));
#227483=CARTESIAN_POINT('Ctrl Pts',(-113.533613233921,-5.71262957189362,
131.870935448366));
#227484=CARTESIAN_POINT('Ctrl Pts',(-113.812060857734,-2.19047621022174,
136.187067415062));
#227485=CARTESIAN_POINT('Ctrl Pts',(-114.090508481547,3.34461777793161,
135.556754794705));
#227486=CARTESIAN_POINT('Ctrl Pts',(-114.36895610536,5.80617142182825,130.559224092919));
#227487=CARTESIAN_POINT('Ctrl Pts',(-114.647403729173,2.9321371763071,125.786961881698));
#227488=CARTESIAN_POINT('Ctrl Pts',(-114.925851352986,-2.63638789137572,
125.625443995184));
#227489=CARTESIAN_POINT('Ctrl Pts',(-115.204298976799,-5.78220128159277,
130.223097480497));
#227490=CARTESIAN_POINT('Ctrl Pts',(-115.482746600612,-3.61445417026275,
135.354903392492));
#227491=CARTESIAN_POINT('Ctrl Pts',(-115.761194224424,1.87479974763623,
136.304982800703));
#227492=CARTESIAN_POINT('Ctrl Pts',(-116.039641848237,5.64120428651674,
132.200259142944));
#227493=CARTESIAN_POINT('Ctrl Pts',(-116.31808947205,4.22361767423897,126.812772933795));
#227494=CARTESIAN_POINT('Ctrl Pts',(-116.596537095863,-1.07526724547036,
125.093360806132));
#227495=CARTESIAN_POINT('Ctrl Pts',(-116.874984719676,-5.38603409631742,
128.622078507325));
#227496=CARTESIAN_POINT('Ctrl Pts',(-117.153432343489,-4.7472987350426,
134.156206857421));
#227497=CARTESIAN_POINT('Ctrl Pts',(-117.431879967302,0.253972245300257,
136.610152259881));
#227498=CARTESIAN_POINT('Ctrl Pts',(-117.710327591115,5.02185513944583,
133.728858771743));
#227499=CARTESIAN_POINT('Ctrl Pts',(-117.988775214928,5.17489849170343,
128.160094349593));
#227500=CARTESIAN_POINT('Ctrl Pts',(-118.26722283874,0.572462937930709,
125.021281448121));
#227501=CARTESIAN_POINT('Ctrl Pts',(-118.545670462553,-4.55603808943068,
127.196835784245));
#227502=CARTESIAN_POINT('Ctrl Pts',(-118.824118086366,-5.49776268743969,
132.687529204804));
#227503=CARTESIAN_POINT('Ctrl Pts',(-119.102565710179,-1.38731195633035,
136.447682691592));
#227504=CARTESIAN_POINT('Ctrl Pts',(-119.381013333992,3.99801068868978,
135.021898883958));
#227505=CARTESIAN_POINT('Ctrl Pts',(-119.659460957805,5.70935682448427,
129.720403447709));
#227506=CARTESIAN_POINT('Ctrl Pts',(-119.937908581618,2.17408295616475,
125.415011696306));
#227507=CARTESIAN_POINT('Ctrl Pts',(-120.216356205431,-3.3590669390133,
126.062168319208));
#227508=CARTESIAN_POINT('Ctrl Pts',(-120.494803829244,-5.80539841678086,
131.067167995328));
#227509=CARTESIAN_POINT('Ctrl Pts',(-120.773251453056,-2.91685235900652,
135.830660530138));
#227510=CARTESIAN_POINT('Ctrl Pts',(-121.051699076869,2.65213852053535,
135.975228993696));
#227511=CARTESIAN_POINT('Ctrl Pts',(-121.330146700682,5.78394366387473,
131.368022030553));
#227512=CARTESIAN_POINT('Ctrl Pts',(-121.608594324495,3.60058714147007,
126.242837765265));
#227513=CARTESIAN_POINT('Ctrl Pts',(-121.887041948308,-1.89153306548558,
125.309470158462));
#227514=CARTESIAN_POINT('Ctrl Pts',(-122.165489572121,-5.64542679178685,
129.425638443252));
#227515=CARTESIAN_POINT('Ctrl Pts',(-122.443937195934,-4.21144909086733,
134.808785051914));
#227516=CARTESIAN_POINT('Ctrl Pts',(-122.722384819747,1.09264458383337,
136.512061232418));
#227517=CARTESIAN_POINT('Ctrl Pts',(-123.00083244356,5.39265126464657,132.97023938455));
#227518=CARTESIAN_POINT('Ctrl Pts',(-123.279280067372,4.73707487890982,
127.438080758883));
#227519=CARTESIAN_POINT('Ctrl Pts',(-123.557727691185,-0.27164190157181,
124.999368871432));
#227520=CARTESIAN_POINT('Ctrl Pts',(-123.836175314998,-5.03073304495359,
127.895160809065));
#227521=CARTESIAN_POINT('Ctrl Pts',(-124.114622938811,-5.16682628499523,
133.464365248398));
#227522=CARTESIAN_POINT('Ctrl Pts',(-124.393070562624,-0.554858582622917,
136.589155380447));
#227523=CARTESIAN_POINT('Ctrl Pts',(-124.671518186437,4.56699705083122,
134.398001728342));
#227524=CARTESIAN_POINT('Ctrl Pts',(-124.94996581025,5.49200550478084,128.904467454562));
#227525=CARTESIAN_POINT('Ctrl Pts',(-125.228413434063,1.37012919922165,
125.156842182641));
#227526=CARTESIAN_POINT('Ctrl Pts',(-125.506861057876,-4.0108289058903,
126.599010455801));
#227527=CARTESIAN_POINT('Ctrl Pts',(-125.785308681688,-5.70603118637341,
131.905690084846));
#227528=CARTESIAN_POINT('Ctrl Pts',(-126.063756305501,-2.1576695617001,
136.200301736396));
#227529=CARTESIAN_POINT('Ctrl Pts',(-126.342203929314,3.37348498215772,
135.536307106118));
#227530=CARTESIAN_POINT('Ctrl Pts',(-126.620651553127,5.8045716313158,130.523884821299));
#227531=CARTESIAN_POINT('Ctrl Pts',(-126.89909917694,2.90154052038371,125.769206091244));
#227532=CARTESIAN_POINT('Ctrl Pts',(-127.177546800753,-2.66786458064647,
125.641588389905));
#227533=CARTESIAN_POINT('Ctrl Pts',(-127.455994424566,-5.7856324644928,
130.258306150342));
#227534=CARTESIAN_POINT('Ctrl Pts',(-127.734442048379,-3.5866867573295,
135.376821289913));
#227535=CARTESIAN_POINT('Ctrl Pts',(-128.012889672192,1.90824886043053,
136.293468448719));
#227536=CARTESIAN_POINT('Ctrl Pts',(-128.291337296005,5.64959699859458,
132.16589366852));
#227537=CARTESIAN_POINT('Ctrl Pts',(-128.569784919818,4.19924149320669,
126.787136529081));
#227538=CARTESIAN_POINT('Ctrl Pts',(-128.84823254363,-1.11001180008614,
125.100012074652));
#227539=CARTESIAN_POINT('Ctrl Pts',(-129.126680167443,-5.39921847619124,
128.654905258242));
#227540=CARTESIAN_POINT('Ctrl Pts',(-129.405127791256,-4.72680713916258,
134.185042910317));
#227541=CARTESIAN_POINT('Ctrl Pts',(-129.683575415069,0.289309041389885,
136.608498690867));
#227542=CARTESIAN_POINT('Ctrl Pts',(-129.962023038882,5.03956434643776,
133.69823512996));
#227543=CARTESIAN_POINT('Ctrl Pts',(-130.240470662695,5.15870621351431,
128.128642265792));
#227544=CARTESIAN_POINT('Ctrl Pts',(-130.518918286508,0.537249087180579,
125.017903850796));
#227545=CARTESIAN_POINT('Ctrl Pts',(-130.79736591032,-4.57791370419536,
127.224636520332));
#227546=CARTESIAN_POINT('Ctrl Pts',(-131.075813534134,-5.4861974449331,
132.720960755981));
#227547=CARTESIAN_POINT('Ctrl Pts',(-131.354261157946,-1.35293374942274,
136.456023095549));
#227548=CARTESIAN_POINT('Ctrl Pts',(-131.632708781759,4.02360996731925,
134.99748371691));
#227549=CARTESIAN_POINT('Ctrl Pts',(-131.911156405572,5.7026526883694,129.685669055425));
#227550=CARTESIAN_POINT('Ctrl Pts',(-132.189604029385,2.1412361788793,125.401877288427));
#227551=CARTESIAN_POINT('Ctrl Pts',(-132.468051653198,-3.38787177379785,
126.082703774923));
#227552=CARTESIAN_POINT('Ctrl Pts',(-132.746499277011,-5.80369107309236,
131.102502234048));
#227553=CARTESIAN_POINT('Ctrl Pts',(-133.024946900823,-2.88620180228584,
135.848323112653));
#227554=CARTESIAN_POINT('Ctrl Pts',(-133.303394524637,2.68356592602436,
135.95898886954));
#227555=CARTESIAN_POINT('Ctrl Pts',(-133.581842148449,5.78726766780228,
131.332803080451));
#227556=CARTESIAN_POINT('Ctrl Pts',(-133.860289772262,3.57275314661281,
126.221004483821));
#227557=CARTESIAN_POINT('Ctrl Pts',(-134.138737396075,-1.92494697761906,
125.321086264707));
#227558=CARTESIAN_POINT('Ctrl Pts',(-134.417185019888,-5.65371486830715,
129.460029303025));
#227559=CARTESIAN_POINT('Ctrl Pts',(-134.695632643701,-4.1869949943469,
134.834347145171));
#227560=CARTESIAN_POINT('Ctrl Pts',(-134.974080267514,1.1273687333409,136.505304244234));
#227561=CARTESIAN_POINT('Ctrl Pts',(-135.252527891327,5.40573567011315,
132.937372656969));
#227562=CARTESIAN_POINT('Ctrl Pts',(-135.53097551514,4.71649561092,127.409307208922));
#227563=CARTESIAN_POINT('Ctrl Pts',(-135.809423138953,-0.306973501088704,
125.001129985841));
#227564=CARTESIAN_POINT('Ctrl Pts',(-136.087870762765,-5.04834896208586,
127.925838209736));
#227565=CARTESIAN_POINT('Ctrl Pts',(-136.366318386578,-5.15053835248403,
133.49576790279));
#227566=CARTESIAN_POINT('Ctrl Pts',(-136.644766010391,-0.519634614735935,
136.592425783278));
#227567=CARTESIAN_POINT('Ctrl Pts',(-136.923213634204,4.58878794839197,
134.37013453918));
#227568=CARTESIAN_POINT('Ctrl Pts',(-137.201661258017,5.48033856170195,
128.871071258858));
#227569=CARTESIAN_POINT('Ctrl Pts',(-137.48010888183,1.33572576623031,125.148606452753));
#227570=CARTESIAN_POINT('Ctrl Pts',(-137.758556505643,-4.03635375457527,
126.623503425159));
#227571=CARTESIAN_POINT('Ctrl Pts',(-138.037004129456,-5.69922136176977,
131.940403911158));
#227572=CARTESIAN_POINT('Ctrl Pts',(-138.315451753269,-2.12478295993955,
136.213336109146));
#227573=CARTESIAN_POINT('Ctrl Pts',(-138.593899377082,3.40222718065648,
135.515684073514));
#227574=CARTESIAN_POINT('Ctrl Pts',(-138.872347000894,5.80275675026745,
130.488555942812));
#227575=CARTESIAN_POINT('Ctrl Pts',(-139.150794624707,2.870836346809,125.751636880291));
#227576=CARTESIAN_POINT('Ctrl Pts',(-139.42924224852,-2.69924241121433,
125.65792409305));
#227577=CARTESIAN_POINT('Ctrl Pts',(-139.707689872333,-5.78884925865424,
130.293535054436));
#227578=CARTESIAN_POINT('Ctrl Pts',(-139.986137496146,-3.55878643839929,
135.398569753122));
#227579=CARTESIAN_POINT('Ctrl Pts',(-140.264585119959,1.94162726236197,
136.281750695826));
#227580=CARTESIAN_POINT('Ctrl Pts',(-140.543032743772,5.65778036277742,
132.131477741989));
#227581=CARTESIAN_POINT('Ctrl Pts',(-140.821480367585,4.17470970773734,
126.761648984083));
#227582=CARTESIAN_POINT('Ctrl Pts',(-141.099927991397,-1.14471522280625,
125.106874719905));
#227583=CARTESIAN_POINT('Ctrl Pts',(-141.37837561521,-5.41220278603824,
128.687811658017));
#227584=CARTESIAN_POINT('Ctrl Pts',(-141.656823239023,-4.70614038970644,
134.213753690789));
#227585=CARTESIAN_POINT('Ctrl Pts',(-141.935270862836,0.324635117026387,
136.60663004738));
#227586=CARTESIAN_POINT('Ctrl Pts',(-142.213718486649,5.05708681051884,
133.667504254592));
#227587=CARTESIAN_POINT('Ctrl Pts',(-142.492166110462,5.14232277757003,
128.097289331719));
#227588=CARTESIAN_POINT('Ctrl Pts',(-142.770613734275,0.502015328467386,
125.014740672754));
#227589=CARTESIAN_POINT('Ctrl Pts',(-143.049061358088,-4.59961968268416,
127.252569904414));
#227590=CARTESIAN_POINT('Ctrl Pts',(-143.327508981901,-5.4744289093626,
132.754321286837));
#227591=CARTESIAN_POINT('Ctrl Pts',(-143.605956605714,-1.31850540905707,
136.464154075075));
#227592=CARTESIAN_POINT('Ctrl Pts',(-143.884404229526,4.04906014960179,
134.972913172143));
#227593=CARTESIAN_POINT('Ctrl Pts',(-144.162851853339,5.69573723836169,
129.650976116669));
#227594=CARTESIAN_POINT('Ctrl Pts',(-144.441299477152,2.10831005730047,
125.388943071553));
#227595=CARTESIAN_POINT('Ctrl Pts',(-144.719747100965,-3.41655106974776,
126.103414193369));
#227596=CARTESIAN_POINT('Ctrl Pts',(-144.998194724778,-5.80176867149642,
131.13782542502));
#227597=CARTESIAN_POINT('Ctrl Pts',(-145.276642348591,-2.85544429629671,
135.865798789283));
#227598=CARTESIAN_POINT('Ctrl Pts',(-145.555089972404,2.71489389099137,
135.942557738738));
#227599=CARTESIAN_POINT('Ctrl Pts',(-145.833537596217,5.79037722239768,
131.29756454872));
#227600=CARTESIAN_POINT('Ctrl Pts',(-146.111985220029,3.54478676207412,
126.199341040322));
#227601=CARTESIAN_POINT('Ctrl Pts',(-146.390432843843,-1.95828956013508,
125.332905555698));
#227602=CARTESIAN_POINT('Ctrl Pts',(-146.668880467655,-5.66179344434354,
129.49446997749));
#227603=CARTESIAN_POINT('Ctrl Pts',(-146.947328091469,-4.16238574718705,
134.859759905796));
#227604=CARTESIAN_POINT('Ctrl Pts',(-147.225775715281,1.16205110778606,
136.498336005488));
#227605=CARTESIAN_POINT('Ctrl Pts',(-147.504223339094,5.41861976405632,
132.904426889841));
#227606=CARTESIAN_POINT('Ctrl Pts',(-147.782670962907,4.6957415714508,127.380659463914));
#227607=CARTESIAN_POINT('Ctrl Pts',(-148.06111858672,-0.342293725589094,
125.003106141093));
#227608=CARTESIAN_POINT('Ctrl Pts',(-148.339566210533,-5.06577781079073,
127.956622275114));
#227609=CARTESIAN_POINT('Ctrl Pts',(-148.618013834346,-5.1340595648799,
133.527070826096));
#227610=CARTESIAN_POINT('Ctrl Pts',(-148.896461458158,-0.48439139159784,
136.595481707227));
#227611=CARTESIAN_POINT('Ctrl Pts',(-149.174909081971,4.61040880672808,
134.342135218952));
#227612=CARTESIAN_POINT('Ctrl Pts',(-149.453356705784,5.4684685426618,128.837746701901));
#227613=CARTESIAN_POINT('Ctrl Pts',(-149.731804329597,1.30127283742975,
125.140580298914));
#227614=CARTESIAN_POINT('Ctrl Pts',(-150.01025195341,-4.06172903468827,
126.648151317718));
#227615=CARTESIAN_POINT('Ctrl Pts',(-150.288699577223,-5.69220035042211,
131.975075640969));
#227616=CARTESIAN_POINT('Ctrl Pts',(-150.567147201036,-2.09181762356486,
136.226170050321));
#227617=CARTESIAN_POINT('Ctrl Pts',(-150.845594824849,3.43084330837664,
135.494886461086));
#227618=CARTESIAN_POINT('Ctrl Pts',(-151.124042448661,5.80072684593324,
130.453238766583));
#227619=CARTESIAN_POINT('Ctrl Pts',(-151.402490072475,2.84002579333802,
125.734254899877));
#227620=CARTESIAN_POINT('Ctrl Pts',(-151.680937696287,-2.73052022036177,
125.674450499292));
#227621=CARTESIAN_POINT('Ctrl Pts',(-151.9593853201,-5.79185154487752,130.32878288736));
#227622=CARTESIAN_POINT('Ctrl Pts',(-152.237832943913,-3.53075424732904,
135.420147976222));
#227623=CARTESIAN_POINT('Ctrl Pts',(-152.516280567726,1.97493371658077,
136.269829976228));
#227624=CARTESIAN_POINT('Ctrl Pts',(-152.794728191539,5.66575407582884,
132.097012638644));
#227625=CARTESIAN_POINT('Ctrl Pts',(-153.073175815352,4.15002322686382,
126.736311243251));
#227626=CARTESIAN_POINT('Ctrl Pts',(-153.351623439165,-1.17937622768304,
125.113948487592));
#227627=CARTESIAN_POINT('Ctrl Pts',(-153.630071062978,-5.42498654472129,
128.720796487292));
#227628=CARTESIAN_POINT('Ctrl Pts',(-153.90851868679,-4.6852992524868,134.242338134946));
#227629=CARTESIAN_POINT('Ctrl Pts',(-154.186966310604,0.359949163189457,
136.604546398667));
#227630=CARTESIAN_POINT('Ctrl Pts',(-154.465413934416,5.0744218823891,133.636667284384));
#227631=CARTESIAN_POINT('Ctrl Pts',(-154.743861558229,5.12574879096345,
128.066036709167));
#227632=CARTESIAN_POINT('Ctrl Pts',(-155.022309182042,0.466762967392146,
125.011792031209));
#227633=CARTESIAN_POINT('Ctrl Pts',(-155.300756805855,-4.62115522057418,
127.280634901405));
#227634=CARTESIAN_POINT('Ctrl Pts',(-155.579204429668,-5.46245751681569,
132.787609561181));
#227635=CARTESIAN_POINT('Ctrl Pts',(-155.857652053481,-1.28402821098903,
136.472075328871));
#227636=CARTESIAN_POINT('Ctrl Pts',(-156.136099677293,4.07436029247137,
134.948188160129));
#227637=CARTESIAN_POINT('Ctrl Pts',(-156.414547301107,5.68861073071636,
129.616325916999));
#227638=CARTESIAN_POINT('Ctrl Pts',(-156.692994924919,2.07530581151645,
125.376209524969));
#227639=CARTESIAN_POINT('Ctrl Pts',(-156.971442548732,-3.44510376414151,
126.124298807112));
#227640=CARTESIAN_POINT('Ctrl Pts',(-157.249890172545,-5.79963128322921,
131.173136259331));
#227641=CARTESIAN_POINT('Ctrl Pts',(-157.528337796358,-2.82458098076833,
135.883086912459));
#227642=CARTESIAN_POINT('Ctrl Pts',(-157.806785420171,2.74612125456611,
135.925936210153));
#227643=CARTESIAN_POINT('Ctrl Pts',(-158.085233043984,5.79327221243612,
131.262307741136));
#227644=CARTESIAN_POINT('Ctrl Pts',(-158.363680667797,3.51668902415852,
126.177848237519));
#227645=CARTESIAN_POINT('Ctrl Pts',(-158.64212829161,-1.9915595775106,125.344927593469));
#227646=CARTESIAN_POINT('Ctrl Pts',(-158.920575915422,-5.66966222054205,
129.528959190434));
#227647=CARTESIAN_POINT('Ctrl Pts',(-159.199023539236,-4.13762226129274,
134.885022392109));
#227648=CARTESIAN_POINT('Ctrl Pts',(-159.477471163048,1.19669042199943,
136.491156774389));
#227649=CARTESIAN_POINT('Ctrl Pts',(-159.755918786861,5.43130306905165,
132.871403303985));
#227650=CARTESIAN_POINT('Ctrl Pts',(-160.034366410674,4.67481352955083,
127.352138585409));
#227651=CARTESIAN_POINT('Ctrl Pts',(-160.312814034487,-0.377601266270116,
125.005297263965));
#227652=CARTESIAN_POINT('Ctrl Pts',(-160.5912616583,-5.08301894523598,127.987511864483));
#227653=CARTESIAN_POINT('Ctrl Pts',(-160.869709282113,-5.1173905328107,
133.558272858373));
#227654=CARTESIAN_POINT('Ctrl Pts',(-161.148156905926,-0.449130219157962,
136.598323039052));
#227655=CARTESIAN_POINT('Ctrl Pts',(-161.426604529739,4.63185882466967,
134.314004805186));
#227656=CARTESIAN_POINT('Ctrl Pts',(-161.705052153551,5.45639588750942,
128.804495018547));
#227657=CARTESIAN_POINT('Ctrl Pts',(-161.983499777364,1.26677168948586,
125.13276401854));
#227658=CARTESIAN_POINT('Ctrl Pts',(-162.261947401177,-4.08695380593746,
126.67295322014));
#227659=CARTESIAN_POINT('Ctrl Pts',(-162.54039502499,-5.68496841249774,
132.009703989503));
#227660=CARTESIAN_POINT('Ctrl Pts',(-162.818842648803,-2.05877477411906,
136.238803084352));
#227661=CARTESIAN_POINT('Ctrl Pts',(-163.097290272616,3.45933230493559,
135.473915039499));
#227662=CARTESIAN_POINT('Ctrl Pts',(-163.375737896429,5.79848199353304,
130.417934601304));
#227663=CARTESIAN_POINT('Ctrl Pts',(-163.654185520242,2.80911000166655,
125.717060794092));
#227664=CARTESIAN_POINT('Ctrl Pts',(-163.932633144055,-2.76169684907854,
125.691166996241));
#227665=CARTESIAN_POINT('Ctrl Pts',(-164.211080767867,-5.79463921191188,
130.36404834299));
#227666=CARTESIAN_POINT('Ctrl Pts',(-164.489528391681,-3.50259122286156,
135.441555159625));
#227667=CARTESIAN_POINT('Ctrl Pts',(-164.767976015493,2.00816698890481,
136.257706731653));
#227668=CARTESIAN_POINT('Ctrl Pts',(-165.046423639306,5.67351784227885,
132.062499635604));
#227669=CARTESIAN_POINT('Ctrl Pts',(-165.324871263119,4.12518296535417,
126.711124245485));
#227670=CARTESIAN_POINT('Ctrl Pts',(-165.603318886932,-1.21399353033979,
125.121233115594));
#227671=CARTESIAN_POINT('Ctrl Pts',(-165.881766510745,-5.43756927853226,
128.753858523801));
#227672=CARTESIAN_POINT('Ctrl Pts',(-166.160214134558,-4.66428449978105,
134.270795183582));
#227673=CARTESIAN_POINT('Ctrl Pts',(-166.438661758371,0.395249871304121,
136.602247821935));
#227674=CARTESIAN_POINT('Ctrl Pts',(-166.717109382183,5.09156891968999,
133.60572536201));
#227675=CARTESIAN_POINT('Ctrl Pts',(-166.995557005996,5.10898486785074,
128.034885556215));
#227676=CARTESIAN_POINT('Ctrl Pts',(-167.274004629809,0.431493310242956,
125.009058035423));
#227677=CARTESIAN_POINT('Ctrl Pts',(-167.552452253622,-4.64251951985801,
127.30883047135));
#227678=CARTESIAN_POINT('Ctrl Pts',(-167.830899877435,-5.45028371089662,
132.820824345507));
#227679=CARTESIAN_POINT('Ctrl Pts',(-168.109347501248,-1.24950343278299,
136.479786563416));
#227680=CARTESIAN_POINT('Ctrl Pts',(-168.387795125061,4.09950945842204,
134.923309597059));
#227681=CARTESIAN_POINT('Ctrl Pts',(-168.666242748874,5.68127342950807,
129.581719740392));
#227682=CARTESIAN_POINT('Ctrl Pts',(-168.944690372687,2.04222466451309,
125.36367712052));
#227683=CARTESIAN_POINT('Ctrl Pts',(-169.223137996499,-3.47352879894819,
126.145356842267));
#227684=CARTESIAN_POINT('Ctrl Pts',(-169.501585620313,-5.79727898749155,
131.208433428525));
#227685=CARTESIAN_POINT('Ctrl Pts',(-169.780033244125,-2.79361299935373,
135.900186841566));
#227686=CARTESIAN_POINT('Ctrl Pts',(-170.058480867939,2.77724685960862,
135.909124899701));
#227687=CARTESIAN_POINT('Ctrl Pts',(-170.336928491751,5.79595253064181,
131.227033964152));
#227688=CARTESIAN_POINT('Ctrl Pts',(-170.615376115564,3.48846097403773,
126.156526871832));
#227689=CARTESIAN_POINT('Ctrl Pts',(-170.893823739377,-2.02475579691427,
125.357151932539));
#227690=CARTESIAN_POINT('Ctrl Pts',(-171.17227136319,-5.67732090532164,
129.563495663847));
#227691=CARTESIAN_POINT('Ctrl Pts',(-171.450718987003,-4.11270545428381,
134.910133667999));
#227692=CARTESIAN_POINT('Ctrl Pts',(-171.729166610815,1.23128539240979,
136.483766816968));
#227693=CARTESIAN_POINT('Ctrl Pts',(-172.007614234629,5.44378511511418,
132.838303123102));
#227694=CARTESIAN_POINT('Ctrl Pts',(-172.286061858441,4.65371226071637,
127.323745630264));
#227695=CARTESIAN_POINT('Ctrl Pts',(-172.564509482254,-0.412894814796852,
125.00770327326));
#227696=CARTESIAN_POINT('Ctrl Pts',(-172.842957106067,-5.10007172654484,
128.018505833219));
#227697=CARTESIAN_POINT('Ctrl Pts',(-173.12140472988,-5.10053187395325,
133.589372843419));
#227698=CARTESIAN_POINT('Ctrl Pts',(-173.399852353693,-0.413852404033268,
136.600949673471));
#227699=CARTESIAN_POINT('Ctrl Pts',(-173.678299977506,4.65313720737985,
134.285744340263));
#227700=CARTESIAN_POINT('Ctrl Pts',(-173.956747601319,5.44412104360021,
128.771317440947));
#227701=CARTESIAN_POINT('Ctrl Pts',(-174.235195225131,1.23222360085094,
125.125157901261));
#227702=CARTESIAN_POINT('Ctrl Pts',(-174.513642848945,-4.11202713361109,
126.697908213384));
#227703=CARTESIAN_POINT('Ctrl Pts',(-174.792090472757,-5.67752581597763,
132.044287673595));
#227704=CARTESIAN_POINT('Ctrl Pts',(-175.070538096571,-2.02565563601667,
136.251234743121));
#227705=CARTESIAN_POINT('Ctrl Pts',(-175.348985720383,3.48769311466452,
135.452770585855));
#227706=CARTESIAN_POINT('Ctrl Pts',(-175.627433344196,5.79602227624969,
130.382644755183));
#227707=CARTESIAN_POINT('Ctrl Pts',(-175.905880968009,2.77809011739122,
125.700055200075));
#227708=CARTESIAN_POINT('Ctrl Pts',(-176.184328591822,-2.79277114210269,
125.708072964459));
#227709=CARTESIAN_POINT('Ctrl Pts',(-176.462776215635,-5.79721215645926,
130.399330114555));
#227710=CARTESIAN_POINT('Ctrl Pts',(-176.741223839448,-3.47429840858841,
135.462790510077));
#227711=CARTESIAN_POINT('Ctrl Pts',(-177.019671463261,2.04132584786218,
136.245381411334));
#227712=CARTESIAN_POINT('Ctrl Pts',(-177.298119087073,5.68107137443935,
132.02794001176));
#227713=CARTESIAN_POINT('Ctrl Pts',(-177.576566710886,4.10018984367198,
126.686088924097));
#227714=CARTESIAN_POINT('Ctrl Pts',(-177.855014334699,-1.24856584802001,
125.128728333976));
#227715=CARTESIAN_POINT('Ctrl Pts',(-178.133461958512,-5.4499505212146,
128.786996542421));
#227716=CARTESIAN_POINT('Ctrl Pts',(-178.411909582325,-4.64309691029714,
134.29912378221));
#227717=CARTESIAN_POINT('Ctrl Pts',(-178.690357206138,0.430535933288815,
136.599734402363));
#227718=CARTESIAN_POINT('Ctrl Pts',(-178.968804829951,5.10852728703229,
133.574679634036));
#227719=CARTESIAN_POINT('Ctrl Pts',(-179.247252453763,5.09203162942501,
128.00383702718));
#227720=CARTESIAN_POINT('Ctrl Pts',(-179.525700077576,0.396207663951002,
125.006538786706));
#227721=CARTESIAN_POINT('Ctrl Pts',(-179.80414770139,-4.66371178887382,
127.337155569449));
#227722=CARTESIAN_POINT('Ctrl Pts',(-180.082595325202,-5.43790794271038,
132.853964409027));
#227723=CARTESIAN_POINT('Ctrl Pts',(-180.361042949015,-1.2149323537682,
136.487287492965));
#227724=CARTESIAN_POINT('Ctrl Pts',(-180.639490572828,4.12450671554208,
134.898278404822));
#227725=CARTESIAN_POINT('Ctrl Pts',(-180.917938196641,5.67372560662389,
129.547158869193));
#227726=CARTESIAN_POINT('Ctrl Pts',(-181.196385820454,2.00906784212309,
125.351346322599));
#227727=CARTESIAN_POINT('Ctrl Pts',(-181.474833444267,-3.50182512086801,
126.166587518521));
#227728=CARTESIAN_POINT('Ctrl Pts',(-181.75328106808,-5.79471187144949,
131.243715624654));
#227729=CARTESIAN_POINT('Ctrl Pts',(-182.031728691892,-2.76254149958135,
135.917097942958));
#227730=CARTESIAN_POINT('Ctrl Pts',(-182.310176315705,2.80826955274668,
135.892124430331));
#227731=CARTESIAN_POINT('Ctrl Pts',(-182.588623939518,5.79841807769547,
131.191744524852));
#227732=CARTESIAN_POINT('Ctrl Pts',(-182.867071563331,3.46010365771282,
126.135377733334));
#227733=CARTESIAN_POINT('Ctrl Pts',(-183.145519187144,-2.05787698824661,
125.369578119929));
#227734=CARTESIAN_POINT('Ctrl Pts',(-183.423966810957,-5.68476921488759,
129.598078117967));
#227735=CARTESIAN_POINT('Ctrl Pts',(-183.70241443477,-4.08763624946197,
134.93509280296));
#227736=CARTESIAN_POINT('Ctrl Pts',(-183.980862058583,1.26583473708647,
136.476166407061));
#227737=CARTESIAN_POINT('Ctrl Pts',(-184.259309682396,5.45606543971754,
132.805127573733));
#227738=CARTESIAN_POINT('Ctrl Pts',(-184.537757306209,4.63243854686269,
127.295481650585));
#227739=CARTESIAN_POINT('Ctrl Pts',(-184.816204930021,-0.448173063354899,
125.010324079826));
#227740=CARTESIAN_POINT('Ctrl Pts',(-185.094652553834,-5.11693552282041,
128.049603032828));
#227741=CARTESIAN_POINT('Ctrl Pts',(-185.373100177647,-5.08348421301165,
133.620369628814));
#227742=CARTESIAN_POINT('Ctrl Pts',(-185.65154780146,-0.378559253454916,
136.60336151315));
#227743=CARTESIAN_POINT('Ctrl Pts',(-185.929995425273,4.67424316637891,
134.257354871388));
#227744=CARTESIAN_POINT('Ctrl Pts',(-186.208443049086,5.4316444657843,128.73821519851));
#227745=CARTESIAN_POINT('Ctrl Pts',(-186.486890672899,1.19762985171755,
125.117762228929));
#227746=CARTESIAN_POINT('Ctrl Pts',(-186.765338296712,-4.13694808860639,
126.72301537273));
#227747=CARTESIAN_POINT('Ctrl Pts',(-187.043785920525,-5.66987283665109,
132.078825411735));
#227748=CARTESIAN_POINT('Ctrl Pts',(-187.322233544337,-1.99246143649967,
136.263464565965));
#227749=CARTESIAN_POINT('Ctrl Pts',(-187.600681168151,3.51592468664221,
135.43145388367));
#227750=CARTESIAN_POINT('Ctrl Pts',(-187.879128791963,5.79334778522967,
130.347370535898));
#227751=CARTESIAN_POINT('Ctrl Pts',(-188.157576415776,2.74696728996466,
125.683238747971));
#227752=CARTESIAN_POINT('Ctrl Pts',(-188.436024039589,-2.82374194796541,
125.72516777749));
#227753=CARTESIAN_POINT('Ctrl Pts',(-188.714471663402,-5.79957028317828,
130.434626894674));
#227754=CARTESIAN_POINT('Ctrl Pts',(-188.992919287215,-3.44587685290989,
135.483853240698));
#227755=CARTESIAN_POINT('Ctrl Pts',(-189.271366911028,2.07440906473995,
136.232854471987));
#227756=CARTESIAN_POINT('Ctrl Pts',(-189.54981453484,5.68841439241029,131.993335047731));
#227757=CARTESIAN_POINT('Ctrl Pts',(-189.828262158654,4.07504478794802,
126.661206206783));
#227758=CARTESIAN_POINT('Ctrl Pts',(-190.106709782466,-1.28309189963338,
125.136433864998));
#227759=CARTESIAN_POINT('Ctrl Pts',(-190.385157406279,-5.46212981397553,
128.820209315208));
#227760=CARTESIAN_POINT('Ctrl Pts',(-190.663605030092,-4.62173726915045,
134.327322881104));
#227761=CARTESIAN_POINT('Ctrl Pts',(-190.942052653905,0.465806041606811,
136.597006233083));
#227762=CARTESIAN_POINT('Ctrl Pts',(-191.220500277718,5.12529635601715,
133.543531250871));
#227763=CARTESIAN_POINT('Ctrl Pts',(-191.49894790153,5.07488970389458,127.972892272577));
#227764=CARTESIAN_POINT('Ctrl Pts',(-191.777395525344,0.360907336037817,
125.004234378408));
#227765=CARTESIAN_POINT('Ctrl Pts',(-192.055843149156,-4.68473124233415,
127.365609146106));
#227766=CARTESIAN_POINT('Ctrl Pts',(-192.33429077297,-5.42533067084548,
132.887028523726));
#227767=CARTESIAN_POINT('Ctrl Pts',(-192.612738396782,-1.1803162549878,
136.494577839569));
#227768=CARTESIAN_POINT('Ctrl Pts',(-192.891186020595,4.14935113754904,
134.873095510955));
#227769=CARTESIAN_POINT('Ctrl Pts',(-193.169633644408,5.66596754175055,
129.512644584067));
#227770=CARTESIAN_POINT('Ctrl Pts',(-193.448081268221,1.97583657298603,
125.339217588127));
#227771=CARTESIAN_POINT('Ctrl Pts',(-193.726528892034,-3.52999168137001,
126.187990049162));
#227772=CARTESIAN_POINT('Ctrl Pts',(-194.004976515847,-5.79193003022761,
131.27898154032));
#227773=CARTESIAN_POINT('Ctrl Pts',(-194.28342413966,-2.73136763281852,
135.933819589987));
#227774=CARTESIAN_POINT('Ctrl Pts',(-194.561871763472,2.83918818442447,
135.874935432001));
#227775=CARTESIAN_POINT('Ctrl Pts',(-194.840319387286,5.80066876223446,
131.156440730899));
#227776=CARTESIAN_POINT('Ctrl Pts',(-195.118767011098,3.43161812597426,
126.114401605713));
#227777=CARTESIAN_POINT('Ctrl Pts',(-195.397214634911,-2.09092192419104,
125.382205695184));
#227778=CARTESIAN_POINT('Ctrl Pts',(-195.675662258724,-5.69200687323938,
129.63270527133));
#227779=CARTESIAN_POINT('Ctrl Pts',(-195.954109882537,-4.06241557577554,
134.95989887212));
#227780=CARTESIAN_POINT('Ctrl Pts',(-196.23255750635,1.30033717579212,136.468355826305));
#227781=CARTESIAN_POINT('Ctrl Pts',(-196.511005130163,5.46814358780935,
132.771877885207));
#227782=CARTESIAN_POINT('Ctrl Pts',(-196.789452753976,4.61099317629508,
127.267347693709));
#227783=CARTESIAN_POINT('Ctrl Pts',(-197.067900377789,-0.483434704694746,
125.013159586548));
#227784=CARTESIAN_POINT('Ctrl Pts',(-197.346348001602,-5.13360970916836,
128.080802310993));
#227785=CARTESIAN_POINT('Ctrl Pts',(-197.624795625414,-5.06624818169292,
133.651262065958));
#227786=CARTESIAN_POINT('Ctrl Pts',(-197.903243249227,-0.343252075224855,
136.605558468718));
#227787=CARTESIAN_POINT('Ctrl Pts',(-198.18169087304,4.69517591957924,134.228837450539));
#227788=CARTESIAN_POINT('Ctrl Pts',(-198.460138496853,5.41896661638458,
128.705189517851));
#227789=CARTESIAN_POINT('Ctrl Pts',(-198.738586120666,1.1629917239694,125.110577275591));
#227790=CARTESIAN_POINT('Ctrl Pts',(-199.017033744479,-4.16171574746965,
126.748273767825));
#227791=CARTESIAN_POINT('Ctrl Pts',(-199.295481368292,-5.6620097581009,
132.113315924113));
#227792=CARTESIAN_POINT('Ctrl Pts',(-199.573928992105,-1.95919340559182,
136.275492099704));
#227793=CARTESIAN_POINT('Ctrl Pts',(-199.852376615917,3.54402597473752,
135.409965722843));
#227794=CARTESIAN_POINT('Ctrl Pts',(-200.13082423973,5.79045861957696,130.312113250549));
#227795=CARTESIAN_POINT('Ctrl Pts',(-200.409271863544,2.71574267265526,
125.666612060922));
#227796=CARTESIAN_POINT('Ctrl Pts',(-200.687719487356,-2.85460811903155,
125.742450801881));
#227797=CARTESIAN_POINT('Ctrl Pts',(-200.966167111169,-5.80171350468764,
130.469937375411));
#227798=CARTESIAN_POINT('Ctrl Pts',(-201.244614734982,-3.41732760899753,
135.504742570997));
#227799=CARTESIAN_POINT('Ctrl Pts',(-201.523062358795,2.10741541362659,
136.220126377805));
#227800=CARTESIAN_POINT('Ctrl Pts',(-201.801509982608,5.69554662409457,
131.958686025817));
#227801=CARTESIAN_POINT('Ctrl Pts',(-202.079957606421,4.04974872994014,
126.636477015578));
#227802=CARTESIAN_POINT('Ctrl Pts',(-202.358405230234,-1.31757040580477,
125.144349423131));
#227803=CARTESIAN_POINT('Ctrl Pts',(-202.636852854047,-5.47410670550813,
128.853495611451));
#227804=CARTESIAN_POINT('Ctrl Pts',(-202.915300477859,-4.6002063678289,
134.355391435336));
#227805=CARTESIAN_POINT('Ctrl Pts',(-203.193748101672,0.501058889310003,
136.594063415189));
#227806=CARTESIAN_POINT('Ctrl Pts',(-203.472195725485,5.14187550526088,
133.512281366733));
#227807=CARTESIAN_POINT('Ctrl Pts',(-203.750643349298,5.05755972645996,
127.942052439074));
#227808=CARTESIAN_POINT('Ctrl Pts',(-204.029090973111,0.325593634571106,
125.002144895921));
#227809=CARTESIAN_POINT('Ctrl Pts',(-204.307538596924,-4.70557710135553,
127.394190146963));
#227810=CARTESIAN_POINT('Ctrl Pts',(-204.585986220737,-5.41255236135747,
132.920015464399));
#227811=CARTESIAN_POINT('Ctrl Pts',(-204.864433844549,-1.14565641915494,
136.50165733308));
#227812=CARTESIAN_POINT('Ctrl Pts',(-205.142881468362,4.17404180382362,
134.847761848621));
#227813=CARTESIAN_POINT('Ctrl Pts',(-205.421329092175,5.6579995223666,129.478178163952));
#227814=CARTESIAN_POINT('Ctrl Pts',(-205.699776715988,1.94253208849746,
125.327291366541));
#227815=CARTESIAN_POINT('Ctrl Pts',(-205.978224339801,-3.55802743673226,
126.209563641112));
#227816=CARTESIAN_POINT('Ctrl Pts',(-206.256671963614,-5.78893356690891,
131.314229868733));
#227817=CARTESIAN_POINT('Ctrl Pts',(-206.535119587427,-2.70009255422283,
135.950351163029));
#227818=CARTESIAN_POINT('Ctrl Pts',(-206.81356721124,2.87000160893922,135.857558541658));
#227819=CARTESIAN_POINT('Ctrl Pts',(-207.092014835053,5.80270450085972,
131.121123890489));
#227820=CARTESIAN_POINT('Ctrl Pts',(-207.370462458865,3.40300543436423,
126.09359926625));
#227821=CARTESIAN_POINT('Ctrl Pts',(-207.648910082679,-2.12388938025395,
125.395034190384));
#227822=CARTESIAN_POINT('Ctrl Pts',(-207.927357706491,-5.69903361218359,
129.667375840811));
#227823=CARTESIAN_POINT('Ctrl Pts',(-208.205805330304,-4.03704436778601,
134.984550956282));
#227824=CARTESIAN_POINT('Ctrl Pts',(-208.484252954117,1.33479143002538,
136.460335364123));
#227825=CARTESIAN_POINT('Ctrl Pts',(-208.76270057793,5.48001911182977,132.738555289606));
#227826=CARTESIAN_POINT('Ctrl Pts',(-209.041148201743,4.58937694367963,
127.239344802146));
#227827=CARTESIAN_POINT('Ctrl Pts',(-209.319595825556,-0.518678432184342,
125.016209688352));
#227828=CARTESIAN_POINT('Ctrl Pts',(-209.598043449369,-5.15009366772074,
128.112102511612));
#227829=CARTESIAN_POINT('Ctrl Pts',(-209.876491073182,-5.04882441868487,
133.682049010123));
#227830=CARTESIAN_POINT('Ctrl Pts',(-210.154938696994,-0.307932177662294,
136.607540458767));
#227831=CARTESIAN_POINT('Ctrl Pts',(-210.433386320807,4.71593469130848,
134.200193134443));
#227832=CARTESIAN_POINT('Ctrl Pts',(-210.71183394462,5.40608796518471,128.672241622749));
#227833=CARTESIAN_POINT('Ctrl Pts',(-210.990281568433,1.12831050113542,
125.103603307488));
#227834=CARTESIAN_POINT('Ctrl Pts',(-211.268729192246,-4.18632919242468,
126.773682462711));
#227835=CARTESIAN_POINT('Ctrl Pts',(-211.547176816059,-5.65393687169752,
132.14775793267));
#227836=CARTESIAN_POINT('Ctrl Pts',(-211.825624439872,-1.92585277605142,
136.287316898656));
#227837=CARTESIAN_POINT('Ctrl Pts',(-212.104072063685,3.57199593764717,
135.388306899624));
#227838=CARTESIAN_POINT('Ctrl Pts',(-212.382519687498,5.78735488635066,
130.276874205606));
#227839=CARTESIAN_POINT('Ctrl Pts',(-212.660967311311,2.68441742250212,
125.650175755035));
#227840=CARTESIAN_POINT('Ctrl Pts',(-212.939414935123,-2.88536851154432,
125.759921397201));
#227841=CARTESIAN_POINT('Ctrl Pts',(-213.217862558936,-5.80364174156953,
130.505260248325));
#227842=CARTESIAN_POINT('Ctrl Pts',(-213.496310182749,-3.38865173475374,
135.525457726916));
#227843=CARTESIAN_POINT('Ctrl Pts',(-213.774757806562,2.14034367146046,
136.20719760043));
#227844=CARTESIAN_POINT('Ctrl Pts',(-214.053205430375,5.7024678052036,131.923994229952));
#227845=CARTESIAN_POINT('Ctrl Pts',(-214.331653054188,4.02430260700449,
126.611902266833));
#227846=CARTESIAN_POINT('Ctrl Pts',(-214.610100678001,-1.35200008892003,
125.152474715061));
#227847=CARTESIAN_POINT('Ctrl Pts',(-214.888548301814,-5.48588075200302,
128.886854197714));
#227848=CARTESIAN_POINT('Ctrl Pts',(-215.166995925626,-4.5785050041694,
134.383328404815));
#227849=CARTESIAN_POINT('Ctrl Pts',(-215.445443549439,0.536293170092427,
136.59090605773));
#227850=CARTESIAN_POINT('Ctrl Pts',(-215.723891173253,5.15826412041666,
133.480931139593));
#227851=CARTESIAN_POINT('Ctrl Pts',(-216.002338797065,5.04004233928969,
127.911318669453));
#227852=CARTESIAN_POINT('Ctrl Pts',(-216.280786420879,0.290267868112,125.000270416672));
#227853=CARTESIAN_POINT('Ctrl Pts',(-216.559234044691,-4.72624859348692,
127.422897512942));
#227854=CARTESIAN_POINT('Ctrl Pts',(-216.837681668504,-5.39957348775117,
132.952924008705));
#227855=CARTESIAN_POINT('Ctrl Pts',(-217.116129292317,-1.11095413060172,
136.508525711168));
#227856=CARTESIAN_POINT('Ctrl Pts',(-217.39457691613,4.19857779944424,134.822278356567));
#227857=CARTESIAN_POINT('Ctrl Pts',(-217.673024539943,5.64982184372931,
129.443760886018));
#227858=CARTESIAN_POINT('Ctrl Pts',(-217.951472163756,1.90915562276867,
125.315568099769));
#227859=CARTESIAN_POINT('Ctrl Pts',(-218.229919787568,-3.58593134807924,
126.231307494954));
#227860=CARTESIAN_POINT('Ctrl Pts',(-218.508367411381,-5.78572259252759,
131.349459303753));
#227861=CARTESIAN_POINT('Ctrl Pts',(-218.786815035194,-2.66871742270537,
135.966692049498));
#227862=CARTESIAN_POINT('Ctrl Pts',(-219.065262659007,2.90070868448967,
135.839994403207));
#227863=CARTESIAN_POINT('Ctrl Pts',(-219.34371028282,5.80452521813531,131.085795312298));
#227864=CARTESIAN_POINT('Ctrl Pts',(-219.622157906633,3.37426664313623,
126.07297148578));
#227865=CARTESIAN_POINT('Ctrl Pts',(-219.900605530446,-2.15677813481551,
125.408063130162));
#227866=CARTESIAN_POINT('Ctrl Pts',(-220.179053154259,-5.70584917134113,
129.702088541682));
#227867=CARTESIAN_POINT('Ctrl Pts',(-220.457500778071,-4.01152356563293,
135.009048141953));
#227868=CARTESIAN_POINT('Ctrl Pts',(-220.735948401884,1.36919622307095,
136.452105317718));
#227869=CARTESIAN_POINT('Ctrl Pts',(-221.014396025697,5.49169157172664,
132.705161021709));
#227870=CARTESIAN_POINT('Ctrl Pts',(-221.29284364951,4.56759065001379,127.211474013555));
#227871=CARTESIAN_POINT('Ctrl Pts',(-221.571291273323,-0.553902939853376,
125.019474272218));
#227872=CARTESIAN_POINT('Ctrl Pts',(-221.849738897136,-5.16638678765824,
128.143502474846));
#227873=CARTESIAN_POINT('Ctrl Pts',(-222.128186520948,-5.03121356963114,
133.712729320486));
#227874=CARTESIAN_POINT('Ctrl Pts',(-222.406634144762,-0.272600869560251,
136.609307409853));
#227875=CARTESIAN_POINT('Ctrl Pts',(-222.685081768574,4.73651871234416,
134.171422984523));
#227876=CARTESIAN_POINT('Ctrl Pts',(-222.963529392388,5.39300898940659,
128.639372734101));
#227877=CARTESIAN_POINT('Ctrl Pts',(-223.2419770162,1.09358746834067,125.096840583045));
#227878=CARTESIAN_POINT('Ctrl Pts',(-223.520424640014,-4.21078751141269,
126.799240515859));
#227879=CARTESIAN_POINT('Ctrl Pts',(-223.798872263826,-5.64565447658353,
132.182150161146));
#227880=CARTESIAN_POINT('Ctrl Pts',(-224.077319887639,-1.89244078332859,
136.298938524645));
#227881=CARTESIAN_POINT('Ctrl Pts',(-224.355767511452,3.59983353893359,
135.366478216591));
#227882=CARTESIAN_POINT('Ctrl Pts',(-224.634215135265,5.78403670056078,
130.241654706868));
#227883=CARTESIAN_POINT('Ctrl Pts',(-224.912662759078,2.65299270027449,
125.633930439363));
#227884=CARTESIAN_POINT('Ctrl Pts',(-225.191110382891,-2.91602198566553,
125.77757891607));
#227885=CARTESIAN_POINT('Ctrl Pts',(-225.469558006704,-5.8053549223724,
130.540594204513));
#227886=CARTESIAN_POINT('Ctrl Pts',(-225.748005630516,-3.35985029277391,
135.545997940844));
#227887=CARTESIAN_POINT('Ctrl Pts',(-226.026453254329,2.17319261807209,
136.194068618944));
#227888=CARTESIAN_POINT('Ctrl Pts',(-226.304900878142,5.7091776792716,131.88926094565));
#227889=CARTESIAN_POINT('Ctrl Pts',(-226.583348501955,3.99870736205508,
126.587482871174));
#227890=CARTESIAN_POINT('Ctrl Pts',(-226.861796125768,-1.38637967317499,
125.160809439701));
#227891=CARTESIAN_POINT('Ctrl Pts',(-227.140243749581,-5.49745151716988,
128.920283837883));
#227892=CARTESIAN_POINT('Ctrl Pts',(-227.418691373394,-4.55663398232247,
134.411132754326));
#227893=CARTESIAN_POINT('Ctrl Pts',(-227.697138997207,0.571507578333558,
136.5875342777));
#227894=CARTESIAN_POINT('Ctrl Pts',(-227.97558662102,5.17446159419872,133.44948173115));
#227895=CARTESIAN_POINT('Ctrl Pts',(-228.254034244832,5.02233819149715,
127.880692102567));
#227896=CARTESIAN_POINT('Ctrl Pts',(-228.532481868645,0.254931345670833,
124.998611010119));
#227897=CARTESIAN_POINT('Ctrl Pts',(-228.810929492458,-4.74674495273865,
127.451730180279));
#227898=CARTESIAN_POINT('Ctrl Pts',(-229.089377116271,-5.38639453096373,
132.985752937203));
#227899=CARTESIAN_POINT('Ctrl Pts',(-229.367824740084,-1.07621067523457,
136.515182719319));
#227900=CARTESIAN_POINT('Ctrl Pts',(-229.646272363897,4.22295821522052,
134.796645979094));
#227901=CARTESIAN_POINT('Ctrl Pts',(-229.92471998771,5.64143480886619,129.409394025606));
#227902=CARTESIAN_POINT('Ctrl Pts',(-230.203167611523,1.87570841257552,
125.304048222223));
#227903=CARTESIAN_POINT('Ctrl Pts',(-230.481615235336,-3.61370238142155,
126.25322080496));
#227904=CARTESIAN_POINT('Ctrl Pts',(-230.760062859148,-5.78229722606833,
131.384668539942));
#227905=CARTESIAN_POINT('Ctrl Pts',(-231.038510482961,-2.63724340088164,
135.982841643878));
#227906=CARTESIAN_POINT('Ctrl Pts',(-231.316958106774,2.93130827321233,
135.822243667495));
#227907=CARTESIAN_POINT('Ctrl Pts',(-231.595405730587,5.80613084659478,
131.050456305442));
#227908=CARTESIAN_POINT('Ctrl Pts',(-231.8738533544,3.34540281721704,126.052519028673));
#227909=CARTESIAN_POINT('Ctrl Pts',(-232.152300978213,-2.18958696916944,
125.42129203173));
#227910=CARTESIAN_POINT('Ctrl Pts',(-232.430748602025,-5.71245329815966,
129.736842087648));
#227911=CARTESIAN_POINT('Ctrl Pts',(-232.709196225839,-3.98585411499877,
135.033389521383));
#227912=CARTESIAN_POINT('Ctrl Pts',(-232.987643849651,1.40355028004735,
136.443665992055));
#227913=CARTESIAN_POINT('Ctrl Pts',(-233.266091473464,5.50316053497282,
132.671696318956));
#227914=CARTESIAN_POINT('Ctrl Pts',(-233.544539097277,4.5456351025967,127.183736360699));
#227915=CARTESIAN_POINT('Ctrl Pts',(-233.82298672109,-0.589106922445798,
125.022953217175));
#227916=CARTESIAN_POINT('Ctrl Pts',(-234.101434344904,-5.18248846523346,
128.175001037157));
#227917=CARTESIAN_POINT('Ctrl Pts',(-234.379881968716,-5.01341628710851,
133.743301860178));
#227918=CARTESIAN_POINT('Ctrl Pts',(-234.658329592529,-0.237259460132118,
136.610859256499));
#227919=CARTESIAN_POINT('Ctrl Pts',(-234.936777216342,4.75692721993639,
134.14252806687));
#227920=CARTESIAN_POINT('Ctrl Pts',(-235.215224840155,5.37973017369771,
128.606584069875));
#227921=CARTESIAN_POINT('Ctrl Pts',(-235.493672463967,1.05882391226032,
125.090289352854));
#227922=CARTESIAN_POINT('Ctrl Pts',(-235.772120087781,-4.23508979812022,
126.824946980203));
#227923=CARTESIAN_POINT('Ctrl Pts',(-236.050567711593,-5.63716287966734,
132.216491335124));
#227924=CARTESIAN_POINT('Ctrl Pts',(-236.329015335406,-1.85895866551617,
136.310356547029));
#227925=CARTESIAN_POINT('Ctrl Pts',(-236.607462959219,3.62753774706455,
135.344480482612));
#227926=CARTESIAN_POINT('Ctrl Pts',(-236.885910583032,5.78050418516386,
130.206456059403));
#227927=CARTESIAN_POINT('Ctrl Pts',(-237.164358206845,2.62146967042642,
125.617876715884));
#227928=CARTESIAN_POINT('Ctrl Pts',(-237.442805830658,-2.94656740551997,
125.795422704185));
#227929=CARTESIAN_POINT('Ctrl Pts',(-237.72125345447,-5.80685298361372,
130.575937934662));
#227930=CARTESIAN_POINT('Ctrl Pts',(-237.999701078284,-3.33092435030571,
135.566362451659));
#227931=CARTESIAN_POINT('Ctrl Pts',(-238.278148702096,2.20596103623244,
136.180739919846));
#227932=CARTESIAN_POINT('Ctrl Pts',(-238.55659632591,5.7156759976606,131.854487459968));
#227933=CARTESIAN_POINT('Ctrl Pts',(-238.835043949722,3.97296394353457,
126.56321973347));
#227934=CARTESIAN_POINT('Ctrl Pts',(-239.113491573535,-1.42070788462113,
125.169353288205));
#227935=CARTESIAN_POINT('Ctrl Pts',(-239.391939197348,-5.50881857224844,
128.95378329321));
#227936=CARTESIAN_POINT('Ctrl Pts',(-239.670386821161,-4.53459411272838,
134.438803453569));
#227937=CARTESIAN_POINT('Ctrl Pts',(-239.948834444974,0.606700809151854,
136.583948200045));
#227938=CARTESIAN_POINT('Ctrl Pts',(-240.227282068787,5.1904673264033,133.417934306771));
#227939=CARTESIAN_POINT('Ctrl Pts',(-240.5057296926,5.00444793911587,127.850173873291));
#227940=CARTESIAN_POINT('Ctrl Pts',(-240.784177316413,0.21958537665436,
124.997166737753));
#227941=CARTESIAN_POINT('Ctrl Pts',(-241.062624940225,-4.76706541961049,
127.48068708057));
#227942=CARTESIAN_POINT('Ctrl Pts',(-241.341072564039,-5.37301597934592,
133.018501033406));
#227943=CARTESIAN_POINT('Ctrl Pts',(-241.619520187851,-1.04142734048567,
136.521628110858));
#227944=CARTESIAN_POINT('Ctrl Pts',(-241.897967811664,4.24718214772698,
134.770865666018));
#227945=CARTESIAN_POINT('Ctrl Pts',(-242.176415435477,5.63283872856131,
129.375078856195));
#227946=CARTESIAN_POINT('Ctrl Pts',(-242.45486305929,1.84219169731802,125.292732160775));
#227947=CARTESIAN_POINT('Ctrl Pts',(-242.733310683103,-3.64133950769301,
126.275302759127));
#227948=CARTESIAN_POINT('Ctrl Pts',(-243.011758306915,-5.77865759445851,
131.419856272607));
#227949=CARTESIAN_POINT('Ctrl Pts',(-243.290205930729,-2.60567165503458,
135.998799347738));
#227950=CARTESIAN_POINT('Ctrl Pts',(-243.568653554541,2.96179924122969,
135.80430699228));
#227951=CARTESIAN_POINT('Ctrl Pts',(-243.847101178355,5.80752132674009,
131.015108179419));
#227952=CARTESIAN_POINT('Ctrl Pts',(-244.125548802166,3.31641502616601,
126.032242652805));
#227953=CARTESIAN_POINT('Ctrl Pts',(-244.403996425981,-2.22231466757369,
125.434720404883));
#227954=CARTESIAN_POINT('Ctrl Pts',(-244.682444049792,-5.71884574792013,
129.771635190908));
#227955=CARTESIAN_POINT('Ctrl Pts',(-244.960891673606,-3.96003696707471,
135.05757419259));
#227956=CARTESIAN_POINT('Ctrl Pts',(-245.239339297418,1.43785232795156,
136.435017699859));
#227957=CARTESIAN_POINT('Ctrl Pts',(-245.517786921232,5.51442557658153,
132.638162421391));
#227958=CARTESIAN_POINT('Ctrl Pts',(-245.796234545044,4.52351111499922,
127.156132871406));
#227959=CARTESIAN_POINT('Ctrl Pts',(-246.074682168857,-0.624289075464052,
125.026646394309));
#227960=CARTESIAN_POINT('Ctrl Pts',(-246.353129792671,-5.19839810379266,
128.206597031353));
#227961=CARTESIAN_POINT('Ctrl Pts',(-246.631577416483,-4.99543323060155,
133.773765496319));
#227962=CARTESIAN_POINT('Ctrl Pts',(-246.910025040296,-0.201909258968066,
136.612195941205));
#227963=CARTESIAN_POINT('Ctrl Pts',(-247.188472664109,4.77715945784187,
134.113509452194));
#227964=CARTESIAN_POINT('Ctrl Pts',(-247.466920287922,5.36625201010822,
128.573876845067));
#227965=CARTESIAN_POINT('Ctrl Pts',(-247.745367911734,1.02402112107033,
125.083949859676));
#227966=CARTESIAN_POINT('Ctrl Pts',(-248.023815535548,-4.25923515201858,
126.850800903184));
#227967=CARTESIAN_POINT('Ctrl Pts',(-248.30226315936,-5.62846239560694,
132.250780182078));
#227968=CARTESIAN_POINT('Ctrl Pts',(-248.580710783174,-1.82540766330725,
136.32157054271));
#227969=CARTESIAN_POINT('Ctrl Pts',(-248.859158406986,3.65510753545023,
135.322314512822));
#227970=CARTESIAN_POINT('Ctrl Pts',(-249.137606030799,5.7767574710584,130.171279567513));
#227971=CARTESIAN_POINT('Ctrl Pts',(-249.416053654612,2.58984950105633,
125.602015179472));
#227972=CARTESIAN_POINT('Ctrl Pts',(-249.694501278425,-2.97700363923603,
125.813452100338));
#227973=CARTESIAN_POINT('Ctrl Pts',(-249.972948902238,-5.80813586978118,
130.611290129096));
#227974=CARTESIAN_POINT('Ctrl Pts',(-250.251396526051,-3.30187497921299,
135.586550504748));
#227975=CARTESIAN_POINT('Ctrl Pts',(-250.529844149864,2.23864771169993,
136.167211997028));
#227976=CARTESIAN_POINT('Ctrl Pts',(-250.808291773676,5.72196251956533,
131.819675061465));
#227977=CARTESIAN_POINT('Ctrl Pts',(-251.08673939749,3.94707330538994,126.539113752772));
#227978=CARTESIAN_POINT('Ctrl Pts',(-251.365187021302,-1.45498345124562,
125.178105944033));
#227979=CARTESIAN_POINT('Ctrl Pts',(-251.643634645115,-5.5199814959705,
128.987351322257));
#227980=CARTESIAN_POINT('Ctrl Pts',(-251.922082268928,-4.51238621219265,
134.466339477392));
#227981=CARTESIAN_POINT('Ctrl Pts',(-252.200529892741,0.641871558658502,
136.580147957277));
#227982=CARTESIAN_POINT('Ctrl Pts',(-252.478977516554,5.20628072353487,
133.386290036154));
#227983=CARTESIAN_POINT('Ctrl Pts',(-252.757425140367,4.98637224582674,
127.819765111179));
#227984=CARTESIAN_POINT('Ctrl Pts',(-253.035872764179,0.184231269403876,
124.995937655572));
#227985=CARTESIAN_POINT('Ctrl Pts',(-253.314320387993,-4.78720923844335,
127.509767136124));
#227986=CARTESIAN_POINT('Ctrl Pts',(-253.592768011806,-5.35943833369967,
133.051167092665));
#227987=CARTESIAN_POINT('Ctrl Pts',(-253.871215635618,-1.00660540571931,
136.527861630253));
#227988=CARTESIAN_POINT('Ctrl Pts',(-254.149663259431,4.27124868131666,
134.744938404161));
#227989=CARTESIAN_POINT('Ctrl Pts',(-254.428110883244,5.62403395537261,
129.340816589823));
#227990=CARTESIAN_POINT('Ctrl Pts',(-254.706558507057,1.80860665472018,
125.281620447135));
#227991=CARTESIAN_POINT('Ctrl Pts',(-254.98500613087,-3.66884158147516,
126.297552326988));
#227992=CARTESIAN_POINT('Ctrl Pts',(-255.263453754682,-5.77480406163408,
131.45502159855));
#227993=CARTESIAN_POINT('Ctrl Pts',(-255.541901378496,-2.57400292253984,
136.014563813166));
#227994=CARTESIAN_POINT('Ctrl Pts',(-255.820349002309,2.99217964199006,
135.78618647082));
#227995=CARTESIAN_POINT('Ctrl Pts',(-256.098796626121,5.80869814913581,
130.979749546569));
#227996=CARTESIAN_POINT('Ctrl Pts',(-256.377244249934,3.28730143236016,
126.01214820295));
#227997=CARTESIAN_POINT('Ctrl Pts',(-256.655691873747,-2.25495451926359,
125.448338134603));
#227998=CARTESIAN_POINT('Ctrl Pts',(-256.93413949756,-5.72503666514098,
129.806484721847));
#227999=CARTESIAN_POINT('Ctrl Pts',(-257.212587121373,-3.93405347634203,
135.081566970265));
#228000=CARTESIAN_POINT('Ctrl Pts',(-257.491034745186,1.47206408278265,
136.426225506557));
#228001=CARTESIAN_POINT('Ctrl Pts',(-257.769482368999,5.52555616721843,
132.604438319186));
#228002=CARTESIAN_POINT('Ctrl Pts',(-258.047929992812,4.50108754276566,
127.128895412351));
#228003=CARTESIAN_POINT('Ctrl Pts',(-258.326377616624,-0.659198908970111,
125.030117734768));
#228004=CARTESIAN_POINT('Ctrl Pts',(-258.604825240438,-5.21458571703409,
128.239112839452));
#228005=CARTESIAN_POINT('Ctrl Pts',(-258.883272864251,-4.97637574492231,
133.802560593787));
#228006=CARTESIAN_POINT('Ctrl Pts',(-259.161720488063,-0.168236736403017,
136.616288572087));
#228007=CARTESIAN_POINT('Ctrl Pts',(-259.440168111876,4.80044487344316,
134.078525892203));
#228008=CARTESIAN_POINT('Ctrl Pts',(-259.672207798387,5.25516631655033,
129.4749169549));
#228009=CARTESIAN_POINT('Ctrl Pts',(-259.857849473896,3.17366342871357,
126.795179433485));
#228010=CARTESIAN_POINT('Ctrl Pts',(-259.9506752748,1.64266665146648,126.102093112095));
#228011=CARTESIAN_POINT('Ctrl Pts',(-259.997093138402,0.835778587061721,
125.962806053044));
#228012=CARTESIAN_POINT('Ctrl Pts',(210.385579563201,-2.29217962691353,
126.082387726892));
#228013=CARTESIAN_POINT('Ctrl Pts',(210.339169886847,-3.0789974560272,126.464330840008));
#228014=CARTESIAN_POINT('Ctrl Pts',(210.246352273192,-4.44507089109247,
127.629120819077));
#228015=CARTESIAN_POINT('Ctrl Pts',(210.060718784933,-5.78798125627161,
130.996088365878));
#228016=CARTESIAN_POINT('Ctrl Pts',(209.828679098422,-3.95783017776954,
135.586872998689));
#228017=CARTESIAN_POINT('Ctrl Pts',(209.550231474609,1.89393692750204,136.720289837399));
#228018=CARTESIAN_POINT('Ctrl Pts',(209.271783850796,5.99602695027556,132.40812259401));
#228019=CARTESIAN_POINT('Ctrl Pts',(208.993336226983,4.59288360023261,126.626877830413));
#228020=CARTESIAN_POINT('Ctrl Pts',(208.71488860317,-1.03344059257722,124.682062423228));
#228021=CARTESIAN_POINT('Ctrl Pts',(208.436440979357,-5.70873650289865,
128.364647771496));
#228022=CARTESIAN_POINT('Ctrl Pts',(208.157993355544,-5.13869562717284,
134.288517668348));
#228023=CARTESIAN_POINT('Ctrl Pts',(207.879545731732,0.153933173725622,
137.010984097728));
#228024=CARTESIAN_POINT('Ctrl Pts',(207.601098107919,5.30490488755997,134.029672582798));
#228025=CARTESIAN_POINT('Ctrl Pts',(207.322650484106,5.58103410012833,128.084559773234));
#228026=CARTESIAN_POINT('Ctrl Pts',(207.044202860293,0.728409521696789,
124.638756607567));
#228027=CARTESIAN_POINT('Ctrl Pts',(206.76575523648,-4.79355811073501,126.858871164077));
#228028=CARTESIAN_POINT('Ctrl Pts',(206.487307612667,-5.91049575314416,
132.704682504842));
#228029=CARTESIAN_POINT('Ctrl Pts',(206.208859988854,-1.59596820864792,
136.804198957117));
#228030=CARTESIAN_POINT('Ctrl Pts',(205.930412365042,4.1851717387407,135.390152799229));
#228031=CARTESIAN_POINT('Ctrl Pts',(205.651964741228,6.12034565262566,129.76198992389));
#228032=CARTESIAN_POINT('Ctrl Pts',(205.373517117416,2.43121966936229,125.091713591677));
#228033=CARTESIAN_POINT('Ctrl Pts',(205.095069493603,-3.49207776276838,
125.671081434371));
#228034=CARTESIAN_POINT('Ctrl Pts',(204.81662186979,-6.20632667560231,130.96768173473));
#228035=CARTESIAN_POINT('Ctrl Pts',(204.538174245977,-3.21726438559061,
136.114198085604));
#228036=CARTESIAN_POINT('Ctrl Pts',(204.259726622164,2.72830660529182,136.381233108793));
#228037=CARTESIAN_POINT('Ctrl Pts',(203.981278998351,6.16669716267351,131.523394807979));
#228038=CARTESIAN_POINT('Ctrl Pts',(203.702831374538,3.9381942601484,126.004799186432));
#228039=CARTESIAN_POINT('Ctrl Pts',(203.424383750725,-1.909316761502,124.896766062528));
#228040=CARTESIAN_POINT('Ctrl Pts',(203.145936126912,-6.00225896230248,
129.217523725228));
#228041=CARTESIAN_POINT('Ctrl Pts',(202.867488503099,-4.57941839934143,
134.996506974633));
#228042=CARTESIAN_POINT('Ctrl Pts',(202.589040879287,1.05168395343957,136.923112517541));
#228043=CARTESIAN_POINT('Ctrl Pts',(202.310593255474,5.71634013176502,133.226883983125));
#228044=CARTESIAN_POINT('Ctrl Pts',(202.032145631661,5.12795898713612,127.30447482202));
#228045=CARTESIAN_POINT('Ctrl Pts',(201.753698007848,-0.172765951628197,
124.598289728405));
#228046=CARTESIAN_POINT('Ctrl Pts',(201.475250384035,-5.31472742110118,
127.595180598346));
#228047=CARTESIAN_POINT('Ctrl Pts',(201.196802760222,-5.57271402936141,
133.541151128878));
#228048=CARTESIAN_POINT('Ctrl Pts',(200.918355136409,-0.709648686901125,
136.972144879116));
#228049=CARTESIAN_POINT('Ctrl Pts',(200.639907512596,4.80554913058071,134.735246206027));
#228050=CARTESIAN_POINT('Ctrl Pts',(200.361459888783,5.90468206117194,128.886055711564));
#228051=CARTESIAN_POINT('Ctrl Pts',(200.083012264971,1.57770063730838,124.799693711321));
#228052=CARTESIAN_POINT('Ctrl Pts',(199.804564641158,-4.19911059728431,
126.231327253625));
#228053=CARTESIAN_POINT('Ctrl Pts',(199.526117017345,-6.11714433092778,
131.865355052293));
#228054=CARTESIAN_POINT('Ctrl Pts',(199.247669393532,-2.4138212635637,136.524380797905));
#228055=CARTESIAN_POINT('Ctrl Pts',(198.969221769719,3.50768562329156,135.926987436306));
#228056=CARTESIAN_POINT('Ctrl Pts',(198.690774145906,6.20580078231077,130.622150282517));
#228057=CARTESIAN_POINT('Ctrl Pts',(198.412326522093,3.20108819260905,125.484755525167));
#228058=CARTESIAN_POINT('Ctrl Pts',(198.13387889828,-2.74526806424844,125.235817970576));
#228059=CARTESIAN_POINT('Ctrl Pts',(197.855431274468,-6.16885708386238,
130.104099070135));
#228060=CARTESIAN_POINT('Ctrl Pts',(197.576983650655,-3.92356780882929,
135.615886322105));
#228061=CARTESIAN_POINT('Ctrl Pts',(197.298536026841,1.92728860557448,136.706116507701));
#228062=CARTESIAN_POINT('Ctrl Pts',(197.020088403029,6.00706094473797,132.372921347066));
#228063=CARTESIAN_POINT('Ctrl Pts',(196.741640779216,4.56663773692898,126.598295504472));
#228064=CARTESIAN_POINT('Ctrl Pts',(196.463193155403,-1.07030245846182,
124.688838023107));
#228065=CARTESIAN_POINT('Ctrl Pts',(196.184745531591,-5.72368698170812,
128.399247046161));
#228066=CARTESIAN_POINT('Ctrl Pts',(195.906297907777,-5.11728278641862,
134.319837945007));
#228067=CARTESIAN_POINT('Ctrl Pts',(195.627850283965,0.191654296427489,
137.009876920548));
#228068=CARTESIAN_POINT('Ctrl Pts',(195.349402660151,5.32447044368961,133.997349569974));
#228069=CARTESIAN_POINT('Ctrl Pts',(195.070955036339,5.56435836804288,128.050621358318));
#228070=CARTESIAN_POINT('Ctrl Pts',(194.792507412526,0.690872786183208,
124.634444998269));
#228071=CARTESIAN_POINT('Ctrl Pts',(194.514059788713,-4.81749113516689,
126.888119675218));
#228072=CARTESIAN_POINT('Ctrl Pts',(194.2356121649,-5.89881605082435,132.740628459178));
#228073=CARTESIAN_POINT('Ctrl Pts',(193.957164541087,-1.55941718895885,
136.81380168864));
#228074=CARTESIAN_POINT('Ctrl Pts',(193.678716917274,4.21300988779493,135.364592151301));
#228075=CARTESIAN_POINT('Ctrl Pts',(193.400269293461,6.11388669464029,129.724752614155));
#228076=CARTESIAN_POINT('Ctrl Pts',(193.121821669648,2.39640030908087,125.077020090361));
#228077=CARTESIAN_POINT('Ctrl Pts',(192.843374045836,-3.52326088986039,
125.692433714928));
#228078=CARTESIAN_POINT('Ctrl Pts',(192.564926422022,-6.20521745188322,
131.005458431507));
#228079=CARTESIAN_POINT('Ctrl Pts',(192.28647879821,-3.1848823173506,136.133684081248));
#228080=CARTESIAN_POINT('Ctrl Pts',(192.008031174397,2.76220407667619,136.36452181979));
#228081=CARTESIAN_POINT('Ctrl Pts',(191.729583550584,6.17095986540858,131.485843042463));
#228082=CARTESIAN_POINT('Ctrl Pts',(191.451135926771,3.90890500597959,125.980915208923));
#228083=CARTESIAN_POINT('Ctrl Pts',(191.172688302958,-1.94524259331895,
124.908498067517));
#228084=CARTESIAN_POINT('Ctrl Pts',(190.894240679145,-6.01180727974115,
129.254090580708));
#228085=CARTESIAN_POINT('Ctrl Pts',(190.615793055332,-4.5538147691942,135.024305522869));
#228086=CARTESIAN_POINT('Ctrl Pts',(190.337345431519,1.08891104802307,136.916597252826));
#228087=CARTESIAN_POINT('Ctrl Pts',(190.058897807707,5.73098080836918,133.192042114338));
#228088=CARTESIAN_POINT('Ctrl Pts',(189.780450183893,5.10655917980125,127.273324325042));
#228089=CARTESIAN_POINT('Ctrl Pts',(189.502002560081,-0.210540865719208,
124.599456387862));
#228090=CARTESIAN_POINT('Ctrl Pts',(189.223554936268,-5.33416414113684,
127.627592311355));
#228091=CARTESIAN_POINT('Ctrl Pts',(188.945107312455,-5.55595115925501,
133.575023114497));
#228092=CARTESIAN_POINT('Ctrl Pts',(188.666659688642,-0.672090485321342,
136.976350437346));
#228093=CARTESIAN_POINT('Ctrl Pts',(188.388212064829,4.82938851117716,134.705920634282));
#228094=CARTESIAN_POINT('Ctrl Pts',(188.109764441016,5.89289539464864,128.850147777659));
#228095=CARTESIAN_POINT('Ctrl Pts',(187.831316817203,1.54111929438253,124.790201052305));
#228096=CARTESIAN_POINT('Ctrl Pts',(187.552869193391,-4.22687014955807,
126.256973159398));
#228097=CARTESIAN_POINT('Ctrl Pts',(187.274421569578,-6.11057242014135,
131.902572188318));
#228098=CARTESIAN_POINT('Ctrl Pts',(186.995973945765,-2.37895715467313,
136.538968434335));
#228099=CARTESIAN_POINT('Ctrl Pts',(186.717526321952,3.53880351742172,135.905540247907));
#228100=CARTESIAN_POINT('Ctrl Pts',(186.439078698139,6.20457663716883,130.584377187674));
#228101=CARTESIAN_POINT('Ctrl Pts',(186.160631074326,3.16864693777749,125.465368152723));
#228102=CARTESIAN_POINT('Ctrl Pts',(185.882183450513,-2.77911450042273,
125.25263236868));
#228103=CARTESIAN_POINT('Ctrl Pts',(185.6037358267,-6.17300548002561,130.14166362836));
#228104=CARTESIAN_POINT('Ctrl Pts',(185.325288202887,-3.89420599156785,
135.639681046572));
#228105=CARTESIAN_POINT('Ctrl Pts',(185.046840579075,1.96317856060187,136.694275209062));
#228106=CARTESIAN_POINT('Ctrl Pts',(184.768392955261,6.0164979221829,132.336325600291));
#228107=CARTESIAN_POINT('Ctrl Pts',(184.489945331449,4.54094961554151,126.570575013045));
#228108=CARTESIAN_POINT('Ctrl Pts',(184.211497707636,-1.10750955006109,
124.695466564429));
#228109=CARTESIAN_POINT('Ctrl Pts',(183.933050083823,-5.73822154400692,
128.434133314579));
#228110=CARTESIAN_POINT('Ctrl Pts',(183.65460246001,-5.09578826671723,134.350923164133));
#228111=CARTESIAN_POINT('Ctrl Pts',(183.376154836197,0.229425484589131,
137.008595292604));
#228112=CARTESIAN_POINT('Ctrl Pts',(183.097707212384,5.34380842361613,133.964878848429));
#228113=CARTESIAN_POINT('Ctrl Pts',(182.819259588571,5.54749248089459,128.016800549989));
#228114=CARTESIAN_POINT('Ctrl Pts',(182.540811964758,0.653301958305029,
124.630353773773));
#228115=CARTESIAN_POINT('Ctrl Pts',(182.262364340946,-4.84124114839195,
126.917517669999));
#228116=CARTESIAN_POINT('Ctrl Pts',(181.983916717133,-5.88692014749505,
132.776500352206));
#228117=CARTESIAN_POINT('Ctrl Pts',(181.70546909332,-1.52280712308763,136.82318296266));
#228118=CARTESIAN_POINT('Ctrl Pts',(181.427021469507,4.24069125417353,135.33886187379));
#228119=CARTESIAN_POINT('Ctrl Pts',(181.148573845694,6.10720153813428,129.687555653153));
#228120=CARTESIAN_POINT('Ctrl Pts',(180.870126221881,2.36149196193127,125.062538635854));
#228121=CARTESIAN_POINT('Ctrl Pts',(180.591678598068,-3.55431336199069,
125.713975516152));
#228122=CARTESIAN_POINT('Ctrl Pts',(180.313230974255,-6.20387834410407,
131.04322762551));
#228123=CARTESIAN_POINT('Ctrl Pts',(180.034783350442,-3.15238220429199,
136.15297262387));
#228124=CARTESIAN_POINT('Ctrl Pts',(179.75633572663,2.79599917883219,136.347604482659));
#228125=CARTESIAN_POINT('Ctrl Pts',(179.477888102817,6.17499390876314,131.448266031944));
#228126=CARTESIAN_POINT('Ctrl Pts',(179.199440479004,3.8794709017638,125.957209961944));
#228127=CARTESIAN_POINT('Ctrl Pts',(178.920992855191,-1.98109634126673,
124.920448547985));
#228128=CARTESIAN_POINT('Ctrl Pts',(178.642545231378,-6.02113282860982,
129.290714880887));
#228129=CARTESIAN_POINT('Ctrl Pts',(178.364097607565,-4.52804239515191,
135.051947700091));
#228130=CARTESIAN_POINT('Ctrl Pts',(178.085649983752,1.12609779228193,136.909855496619));
#228131=CARTESIAN_POINT('Ctrl Pts',(177.807202359939,5.74540912154417,133.157111769304));
#228132=CARTESIAN_POINT('Ctrl Pts',(177.528754736127,5.08497014694685,127.242304671825));
#228133=CARTESIAN_POINT('Ctrl Pts',(177.250307112313,-0.248307978092709,
124.600852972375));
#228134=CARTESIAN_POINT('Ctrl Pts',(176.971859488501,-5.35340320178418,
127.660121740658));
#228135=CARTESIAN_POINT('Ctrl Pts',(176.693411864688,-5.53898241132168,
133.608792432211));
#228136=CARTESIAN_POINT('Ctrl Pts',(176.414964240875,-0.634507379188621,
136.980327290216));
#228137=CARTESIAN_POINT('Ctrl Pts',(176.136516617062,4.85304893701009,134.676450488799));
#228138=CARTESIAN_POINT('Ctrl Pts',(175.858068993249,5.88089036471739,128.814312257825));
#228139=CARTESIAN_POINT('Ctrl Pts',(175.579621369436,1.50448084471559,124.780931250186));
#228140=CARTESIAN_POINT('Ctrl Pts',(175.301173745623,-4.25447307360455,
126.282787570284));
#228141=CARTESIAN_POINT('Ctrl Pts',(175.02272612181,-6.10377407984646,131.939748629711));
#228142=CARTESIAN_POINT('Ctrl Pts',(174.744278497998,-2.34400489265046,
136.553343572764));
#228143=CARTESIAN_POINT('Ctrl Pts',(174.465830874185,3.56979027988629,135.883904033421));
#228144=CARTESIAN_POINT('Ctrl Pts',(174.187383250372,6.20312257915782,130.546612244398));
#228145=CARTESIAN_POINT('Ctrl Pts',(173.908935626559,3.13608826756835,125.446178618609));
#228146=CARTESIAN_POINT('Ctrl Pts',(173.630488002746,-2.81285795548731,
125.269652488117));
#228147=CARTESIAN_POINT('Ctrl Pts',(173.352040378933,-6.17692513320066,
130.179252743065));
#228148=CARTESIAN_POINT('Ctrl Pts',(173.07359275512,-3.86469987307124,135.663296596462));
#228149=CARTESIAN_POINT('Ctrl Pts',(172.795145131307,1.99899576932572,136.682215657471));
#228150=CARTESIAN_POINT('Ctrl Pts',(172.516697507494,6.02571195608475,132.29967308599));
#228151=CARTESIAN_POINT('Ctrl Pts',(172.238249883681,4.51509322759614,126.543011406101));
#228152=CARTESIAN_POINT('Ctrl Pts',(171.959802259869,-1.14467560248665,
124.702321473066));
#228153=CARTESIAN_POINT('Ctrl Pts',(171.681354636056,-5.75254347439624,
128.469107412642));
#228154=CARTESIAN_POINT('Ctrl Pts',(171.402907012243,-5.07410492070761,
134.38187696408));
#228155=CARTESIAN_POINT('Ctrl Pts',(171.12445938843,0.267188171305193,137.007083764462));
#228156=CARTESIAN_POINT('Ctrl Pts',(170.846011764617,5.36294838675633,133.932291012718));
#228157=CARTESIAN_POINT('Ctrl Pts',(170.567564140804,5.53042102937231,127.983083035723));
#228158=CARTESIAN_POINT('Ctrl Pts',(170.289116516991,0.615706922082464,
124.62649132937));
#228159=CARTESIAN_POINT('Ctrl Pts',(170.010668893178,-4.86481176764585,
126.947059693175));
#228160=CARTESIAN_POINT('Ctrl Pts',(169.732221269365,-5.87480610217478,
132.812299166869));
#228161=CARTESIAN_POINT('Ctrl Pts',(169.453773645553,-1.48614062903852,
136.832341207004));
#228162=CARTESIAN_POINT('Ctrl Pts',(169.17532602174,4.26821548017818,135.312963568669));
#228163=CARTESIAN_POINT('Ctrl Pts',(168.896878397927,6.10029007702938,129.650400075769));
#228164=CARTESIAN_POINT('Ctrl Pts',(168.618430774114,2.32649610882855,125.048269946673));
#228165=CARTESIAN_POINT('Ctrl Pts',(168.339983150301,-3.58523412773234,
125.735705943466));
#228166=CARTESIAN_POINT('Ctrl Pts',(168.061535526488,-6.2023093493314,131.08098796821));
#228167=CARTESIAN_POINT('Ctrl Pts',(167.783087902675,-3.11976527855146,
136.172062971709));
#228168=CARTESIAN_POINT('Ctrl Pts',(167.504640278862,2.82969067421049,136.330481738588));
#228169=CARTESIAN_POINT('Ctrl Pts',(167.22619265505,6.17879913544756,131.410665161273));
#228170=CARTESIAN_POINT('Ctrl Pts',(166.947745031236,3.84989304232704,125.933684327914));
#228171=CARTESIAN_POINT('Ctrl Pts',(166.669297407424,-2.01687667896098,
124.93261705898));
#228172=CARTESIAN_POINT('Ctrl Pts',(166.39084978361,-6.03023526218728,129.327395269766));
#228173=CARTESIAN_POINT('Ctrl Pts',(166.112402159798,-4.50210223283349,
135.079432481411));
#228174=CARTESIAN_POINT('Ctrl Pts',(165.833954535985,1.16324280857304,136.902887499053));
#228175=CARTESIAN_POINT('Ctrl Pts',(165.555506912173,5.75962453647134,133.122094242209));
#228176=CARTESIAN_POINT('Ctrl Pts',(165.277059288359,5.06319268865361,127.2114170119));
#228177=CARTESIAN_POINT('Ctrl Pts',(164.998611664547,-0.286065889322858,
124.602479430144));
#228178=CARTESIAN_POINT('Ctrl Pts',(164.720164040733,-5.37244389010723,
127.692767680889));
#228179=CARTESIAN_POINT('Ctrl Pts',(164.441716416921,-5.52180841435808,
133.642457830674));
#228180=CARTESIAN_POINT('Ctrl Pts',(164.163268793108,-0.596900761151562,
136.984075290369));
#228181=CARTESIAN_POINT('Ctrl Pts',(163.884821169295,4.87652953132996,134.646836861603));
#228182=CARTESIAN_POINT('Ctrl Pts',(163.606373545482,5.86866741623098,128.778550479967));
#228183=CARTESIAN_POINT('Ctrl Pts',(163.327925921669,1.46778664595768,124.771884648456));
#228184=CARTESIAN_POINT('Ctrl Pts',(163.049478297856,-4.28191834658676,
126.308769529723));
#228185=CARTESIAN_POINT('Ctrl Pts',(162.771030674043,-6.09674956195837,
131.976882998882));
#228186=CARTESIAN_POINT('Ctrl Pts',(162.49258305023,-2.30896577266445,136.567505680515));
#228187=CARTESIAN_POINT('Ctrl Pts',(162.214135426418,3.60064476245918,135.862079594585));
#228188=CARTESIAN_POINT('Ctrl Pts',(161.935687802605,6.20143866215845,130.508856852083));
#228189=CARTESIAN_POINT('Ctrl Pts',(161.657240178792,3.10341338845521,125.427187633898));
#228190=CARTESIAN_POINT('Ctrl Pts',(161.378792554979,-2.84649717906582,
125.2868776982));
#228191=CARTESIAN_POINT('Ctrl Pts',(161.100344931166,-6.18061589814333,
130.216865021372));
#228192=CARTESIAN_POINT('Ctrl Pts',(160.821897307353,-3.83505054669964,
135.686732096692));
#228193=CARTESIAN_POINT('Ctrl Pts',(160.54344968354,2.0347389045262,136.6699382998));
#228194=CARTESIAN_POINT('Ctrl Pts',(160.265002059727,6.03470270501411,132.262965162335));
#228195=CARTESIAN_POINT('Ctrl Pts',(159.986554435914,4.48906953121078,126.51560570502));
#228196=CARTESIAN_POINT('Ctrl Pts',(159.708106812101,-1.18179923853688,
124.709402495009));
#228197=CARTESIAN_POINT('Ctrl Pts',(159.429659188289,-5.76665224217155,
128.50416804437));
#228198=CARTESIAN_POINT('Ctrl Pts',(159.151211564475,-5.05223355187421,
134.412698197843));
#228199=CARTESIAN_POINT('Ctrl Pts',(158.872763940663,0.304940957265202,
137.005342392132));
#228200=CARTESIAN_POINT('Ctrl Pts',(158.59431631685,5.38188962387183,133.899587270395));
#228201=CARTESIAN_POINT('Ctrl Pts',(158.315868693037,5.51314464606502,127.949470064936));
#228202=CARTESIAN_POINT('Ctrl Pts',(158.037421069224,0.57808907061355,124.622857808186));
#228203=CARTESIAN_POINT('Ctrl Pts',(157.758973445411,-4.88820211951067,
126.976744650055));
#228204=CARTESIAN_POINT('Ctrl Pts',(157.480525821598,-5.86247436375394,
132.848023576631));
#228205=CARTESIAN_POINT('Ctrl Pts',(157.202078197785,-1.44941906550188,
136.841276082311));
#228206=CARTESIAN_POINT('Ctrl Pts',(156.923630573973,4.29558154588865,135.286898195607));
#228207=CARTESIAN_POINT('Ctrl Pts',(156.645182950159,6.09315256743229,129.613287258817));
#228208=CARTESIAN_POINT('Ctrl Pts',(156.366735326347,2.29141404655692,125.034214551549));
#228209=CARTESIAN_POINT('Ctrl Pts',(156.088287702534,-3.61602204130483,
125.757624191644));
#228210=CARTESIAN_POINT('Ctrl Pts',(155.809840078721,-6.2005105257049,131.11873806038));
#228211=CARTESIAN_POINT('Ctrl Pts',(155.531392454908,-3.08703274876129,
136.190954417361));
#228212=CARTESIAN_POINT('Ctrl Pts',(155.252944831095,2.86327731436015,136.313154222067));
#228213=CARTESIAN_POINT('Ctrl Pts',(154.974497207282,6.18237540445775,131.373041823765));
#228214=CARTESIAN_POINT('Ctrl Pts',(154.696049583469,3.82017252368788,125.910339178587));
#228215=CARTESIAN_POINT('Ctrl Pts',(154.417601959656,-2.05258228054818,
124.945003149591));
#228216=CARTESIAN_POINT('Ctrl Pts',(154.139154335844,-6.03911424317947,
129.364130388138));
#228217=CARTESIAN_POINT('Ctrl Pts',(153.860706712031,-4.47599524346119,
135.106758848372));
#228218=CARTESIAN_POINT('Ctrl Pts',(153.582259088218,1.20034472047403,136.895693518332));
#228219=CARTESIAN_POINT('Ctrl Pts',(153.303811464405,5.77362652639317,133.086990830643));
#228220=CARTESIAN_POINT('Ctrl Pts',(153.025363840592,5.04122761189337,127.180662489822));
#228221=CARTESIAN_POINT('Ctrl Pts',(152.746916216779,-0.323813200276178,
124.604335700902));
#228222=CARTESIAN_POINT('Ctrl Pts',(152.468468592966,-5.39128550054617,
127.725528922339));
#228223=CARTESIAN_POINT('Ctrl Pts',(152.190020969154,-5.5044298047531,133.6760180624));
#228224=CARTESIAN_POINT('Ctrl Pts',(151.91157334534,-0.55927202473736,136.987594298923));
#228225=CARTESIAN_POINT('Ctrl Pts',(151.633125721528,4.89982942405471,134.617080850036));
#228226=CARTESIAN_POINT('Ctrl Pts',(151.354678097715,5.85622700211526,128.742863769248));
#228227=CARTESIAN_POINT('Ctrl Pts',(151.076230473902,1.43103805782584,124.763061582343));
#228228=CARTESIAN_POINT('Ctrl Pts',(150.797782850089,-4.3092049515099,126.334918074943));
#228229=CARTESIAN_POINT('Ctrl Pts',(150.519335226276,-6.0894991267732,132.013973919806));
#228230=CARTESIAN_POINT('Ctrl Pts',(150.240887602463,-2.27384109310269,
136.581454232806));
#228231=CARTESIAN_POINT('Ctrl Pts',(149.96243997865,3.63136582181627,135.840067740113));
#228232=CARTESIAN_POINT('Ctrl Pts',(149.683992354837,6.19952494856889,130.471112409769));
#228233=CARTESIAN_POINT('Ctrl Pts',(149.405544731024,3.0706235112177,125.40839590231));
#228234=CARTESIAN_POINT('Ctrl Pts',(149.127097107212,-2.88003092464457,
125.30430736064));
#228235=CARTESIAN_POINT('Ctrl Pts',(148.848649483398,-6.18407763809098,
130.254499069545));
#228236=CARTESIAN_POINT('Ctrl Pts',(148.570201859586,-3.80525911111971,
135.709986678852));
#228237=CARTESIAN_POINT('Ctrl Pts',(148.291754235773,2.07040664172831,136.657443590992));
#228238=CARTESIAN_POINT('Ctrl Pts',(148.01330661196,6.04346983581547,132.226203189553));
#228239=CARTESIAN_POINT('Ctrl Pts',(147.734858988147,4.46287949070312,126.488358925329));
#228240=CARTESIAN_POINT('Ctrl Pts',(147.456411364334,-1.21887908258166,
124.716709367866));
#228241=CARTESIAN_POINT('Ctrl Pts',(147.177963740522,-5.78054732452736,
128.53931391058));
#228242=CARTESIAN_POINT('Ctrl Pts',(146.899516116708,-5.03017497066859,
134.44338572333));
#228243=CARTESIAN_POINT('Ctrl Pts',(146.621068492896,0.342682443525903,
137.003371240143));
#228244=CARTESIAN_POINT('Ctrl Pts',(146.342620869082,5.40063143308812,133.866768833311));
#228245=CARTESIAN_POINT('Ctrl Pts',(146.06417324527,5.49566397115542,127.915962883168));
#228246=CARTESIAN_POINT('Ctrl Pts',(145.785725621457,0.540449797841529,
124.619453344862));
#228247=CARTESIAN_POINT('Ctrl Pts',(145.507277997644,-4.91141133724831,
127.006571440652));
#228248=CARTESIAN_POINT('Ctrl Pts',(145.228830373831,-5.84992538918966,
132.883672257711));
#228249=CARTESIAN_POINT('Ctrl Pts',(144.950382750018,-1.41264379320865,
136.849987257496));
#228250=CARTESIAN_POINT('Ctrl Pts',(144.671935126205,4.32278843724517,135.260666720466));
#228251=CARTESIAN_POINT('Ctrl Pts',(144.393487502392,6.08578927382608,129.576218577526));
#228252=CARTESIAN_POINT('Ctrl Pts',(144.11503987858,2.25624707509518,125.020372971309));
#228253=CARTESIAN_POINT('Ctrl Pts',(143.836592254767,-3.64667596185081,
125.779729448496));
#228254=CARTESIAN_POINT('Ctrl Pts',(143.558144630954,-6.19848193988065,
131.156476503179));
#228255=CARTESIAN_POINT('Ctrl Pts',(143.279697007141,-3.05418582783736,
136.209646260801));
#228256=CARTESIAN_POINT('Ctrl Pts',(143.001249383328,2.89675785471595,136.295622575173));
#228257=CARTESIAN_POINT('Ctrl Pts',(142.722801759515,6.18572258327378,131.335397413564));
#228258=CARTESIAN_POINT('Ctrl Pts',(142.444354135702,3.79031044715096,125.887175379022));
#228259=CARTESIAN_POINT('Ctrl Pts',(142.165906511889,-2.0882118229442,124.957606360848));
#228260=CARTESIAN_POINT('Ctrl Pts',(141.887458888076,-6.04776944257254,
129.400918874772));
#228261=CARTESIAN_POINT('Ctrl Pts',(141.609011264264,-4.44972239443904,
135.133925788383));
#228262=CARTESIAN_POINT('Ctrl Pts',(141.33056364045,1.2374021531599,136.888273821029));
#228263=CARTESIAN_POINT('Ctrl Pts',(141.052116016638,5.78741457246075,133.051802835376));
#228264=CARTESIAN_POINT('Ctrl Pts',(140.773668392825,5.01907573059014,127.15004224521));
#228265=CARTESIAN_POINT('Ctrl Pts',(140.495220769012,-0.361548512212229,
124.606421715863));
#228266=CARTESIAN_POINT('Ctrl Pts',(140.216773145199,-5.4099273349182,127.758404251031));
#228267=CARTESIAN_POINT('Ctrl Pts',(139.938325521386,-5.48684722647749,
133.709471883804));
#228268=CARTESIAN_POINT('Ctrl Pts',(139.659877897573,-0.521622564292735,
136.990884185479));
#228269=CARTESIAN_POINT('Ctrl Pts',(139.38143027376,4.92294775179823,134.58718355672));
#228270=CARTESIAN_POINT('Ctrl Pts',(139.102982649947,5.84356958335437,128.707253448052));
#228271=CARTESIAN_POINT('Ctrl Pts',(138.824535026135,1.39423644205237,124.754462378786));
#228272=CARTESIAN_POINT('Ctrl Pts',(138.546087402322,-4.33633187725888,
126.361232236999));
#228273=CARTESIAN_POINT('Ctrl Pts',(138.267639778509,-6.08202304295846,
132.051020018064));
#228274=CARTESIAN_POINT('Ctrl Pts',(137.989192154696,-2.23863215552307,
136.595188712768));
#228275=CARTESIAN_POINT('Ctrl Pts',(137.710744530883,3.66195231957746,135.817869285661));
#228276=CARTESIAN_POINT('Ctrl Pts',(137.43229690707,6.19738150930245,130.433380316089));
#228277=CARTESIAN_POINT('Ctrl Pts',(137.153849283257,3.03771985089675,125.389804120178));
#228278=CARTESIAN_POINT('Ctrl Pts',(136.875401659444,-2.91345794961824,
125.321940829576));
#228279=CARTESIAN_POINT('Ctrl Pts',(136.596954035631,-6.1873102247676,130.29215349304));
#228280=CARTESIAN_POINT('Ctrl Pts',(136.318506411819,-3.77532667026395,
135.733059481234));
#228281=CARTESIAN_POINT('Ctrl Pts',(136.040058788006,2.10599765925102,136.644731994041));
#228282=CARTESIAN_POINT('Ctrl Pts',(135.761611164193,6.05201302361958,132.189388529871));
#228283=CARTESIAN_POINT('Ctrl Pts',(135.48316354038,4.4365240765547,126.461272076668));
#228284=CARTESIAN_POINT('Ctrl Pts',(135.204715916567,-1.25591376061384,
124.724241820878));
#228285=CARTESIAN_POINT('Ctrl Pts',(134.926268292754,-5.79422820657625,
128.574543708929));
#228286=CARTESIAN_POINT('Ctrl Pts',(134.647820668941,-5.00792999447956,
134.473938403405));
#228287=CARTESIAN_POINT('Ctrl Pts',(134.369373045128,0.380411231562576,
137.001170381535));
#228288=CARTESIAN_POINT('Ctrl Pts',(134.090925421316,5.41917311992063,133.833836917565));
#228289=CARTESIAN_POINT('Ctrl Pts',(133.812477797503,5.4779796523963,127.88256273204));
#228290=CARTESIAN_POINT('Ctrl Pts',(133.53403017369,0.502790498503515,124.616278065551));
#228291=CARTESIAN_POINT('Ctrl Pts',(133.255582549877,-4.93443856083268,
127.036538959725));
#228292=CARTESIAN_POINT('Ctrl Pts',(132.977134926064,-5.83715964348875,
132.919243889133));
#228293=CARTESIAN_POINT('Ctrl Pts',(132.698687302251,-1.37581617488021,
136.858474409763));
#228294=CARTESIAN_POINT('Ctrl Pts',(132.420239678438,4.34983514608645,135.234270115264));
#228295=CARTESIAN_POINT('Ctrl Pts',(132.141792054625,6.07820046906025,129.539195405491));
#228296=CARTESIAN_POINT('Ctrl Pts',(131.863344430812,2.22099649756843,125.006745718858));
#228297=CARTESIAN_POINT('Ctrl Pts',(131.584896806999,-3.67719475347803,
125.802020894903));
#228298=CARTESIAN_POINT('Ctrl Pts',(131.306449183186,-6.1962236670286,131.194201898194));
#228299=CARTESIAN_POINT('Ctrl Pts',(131.028001559374,-3.02122573293442,
136.228137809392));
#228300=CARTESIAN_POINT('Ctrl Pts',(130.749553935561,2.93013105464412,136.277887447547));
#228301=CARTESIAN_POINT('Ctrl Pts',(130.471106311748,6.18884054786473,131.2977333256));
#228302=CARTESIAN_POINT('Ctrl Pts',(130.192658687935,3.76030791926647,125.864193787566));
#228303=CARTESIAN_POINT('Ctrl Pts',(129.914211064122,-2.12376398588317,
124.970426225734));
#228304=CARTESIAN_POINT('Ctrl Pts',(129.635763440309,-6.05620053964477,
129.437759366456));
#228305=CARTESIAN_POINT('Ctrl Pts',(129.357315816496,-4.42328465931731,
135.160932294765));
#228306=CARTESIAN_POINT('Ctrl Pts',(129.078868192683,1.27441373345414,136.880628682086));
#228307=CARTESIAN_POINT('Ctrl Pts',(128.800420568871,5.80098816375315,133.01653156031));
#228308=CARTESIAN_POINT('Ctrl Pts',(128.521972945058,4.99673786558976,127.11955741271));
#228309=CARTESIAN_POINT('Ctrl Pts',(128.243525321245,-0.399270426835251,
124.608737397728));
#228310=CARTESIAN_POINT('Ctrl Pts',(127.965077697432,-5.42836870244348,
127.791392448756));
#228311=CARTESIAN_POINT('Ctrl Pts',(127.686630073619,-5.46906133106002,
133.742818055242));
#228312=CARTESIAN_POINT('Ctrl Pts',(127.408182449806,-0.483953774931917,
136.993944828129));
#228313=CARTESIAN_POINT('Ctrl Pts',(127.129734825993,4.9458836579024,134.557146089508));
#228314=CARTESIAN_POINT('Ctrl Pts',(126.85128720218,5.8306956289736,128.671720835934));
#228315=CARTESIAN_POINT('Ctrl Pts',(126.572839578367,1.35738316233494,124.746087356435));
#228316=CARTESIAN_POINT('Ctrl Pts',(126.294391954555,-4.36329811863544,
126.387711040812));
#228317=CARTESIAN_POINT('Ctrl Pts',(126.015944330741,-6.07432158754323,
132.088019920899));
#228318=CARTESIAN_POINT('Ctrl Pts',(125.737496706929,-2.20334026460562,
136.608708611466));
#228319=CARTESIAN_POINT('Ctrl Pts',(125.459049083116,3.69240312234872,135.795485053802));
#228320=CARTESIAN_POINT('Ctrl Pts',(125.180601459303,6.19500842378515,130.39566196922));
#228321=CARTESIAN_POINT('Ctrl Pts',(124.90215383549,3.00470362674961,125.371412976429));
#228322=CARTESIAN_POINT('Ctrl Pts',(124.623706211677,-2.9467770153362,125.339777451594));
#228323=CARTESIAN_POINT('Ctrl Pts',(124.345258587864,-6.19031353838844,
130.329826896558));
#228324=CARTESIAN_POINT('Ctrl Pts',(124.066810964051,-3.74525433329013,
135.755949648866));
#228325=CARTESIAN_POINT('Ctrl Pts',(123.788363340238,2.14151063825588,136.631803979981));
#228326=CARTESIAN_POINT('Ctrl Pts',(123.509915716426,6.0603319518555,132.152522547471));
#228327=CARTESIAN_POINT('Ctrl Pts',(123.231468092613,4.4100042653751,126.43434616275));
#228328=CARTESIAN_POINT('Ctrl Pts',(122.9530204688,-1.29290190029971,124.731999574929));
#228329=CARTESIAN_POINT('Ctrl Pts',(122.674572844987,-5.80769438136815,
128.609856133963));
#228330=CARTESIAN_POINT('Ctrl Pts',(122.396125221174,-4.98549944760296,
134.504355105923));
#228331=CARTESIAN_POINT('Ctrl Pts',(122.117677597361,0.418125923321227,
136.998739897863));
#228332=CARTESIAN_POINT('Ctrl Pts',(121.839229973548,5.43751399730024,133.80079274346));
#228333=CARTESIAN_POINT('Ctrl Pts',(121.560782349735,5.46009234508668,127.849270849208));
#228334=CARTESIAN_POINT('Ctrl Pts',(121.282334725922,0.465112568078527,
124.613332087916));
#228335=CARTESIAN_POINT('Ctrl Pts',(121.00388710211,-4.95728293698158,127.066646096814));
#228336=CARTESIAN_POINT('Ctrl Pts',(120.725439478297,-5.82417759969065,
132.954737152777));
#228337=CARTESIAN_POINT('Ctrl Pts',(120.446991854484,-1.33893757517749,
136.866737224615));
#228338=CARTESIAN_POINT('Ctrl Pts',(120.168544230671,4.37672067018674,135.207709358136));
#228339=CARTESIAN_POINT('Ctrl Pts',(119.890096606858,6.07038643434081,129.502219114618));
#228340=CARTESIAN_POINT('Ctrl Pts',(119.611648983045,2.18566362019961,124.993333299159));
#228341=CARTESIAN_POINT('Ctrl Pts',(119.333201359232,-3.7075772853013,125.82449770485));
#228342=CARTESIAN_POINT('Ctrl Pts',(119.054753735419,-6.19373579082994,
131.231912847497));
#228343=CARTESIAN_POINT('Ctrl Pts',(118.776306111606,-2.98815368540088,
136.246428377926));
#228344=CARTESIAN_POINT('Ctrl Pts',(118.497858487794,2.96339567748857,136.259949496373));
#228345=CARTESIAN_POINT('Ctrl Pts',(118.219410863981,6.1917291826932,131.26005095553));
#228346=CARTESIAN_POINT('Ctrl Pts',(117.940963240168,3.73016605178927,125.841395255808));
#228347=CARTESIAN_POINT('Ctrl Pts',(117.662515616355,-2.15923745196658,
124.983462269205));
#228348=CARTESIAN_POINT('Ctrl Pts',(117.384067992542,-6.06440722197891,
129.474650498052));
#228349=CARTESIAN_POINT('Ctrl Pts',(117.105620368729,-4.39668301775581,
135.187777366781));
#228350=CARTESIAN_POINT('Ctrl Pts',(116.827172744916,1.31137808987868,136.872758384795));
#228351=CARTESIAN_POINT('Ctrl Pts',(116.548725121103,5.81434679729579,132.981178312436));
#228352=CARTESIAN_POINT('Ctrl Pts',(116.27027749729,4.97421484463032,127.089209121948));
#228353=CARTESIAN_POINT('Ctrl Pts',(115.991829873478,-0.436977546345769,
124.611282660692));
#228354=CARTESIAN_POINT('Ctrl Pts',(115.713382249665,-5.44660891977013,
127.824492293124));
#228355=CARTESIAN_POINT('Ctrl Pts',(115.434934625852,-5.45107277756375,
133.776055341058));
#228356=CARTESIAN_POINT('Ctrl Pts',(115.156487002039,-0.446267052485976,
136.99677611346));
#228357=CARTESIAN_POINT('Ctrl Pts',(114.878039378226,4.9686362924688,134.526969561451));
#228358=CARTESIAN_POINT('Ctrl Pts',(114.599591754413,5.81760561602206,128.636267249567));
#228359=CARTESIAN_POINT('Ctrl Pts',(114.3211441306,1.32047958428524,124.737936825626));
#228360=CARTESIAN_POINT('Ctrl Pts',(114.042696506787,-4.39010267639563,
126.414353505198));
#228361=CARTESIAN_POINT('Ctrl Pts',(113.764248882975,-6.06639504590774,
132.124972257267));
#228362=CARTESIAN_POINT('Ctrl Pts',(113.485801259161,-2.16796672810439,
136.622013427915));
#228363=CARTESIAN_POINT('Ctrl Pts',(113.207353635349,3.72271710176439,135.772915873991));
#228364=CARTESIAN_POINT('Ctrl Pts',(112.928906011536,6.19240577995249,130.357958766832));
#228365=CARTESIAN_POINT('Ctrl Pts',(112.650458387723,2.97157606220462,125.353223152553));
#228366=CARTESIAN_POINT('Ctrl Pts',(112.37201076391,-2.9799868871482,125.357816565752));
#228367=CARTESIAN_POINT('Ctrl Pts',(112.093563140097,-6.19308746766462,
130.367517884098));
#228368=CARTESIAN_POINT('Ctrl Pts',(111.815115516284,-3.71504321453968,
135.778656333547));
#228369=CARTESIAN_POINT('Ctrl Pts',(111.536667892471,2.1769442627965,136.618660027865));
#228370=CARTESIAN_POINT('Ctrl Pts',(111.258220268658,6.06842631226225,132.115606608435));
#228371=CARTESIAN_POINT('Ctrl Pts',(110.979772644846,4.38332103986566,126.407582181323));
#228372=CARTESIAN_POINT('Ctrl Pts',(110.701325021032,-1.32984213103019,
124.739982342551));
#228373=CARTESIAN_POINT('Ctrl Pts',(110.42287739722,-5.82094534990898,128.645249877167));
#228374=CARTESIAN_POINT('Ctrl Pts',(110.144429773407,-4.96288416121089,
134.534634703787));
#228375=CARTESIAN_POINT('Ctrl Pts',(109.865982149594,0.455825121270016,
136.996079879188));
#228376=CARTESIAN_POINT('Ctrl Pts',(109.587534525781,5.45565338559904,133.767637535461));
#228377=CARTESIAN_POINT('Ctrl Pts',(109.309086901968,5.44200271204727,127.816088468313));
#228378=CARTESIAN_POINT('Ctrl Pts',(109.030639278155,0.427417402736423,
124.610615521118));
#228379=CARTESIAN_POINT('Ctrl Pts',(108.752191654342,-4.97994361918818,
127.096891736289));
#228380=CARTESIAN_POINT('Ctrl Pts',(108.473744030529,-5.81097973884976,
132.990150733429));
#228381=CARTESIAN_POINT('Ctrl Pts',(108.195296406717,-1.30200936065053,
136.874775395874));
#228382=CARTESIAN_POINT('Ctrl Pts',(107.916848782904,4.40344401329306,135.180985433302));
#228383=CARTESIAN_POINT('Ctrl Pts',(107.638401159091,6.06234745921968,129.465291075077));
#228384=CARTESIAN_POINT('Ctrl Pts',(107.359953535278,2.15024975226158,124.980136209215));
#228385=CARTESIAN_POINT('Ctrl Pts',(107.081505911465,-3.73782243148481,
125.847159045447));
#228386=CARTESIAN_POINT('Ctrl Pts',(106.803058287652,-6.19101840347381,
131.269607953695));
#228387=CARTESIAN_POINT('Ctrl Pts',(106.524610663839,-2.95497091073364,
136.264517288637));
#228388=CARTESIAN_POINT('Ctrl Pts',(106.246163040026,2.99655049061638,136.241809386346));
#228389=CARTESIAN_POINT('Ctrl Pts',(105.967715416213,6.1943883807198,131.222351699685));
#228390=CARTESIAN_POINT('Ctrl Pts',(105.689267792401,3.69988596163724,125.818780628557));
#228391=CARTESIAN_POINT('Ctrl Pts',(105.410820168588,-2.19463090671215,
124.996714008204));
#228392=CARTESIAN_POINT('Ctrl Pts',(105.132372544775,-6.07238918547325,
129.511590902545));
#228393=CARTESIAN_POINT('Ctrl Pts',(104.853924920962,-4.36991845548819,
135.214460009678));
#228394=CARTESIAN_POINT('Ctrl Pts',(104.575477297149,1.34829385270585,136.864663220793));
#228395=CARTESIAN_POINT('Ctrl Pts',(104.297029673336,5.82748997807964,132.945744401783));
#228396=CARTESIAN_POINT('Ctrl Pts',(104.018582049523,4.95150750231056,127.058998497491));
#228397=CARTESIAN_POINT('Ctrl Pts',(103.74013442571,-0.474668473492613,
124.614057410436));
#228398=CARTESIAN_POINT('Ctrl Pts',(103.461686801897,-5.46464731100027,
127.857702557609));
#228399=CARTESIAN_POINT('Ctrl Pts',(103.183239178085,-5.43288223256107,
133.809182509633));
#228400=CARTESIAN_POINT('Ctrl Pts',(102.904791554272,-0.408563793450433,
136.999377936557));
#228401=CARTESIAN_POINT('Ctrl Pts',(102.626343930459,4.99120481239017,134.496655090749));
#228402=CARTESIAN_POINT('Ctrl Pts',(102.347896306646,5.80430002955499,128.600894002697));
#228403=CARTESIAN_POINT('Ctrl Pts',(102.069448682833,1.28352707537895,124.730011088381));
#228404=CARTESIAN_POINT('Ctrl Pts',(101.79100105902,-4.41674455728669,126.441158642913));
#228405=CARTESIAN_POINT('Ctrl Pts',(101.512553435207,-6.05824371177293,
132.161875657885));
#228406=CARTESIAN_POINT('Ctrl Pts',(101.234105811394,-2.13251285679878,
136.635102669099));
#228407=CARTESIAN_POINT('Ctrl Pts',(100.955658187581,3.75289313452884,135.750162582539));
#228408=CARTESIAN_POINT('Ctrl Pts',(100.677210563769,6.18957367424645,130.320272106026));
#228409=CARTESIAN_POINT('Ctrl Pts',(100.398762939956,2.93833838481571,125.33523532258));
#228410=CARTESIAN_POINT('Ctrl Pts',(100.120315316143,-3.01308633445025,
125.376057503601));
#228411=CARTESIAN_POINT('Ctrl Pts',(99.8418676923298,-6.19563190980719,
130.405225059005));
#228412=CARTESIAN_POINT('Ctrl Pts',(99.5634200685172,-3.68469443349671,
135.801178693871));
#228413=CARTESIAN_POINT('Ctrl Pts',(99.2849724447041,2.2122972198669,136.605300624745));
#228414=CARTESIAN_POINT('Ctrl Pts',(99.0065248208913,6.07629580490035,132.078642080696));
#228415=CARTESIAN_POINT('Ctrl Pts',(98.7280771970783,4.35647538878314,126.380981124141));
#228416=CARTESIAN_POINT('Ctrl Pts',(98.4496295732656,-1.36673308397146,
124.748189827941));
#228417=CARTESIAN_POINT('Ctrl Pts',(98.1711819494526,-5.8339806211792,128.680723627015));
#228418=CARTESIAN_POINT('Ctrl Pts',(97.8927343256397,-4.94008497332115,
134.564776074971));
#228419=CARTESIAN_POINT('Ctrl Pts',(97.6142867018267,0.493507428451318,
136.993190424079));
#228420=CARTESIAN_POINT('Ctrl Pts',(97.3358390780141,5.47359061265531,133.734372522146));
#228421=CARTESIAN_POINT('Ctrl Pts',(97.0573914542009,5.42371142359607,127.783016818942));
#228422=CARTESIAN_POINT('Ctrl Pts',(96.7789438303882,0.389706399285272,
124.608128465823));
#228423=CARTESIAN_POINT('Ctrl Pts',(96.5004962065753,-5.0024197677526,127.127274757387));
#228424=CARTESIAN_POINT('Ctrl Pts',(96.2220485827623,-5.79756655001767,
133.025483318824));
#228425=CARTESIAN_POINT('Ctrl Pts',(95.9436009589496,-1.26503289968789,
136.882588625681));
#228426=CARTESIAN_POINT('Ctrl Pts',(95.6651533351365,4.4300041851621,135.154099331026));
#228427=CARTESIAN_POINT('Ctrl Pts',(95.3867057113237,6.05408384158403,129.428412655251));
#228428=CARTESIAN_POINT('Ctrl Pts',(95.1082580875108,2.11475620602821,124.967154938047));
#228429=CARTESIAN_POINT('Ctrl Pts',(94.8298104636979,-3.76792907128354,
125.870004076972));
#228430=CARTESIAN_POINT('Ctrl Pts',(94.5513628398851,-6.18807160565406,
131.307285819983));
#228431=CARTESIAN_POINT('Ctrl Pts',(94.2729152160721,-2.92167863853249,
136.282403871234));
#228432=CARTESIAN_POINT('Ctrl Pts',(93.9944675922592,3.02959426546386,136.223467789656));
#228433=CARTESIAN_POINT('Ctrl Pts',(93.7160199684464,6.19681804340696,131.184636955029));
#228434=CARTESIAN_POINT('Ctrl Pts',(93.4375723446334,3.66946877085029,125.796350743805));
#228435=CARTESIAN_POINT('Ctrl Pts',(93.1591247208205,-2.22994303860241,
125.010180951684));
#228436=CARTESIAN_POINT('Ctrl Pts',(92.8806770970077,-6.08014613435319,
129.548579211095));
#228437=CARTESIAN_POINT('Ctrl Pts',(92.6022294731947,-4.3429919642852,135.24097923472));
#228438=CARTESIAN_POINT('Ctrl Pts',(92.323781849382,1.38515965400848,136.856343490049));
#228439=CARTESIAN_POINT('Ctrl Pts',(92.045334225569,5.84041721907928,132.910231141365));
#228440=CARTESIAN_POINT('Ctrl Pts',(91.7668866017561,4.9286166800594,127.028926658805));
#228441=CARTESIAN_POINT('Ctrl Pts',(91.4884389779432,-0.512341811624615,
124.617061544141));
#228442=CARTESIAN_POINT('Ctrl Pts',(91.2099913541303,-5.48248320771468,
127.891022011592));
#228443=CARTESIAN_POINT('Ctrl Pts',(90.9315437303175,-5.41449037010934,
133.842198333429));
#228444=CARTESIAN_POINT('Ctrl Pts',(90.6530961065044,-0.370845394933272,
137.00175020101));
#228445=CARTESIAN_POINT('Ctrl Pts',(90.3746484826917,5.01358838138169,134.466203800718));
#228446=CARTESIAN_POINT('Ctrl Pts',(90.0962008588786,5.79077936261581,128.565602406094));
#228447=CARTESIAN_POINT('Ctrl Pts',(89.817753235066,1.24652700490487,124.722310438393));
#228448=CARTESIAN_POINT('Ctrl Pts',(89.5393056112528,-4.44322277408392,
126.468125460682));
#228449=CARTESIAN_POINT('Ctrl Pts',(89.2608579874402,-6.04986788718945,
132.198728755283));
#228450=CARTESIAN_POINT('Ctrl Pts',(88.9824103636271,-2.09697996444503,
136.647975849991));
#228451=CARTESIAN_POINT('Ctrl Pts',(88.7039627398144,3.78293010245805,135.727226022576));
#228452=CARTESIAN_POINT('Ctrl Pts',(88.4255151160013,6.18651221161165,130.282603383299));
#228453=CARTESIAN_POINT('Ctrl Pts',(88.1470674921886,2.9049918262175,125.317450153056));
#228454=CARTESIAN_POINT('Ctrl Pts',(87.8686198683756,-3.04607413073006,
125.394499589218));
#228455=CARTESIAN_POINT('Ctrl Pts',(87.5901722445627,-6.19794677053091,
130.442947024027));
#228456=CARTESIAN_POINT('Ctrl Pts',(87.3117246207499,-3.65420911474647,
135.823515895262));
#228457=CARTESIAN_POINT('Ctrl Pts',(87.033276996937,2.24756819945024,136.59172626566));
#228458=CARTESIAN_POINT('Ctrl Pts',(86.754829373124,6.08394013816284,132.041630333989));
#228459=CARTESIAN_POINT('Ctrl Pts',(86.4763817493112,4.32946830690299,126.35454397691));
#228460=CARTESIAN_POINT('Ctrl Pts',(86.1979341254982,-1.40357339211569,
124.756621726966));
#228461=CARTESIAN_POINT('Ctrl Pts',(85.9194865016854,-5.84679971215209,
128.716276069012));
#228462=CARTESIAN_POINT('Ctrl Pts',(85.6410388778725,-4.91710272876601,
134.594778102578));
#228463=CARTESIAN_POINT('Ctrl Pts',(85.3625912540596,0.531171448533366,
136.990071639606));
#228464=CARTESIAN_POINT('Ctrl Pts',(85.0841436302467,5.49132501379855,133.700998936161));
#228465=CARTESIAN_POINT('Ctrl Pts',(84.8056960064338,5.4052191575235,127.750057126576));
#228466=CARTESIAN_POINT('Ctrl Pts',(84.527248382621,0.351980955120191,124.60587101419));
#228467=CARTESIAN_POINT('Ctrl Pts',(84.2488007588079,-5.02471054981291,
127.157794034254));
#228468=CARTESIAN_POINT('Ctrl Pts',(83.9703531349953,-5.78393853022499,
133.0607335997));
#228469=CARTESIAN_POINT('Ctrl Pts',(83.6919055111822,-1.22800956246596,
136.890176624513));
#228470=CARTESIAN_POINT('Ctrl Pts',(83.4134578873695,4.45640020159694,135.127052047582));
#228471=CARTESIAN_POINT('Ctrl Pts',(83.1350102635564,6.04559588764522,129.391585221682));
#228472=CARTESIAN_POINT('Ctrl Pts',(82.8565626397436,2.07918429672594,124.954389966684));
#228473=CARTESIAN_POINT('Ctrl Pts',(82.5781150159307,-3.79789608908488,
125.893031952893));
#228474=CARTESIAN_POINT('Ctrl Pts',(82.2996673921181,-6.18489550656524,
131.344945050191));
#228475=CARTESIAN_POINT('Ctrl Pts',(82.0212197683047,-2.88827810245507,
136.300087462925));
#228476=CARTESIAN_POINT('Ctrl Pts',(81.7427721444922,3.06252577758164,136.204925385956));
#228477=CARTESIAN_POINT('Ctrl Pts',(81.464324520679,6.19901808072266,131.146908119091));
#228478=CARTESIAN_POINT('Ctrl Pts',(81.1858768968663,3.6389156065486,125.774106432701));
#228479=CARTESIAN_POINT('Ctrl Pts',(80.9074292730533,-2.26517253913331,
125.023862600622));
#228480=CARTESIAN_POINT('Ctrl Pts',(80.6289816492404,-6.08767778118217,
129.585614053086));
#228481=CARTESIAN_POINT('Ctrl Pts',(80.3505340254275,-4.31590454191782,
135.267334059228));
#228482=CARTESIAN_POINT('Ctrl Pts',(80.0720864016147,1.42197412771073,136.847799500855));
#228483=CARTESIAN_POINT('Ctrl Pts',(79.7936387778018,5.85312804127117,132.874639847142));
#228484=CARTESIAN_POINT('Ctrl Pts',(79.5151911539889,4.90554322610457,126.998994720211));
#228485=CARTESIAN_POINT('Ctrl Pts',(79.236743530176,-0.54999616474248,124.62029495049));
#228486=CARTESIAN_POINT('Ctrl Pts',(78.9582959063631,-5.50011594899764,
127.924449420408));
#228487=CARTESIAN_POINT('Ctrl Pts',(78.6798482825503,-5.39589787172579,
133.87510158903));
#228488=CARTESIAN_POINT('Ctrl Pts',(78.4014006587372,-0.333113254603616,
137.003892818912));
#228489=CARTESIAN_POINT('Ctrl Pts',(78.1229530349246,5.035786170012,134.435616819741));
#228490=CARTESIAN_POINT('Ctrl Pts',(77.8445054111114,5.77704411621779,128.530393767498));
#228491=CARTESIAN_POINT('Ctrl Pts',(77.5660577872988,1.20948074391421,124.71483516101));
#228492=CARTESIAN_POINT('Ctrl Pts',(77.2876101634857,-4.46953634562727,
126.49525295924));
#228493=CARTESIAN_POINT('Ctrl Pts',(77.009162539673,-6.04126788252658,132.235530183857));
#228494=CARTESIAN_POINT('Ctrl Pts',(76.73071491586,-2.06136936772754,136.660632493573));
#228495=CARTESIAN_POINT('Ctrl Pts',(76.4522672920471,3.81282689252116,135.704107044024));
#228496=CARTESIAN_POINT('Ctrl Pts',(76.1738196682342,6.18322150549176,130.244953994479));
#228497=CARTESIAN_POINT('Ctrl Pts',(75.8953720444213,2.87153762207887,125.299868303017));
#228498=CARTESIAN_POINT('Ctrl Pts',(75.6169244206085,-3.07894905361277,
125.413142139227));
#228499=CARTESIAN_POINT('Ctrl Pts',(75.3384767967955,-6.20003196405775,
130.480682381363));
#228500=CARTESIAN_POINT('Ctrl Pts',(75.0600291729826,-3.62358838793365,
135.84566711001));
#228501=CARTESIAN_POINT('Ctrl Pts',(74.7815815491698,2.28275589456742,136.577937453613));
#228502=CARTESIAN_POINT('Ctrl Pts',(74.5031339253568,6.09135902878616,132.004572739798));
#228503=CARTESIAN_POINT('Ctrl Pts',(74.224686301544,4.30230079498258,126.328271719272));
#228504=CARTESIAN_POINT('Ctrl Pts',(73.946238677731,-1.44036169033171,124.76527772718));
#228505=CARTESIAN_POINT('Ctrl Pts',(73.6677910539182,-5.85940214781156,
128.75190588575));
#228506=CARTESIAN_POINT('Ctrl Pts',(73.3893434301052,-4.89393827916089,
134.624639674871));
#228507=CARTESIAN_POINT('Ctrl Pts',(73.1108958062924,0.56881578586215,136.986723641335));
#228508=CARTESIAN_POINT('Ctrl Pts',(72.8324481824796,5.50885593187395,133.66751801418));
#228509=CARTESIAN_POINT('Ctrl Pts',(72.5540005586665,5.38652659906729,127.717210612549));
#228510=CARTESIAN_POINT('Ctrl Pts',(72.2755529348538,0.314242468171368,
124.603843249867));
#228511=CARTESIAN_POINT('Ctrl Pts',(71.9971053110409,-5.04681513937595,
127.188448435987));
#228512=CARTESIAN_POINT('Ctrl Pts',(71.7186576872279,-5.77009618446306,
133.095900269846));
#228513=CARTESIAN_POINT('Ctrl Pts',(71.4402100634152,-1.19094072089807,
136.897539111196));
#228514=CARTESIAN_POINT('Ctrl Pts',(71.1617624396021,4.48263108448347,135.099844585217));
#228515=CARTESIAN_POINT('Ctrl Pts',(70.8833148157894,6.03688391192757,129.354810139024));
#228516=CARTESIAN_POINT('Ctrl Pts',(70.6048671919763,2.04353534248492,124.941841768133));
#228517=CARTESIAN_POINT('Ctrl Pts',(70.3264195681636,-3.82772237444985,
125.916241819903));
#228518=CARTESIAN_POINT('Ctrl Pts',(70.0479719443506,-6.18149022389895,
131.382584248845));
#228519=CARTESIAN_POINT('Ctrl Pts',(69.7695243205378,-2.85477054017052,
136.317567408437));
#228520=CARTESIAN_POINT('Ctrl Pts',(69.4910766967249,3.09534380668036,136.186182862342));
#228521=CARTESIAN_POINT('Ctrl Pts',(69.2126290729119,6.20098841114368,131.109166589932));
#228522=CARTESIAN_POINT('Ctrl Pts',(68.934181449099,3.60822760089105,125.752048519516));
#228523=CARTESIAN_POINT('Ctrl Pts',(68.6557338252862,-2.30031810286251,
125.037758448041));
#228524=CARTESIAN_POINT('Ctrl Pts',(68.3772862014732,-6.09498384687224,
129.622694056181));
#228525=CARTESIAN_POINT('Ctrl Pts',(68.0988385776604,-4.28865719212064,
135.293523506613));
#228526=CARTESIAN_POINT('Ctrl Pts',(67.8203909538475,1.45873590963839,136.83903156981));
#228527=CARTESIAN_POINT('Ctrl Pts',(67.5419433300346,5.86562197365073,132.83897183796));
#228528=CARTESIAN_POINT('Ctrl Pts',(67.2634957062218,4.88228799544191,126.969203790852));
#228529=CARTESIAN_POINT('Ctrl Pts',(66.9850480824087,-0.587630137549865,
124.623757509667));
#228530=CARTESIAN_POINT('Ctrl Pts',(66.706600458596,-5.51754488146136,127.957983545393));
#228531=CARTESIAN_POINT('Ctrl Pts',(66.428152834783,-5.37710542636232,133.907891057196));
#228532=CARTESIAN_POINT('Ctrl Pts',(66.1497052109702,-0.295368770640213,
137.00580571087));
#228533=CARTESIAN_POINT('Ctrl Pts',(65.8712575871573,5.05779735573374,134.404895281231));
#228534=CARTESIAN_POINT('Ctrl Pts',(65.5928099633443,5.76309479932555,128.495269391582));
#228535=CARTESIAN_POINT('Ctrl Pts',(65.3143623395316,1.17238966517029,124.707585533234));
#228536=CARTESIAN_POINT('Ctrl Pts',(65.0359147157185,-4.49568429685739,
126.522540133366));
#228537=CARTESIAN_POINT('Ctrl Pts',(64.7574670919057,-6.03244401646077,
132.272278579917));
#228538=CARTESIAN_POINT('Ctrl Pts',(64.4790194680927,-2.02568238621027,
136.673072130848));
#228539=CARTESIAN_POINT('Ctrl Pts',(64.20057184428,3.84258239688126,135.680806503568));
#228540=CARTESIAN_POINT('Ctrl Pts',(63.922124220467,6.17970167782515,130.207325334677));
#228541=CARTESIAN_POINT('Ctrl Pts',(63.6436765966542,2.8379770120581,125.282490423967));
#228542=CARTESIAN_POINT('Ctrl Pts',(63.3652289728412,-3.11170988490585,
125.431984462817));
#228543=CARTESIAN_POINT('Ctrl Pts',(63.0867813490283,-6.20188741312008,
130.518429732716));
#228544=CARTESIAN_POINT('Ctrl Pts',(62.8083337252156,-3.59283338772076,
135.86763151729));
#228545=CARTESIAN_POINT('Ctrl Pts',(62.5298861014024,2.31785900132509,136.563934699553));
#228546=CARTESIAN_POINT('Ctrl Pts',(62.2514384775899,6.09855220186056,131.967470671305));
#228547=CARTESIAN_POINT('Ctrl Pts',(61.9729908537767,4.27497385972414,126.302165324755));
#228548=CARTESIAN_POINT('Ctrl Pts',(61.6945432299639,-1.47709661541541,
124.774157507831));
#228549=CARTESIAN_POINT('Ctrl Pts',(61.416095606151,-5.87178746116934,128.787611756953));
#228550=CARTESIAN_POINT('Ctrl Pts',(61.1376479823382,-4.8705924828735,134.65435968532));
#228551=CARTESIAN_POINT('Ctrl Pts',(60.8592003585251,0.606439045512412,
136.983146553331));
#228552=CARTESIAN_POINT('Ctrl Pts',(60.5807527347125,5.52618271726667,133.633930996847));
#228553=CARTESIAN_POINT('Ctrl Pts',(60.3023051108993,5.36763444088732,127.684478494003));
#228554=CARTESIAN_POINT('Ctrl Pts',(60.0238574870866,0.276492336852797,
124.602045247997));
#228555=CARTESIAN_POINT('Ctrl Pts',(59.7454098632736,-5.06873271734795,
127.219236826675));
#228556=CARTESIAN_POINT('Ctrl Pts',(59.4669622394608,-5.75604002566515,
133.130982026147));
#228557=CARTESIAN_POINT('Ctrl Pts',(59.1885146156479,-1.15382774858414,
136.904675812908));
#228558=CARTESIAN_POINT('Ctrl Pts',(58.9100669918351,4.50869586182645,135.072477952114));
#228559=CARTESIAN_POINT('Ctrl Pts',(58.6316193680221,6.02794823725661,129.318088769994));
#228560=CARTESIAN_POINT('Ctrl Pts',(58.3531717442092,2.00781066429043,124.929510807376));
#228561=CARTESIAN_POINT('Ctrl Pts',(58.0747241203963,-3.85740682215468,
125.939632817953));
#228562=CARTESIAN_POINT('Ctrl Pts',(57.7962764965834,-6.17785588383907,
131.42020202121));
#228563=CARTESIAN_POINT('Ctrl Pts',(57.5178288727705,-2.82115719331391,
136.334843060042));
#228564=CARTESIAN_POINT('Ctrl Pts',(57.2393812489577,3.12804713667602,136.167240913326));
#228565=CARTESIAN_POINT('Ctrl Pts',(56.9609336251447,6.20272896165862,131.071413766074));
#228566=CARTESIAN_POINT('Ctrl Pts',(56.6824860013319,3.57740589103289,125.730177821614));
#228567=CARTESIAN_POINT('Ctrl Pts',(56.404038377519,-2.33537842745856,125.051867979023));
#228568=CARTESIAN_POINT('Ctrl Pts',(56.125590753706,-6.10206406069443,129.659817846364));
#228569=CARTESIAN_POINT('Ctrl Pts',(55.8471431298932,-4.26125092455389,
135.319546606417));
#228570=CARTESIAN_POINT('Ctrl Pts',(55.5686955060803,1.49544363757083,136.830040021814));
#228571=CARTESIAN_POINT('Ctrl Pts',(55.2902478822675,5.87789855325116,132.80322843551));
#228572=CARTESIAN_POINT('Ctrl Pts',(55.0118002584545,4.85885184980179,126.939554974638));
#228573=CARTESIAN_POINT('Ctrl Pts',(54.7333526346416,-0.625242335506623,
124.627449093364));
#228574=CARTESIAN_POINT('Ctrl Pts',(54.4549050108287,-5.53476935927053,
127.991623143927));
#228575=CARTESIAN_POINT('Ctrl Pts',(54.1764573870159,-5.35811373037978,
133.9405655229));
#228576=CARTESIAN_POINT('Ctrl Pts',(53.8980097632029,-0.257613341678002,
137.007488805997));
#228577=CARTESIAN_POINT('Ctrl Pts',(53.61956213939,5.07962112291461,134.374040323585));
#228578=CARTESIAN_POINT('Ctrl Pts',(53.3411145155772,5.74893192883615,128.460230579889));
#228579=CARTESIAN_POINT('Ctrl Pts',(53.0626668917642,1.13525514309568,124.7005618237));
#228580=CARTESIAN_POINT('Ctrl Pts',(52.7842192679514,-4.52166565885288,
126.549985971924));
#228581=CARTESIAN_POINT('Ctrl Pts',(52.5057716441385,-6.0233966159634,132.308972581737));
#228582=CARTESIAN_POINT('Ctrl Pts',(52.2273240203255,-1.98992034228702,
136.685294300858));
#228583=CARTESIAN_POINT('Ctrl Pts',(51.9488763965128,3.87219551293788,135.657325264614));
#228584=CARTESIAN_POINT('Ctrl Pts',(51.6704287726998,6.17595285904027,130.169718798237));
#228585=CARTESIAN_POINT('Ctrl Pts',(51.391981148887,2.80431123975502,125.265317159845));
#228586=CARTESIAN_POINT('Ctrl Pts',(51.113533525074,-3.14435541064497,125.451025861782));
#228587=CARTESIAN_POINT('Ctrl Pts',(50.8350859012611,-6.20351304896362,
130.556187679343));
#228588=CARTESIAN_POINT('Ctrl Pts',(50.5566382774483,-3.5619452537452,135.889408303207));
#228589=CARTESIAN_POINT('Ctrl Pts',(50.2781906536353,2.35287621896542,136.549718522358));
#228590=CARTESIAN_POINT('Ctrl Pts',(49.9997430298226,6.10551939084041,131.930325503341));
#228591=CARTESIAN_POINT('Ctrl Pts',(49.7212954060095,4.2474885137371,126.27622576074));
#228592=CARTESIAN_POINT('Ctrl Pts',(49.4428477821967,-1.51377680614101,
124.783260739875));
#228593=CARTESIAN_POINT('Ctrl Pts',(49.1644001583838,-5.88395519328364,
128.823392359526));
#228594=CARTESIAN_POINT('Ctrl Pts',(48.8859525345709,-4.84706620499019,
134.683937032636));
#228595=CARTESIAN_POINT('Ctrl Pts',(48.607504910758,0.644039833341117,136.97934050814));
#228596=CARTESIAN_POINT('Ctrl Pts',(48.3290572869451,5.54330472792681,133.600239128744));
#228597=CARTESIAN_POINT('Ctrl Pts',(48.0506096631323,5.34854338303893,127.651861983834));
#228598=CARTESIAN_POINT('Ctrl Pts',(47.7721620393193,0.23873196000854,124.600477075203));
#228599=CARTESIAN_POINT('Ctrl Pts',(47.4937144155065,-5.09046247156518,
127.250158065443));
#228600=CARTESIAN_POINT('Ctrl Pts',(47.2152667916935,-5.74177057468722,
133.165977568637));
#228601=CARTESIAN_POINT('Ctrl Pts',(46.9368191678807,-1.11667202075834,
136.911586465198));
#228602=CARTESIAN_POINT('Ctrl Pts',(46.6583715440677,4.53459356778643,135.044953162355));
#228603=CARTESIAN_POINT('Ctrl Pts',(46.379923920255,6.01878919474683,129.281422475313));
#228604=CARTESIAN_POINT('Ctrl Pts',(46.101476296442,1.97201158593325,124.917397541337));
#228605=CARTESIAN_POINT('Ctrl Pts',(45.8230286726291,-3.88694833223118,
125.963204080281));
#228606=CARTESIAN_POINT('Ctrl Pts',(45.5445810488162,-6.17399262105761,
131.457796973343));
#228607=CARTESIAN_POINT('Ctrl Pts',(45.2661334250033,-2.78743930743976,
136.351913777587));
#228608=CARTESIAN_POINT('Ctrl Pts',(44.9876858011905,3.16063455573481,136.148100240809));
#228609=CARTESIAN_POINT('Ctrl Pts',(44.7092381773775,6.20423966777097,131.033651046464));
#228610=CARTESIAN_POINT('Ctrl Pts',(44.4307905535647,3.54645161908363,125.708495149421));
#228611=CARTESIAN_POINT('Ctrl Pts',(44.1523429297517,-2.37035221374829,
125.066190670735));
#228612=CARTESIAN_POINT('Ctrl Pts',(43.8738953059389,-6.10891816028884,
129.696984048001));
#228613=CARTESIAN_POINT('Ctrl Pts',(43.5954476821259,-4.23368675476706,
135.345402394343));
#228614=CARTESIAN_POINT('Ctrl Pts',(43.3170000583131,1.53209595128933,136.820825190051));
#228615=CARTESIAN_POINT('Ctrl Pts',(43.0385524345002,5.88995732515911,132.767410964279));
#228616=CARTESIAN_POINT('Ctrl Pts',(42.7601048106873,4.83523565761953,126.910049370218));
#228617=CARTESIAN_POINT('Ctrl Pts',(42.4816571868744,-0.662831364878718,
124.631369564788));
#228618=CARTESIAN_POINT('Ctrl Pts',(42.2032095630615,-5.55178874416567,
128.025366969483));
#228619=CARTESIAN_POINT('Ctrl Pts',(41.9247619392486,-5.33892348752252,
133.973123775378));
#228620=CARTESIAN_POINT('Ctrl Pts',(41.6463143154357,-0.219848366758665,
137.008942041929));
#228621=CARTESIAN_POINT('Ctrl Pts',(41.3678666916229,5.10125666286673,134.343053090145));
#228622=CARTESIAN_POINT('Ctrl Pts',(41.0894190678099,5.73455602955998,128.425278630796));
#228623=CARTESIAN_POINT('Ctrl Pts',(40.8109714439971,1.09807855372398,124.693764292674));
#228624=CARTESIAN_POINT('Ctrl Pts',(40.5325238201841,-4.5474794688646,126.5775894579));
#228625=CARTESIAN_POINT('Ctrl Pts',(40.2540761963713,-6.01412601628932,
132.345610829607));
#228626=CARTESIAN_POINT('Ctrl Pts',(39.9756285725584,-1.95408456113369,
136.697298550707));
#228627=CARTESIAN_POINT('Ctrl Pts',(39.6971809487455,3.90166514336576,135.633664197272));
#228628=CARTESIAN_POINT('Ctrl Pts',(39.4187333249326,6.171975188051,130.132135778682));
#228629=CARTESIAN_POINT('Ctrl Pts',(39.1402857011198,2.77054155266769,125.248349147017));
#228630=CARTESIAN_POINT('Ctrl Pts',(38.8618380773068,-3.17688442113803,
125.470265630536));
#228631=CARTESIAN_POINT('Ctrl Pts',(38.583390453494,-6.20490881134979,130.593954822108));
#228632=CARTESIAN_POINT('Ctrl Pts',(38.304942829681,-3.53092513057837,135.910996660811));
#228633=CARTESIAN_POINT('Ctrl Pts',(38.0264952058682,2.38780624991219,136.535289448812));
#228634=CARTESIAN_POINT('Ctrl Pts',(37.7480475820552,6.11226033755391,131.893138612335));
#228635=CARTESIAN_POINT('Ctrl Pts',(37.4695999582424,4.21984577550119,126.250453988427));
#228636=CARTESIAN_POINT('Ctrl Pts',(37.1911523344295,-1.55040090331038,
124.792587085991));
#228637=CARTESIAN_POINT('Ctrl Pts',(36.9127047106166,-5.89590489327443,
128.859246367608));
#228638=CARTESIAN_POINT('Ctrl Pts',(36.6342570868037,-4.82336031728617,
134.713370620821));
#228639=CARTESIAN_POINT('Ctrl Pts',(36.3558094629908,0.681616756036961,
136.975305646799));
#228640=CARTESIAN_POINT('Ctrl Pts',(36.0773618391779,5.56022132939171,133.566443658335));
#228641=CARTESIAN_POINT('Ctrl Pts',(35.798914215365,5.32925413294858,127.619362290662));
#228642=CARTESIAN_POINT('Ctrl Pts',(35.5204665915522,0.200962736863706,
124.599138789596));
#228643=CARTESIAN_POINT('Ctrl Pts',(35.2420189677392,-5.11200359682353,
127.281211006494));
#228644=CARTESIAN_POINT('Ctrl Pts',(34.9635713439263,-5.72728836028912,
133.200885600541));
#228645=CARTESIAN_POINT('Ctrl Pts',(34.6851237201134,-1.07947491424015,
136.918270811987));
#228646=CARTESIAN_POINT('Ctrl Pts',(34.4066760963006,4.56032324271418,135.017271235878));
#228647=CARTESIAN_POINT('Ctrl Pts',(34.1282284724876,6.00940712379002,129.244812613665));
#228648=CARTESIAN_POINT('Ctrl Pts',(33.8497808486748,1.93613943396156,124.905502418881));
#228649=CARTESIAN_POINT('Ctrl Pts',(33.5713332248619,-3.91634581000783,
125.986954733445));
#228650=CARTESIAN_POINT('Ctrl Pts',(33.292885601049,-6.16990057870911,131.495367712155));
#228651=CARTESIAN_POINT('Ctrl Pts',(33.0144379772361,-2.753618131977,136.368778928511));
#228652=CARTESIAN_POINT('Ctrl Pts',(32.7359903534233,3.19310485631782,136.128761554055));
#228653=CARTESIAN_POINT('Ctrl Pts',(32.4575427296103,6.20552047350092,130.995879830412));
#228654=CARTESIAN_POINT('Ctrl Pts',(32.1790951057975,3.51536593206519,125.687001306397));
#228655=CARTESIAN_POINT('Ctrl Pts',(31.9006474819845,-2.40523816576522,
125.080725992446));
#228656=CARTESIAN_POINT('Ctrl Pts',(31.6221998581717,-6.11554589167424,
129.734191283883));
#228657=CARTESIAN_POINT('Ctrl Pts',(31.3437522343588,-4.20596570416061,
135.371089912296));
#228658=CARTESIAN_POINT('Ctrl Pts',(31.0653046105458,1.56869149262894,136.811387415981));
#228659=CARTESIAN_POINT('Ctrl Pts',(30.786856986733,5.90179784253235,132.731520751495));
#228660=CARTESIAN_POINT('Ctrl Pts',(30.5084093629201,4.81144029400183,126.880688070935));
#228661=CARTESIAN_POINT('Ctrl Pts',(30.2299617391072,-0.700395832790832,
124.635518778667));
#228662=CARTESIAN_POINT('Ctrl Pts',(29.9515141152943,-5.56860240548724,
128.05921377167));
#228663=CARTESIAN_POINT('Ctrl Pts',(29.6730664914815,-5.31953540889204,
134.005564608172));
#228664=CARTESIAN_POINT('Ctrl Pts',(29.3946188676685,-0.182075245277261,
137.010165364815));
#228665=CARTESIAN_POINT('Ctrl Pts',(29.1161712438556,5.12270317387725,134.311934729152));
#228666=CARTESIAN_POINT('Ctrl Pts',(28.8377236200427,5.71996763420123,128.390414839463));
#228667=CARTESIAN_POINT('Ctrl Pts',(28.5592759962298,1.06086127464794,124.687193192043));
#228668=CARTESIAN_POINT('Ctrl Pts',(28.280828372417,-4.57312477035222,126.605349568435));
#228669=CARTESIAN_POINT('Ctrl Pts',(28.0023807486041,-6.00463256096402,
132.382191965885));
#228670=CARTESIAN_POINT('Ctrl Pts',(27.7239331247912,-1.91817637065835,
136.709084435575));
#228671=CARTESIAN_POINT('Ctrl Pts',(27.4454855009783,3.93099019615694,135.60982417831));
#228672=CARTESIAN_POINT('Ctrl Pts',(27.1670378771654,6.16776881225138,130.094577668667));
#228673=CARTESIAN_POINT('Ctrl Pts',(26.8885902533525,2.73666920214424,125.231587014236));
#228674=CARTESIAN_POINT('Ctrl Pts',(26.6101426295396,-3.20929571101057,
125.48970305614));
#228675=CARTESIAN_POINT('Ctrl Pts',(26.3316950057267,-6.2060746485581,130.631729761538));
#228676=CARTESIAN_POINT('Ctrl Pts',(26.0532473819138,-3.49977416768234,
135.932395790139));
#228677=CARTESIAN_POINT('Ctrl Pts',(25.774799758101,2.42264779982026,136.52064801359));
#228678=CARTESIAN_POINT('Ctrl Pts',(25.4963521342881,6.11877479221284,131.85591137626));
#228679=CARTESIAN_POINT('Ctrl Pts',(25.2179045104751,4.19204666932822,126.224850962798));
#228680=CARTESIAN_POINT('Ctrl Pts',(24.9394568866623,-1.58696754980412,
124.802136200585));
#228681=CARTESIAN_POINT('Ctrl Pts',(24.6610092628494,-5.90763611834117,
128.895172452612));
#228682=CARTESIAN_POINT('Ctrl Pts',(24.3825616390365,-4.79947569819179,
134.742659359205));
#228683=CARTESIAN_POINT('Ctrl Pts',(24.1041140152236,0.719168421173241,
136.97104211882));
#228684=CARTESIAN_POINT('Ctrl Pts',(23.8256663914108,5.57693189481048,133.532545837923));
#228685=CARTESIAN_POINT('Ctrl Pts',(23.5472187675978,5.3097674053865,127.586980618775));
#228686=CARTESIAN_POINT('Ctrl Pts',(23.2687711437849,0.163186066970757,
124.598030440764));
#228687=CARTESIAN_POINT('Ctrl Pts',(22.990323519972,-5.13335529490864,127.312394499151));
#228688=CARTESIAN_POINT('Ctrl Pts',(22.7118758961592,-5.71259391911463,
133.235704828331));
#228689=CARTESIAN_POINT('Ctrl Pts',(22.4334282723462,-1.04223780738205,
136.924728605587));
#228690=CARTESIAN_POINT('Ctrl Pts',(22.1549806485334,4.58588393318709,134.98943319845));
#228691=CARTESIAN_POINT('Ctrl Pts',(21.8765330247205,5.9998023720423,129.208260541641));
#228692=CARTESIAN_POINT('Ctrl Pts',(21.5980854009075,1.90019553763114,124.893825880784));
#228693=CARTESIAN_POINT('Ctrl Pts',(21.3196377770947,-3.94559816615024,
126.010883897355));
#228694=CARTESIAN_POINT('Ctrl Pts',(21.0411901532818,-6.16557990842568,
131.532912845442));
#228695=CARTESIAN_POINT('Ctrl Pts',(20.7627425294689,-2.71969492018171,
136.385437887866));
#228696=CARTESIAN_POINT('Ctrl Pts',(20.484294905656,3.22545683522612,136.109225569666));
#228697=CARTESIAN_POINT('Ctrl Pts',(20.2058472818431,6.20657133138755,130.958101517545));
#228698=CARTESIAN_POINT('Ctrl Pts',(19.9273996580302,3.48414998186958,125.665697089004));
#228699=CARTESIAN_POINT('Ctrl Pts',(19.6489520342174,-2.44003499079723,
125.095473405541));
#228700=CARTESIAN_POINT('Ctrl Pts',(19.3705044104044,-6.12194700925765,
129.771438175283));
#228701=CARTESIAN_POINT('Ctrl Pts',(19.0920567865916,-4.17808879994825,
135.396608208416));
#228702=CARTESIAN_POINT('Ctrl Pts',(18.8136091627787,1.60522890552839,136.801727049323));
#228703=CARTESIAN_POINT('Ctrl Pts',(18.5351615389658,5.91341966661616,132.695559127084));
#228704=CARTESIAN_POINT('Ctrl Pts',(18.2567139151529,4.78746664069464,126.85147216478));
#228705=CARTESIAN_POINT('Ctrl Pts',(17.97826629134,-0.737934347277788,124.63989658125));
#228706=CARTESIAN_POINT('Ctrl Pts',(17.6998186675271,-5.58520972019883,
128.093162296283));
#228707=CARTESIAN_POINT('Ctrl Pts',(17.4213710437142,-5.29995021292075,
134.037886819174));
#228708=CARTESIAN_POINT('Ctrl Pts',(17.1429234199013,-0.144295376930669,
137.011158729324));
#228709=CARTESIAN_POINT('Ctrl Pts',(16.8644757960885,5.14395986123776,134.280686393713));
#228710=CARTESIAN_POINT('Ctrl Pts',(16.5860281722755,5.70516728333829,128.355640497777));
#228711=CARTESIAN_POINT('Ctrl Pts',(16.3075805484627,1.02360468496723,124.6808487653));
#228712=CARTESIAN_POINT('Ctrl Pts',(16.0291329246498,-4.5986006130197,126.633265274869));
#228713=CARTESIAN_POINT('Ctrl Pts',(15.7506853008369,-5.99491660177097,
132.418714635041));
#228714=CARTESIAN_POINT('Ctrl Pts',(15.472237677024,-1.88219710145218,136.720651518731));
#228715=CARTESIAN_POINT('Ctrl Pts',(15.1937900532111,3.96016958466077,135.585806091128));
#228716=CARTESIAN_POINT('Ctrl Pts',(14.9153424293982,6.16333388751023,130.057045859918));
#228717=CARTESIAN_POINT('Ctrl Pts',(14.6368948055853,2.70269544333712,125.215031382631));
#228718=CARTESIAN_POINT('Ctrl Pts',(14.3584471817724,-3.24158807925031,
125.509337418335));
#228719=CARTESIAN_POINT('Ctrl Pts',(14.0799995579596,-6.20701051738803,
130.669511097867));
#228720=CARTESIAN_POINT('Ctrl Pts',(13.8015519341466,-3.46849351936748,
135.953604898237));
#228721=CARTESIAN_POINT('Ctrl Pts',(13.5231043103337,2.45739957762318,136.505794759238));
#228722=CARTESIAN_POINT('Ctrl Pts',(13.2446566865208,6.12506251342167,131.818645174584));
#228723=CARTESIAN_POINT('Ctrl Pts',(12.966209062708,4.16409222532429,126.199417632585));
#228724=CARTESIAN_POINT('Ctrl Pts',(12.687761438895,-1.62347539063169,124.811907729812));
#228725=CARTESIAN_POINT('Ctrl Pts',(12.4093138150822,-5.91914843377905,
128.931169283287));
#228726=CARTESIAN_POINT('Ctrl Pts',(12.1308661912693,-4.77541323276041,
134.771802162479));
#228727=CARTESIAN_POINT('Ctrl Pts',(11.8524185674564,0.756693437259193,
136.96655008219));
#228728=CARTESIAN_POINT('Ctrl Pts',(11.5739709436435,5.59343580496719,133.498546923603));
#228729=CARTESIAN_POINT('Ctrl Pts',(11.2955233198306,5.2900839224404,127.554718168085));
#228730=CARTESIAN_POINT('Ctrl Pts',(11.0170756960177,0.125403350157864,
124.597152069781));
#228731=CARTESIAN_POINT('Ctrl Pts',(10.7386280722048,-5.15451677462551,
127.343707387895));
#228732=CARTESIAN_POINT('Ctrl Pts',(10.460180448392,-5.69768779567166,133.270433961767));
#228733=CARTESIAN_POINT('Ctrl Pts',(10.1817328245791,-1.0049620800187,136.930959606699));
#228734=CARTESIAN_POINT('Ctrl Pts',(9.90328520076621,4.61127469204443,134.961440081617));
#228735=CARTESIAN_POINT('Ctrl Pts',(9.62483757695328,5.98997529541125,129.171767613693));
#228736=CARTESIAN_POINT('Ctrl Pts',(9.34638995314043,1.86418122885626,124.882368359726));
#228737=CARTESIAN_POINT('Ctrl Pts',(9.0679423293275,-3.97470431670162,126.034990685308));
#228738=CARTESIAN_POINT('Ctrl Pts',(8.78949470551463,-6.16103077031137,
131.57043098196));
#228739=CARTESIAN_POINT('Ctrl Pts',(8.5110470817017,-2.68567092909101,136.401890038352));
#228740=CARTESIAN_POINT('Ctrl Pts',(8.2325994578889,3.25768929364524,136.089493011555));
#228741=CARTESIAN_POINT('Ctrl Pts',(7.95415183407592,6.20739220249103,130.920317507753));
#228742=CARTESIAN_POINT('Ctrl Pts',(7.67570421026306,3.45280492521512,125.644583286679));
#228743=CARTESIAN_POINT('Ctrl Pts',(7.39725658645018,-2.47474139943534,
125.110432363552));
#228744=CARTESIAN_POINT('Ctrl Pts',(7.11880896263729,-6.1281212758433,129.808723342005));
#228745=CARTESIAN_POINT('Ctrl Pts',(6.84036133882437,-4.15005707511893,
135.421956337113));
#228746=CARTESIAN_POINT('Ctrl Pts',(6.56191371501151,1.64170683608044,136.791844448048));
#228747=CARTESIAN_POINT('Ctrl Pts',(6.28346609119863,5.92482236675955,132.659527423617));
#228748=CARTESIAN_POINT('Ctrl Pts',(6.00501846738572,4.76331558605049,126.822402734361));
#228749=CARTESIAN_POINT('Ctrl Pts',(5.72657084357281,-0.775445517336138,
124.644502810313));
#228750=CARTESIAN_POINT('Ctrl Pts',(5.44812321975995,-5.60161007291028,
128.127211285347));
#228751=CARTESIAN_POINT('Ctrl Pts',(5.16967559594705,-5.28016862534525,
134.070089210674));
#228752=CARTESIAN_POINT('Ctrl Pts',(4.89122797213414,-0.106510161665837,
137.011922098645));
#228753=CARTESIAN_POINT('Ctrl Pts',(4.6127803483213,5.16502593727395,134.249309241742));
#228754=CARTESIAN_POINT('Ctrl Pts',(4.33433272450837,5.69015552540359,128.320956894316));
#228755=CARTESIAN_POINT('Ctrl Pts',(4.05588510069549,0.986310165238503,
124.674731247541));
#228756=CARTESIAN_POINT('Ctrl Pts',(3.77743747688256,-4.62390605285035,
126.661335542776));
#228757=CARTESIAN_POINT('Ctrl Pts',(3.49898985306972,-5.98497849873861,
132.455177483715));
#228758=CARTESIAN_POINT('Ctrl Pts',(3.22054222925682,-1.84614808674025,
136.731999371551));
#228759=CARTESIAN_POINT('Ctrl Pts',(2.94209460544391,3.9892022276243,135.561610825727));
#228760=CARTESIAN_POINT('Ctrl Pts',(2.66364698163102,6.15867057816533,130.019541743194));
#228761=CARTESIAN_POINT('Ctrl Pts',(2.38519935781816,2.66862153515642,125.198682865676));
#228762=CARTESIAN_POINT('Ctrl Pts',(2.10675173400524,-3.27376032925169,
125.529167989562));
#228763=CARTESIAN_POINT('Ctrl Pts',(1.82830411019233,-6.20771638316062,
130.707297431096));
#228764=CARTESIAN_POINT('Ctrl Pts',(1.54985648637947,-3.43708434474973,
135.974623199195));
#228765=CARTESIAN_POINT('Ctrl Pts',(1.27140886256659,2.49206029558105,136.490730236146));
#228766=CARTESIAN_POINT('Ctrl Pts',(0.992961238753657,6.13112326818657,
131.78134138822));
#228767=CARTESIAN_POINT('Ctrl Pts',(0.714513614940807,4.13598347935162,
126.174154940227));
#228768=CARTESIAN_POINT('Ctrl Pts',(0.436065991127901,-1.65992307298164,
124.821901311585));
#228769=CARTESIAN_POINT('Ctrl Pts',(0.157618367314999,-5.93044141299494,
128.967235525755));
#228770=CARTESIAN_POINT('Ctrl Pts',(-0.120829256497892,-4.75117381263555,
134.800797950748));
#228771=CARTESIAN_POINT('Ctrl Pts',(-0.399276880310752,0.794190413791566,
136.961829703365));
#228772=CARTESIAN_POINT('Ctrl Pts',(-0.67772450412367,5.60973244830296,
133.464448175219));
#228773=CARTESIAN_POINT('Ctrl Pts',(-0.956172127936585,5.27020441348929,
127.522576134092));
#228774=CARTESIAN_POINT('Ctrl Pts',(-1.23461975174943,0.0876159864779326,
124.596503709192));
#228775=CARTESIAN_POINT('Ctrl Pts',(-1.51306737556233,-5.17548725182775,
127.375148512417));
#228776=CARTESIAN_POINT('Ctrl Pts',(-1.79151499937523,-5.6825705423121,
133.305071713949));
#228777=CARTESIAN_POINT('Ctrl Pts',(-2.06996262318813,-0.967649113415911,
136.936963584433));
#228778=CARTESIAN_POINT('Ctrl Pts',(-2.34841024700098,4.63649457842225,
134.933292922676));
#228779=CARTESIAN_POINT('Ctrl Pts',(-2.62685787081389,5.97992625804282,
129.13533518208));
#228780=CARTESIAN_POINT('Ctrl Pts',(-2.90530549462681,1.82809784216042,
124.871130280269));
#228781=CARTESIAN_POINT('Ctrl Pts',(-3.18375311843967,-4.00366318312286,
126.059274204017));
#228782=CARTESIAN_POINT('Ctrl Pts',(-3.46220074225256,-6.15625333293613,
131.607920731459));
#228783=CARTESIAN_POINT('Ctrl Pts',(-3.74064836606547,-2.65154741947636,
136.418134770325));
#228784=CARTESIAN_POINT('Ctrl Pts',(-4.01909598987837,3.28980103718956,
136.06956461092));
#228785=CARTESIAN_POINT('Ctrl Pts',(-4.29754361369122,6.20798305639367,
130.882529201136));
#228786=CARTESIAN_POINT('Ctrl Pts',(-4.57599123750414,3.42133192360438,
125.623660681799));
#228787=CARTESIAN_POINT('Ctrl Pts',(-4.85443886131705,-2.5093561056208,
125.125602312169));
#228788=CARTESIAN_POINT('Ctrl Pts',(-5.13288648512991,-6.13406846264146,
129.846045402432));
#228789=CARTESIAN_POINT('Ctrl Pts',(-5.41133410894279,-4.12187156839848,
135.447133359102));
#228790=CARTESIAN_POINT('Ctrl Pts',(-5.68978173275571,1.67812393258193,
136.781739978358));
#228791=CARTESIAN_POINT('Ctrl Pts',(-5.9682293565686,5.93600552043131,132.623426976261));
#228792=CARTESIAN_POINT('Ctrl Pts',(-6.24667698038146,4.73898802499559,
126.793480856855));
#228793=CARTESIAN_POINT('Ctrl Pts',(-6.52512460419438,-0.812927952975666,
124.649337295173));
#228794=CARTESIAN_POINT('Ctrl Pts',(-6.80357222800728,-5.61780285590049,
128.161359477164));
#228795=CARTESIAN_POINT('Ctrl Pts',(-7.08201985182013,-5.26019137917956,
134.1021705894));
#228796=CARTESIAN_POINT('Ctrl Pts',(-7.36046747563304,-0.0687209996277829,
137.012455444495));
#228797=CARTESIAN_POINT('Ctrl Pts',(-7.63891509944595,5.18590062137458,
134.217804435933));
#228798=CARTESIAN_POINT('Ctrl Pts',(-7.91736272325884,5.67493291666336,
128.286365314294));
#228799=CARTESIAN_POINT('Ctrl Pts',(-8.1958103470717,0.948979097423875,
124.668840865451));
#228800=CARTESIAN_POINT('Ctrl Pts',(-8.47425797088461,-4.64904015214177,
126.689559331999));
#228801=CARTESIAN_POINT('Ctrl Pts',(-8.75270559469752,-5.97481862012702,
132.491579160764));
#228802=CARTESIAN_POINT('Ctrl Pts',(-9.03115321851038,-1.81003066233205,
136.743127573537));
#228803=CARTESIAN_POINT('Ctrl Pts',(-9.30960084232328,4.0180870492325,135.537239278668));
#228804=CARTESIAN_POINT('Ctrl Pts',(-9.58804846613619,6.15377905701727,
129.982066708221));
#228805=CARTESIAN_POINT('Ctrl Pts',(-9.86649608994908,2.63444874022312,
125.182542069172));
#228806=CARTESIAN_POINT('Ctrl Pts',(-10.144943713762,-3.30581126886015,
125.549194034992));
#228807=CARTESIAN_POINT('Ctrl Pts',(-10.4233913375749,-6.20819221971975,
130.745087361036));
#228808=CARTESIAN_POINT('Ctrl Pts',(-10.7018389613878,-3.40554780770759,
135.995449914173));
#228809=CARTESIAN_POINT('Ctrl Pts',(-10.9802865852006,2.52662866932821,
136.475455002538));
#228810=CARTESIAN_POINT('Ctrl Pts',(-11.2587342090136,6.13695683192405,
131.744001399476));
#228811=CARTESIAN_POINT('Ctrl Pts',(-11.5371818328265,4.10772147299012,
126.149063821843));
#228812=CARTESIAN_POINT('Ctrl Pts',(-11.8156294566394,-1.69630924627168,
124.832116575588));
#228813=CARTESIAN_POINT('Ctrl Pts',(-12.0940770804522,-5.94151463752335,
129.003369843568));
#228814=CARTESIAN_POINT('Ctrl Pts',(-12.3725247042651,-4.72675833601782,
134.829645649562));
#228815=CARTESIAN_POINT('Ctrl Pts',(-12.6509723280781,0.83165796130609,
136.956881157257));
#228816=CARTESIAN_POINT('Ctrl Pts',(-12.9294199518909,5.62582122093989,
133.430250856313));
#228817=CARTESIAN_POINT('Ctrl Pts',(-13.2078675757038,5.25012961517551,
127.490555707831));
#228818=CARTESIAN_POINT('Ctrl Pts',(-13.4863151995167,0.0498253761554086,
124.596085383024));
#228819=CARTESIAN_POINT('Ctrl Pts',(-13.7647628233296,-5.19626594944658,
127.406716707655));
#228820=CARTESIAN_POINT('Ctrl Pts',(-14.0432104471424,-5.66724271921134,
133.339616801361));
#228821=CARTESIAN_POINT('Ctrl Pts',(-14.3216580709554,-0.930300290219375,
136.942740316309));
#228822=CARTESIAN_POINT('Ctrl Pts',(-14.6001056947683,4.6615426577884,134.904992764631));
#228823=CARTESIAN_POINT('Ctrl Pts',(-14.8785533185811,5.96965563230779,
129.098964596818));
#228824=CARTESIAN_POINT('Ctrl Pts',(-15.157000942394,1.79194671462675,124.860112058844));
#228825=CARTESIAN_POINT('Ctrl Pts',(-15.4354485662069,-4.03247369233249,
126.08373355365));
#228826=CARTESIAN_POINT('Ctrl Pts',(-15.7138961900198,-6.15124777332969,
131.645380704742));
#228827=CARTESIAN_POINT('Ctrl Pts',(-15.9923438138327,-2.61732565579698,
136.434171481834));
#228828=CARTESIAN_POINT('Ctrl Pts',(-16.2707914376456,3.32179087594663,
136.049441106215));
#228829=CARTESIAN_POINT('Ctrl Pts',(-16.5492390614585,6.2083438712012,130.844737997954));
#228830=CARTESIAN_POINT('Ctrl Pts',(-16.8276866852714,3.38973214328102,
125.602930049661));
#228831=CARTESIAN_POINT('Ctrl Pts',(-17.1061343090842,-2.54387782669295,
125.140982689263));
#228832=CARTESIAN_POINT('Ctrl Pts',(-17.3845819328972,-6.13978834927694,
129.883402973582));
#228833=CARTESIAN_POINT('Ctrl Pts',(-17.66302955671,-4.09353332421128,135.47213834144));
#228834=CARTESIAN_POINT('Ctrl Pts',(-17.9414771805229,1.71447884558397,
136.771414014676));
#228835=CARTESIAN_POINT('Ctrl Pts',(-18.2199248043358,5.94696871323555,
132.587259122732));
#228836=CARTESIAN_POINT('Ctrl Pts',(-18.4983724281487,4.71448485899666,
126.764707603974));
#228837=CARTESIAN_POINT('Ctrl Pts',(-18.7768200519616,-0.850380265270943,
124.654399856686));
#228838=CARTESIAN_POINT('Ctrl Pts',(-19.0552676757745,-5.63378746913994,
128.19560560636));
#228839=CARTESIAN_POINT('Ctrl Pts',(-19.3337152995874,-5.24001921468789,
134.134129766565));
#228840=CARTESIAN_POINT('Ctrl Pts',(-19.6121629234003,-0.0309292911078312,
137.012758747106));
#228841=CARTESIAN_POINT('Ctrl Pts',(-19.8906105472132,5.2065831400206,134.18617314371));
#228842=CARTESIAN_POINT('Ctrl Pts',(-20.1690581710261,5.65950002119693,
128.251867039513));
#228843=CARTESIAN_POINT('Ctrl Pts',(-20.447505794839,0.911612864839816,
124.663177837304));
#228844=CARTESIAN_POINT('Ctrl Pts',(-20.7259534186518,-4.67400197954067,
126.717935596697));
#228845=CARTESIAN_POINT('Ctrl Pts',(-21.0044010424647,-5.96443734241423,
132.527918317308));
#228846=CARTESIAN_POINT('Ctrl Pts',(-21.2828486662776,-1.77384616657202,
136.754035712331));
#228847=CARTESIAN_POINT('Ctrl Pts',(-21.5612962900905,4.0468229791472,135.512692353051));
#228848=CARTESIAN_POINT('Ctrl Pts',(-21.8397439139034,6.14865950532324,
129.944622143653));
#228849=CARTESIAN_POINT('Ctrl Pts',(-22.1181915377163,2.60017832482316,
125.166609591221));
#228850=CARTESIAN_POINT('Ctrl Pts',(-22.3966391615293,-3.33773971041633,
125.569414812551));
#228851=CARTESIAN_POINT('Ctrl Pts',(-22.6750867853421,-6.20843800943312,
130.782879487369));
#228852=CARTESIAN_POINT('Ctrl Pts',(-22.953534409155,-3.37388507683905,
136.016084271426));
#228853=CARTESIAN_POINT('Ctrl Pts',(-23.2319820329679,2.56110341792085,
136.45996962444));
#228854=CARTESIAN_POINT('Ctrl Pts',(-23.5104296567807,6.14256298846929,
131.706626591997));
#228855=CARTESIAN_POINT('Ctrl Pts',(-23.7888772805937,4.07930725349882,
126.124145207193));
#228856=CARTESIAN_POINT('Ctrl Pts',(-24.0673249044065,-1.73263256219878,
124.842553143289));
#228857=CARTESIAN_POINT('Ctrl Pts',(-24.3457725282195,-5.95236769704188,
129.039570897758));
#228858=CARTESIAN_POINT('Ctrl Pts',(-24.6242201520323,-4.70216770763169,
134.858344189959));
#228859=CARTESIAN_POINT('Ctrl Pts',(-24.9026677758452,0.86909469142902,
136.951704627238));
#228860=CARTESIAN_POINT('Ctrl Pts',(-25.1811153996581,5.64170152670257,
133.395956234079));
#228861=CARTESIAN_POINT('Ctrl Pts',(-25.459563023471,5.22986027137813,127.458658075828));
#228862=CARTESIAN_POINT('Ctrl Pts',(-25.7380106472839,0.0120329195352371,
124.595897106778));
#228863=CARTESIAN_POINT('Ctrl Pts',(-26.0164582710968,-5.21685209751974,
127.438410803838));
#228864=CARTESIAN_POINT('Ctrl Pts',(-26.2949058949097,-5.6517048943475,
133.374067943923));
#228865=CARTESIAN_POINT('Ctrl Pts',(-26.5733535187226,-0.892916994403456,
136.948289588268));
#228866=CARTESIAN_POINT('Ctrl Pts',(-26.8518011425354,4.68641800197708,
134.876540656153));
#228867=CARTESIAN_POINT('Ctrl Pts',(-27.1302487663484,5.95916379878798,
129.062657205632));
#228868=CARTESIAN_POINT('Ctrl Pts',(-27.4086963901612,1.75572918584856,
124.849314103734));
#228869=CARTESIAN_POINT('Ctrl Pts',(-27.6871440139742,-4.06113477674652,
126.108367827853));
#228870=CARTESIAN_POINT('Ctrl Pts',(-27.965591637787,-6.1460142769749,131.682809513716));
#228871=CARTESIAN_POINT('Ctrl Pts',(-28.2440392616,-2.5830069061529,136.449999578631));
#228872=CARTESIAN_POINT('Ctrl Pts',(-28.5224868854127,3.3536576245212,136.029123243122));
#228873=CARTESIAN_POINT('Ctrl Pts',(-28.8009345092257,6.20847463354345,
130.806945298572));
#228874=CARTESIAN_POINT('Ctrl Pts',(-29.0793821330386,3.35800675518651,
125.582392158445));
#228875=CARTESIAN_POINT('Ctrl Pts',(-29.3578297568515,-2.57830528343674,
125.156572924908));
#228876=CARTESIAN_POINT('Ctrl Pts',(-29.6362773806644,-6.14528072379723,
129.920794671155));
#228877=CARTESIAN_POINT('Ctrl Pts',(-29.9147250044772,-4.06504339264135,
135.496970357558));
#228878=CARTESIAN_POINT('Ctrl Pts',(-30.1931726282902,1.75077022794215,
136.760866939637));
#228879=CARTESIAN_POINT('Ctrl Pts',(-30.471620252103,5.95771153892721,132.551025203244));
#228880=CARTESIAN_POINT('Ctrl Pts',(-30.750067875916,4.68980699602731,126.736084041921));
#228881=CARTESIAN_POINT('Ctrl Pts',(-31.0285154997288,-0.887801066412759,
124.659690307256));
#228882=CARTESIAN_POINT('Ctrl Pts',(-31.3069631235417,-5.6495633203129,
128.229948403933));
#228883=CARTESIAN_POINT('Ctrl Pts',(-31.5854107473546,-5.21965287935721,
134.16596555791));
#228884=CARTESIAN_POINT('Ctrl Pts',(-31.8638583711675,0.00686356350839004,
137.012831995241));
#228885=CARTESIAN_POINT('Ctrl Pts',(-32.1423059949804,5.22707272681363,
134.154416537178));
#228886=CARTESIAN_POINT('Ctrl Pts',(-32.4207536187933,5.64385741087595,
128.217463348321));
#228887=CARTESIAN_POINT('Ctrl Pts',(-32.6992012426062,0.874212852105795,
124.657742372942));
#228888=CARTESIAN_POINT('Ctrl Pts',(-32.9776488664191,-4.69879061007736,
126.746463285377));
#228889=CARTESIAN_POINT('Ctrl Pts',(-33.2560964902319,-5.9538350502823,
132.564193606789));
#228890=CARTESIAN_POINT('Ctrl Pts',(-33.5345441140448,-1.73759594028995,
136.764723383724));
#228891=CARTESIAN_POINT('Ctrl Pts',(-33.8129917378578,4.07540895254819,
135.487970958469));
#228892=CARTESIAN_POINT('Ctrl Pts',(-34.0914393616706,6.14331211279008,
129.907209437008));
#228893=CARTESIAN_POINT('Ctrl Pts',(-34.3698869854835,2.56581155885918,
125.150886022208));
#228894=CARTESIAN_POINT('Ctrl Pts',(-34.6483346092964,-3.3695444708001,
125.589829572953));
#228895=CARTESIAN_POINT('Ctrl Pts',(-34.9267822331094,-6.2084537431929,
130.820672409693));
#228896=CARTESIAN_POINT('Ctrl Pts',(-35.2052298569221,-3.34209732541825,
136.036525506343));
#228897=CARTESIAN_POINT('Ctrl Pts',(-35.4836774807351,2.59548326388451,
136.444274675672));
#228898=CARTESIAN_POINT('Ctrl Pts',(-35.7621251045479,6.14794153008404,
131.66921835072));
#228899=CARTESIAN_POINT('Ctrl Pts',(-36.0405727283609,4.05074187377708,
126.099400019648));
#228900=CARTESIAN_POINT('Ctrl Pts',(-36.3190203521737,-1.76889167478912,
124.85321062796));
#228901=CARTESIAN_POINT('Ctrl Pts',(-36.5974679759867,-5.96300018938643,
129.075837346879));
#228902=CARTESIAN_POINT('Ctrl Pts',(-36.8759155997995,-4.67740283869194,
134.886892508504));
#228903=CARTESIAN_POINT('Ctrl Pts',(-37.1543632236125,0.906499216928551,
136.946300305126));
#228904=CARTESIAN_POINT('Ctrl Pts',(-37.4328108474252,5.65737277714046,
133.361565579315));
#228905=CARTESIAN_POINT('Ctrl Pts',(-37.7112584712383,5.2093971331851,127.426884420063));
#228906=CARTESIAN_POINT('Ctrl Pts',(-37.9897060950511,-0.0257599829691867,
124.595938887431));
#228907=CARTESIAN_POINT('Ctrl Pts',(-38.268153718864,-5.23724493321992,
127.470229626529));
#228908=CARTESIAN_POINT('Ctrl Pts',(-38.5466013426768,-5.63595764348039,
133.408423865036));
#228909=CARTESIAN_POINT('Ctrl Pts',(-38.8250489664898,-0.855500611219946,
136.953611194679));
#228910=CARTESIAN_POINT('Ctrl Pts',(-39.1034965903026,4.71111968922328,
134.847937651547));
#228911=CARTESIAN_POINT('Ctrl Pts',(-39.3819442141156,5.94845114626212,
129.026414353905));
#228912=CARTESIAN_POINT('Ctrl Pts',(-39.6603918379284,1.71944659787975,
124.838736815064));
#228913=CARTESIAN_POINT('Ctrl Pts',(-39.9388394617414,-4.08964537431793,
126.133176113797));
#228914=CARTESIAN_POINT('Ctrl Pts',(-40.2172870855541,-6.14055303780089,
131.720205771443));
#228915=CARTESIAN_POINT('Ctrl Pts',(-40.495734709367,-2.54859244223803,
136.465618474199));
#228916=CARTESIAN_POINT('Ctrl Pts',(-40.7741823331801,3.3854001020792,136.008611774531));
#228917=CARTESIAN_POINT('Ctrl Pts',(-41.0526299569928,6.20837533857501,
130.769152503414));
#228918=CARTESIAN_POINT('Ctrl Pts',(-41.3310775808058,3.3261569349168,125.562047769191));
#228919=CARTESIAN_POINT('Ctrl Pts',(-41.6095252046187,-2.61263720013008,
125.172372441404));
#228920=CARTESIAN_POINT('Ctrl Pts',(-41.8879728284316,-6.15054538268038,
129.958219109591));
#228921=CARTESIAN_POINT('Ctrl Pts',(-42.1664204522444,-4.03640282939359,
135.521628487296));
#228922=CARTESIAN_POINT('Ctrl Pts',(-42.4448680760573,1.78699673486542,
136.750099144066));
#228923=CARTESIAN_POINT('Ctrl Pts',(-42.7233156998703,5.96823359942677,
132.514726560457));
#228924=CARTESIAN_POINT('Ctrl Pts',(-43.0017633236831,4.66495535053527,
126.707611231352));
#228925=CARTESIAN_POINT('Ctrl Pts',(-43.2802109474961,-0.925188969759574,
124.665208450844));
#228926=CARTESIAN_POINT('Ctrl Pts',(-43.5586585713089,-5.6651298248394,
128.264386597296));
#228927=CARTESIAN_POINT('Ctrl Pts',(-43.8371061951219,-5.19909312786956,
134.197676783747));
#228928=CARTESIAN_POINT('Ctrl Pts',(-44.1155538189346,0.0446561637927345,
137.012675186187));
#228929=CARTESIAN_POINT('Ctrl Pts',(-44.3940014427476,5.24736862250453,
134.122535793092));
#228930=CARTESIAN_POINT('Ctrl Pts',(-44.6724490665605,5.62800566534308,
128.183155515557));
#228931=CARTESIAN_POINT('Ctrl Pts',(-44.9508966903734,0.836780445093053,
124.65253467378));
#228932=CARTESIAN_POINT('Ctrl Pts',(-45.2293443141862,-4.72340512520001,
126.775141340936));
#228933=CARTESIAN_POINT('Ctrl Pts',(-45.5077919379991,-5.94301213660306,
132.600403685011));
#228934=CARTESIAN_POINT('Ctrl Pts',(-45.7862395618121,-1.7012813267513,
136.775190191685));
#228935=CARTESIAN_POINT('Ctrl Pts',(-46.0646871856249,4.10384391017172,
135.463076010984));
#228936=CARTESIAN_POINT('Ctrl Pts',(-46.3431348094379,6.13773707756737,
129.869829974632));
#228937=CARTESIAN_POINT('Ctrl Pts',(-46.6215824332507,2.5313497158043,125.135371944775));
#228938=CARTESIAN_POINT('Ctrl Pts',(-46.9000300570636,-3.40122437147435,
125.610437559721));
#228939=CARTESIAN_POINT('Ctrl Pts',(-47.1784776808764,-6.20823942041608,
130.858464727578));
#228940=CARTESIAN_POINT('Ctrl Pts',(-47.4569253046894,-3.31018573135201,
136.056772861467));
#228941=CARTESIAN_POINT('Ctrl Pts',(-47.7353729285023,2.62976693326135,
136.428370737814));
#228942=CARTESIAN_POINT('Ctrl Pts',(-48.0138205523151,6.15309225746451,
131.631778061822));
#228943=CARTESIAN_POINT('Ctrl Pts',(-48.2922681761281,4.02202639232555,
126.074829176147));
#228944=CARTESIAN_POINT('Ctrl Pts',(-48.570715799941,-1.80508524044794,
124.864088634681));
#228945=CARTESIAN_POINT('Ctrl Pts',(-48.8491634237538,-5.97341172056607,
129.112167847066));
#228946=CARTESIAN_POINT('Ctrl Pts',(-49.1276110475668,-4.65246464686987,
134.915289547327));
#228947=CARTESIAN_POINT('Ctrl Pts',(-49.4060586713796,0.943870151766231,
136.940668391181));
#228948=CARTESIAN_POINT('Ctrl Pts',(-49.6845062951925,5.6728343915496,133.327080166382));
#228949=CARTESIAN_POINT('Ctrl Pts',(-49.9629539190054,5.18874095886556,
127.395235917922));
#228950=CARTESIAN_POINT('Ctrl Pts',(-50.2414015428183,-0.0635519309279763,
124.596210723434));
#228951=CARTESIAN_POINT('Ctrl Pts',(-50.5198491666312,-5.25744370088312,
127.50217199667));
#228952=CARTESIAN_POINT('Ctrl Pts',(-50.798296790444,-5.6200015501302,133.442683291627));
#228953=CARTESIAN_POINT('Ctrl Pts',(-51.076744414257,-0.818052527146474,
136.958704938348));
#228954=CARTESIAN_POINT('Ctrl Pts',(-51.3551920380699,4.73564680419706,
134.819184810706));
#228955=CARTESIAN_POINT('Ctrl Pts',(-51.6336396618827,5.93751807169133,
128.990237384633));
#228956=CARTESIAN_POINT('Ctrl Pts',(-51.9120872856956,1.68310029518491,
124.828380584778));
#228957=CARTESIAN_POINT('Ctrl Pts',(-52.1905349095086,-4.11800442857602,
126.1581574922));
#228958=CARTESIAN_POINT('Ctrl Pts',(-52.4689825333214,-6.13486425817587,
131.757568092191));
#228959=CARTESIAN_POINT('Ctrl Pts',(-52.7474301571343,-2.51408353929296,
136.481027589776));
#228960=CARTESIAN_POINT('Ctrl Pts',(-53.0258777809472,3.41701713239144,
135.987907460498));
#228961=CARTESIAN_POINT('Ctrl Pts',(-53.3043254047601,6.20804598997526,
130.731361012906));
#228962=CARTESIAN_POINT('Ctrl Pts',(-53.5827730285729,3.29418386267868,
125.541897635768));
#228963=CARTESIAN_POINT('Ctrl Pts',(-53.8612206523859,-2.64687230459117,
125.188380653292));
#228964=CARTESIAN_POINT('Ctrl Pts',(-54.1396682761987,-6.15558213084251,
129.995674902111));
#228965=CARTESIAN_POINT('Ctrl Pts',(-54.4181159000117,-4.0076126957546,
135.546111816938));
#228966=CARTESIAN_POINT('Ctrl Pts',(-54.6965635238244,1.82315702396754,
136.739111026966));
#228967=CARTESIAN_POINT('Ctrl Pts',(-54.9750111476374,5.97853450483549,
132.478364539431));
#228968=CARTESIAN_POINT('Ctrl Pts',(-55.2534587714502,4.63993084340721,
126.679290227339));
#228969=CARTESIAN_POINT('Ctrl Pts',(-55.5319063952633,-0.962542589888887,
124.670954082973));
#228970=CARTESIAN_POINT('Ctrl Pts',(-55.810354019076,-5.68048640589689,
128.298918910331));
#228971=CARTESIAN_POINT('Ctrl Pts',(-56.088801642889,-5.1783407220741,134.229262269005));
#228972=CARTESIAN_POINT('Ctrl Pts',(-56.3672492667019,0.0824471093265141,
137.012288325754));
#228973=CARTESIAN_POINT('Ctrl Pts',(-56.6456968905149,5.26747007502141,
134.090532092806));
#228974=CARTESIAN_POINT('Ctrl Pts',(-56.9241445143275,5.6119453719906,128.148944812513));
#228975=CARTESIAN_POINT('Ctrl Pts',(-57.2025921381407,0.799317030873196,
124.64755493279));
#228976=CARTESIAN_POINT('Ctrl Pts',(-57.4810397619534,-4.74784461280872,
126.803968700697));
#228977=CARTESIAN_POINT('Ctrl Pts',(-57.7594873857663,-5.93196900242356,
132.636547210196));
#228978=CARTESIAN_POINT('Ctrl Pts',(-58.0379350095792,-1.66490367160747,
136.785435748359));
#228979=CARTESIAN_POINT('Ctrl Pts',(-58.3163826333922,4.13212679834998,
135.438008433087));
#228980=CARTESIAN_POINT('Ctrl Pts',(-58.5948302572049,6.13193460624012,
129.832485141631));
#228981=CARTESIAN_POINT('Ctrl Pts',(-58.873277881018,2.49679407265481,125.120067933803));
#228982=CARTESIAN_POINT('Ctrl Pts',(-59.1517255048308,-3.43277823852872,
125.631238009216));
#228983=CARTESIAN_POINT('Ctrl Pts',(-59.4301731286437,-6.20779504904446,
130.896255040614));
#228984=CARTESIAN_POINT('Ctrl Pts',(-59.7086207524566,-3.27815147713605,
136.076825586523));
#228985=CARTESIAN_POINT('Ctrl Pts',(-59.9870683762695,2.66395315565763,
136.412258400192));
#228986=CARTESIAN_POINT('Ctrl Pts',(-60.2655160000824,6.15801497974849,
131.594307112665));
#228987=CARTESIAN_POINT('Ctrl Pts',(-60.5439636238952,3.99316187320697,
126.050433587173));
#228988=CARTESIAN_POINT('Ctrl Pts',(-60.8224112477081,-1.84121191800936,
124.875186760365));
#228989=CARTESIAN_POINT('Ctrl Pts',(-61.1008588715211,-5.98360190477769,
129.148561052078));
#228990=CARTESIAN_POINT('Ctrl Pts',(-61.3793064953339,-4.62735405625939,
134.943534254169));
#228991=CARTESIAN_POINT('Ctrl Pts',(-61.6577541191468,0.981206111148332,
136.934809094094));
#228992=CARTESIAN_POINT('Ctrl Pts',(-61.9362017429597,5.68808579699418,
133.292501273148));
#228993=CARTESIAN_POINT('Ctrl Pts',(-62.2146493667725,5.16789251384163,
127.36371374215));
#228994=CARTESIAN_POINT('Ctrl Pts',(-62.4930969905855,-0.10134152394658,
124.596712604715));
#228995=CARTESIAN_POINT('Ctrl Pts',(-62.7715446143984,-5.27744765203657,
127.534236730624));
#228996=CARTESIAN_POINT('Ctrl Pts',(-63.0499922382113,-5.60383720555579,
133.476844954201));
#228997=CARTESIAN_POINT('Ctrl Pts',(-63.3284398620242,-0.780574129835986,
136.963570630527));
#228998=CARTESIAN_POINT('Ctrl Pts',(-63.606887485837,4.75999843803683,134.790283199078));
#228999=CARTESIAN_POINT('Ctrl Pts',(-63.88533510965,5.92636498020503,128.954127638363));
#229000=CARTESIAN_POINT('Ctrl Pts',(-64.1637827334628,1.64669162458969,
124.818245796629));
#229001=CARTESIAN_POINT('Ctrl Pts',(-64.4422303572757,-4.14621088866563,
126.183311037368));
#229002=CARTESIAN_POINT('Ctrl Pts',(-64.7206779810887,-6.12894814889968,
131.794895091487));
#229003=CARTESIAN_POINT('Ctrl Pts',(-64.9991256049015,-2.47948147605779,
136.49622635437));
#229004=CARTESIAN_POINT('Ctrl Pts',(-65.2775732287142,3.44850754387722,
135.967011068231));
#229005=CARTESIAN_POINT('Ctrl Pts',(-65.5560208525274,6.20748659994837,
130.693572227424));
#229006=CARTESIAN_POINT('Ctrl Pts',(-65.83446847634,3.26208872324607,125.521942504845));
#229007=CARTESIAN_POINT('Ctrl Pts',(-66.1129161001531,-2.68100932822562,
125.204596967384));
#229008=CARTESIAN_POINT('Ctrl Pts',(-66.3913637239659,-6.1603907816451,
130.033160660777));
#229009=CARTESIAN_POINT('Ctrl Pts',(-66.6698113477789,-3.97867405855336,
135.570419439246));
#229010=CARTESIAN_POINT('Ctrl Pts',(-66.9482589715917,1.85924975531565,
136.727902995508));
#229011=CARTESIAN_POINT('Ctrl Pts',(-67.2267065954047,5.98861387344954,
132.441940487574));
#229012=CARTESIAN_POINT('Ctrl Pts',(-67.5051542192175,4.61473440193538,
126.651122079325));
#229013=CARTESIAN_POINT('Ctrl Pts',(-67.7836018430304,-0.999860542648545,
124.676926990737));
#229014=CARTESIAN_POINT('Ctrl Pts',(-68.0620494668433,-5.69563249444164,
128.33354406343));
#229015=CARTESIAN_POINT('Ctrl Pts',(-68.3404970906562,-5.15739643095884,
134.260720843274));
#229016=CARTESIAN_POINT('Ctrl Pts',(-68.618944714469,0.120234999752325,
137.011671428276));
#229017=CARTESIAN_POINT('Ctrl Pts',(-68.8973923382821,5.28737633949755,
134.058406622227));
#229018=CARTESIAN_POINT('Ctrl Pts',(-69.1758399620947,5.59567712593856,
128.114832506878));
#229019=CARTESIAN_POINT('Ctrl Pts',(-69.4542875859078,0.761823997666808,
124.642803334499));
#229020=CARTESIAN_POINT('Ctrl Pts',(-69.7327352097205,-4.77210816728929,
126.832944296451));
#229021=CARTESIAN_POINT('Ctrl Pts',(-70.0111828335336,-5.92070605695121,
132.672622843033));
#229022=CARTESIAN_POINT('Ctrl Pts',(-70.2896304573463,-1.62846432284579,
136.795459674095));
#229023=CARTESIAN_POINT('Ctrl Pts',(-70.5680780811594,4.16025656905012,
135.412769153666));
#229024=CARTESIAN_POINT('Ctrl Pts',(-70.8465257049722,6.12590491382102,
129.795176321834));
#229025=CARTESIAN_POINT('Ctrl Pts',(-71.1249733287852,2.46214590988275,
125.104974556385));
#229026=CARTESIAN_POINT('Ctrl Pts',(-71.4034209525978,-3.46420490272305,
125.652230150673));
#229027=CARTESIAN_POINT('Ctrl Pts',(-71.681868576411,-6.20712064554441,
130.93404194847));
#229028=CARTESIAN_POINT('Ctrl Pts',(-71.9603162002238,-3.24599574981168,
136.09668293845));
#229029=CARTESIAN_POINT('Ctrl Pts',(-72.2387638240367,2.69804066428979,
136.395938259856));
#229030=CARTESIAN_POINT('Ctrl Pts',(-72.5172114478495,6.16270951452303,
131.556806891751));
#229031=CARTESIAN_POINT('Ctrl Pts',(-72.7956590716624,3.96414938600637,
126.026214156713));
#229032=CARTESIAN_POINT('Ctrl Pts',(-73.0741066954753,-1.87727036878649,
124.886504593767));
#229033=CARTESIAN_POINT('Ctrl Pts',(-73.3525543192881,-5.99357036442037,
129.185015613353));
#229034=CARTESIAN_POINT('Ctrl Pts',(-73.6310019431012,-4.60207199734241,
134.971625582408));
#229035=CARTESIAN_POINT('Ctrl Pts',(-73.909449566914,1.01850571157763,136.928722630985));
#229036=CARTESIAN_POINT('Ctrl Pts',(-74.187897190727,5.70312642832773,133.257830180947));
#229037=CARTESIAN_POINT('Ctrl Pts',(-74.4663448145398,5.14685257066011,
127.332319060812));
#229038=CARTESIAN_POINT('Ctrl Pts',(-74.7447924383527,-0.139127361718492,
124.597444512675));
#229039=CARTESIAN_POINT('Ctrl Pts',(-75.0232400621657,-5.29725604542678,
127.566422640223));
#229040=CARTESIAN_POINT('Ctrl Pts',(-75.3016876859784,-5.58746520873256,
133.510907586884));
#229041=CARTESIAN_POINT('Ctrl Pts',(-75.5801353097915,-0.743066808063574,
136.968208090913));
#229042=CARTESIAN_POINT('Ctrl Pts',(-75.8585829336042,4.7841736883842,134.761233887624));
#229043=CARTESIAN_POINT('Ctrl Pts',(-76.1370305574171,5.91499228508486,
128.918086453158));
#229044=CARTESIAN_POINT('Ctrl Pts',(-76.41547818123,1.61022193523031,124.808332826166));
#229045=CARTESIAN_POINT('Ctrl Pts',(-76.693925805043,-4.17426370938676,
126.208635817229));
#229046=CARTESIAN_POINT('Ctrl Pts',(-76.9723734288558,-6.12280492919574,
131.832185386163));
#229047=CARTESIAN_POINT('Ctrl Pts',(-77.2508210526686,-2.44478753472383,
136.511214204787));
#229048=CARTESIAN_POINT('Ctrl Pts',(-77.5292686764817,3.47987016964863,
135.945923372052));
#229049=CARTESIAN_POINT('Ctrl Pts',(-77.8077163002943,6.20669718922256,
130.655787547247));
#229050=CARTESIAN_POINT('Ctrl Pts',(-78.0861639241075,3.22987270591563,
125.502183115868));
#229051=CARTESIAN_POINT('Ctrl Pts',(-78.3646115479203,-2.71504700607423,
125.221020782777));
#229052=CARTESIAN_POINT('Ctrl Pts',(-78.6430591717333,-6.16497115690175,
130.070674996542));
#229053=CARTESIAN_POINT('Ctrl Pts',(-78.921506795546,-3.94958799012119,
135.594550453492));
#229054=CARTESIAN_POINT('Ctrl Pts',(-79.199954419359,1.89527359148086,136.71647546501));
#229055=CARTESIAN_POINT('Ctrl Pts',(-79.4784020431719,5.9984713317742,132.405455754592));
#229056=CARTESIAN_POINT('Ctrl Pts',(-79.7568496669848,4.58936695978296,
126.623107831093));
#229057=CARTESIAN_POINT('Ctrl Pts',(-80.0352972907976,-1.0371414452086,
124.683126952807));
#229058=CARTESIAN_POINT('Ctrl Pts',(-80.3137449146107,-5.71056752923021,
128.368260773546));
#229059=CARTESIAN_POINT('Ctrl Pts',(-80.5921925384234,-5.13626103062165,
134.292051340844));
#229060=CARTESIAN_POINT('Ctrl Pts',(-80.8706401622364,0.158018434826916,
137.010824516613));
#229061=CARTESIAN_POINT('Ctrl Pts',(-81.1490877860493,5.30708667829958,
134.026160571776));
#229062=CARTESIAN_POINT('Ctrl Pts',(-81.4275354098621,5.57920153001237,
128.080819862696));
#229063=CARTESIAN_POINT('Ctrl Pts',(-81.705983033675,0.724302734791404,
124.63828005498));
#229064=CARTESIAN_POINT('Ctrl Pts',(-81.984430657488,-4.79619488954742,
126.862067054498));
#229065=CARTESIAN_POINT('Ctrl Pts',(-82.2628782813007,-5.90922371753823,
132.708629246728));
#229066=CARTESIAN_POINT('Ctrl Pts',(-82.5413259051138,-1.59196463073914,
136.805261597452));
#229067=CARTESIAN_POINT('Ctrl Pts',(-82.8197735289264,4.18823217991362,
135.387359107972));
#229068=CARTESIAN_POINT('Ctrl Pts',(-83.0982211527395,6.11964822374235,
129.757904897731));
#229069=CARTESIAN_POINT('Ctrl Pts',(-83.3766687765523,2.42740651138818,
125.090092371815));
#229070=CARTESIAN_POINT('Ctrl Pts',(-83.6551164003652,-3.49550319953123,
125.67341320622));
#229071=CARTESIAN_POINT('Ctrl Pts',(-83.9335640241781,-6.20621623490623,
130.971824050937));
#229072=CARTESIAN_POINT('Ctrl Pts',(-84.2120116479911,-3.21371974092037,
136.116344181428));
#229073=CARTESIAN_POINT('Ctrl Pts',(-84.4904592718038,2.73202819603347,
136.379410921554));
#229074=CARTESIAN_POINT('Ctrl Pts',(-84.7689068956169,6.16717568783019,
131.519278788663));
#229075=CARTESIAN_POINT('Ctrl Pts',(-85.0473545194296,3.9349900057924,126.002171782228));
#229076=CARTESIAN_POINT('Ctrl Pts',(-85.3258021432425,-1.91325925661942,
124.898041715501));
#229077=CARTESIAN_POINT('Ctrl Pts',(-85.6042497670555,-6.00331673010926,
129.221530180052));
#229078=CARTESIAN_POINT('Ctrl Pts',(-85.8826973908683,-4.57661940695503,
134.999562491112));
#229079=CARTESIAN_POINT('Ctrl Pts',(-86.1611450146813,1.05576757090286,
136.922409227389));
#229080=CARTESIAN_POINT('Ctrl Pts',(-86.4395926384942,5.71795572821454,
133.223068174528));
#229081=CARTESIAN_POINT('Ctrl Pts',(-86.718040262307,5.12562190896342,127.301053037252));
#229082=CARTESIAN_POINT('Ctrl Pts',(-86.9964878861199,-0.176908044074368,
124.598406420195));
#229083=CARTESIAN_POINT('Ctrl Pts',(-87.2749355099329,-5.31686814704595,
127.598728532803));
#229084=CARTESIAN_POINT('Ctrl Pts',(-87.5533831337457,-5.57088616633168,
133.544869927476));
#229085=CARTESIAN_POINT('Ctrl Pts',(-87.8318307575586,-0.70553195167748,
136.972617147663));
#229086=CARTESIAN_POINT('Ctrl Pts',(-88.1102783813713,4.80817165941601,
134.732037952774));
#229087=CARTESIAN_POINT('Ctrl Pts',(-88.3887260051845,5.90340040775061,
128.882115164534));
#229088=CARTESIAN_POINT('Ctrl Pts',(-88.6671736289971,1.57369257850503,
124.798642040718));
#229089=CARTESIAN_POINT('Ctrl Pts',(-88.9456212528103,-4.20216185122988,
126.234130893362));
#229090=CARTESIAN_POINT('Ctrl Pts',(-89.2240688766231,-6.11643482670397,
131.869437594414));
#229091=CARTESIAN_POINT('Ctrl Pts',(-89.5025165004358,-2.41000300088966,
136.525990585645));
#229092=CARTESIAN_POINT('Ctrl Pts',(-89.7809641242489,3.51110384754994,
135.924645153375));
#229093=CARTESIAN_POINT('Ctrl Pts',(-90.0594117480617,6.20567778705031,
130.618008372501));
#229094=CARTESIAN_POINT('Ctrl Pts',(-90.3378593718745,3.19753700446471,
125.482620201028));
#229095=CARTESIAN_POINT('Ctrl Pts',(-90.6163069956876,-2.74898407685696,
125.237651490881));
#229096=CARTESIAN_POINT('Ctrl Pts',(-90.8947546195002,-6.16932308688508,
130.108216519297));
#229097=CARTESIAN_POINT('Ctrl Pts',(-91.1732022433134,-3.92035556825405,
135.618503965492));
#229098=CARTESIAN_POINT('Ctrl Pts',(-91.4516498671261,1.93122719758584,
136.70482885892));
#229099=CARTESIAN_POINT('Ctrl Pts',(-91.7300974909391,6.00810651453776,
132.368911692441));
#229100=CARTESIAN_POINT('Ctrl Pts',(-92.0085451147519,4.56382945695037,
126.595248520721));
#229101=CARTESIAN_POINT('Ctrl Pts',(-92.2869927385648,-1.07438391611076,
124.689553739443));
#229102=CARTESIAN_POINT('Ctrl Pts',(-92.5654403623776,-5.72529095683809,
128.403067754236));
#229103=CARTESIAN_POINT('Ctrl Pts',(-92.8438879861907,-5.11493530424405,
134.323252600751));
#229104=CARTESIAN_POINT('Ctrl Pts',(-93.1223356100035,0.195796014469281,
137.009747622148));
#229105=CARTESIAN_POINT('Ctrl Pts',(-93.4007832338166,5.32660036105212,
133.993795136343));
#229106=CARTESIAN_POINT('Ctrl Pts',(-93.6792308576291,5.56251919472255,
128.046908140318));
#229107=CARTESIAN_POINT('Ctrl Pts',(-93.9576784814422,0.686754632612129,
124.633985261843));
#229108=CARTESIAN_POINT('Ctrl Pts',(-94.2361261052551,-4.82010388703947,
126.891335895681));
#229109=CARTESIAN_POINT('Ctrl Pts',(-94.5145737290679,-5.8975224096676,
132.744565087048));
#229110=CARTESIAN_POINT('Ctrl Pts',(-94.7930213528811,-1.55540594779807,
136.814841155217));
#229111=CARTESIAN_POINT('Ctrl Pts',(-95.0714689766937,4.21605259429308,
135.361779237583));
#229112=CARTESIAN_POINT('Ctrl Pts',(-95.3499166005066,6.11316476784841,
129.720672250431));
#229113=CARTESIAN_POINT('Ctrl Pts',(-95.6283642243196,2.39257716445285,
125.075421931555));
#229114=CARTESIAN_POINT('Ctrl Pts',(-95.9068118481323,-3.52667196918255,
125.694786390909));
#229115=CARTESIAN_POINT('Ctrl Pts',(-96.1852594719453,-6.20508185064282,
131.009599947983));
#229116=CARTESIAN_POINT('Ctrl Pts',(-96.4637070957582,-3.18132464646333,
136.135808586901));
#229117=CARTESIAN_POINT('Ctrl Pts',(-96.742154719571,2.76591449146702,136.362676997713));
#229118=CARTESIAN_POINT('Ctrl Pts',(-97.020602343384,6.17141333417382,131.481724194021));
#229119=CARTESIAN_POINT('Ctrl Pts',(-97.299049967197,3.90568481307747,125.978307354616));
#229120=CARTESIAN_POINT('Ctrl Pts',(-97.5774975910097,-1.94917724792726,
124.909797698053));
#229121=CARTESIAN_POINT('Ctrl Pts',(-97.8559452148228,-6.01284064068852,
129.258103399115));
#229122=CARTESIAN_POINT('Ctrl Pts',(-98.1343928386354,-4.55099722825276,
135.027343945068));
#229123=CARTESIAN_POINT('Ctrl Pts',(-98.4128404624484,1.09299030837272,
136.915869117251));
#229124=CARTESIAN_POINT('Ctrl Pts',(-98.6912880862614,5.73257314714861,
133.188216542011));
#229125=CARTESIAN_POINT('Ctrl Pts',(-98.9697357100741,5.10420131546234,
127.269916830042));
#229126=CARTESIAN_POINT('Ctrl Pts',(-99.2481833338871,-0.214682171037078,
124.599598291628));
#229127=CARTESIAN_POINT('Ctrl Pts',(-99.5266309576999,-5.33628323016052,
127.631153211259));
#229128=CARTESIAN_POINT('Ctrl Pts',(-99.8050785815131,-5.55410069269506,
133.578730717485));
#229129=CARTESIAN_POINT('Ctrl Pts',(-100.083526205326,-0.667970951546107,
136.976797637399));
#229130=CARTESIAN_POINT('Ctrl Pts',(-100.361973829139,4.83199146187865,
134.702696476397));
#229131=CARTESIAN_POINT('Ctrl Pts',(-100.640421452952,5.89158977774298,
128.846215105423));
#229132=CARTESIAN_POINT('Ctrl Pts',(-100.918869076765,1.53710490802326,
124.789173799381));
#229133=CARTESIAN_POINT('Ctrl Pts',(-101.197316700577,-4.22990428042106,
126.259795321038));
#229134=CARTESIAN_POINT('Ctrl Pts',(-101.47576432439,-6.10983807746976,
131.906650335846));
#229135=CARTESIAN_POINT('Ctrl Pts',(-101.754211948203,-2.37512916350784,
136.540554949401));
#229136=CARTESIAN_POINT('Ctrl Pts',(-102.032659572016,3.54220742020778,
135.903177200671));
#229137=CARTESIAN_POINT('Ctrl Pts',(-102.311107195829,6.20442843120499,
130.580236103105));
#229138=CARTESIAN_POINT('Ctrl Pts',(-102.589554819642,3.16508281710451,
125.463254485237));
#229139=CARTESIAN_POINT('Ctrl Pts',(-102.868002443455,-2.78281928302352,
125.254488475437));
#229140=CARTESIAN_POINT('Ctrl Pts',(-103.146450067268,-6.1734464103326,
130.145783837928));
#229141=CARTESIAN_POINT('Ctrl Pts',(-103.424897691081,-3.8909778761698,
135.642279087639));
#229142=CARTESIAN_POINT('Ctrl Pts',(-103.703345314893,1.96710924135641,
136.69296360881));
#229143=CARTESIAN_POINT('Ctrl Pts',(-103.981792938706,6.01751906470488,
132.332309655276));
#229144=CARTESIAN_POINT('Ctrl Pts',(-104.260240562519,4.53812283973896,
126.567545180546));
#229145=CARTESIAN_POINT('Ctrl Pts',(-104.538688186332,-1.11158657532129,
124.696207112496));
#229146=CARTESIAN_POINT('Ctrl Pts',(-104.817135810145,-5.73980223168479,
128.437963715717));
#229147=CARTESIAN_POINT('Ctrl Pts',(-105.095583433958,-5.093420042057,134.354323466822));
#229148=CARTESIAN_POINT('Ctrl Pts',(-105.374031057771,0.233566338818549,
137.008440784786));
#229149=CARTESIAN_POINT('Ctrl Pts',(-105.652478681584,5.34591666467016,
133.961311515241));
#229150=CARTESIAN_POINT('Ctrl Pts',(-105.930926305397,5.54563073823764,
128.013098596357));
#229151=CARTESIAN_POINT('Ctrl Pts',(-106.20937392921,0.649181082487974,
124.629919114234));
#229152=CARTESIAN_POINT('Ctrl Pts',(-106.487821553022,-4.84383427380942,
126.920749735436));
#229153=CARTESIAN_POINT('Ctrl Pts',(-106.766269176835,-5.88560256693534,
132.780429032376));
#229154=CARTESIAN_POINT('Ctrl Pts',(-107.044716800648,-1.51878962871805,
136.824197992414));
#229155=CARTESIAN_POINT('Ctrl Pts',(-107.323164424461,4.2437167812931,135.336030490371));
#229156=CARTESIAN_POINT('Ctrl Pts',(-107.601612048274,6.10645478638612,
129.683479759601));
#229157=CARTESIAN_POINT('Ctrl Pts',(-107.880059672087,2.35765915969063,
125.060963779225));
#229158=CARTESIAN_POINT('Ctrl Pts',(-108.1585072959,-3.55771005670707,125.716348912751));
#229159=CARTESIAN_POINT('Ctrl Pts',(-108.436954919713,-6.20371753478999,
131.04736823981));
#229160=CARTESIAN_POINT('Ctrl Pts',(-108.715402543526,-3.14881166685081,
136.155075433609));
#229161=CARTESIAN_POINT('Ctrl Pts',(-108.993850167338,2.79969829492213,
136.345737108415));
#229162=CARTESIAN_POINT('Ctrl Pts',(-109.272297791151,6.17542229652738,
131.444144499421));
#229163=CARTESIAN_POINT('Ctrl Pts',(-109.550745414964,3.87623489377466,
125.954621758183));
#229164=CARTESIAN_POINT('Ctrl Pts',(-109.829193038777,-1.98502301175461,
124.921772105802));
#229165=CARTESIAN_POINT('Ctrl Pts',(-110.10764066259,-6.02214174324697,
129.294733915307));
#229166=CARTESIAN_POINT('Ctrl Pts',(-110.386088286403,-4.52520641067474,
135.054968914823));
#229167=CARTESIAN_POINT('Ctrl Pts',(-110.664535910216,1.13017254468408,
136.909102542919));
#229168=CARTESIAN_POINT('Ctrl Pts',(-110.942983534029,5.74697814347679,
133.153276574838));
#229169=CARTESIAN_POINT('Ctrl Pts',(-111.221431157841,5.08259158390449,
127.238911592946));
#229170=CARTESIAN_POINT('Ctrl Pts',(-111.499878781655,-0.252448342873548,
124.601020082813));
#229171=CARTESIAN_POINT('Ctrl Pts',(-111.778326405467,-5.3555005753377,
127.663695474083));
#229172=CARTESIAN_POINT('Ctrl Pts',(-112.05677402928,-5.53710940981492,
133.612488702192));
#229173=CARTESIAN_POINT('Ctrl Pts',(-112.335221653093,-0.630385199504834,
136.980749405212));
#229174=CARTESIAN_POINT('Ctrl Pts',(-112.613669276906,4.85563221312083,
134.673210545752));
#229175=CARTESIAN_POINT('Ctrl Pts',(-112.892116900719,5.8795608327098,128.810387606114));
#229176=CARTESIAN_POINT('Ctrl Pts',(-113.170564524532,1.50046027955312,
124.779928453004));
#229177=CARTESIAN_POINT('Ctrl Pts',(-113.449012148345,-4.25748996895278,
126.285628149252));
#229178=CARTESIAN_POINT('Ctrl Pts',(-113.727459772158,-6.10301492593933,
131.943822231527));
#229179=CARTESIAN_POINT('Ctrl Pts',(-114.00590739597,-2.3401673148416,136.554906756366));
#229180=CARTESIAN_POINT('Ctrl Pts',(-114.284355019783,3.57317973506622,
135.881520309444));
#229181=CARTESIAN_POINT('Ctrl Pts',(-114.562802643596,6.202949167983,130.542472138726));
#229182=CARTESIAN_POINT('Ctrl Pts',(-114.841250267409,3.13251134643626,
125.444086686097));
#229183=CARTESIAN_POINT('Ctrl Pts',(-115.119697891222,-2.81655137079845,
125.271531112549));
#229184=CARTESIAN_POINT('Ctrl Pts',(-115.398145515035,-6.17734097445314,
130.183375560363));
#229185=CARTESIAN_POINT('Ctrl Pts',(-115.676593138848,-3.86145600246928,
135.665874938939));
#229186=CARTESIAN_POINT('Ctrl Pts',(-115.955040762661,2.00291839317105,
136.680880154352));
#229187=CARTESIAN_POINT('Ctrl Pts',(-116.233488386474,6.02670863349017,
132.295650999397));
#229188=CARTESIAN_POINT('Ctrl Pts',(-116.511936010287,4.51224806071678,
126.539998837124));
#229189=CARTESIAN_POINT('Ctrl Pts',(-116.790383634099,-1.14874804428301,
124.703086825424));
#229190=CARTESIAN_POINT('Ctrl Pts',(-117.068831257912,-5.75410081604829,
128.472947364906));
#229191=CARTESIAN_POINT('Ctrl Pts',(-117.347278881725,-5.07171604131793,
134.385262787713));
#229192=CARTESIAN_POINT('Ctrl Pts',(-117.625726505538,0.271328008281021,
137.006904052952));
#229193=CARTESIAN_POINT('Ctrl Pts',(-117.904174129351,5.3650348733795,133.928710912162));
#229194=CARTESIAN_POINT('Ctrl Pts',(-118.182621753164,5.52853678636705,
127.979392483636));
#229195=CARTESIAN_POINT('Ctrl Pts',(-118.461069376977,0.611583476719488,
124.626081762825));
#229196=CARTESIAN_POINT('Ctrl Pts',(-118.73951700079,-4.86738517051901,
126.95030748382));
#229197=CARTESIAN_POINT('Ctrl Pts',(-119.017964624603,-5.87346463103546,
132.816219753764));
#229198=CARTESIAN_POINT('Ctrl Pts',(-119.296412248415,-1.48211703032935,
136.833331762325));
#229199=CARTESIAN_POINT('Ctrl Pts',(-119.574859872228,4.27122371580729,
135.310113820466));
#229200=CARTESIAN_POINT('Ctrl Pts',(-119.853307496041,6.09951852799569,
129.646328803424));
#229201=CARTESIAN_POINT('Ctrl Pts',(-120.131755119854,2.32265379100196,
125.046718450578));
#229202=CARTESIAN_POINT('Ctrl Pts',(-120.410202743667,-3.58861631197691,
125.738099972737));
#229203=CARTESIAN_POINT('Ctrl Pts',(-120.68865036748,-6.20212333790203,
131.085127526901));
#229204=CARTESIAN_POINT('Ctrl Pts',(-120.967097991293,-3.11618200686478,
136.174144007612));
#229205=CARTESIAN_POINT('Ctrl Pts',(-121.245545615105,2.83337835452712,
136.328591881372));
#229206=CARTESIAN_POINT('Ctrl Pts',(-121.523993238919,6.17920242633619,
131.406541097396));
#229207=CARTESIAN_POINT('Ctrl Pts',(-121.802440862731,3.84664133916317,
125.931115870606));
#229208=CARTESIAN_POINT('Ctrl Pts',(-122.080888486544,-2.02079521982502,
124.933964495032));
#229209=CARTESIAN_POINT('Ctrl Pts',(-122.359336110357,-6.03121969312815,
129.331420371272));
#229210=CARTESIAN_POINT('Ctrl Pts',(-122.63778373417,-4.49924790990888,
135.082436376724));
#229211=CARTESIAN_POINT('Ctrl Pts',(-122.916231357983,1.16731290203685,
136.90210975513));
#229212=CARTESIAN_POINT('Ctrl Pts',(-123.194678981796,5.76117018341619,
133.118249567719));
#229213=CARTESIAN_POINT('Ctrl Pts',(-123.473126605609,5.06079351504635,
127.208038474877));
#229214=CARTESIAN_POINT('Ctrl Pts',(-123.751574229422,-0.290205160143283,
124.602671741062));
#229215=CARTESIAN_POINT('Ctrl Pts',(-124.030021853235,-5.37451947047147,
127.696354115408));
#229216=CARTESIAN_POINT('Ctrl Pts',(-124.308469477047,-5.51991294730918,
133.646142630679));
#229217=CARTESIAN_POINT('Ctrl Pts',(-124.58691710086,-0.592776088308802,
136.984472304668));
#229218=CARTESIAN_POINT('Ctrl Pts',(-124.865364724673,4.87909303712557,
134.64358125345));
#229219=CARTESIAN_POINT('Ctrl Pts',(-125.143812348486,5.86731401838748,
128.774633994209));
#229220=CARTESIAN_POINT('Ctrl Pts',(-125.422259972299,1.46376005097626,
124.770906344175));
#229221=CARTESIAN_POINT('Ctrl Pts',(-125.700707596112,-4.28491789462882,
126.311628420759));
#229222=CARTESIAN_POINT('Ctrl Pts',(-125.979155219925,-6.09596562494584,
131.980951904039));
#229223=CARTESIAN_POINT('Ctrl Pts',(-126.257602843738,-2.30511875041471,
136.569045474729));
#229224=CARTESIAN_POINT('Ctrl Pts',(-126.536050467551,3.60401964443632,
135.859675282198));
#229225=CARTESIAN_POINT('Ctrl Pts',(-126.814498091363,6.20124005219796,
130.50471787872));
#229226=CARTESIAN_POINT('Ctrl Pts',(-127.092945715177,3.09982379940838,
125.42511751388));
#229227=CARTESIAN_POINT('Ctrl Pts',(-127.371393338989,-2.85017909022625,
125.288778770691));
#229228=CARTESIAN_POINT('Ctrl Pts',(-127.649840962802,-6.18100663493216,
130.220990293627));
#229229=CARTESIAN_POINT('Ctrl Pts',(-127.928288586615,-3.83179104109667,
135.689290645038));
#229230=CARTESIAN_POINT('Ctrl Pts',(-128.206736210428,2.03865332610762,
136.6685789433));
#229231=CARTESIAN_POINT('Ctrl Pts',(-128.485183834241,6.03567488037103,
132.258937083203));
#229232=CARTESIAN_POINT('Ctrl Pts',(-128.763631458054,4.48620607868298,
126.512610511197));
#229233=CARTESIAN_POINT('Ctrl Pts',(-129.042079081867,-1.18586694596332,
124.710192623294));
#229234=CARTESIAN_POINT('Ctrl Pts',(-129.32052670568,-5.76818618009069,
128.508017405469));
#229235=CARTESIAN_POINT('Ctrl Pts',(-129.598974329492,-5.04982410627509,
134.416069416958));
#229236=CARTESIAN_POINT('Ctrl Pts',(-129.877421953305,0.30907962358457,
137.005137483589));
#229237=CARTESIAN_POINT('Ctrl Pts',(-130.155869577118,5.38395427874936,
133.895994535135));
#229238=CARTESIAN_POINT('Ctrl Pts',(-130.434317200931,5.51123797253198,
127.945791051148));
#229239=CARTESIAN_POINT('Ctrl Pts',(-130.712764824744,0.573963208500954,
124.622473349811));
#229240=CARTESIAN_POINT('Ctrl Pts',(-130.991212448557,-4.89075570448117,
126.980008045559));
#229241=CARTESIAN_POINT('Ctrl Pts',(-131.26966007237,-5.8611090517438,132.851935924971));
#229242=CARTESIAN_POINT('Ctrl Pts',(-131.548107696183,-1.44538951154951,
136.842242126491));
#229243=CARTESIAN_POINT('Ctrl Pts',(-131.826555319995,4.29857237855583,
135.28403018822));
#229244=CARTESIAN_POINT('Ctrl Pts',(-132.105002943808,6.09235624970348,
129.609220758541));
#229245=CARTESIAN_POINT('Ctrl Pts',(-132.383450567622,2.28756235552218,
125.032686473479));
#229246=CARTESIAN_POINT('Ctrl Pts',(-132.661898191434,-3.6193895897498,
125.760038764874));
#229247=CARTESIAN_POINT('Ctrl Pts',(-132.940345815247,-6.20029931905343,
131.122876410071));
#229248=CARTESIAN_POINT('Ctrl Pts',(-133.21879343906,-3.08343687560774,
136.193013602317));
#229249=CARTESIAN_POINT('Ctrl Pts',(-133.497241062873,2.86695342225543,
136.311241951909));
#229250=CARTESIAN_POINT('Ctrl Pts',(-133.775688686686,6.18275358352724,
131.368915381349));
#229251=CARTESIAN_POINT('Ctrl Pts',(-134.054136310499,3.81690524584148,
125.907790562906));
#229252=CARTESIAN_POINT('Ctrl Pts',(-134.332583934311,-2.05649254658467,
124.946374413949));
#229253=CARTESIAN_POINT('Ctrl Pts',(-134.611031558124,-6.04007415394596,
129.36816140758));
#229254=CARTESIAN_POINT('Ctrl Pts',(-134.889479181937,-4.47312268785726,
135.109745312956));
#229255=CARTESIAN_POINT('Ctrl Pts',(-135.16792680575,1.20441000418008,136.894891013003));
#229256=CARTESIAN_POINT('Ctrl Pts',(-135.446374429563,5.775148741076,133.083136818595));
#229257=CARTESIAN_POINT('Ctrl Pts',(-135.724822053376,5.03880791662344,
127.177298619846));
#229258=CARTESIAN_POINT('Ctrl Pts',(-136.003269677189,-0.327951223754644,
124.604553205172));
#229259=CARTESIAN_POINT('Ctrl Pts',(-136.281717301002,-5.39333921080989,
127.729127925058));
#229260=CARTESIAN_POINT('Ctrl Pts',(-136.560164924815,-5.50251194239939,
133.679691255889));
#229261=CARTESIAN_POINT('Ctrl Pts',(-136.838612548628,-0.555145011576188,
136.987966197812));
#229262=CARTESIAN_POINT('Ctrl Pts',(-137.117060172441,4.90237306454367,
134.613809697415));
#229263=CARTESIAN_POINT('Ctrl Pts',(-137.395507796253,5.8548497885868,128.73895559457));
#229264=CARTESIAN_POINT('Ctrl Pts',(-137.673955420066,1.42700558223168,
124.762107807213));
#229265=CARTESIAN_POINT('Ctrl Pts',(-137.952403043879,-4.3121870410957,
126.33779517211));
#229266=CARTESIAN_POINT('Ctrl Pts',(-138.230850667692,-6.08869043570493,
132.018037977528));
#229267=CARTESIAN_POINT('Ctrl Pts',(-138.509298291505,-2.26998476896503,
136.582970580575));
#229268=CARTESIAN_POINT('Ctrl Pts',(-138.787745915318,3.63472600553235,
135.837642928407));
#229269=CARTESIAN_POINT('Ctrl Pts',(-139.066193539131,6.1993011471828,130.466974722087));
#229270=CARTESIAN_POINT('Ctrl Pts',(-139.344641162943,3.06702138726935,
125.406347671494));
#229271=CARTESIAN_POINT('Ctrl Pts',(-139.623088786757,-2.88370119522,125.306230810748));
#229272=CARTESIAN_POINT('Ctrl Pts',(-139.901536410569,-6.18444325593727,
130.258626643894));
#229273=CARTESIAN_POINT('Ctrl Pts',(-140.179984034382,-3.80198409129777,
135.712525338258));
#229274=CARTESIAN_POINT('Ctrl Pts',(-140.458431658195,2.07431271599591,
136.656060431482));
#229275=CARTESIAN_POINT('Ctrl Pts',(-140.736879282008,6.04441747309895,
132.222169267145));
#229276=CARTESIAN_POINT('Ctrl Pts',(-141.015326905821,4.45999785863389,
126.485381217648));
#229277=CARTESIAN_POINT('Ctrl Pts',(-141.293774529634,-1.22294190490765,
124.717524242802));
#229278=CARTESIAN_POINT('Ctrl Pts',(-141.572222153447,-5.78205780187226,
128.543172537875));
#229279=CARTESIAN_POINT('Ctrl Pts',(-141.85066977726,-5.02774504814366,
134.446742213005));
#229280=CARTESIAN_POINT('Ctrl Pts',(-142.129117401072,0.346819785828787,
137.003141142159));
#229281=CARTESIAN_POINT('Ctrl Pts',(-142.407565024885,5.40267417971275,
133.863163596476));
#229282=CARTESIAN_POINT('Ctrl Pts',(-142.686012648698,5.49373493774783,
127.912295544006));
#229283=CARTESIAN_POINT('Ctrl Pts',(-142.964460272511,0.536321671864061,
124.619094008905));
#229284=CARTESIAN_POINT('Ctrl Pts',(-143.242907896324,-4.91394500969209,
127.00985032009));
#229285=CARTESIAN_POINT('Ctrl Pts',(-143.521355520137,-5.84853628690073,
132.887576222521));
#229286=CARTESIAN_POINT('Ctrl Pts',(-143.79980314395,-1.40860843332932,
136.850928754739));
#229287=CARTESIAN_POINT('Ctrl Pts',(-144.078250767763,4.32576175612421,
135.257780560169));
#229288=CARTESIAN_POINT('Ctrl Pts',(-144.356698391576,6.08496821690962,
129.572157000006));
#229289=CARTESIAN_POINT('Ctrl Pts',(-144.635146015388,2.2523861535788,125.018868367886));
#229290=CARTESIAN_POINT('Ctrl Pts',(-144.913593639201,-3.65002874971022,
125.782164476213));
#229291=CARTESIAN_POINT('Ctrl Pts',(-145.192041263014,-6.19824554583293,
131.160613490521));
#229292=CARTESIAN_POINT('Ctrl Pts',(-145.470488886827,-3.05057748646412,
136.211683518503));
#229293=CARTESIAN_POINT('Ctrl Pts',(-145.74893651064,2.90042225397064,136.293687962933));
#229294=CARTESIAN_POINT('Ctrl Pts',(-146.027384134453,6.18607563651005,
131.33126874552));
#229295=CARTESIAN_POINT('Ctrl Pts',(-146.305831758266,3.78702771569254,
125.884646699409));
#229296=CARTESIAN_POINT('Ctrl Pts',(-146.584279382079,-2.09211366925746,
124.959001402698));
#229297=CARTESIAN_POINT('Ctrl Pts',(-146.862727005891,-6.04870479759444,
129.404955662777));
#229298=CARTESIAN_POINT('Ctrl Pts',(-147.141174629705,-4.4468317125993,
135.136894711575));
#229299=CARTESIAN_POINT('Ctrl Pts',(-147.419622253517,1.24146247646836,
136.887446584034));
#229300=CARTESIAN_POINT('Ctrl Pts',(-147.69806987733,5.78891329847519,133.04793962858));
#229301=CARTESIAN_POINT('Ctrl Pts',(-147.976517501143,5.01663560332014,
127.146693166932));
#229302=CARTESIAN_POINT('Ctrl Pts',(-148.254965124956,-0.365685135012239,
124.606664405427));
#229303=CARTESIAN_POINT('Ctrl Pts',(-148.533412748769,-5.41195909898036,
127.762015688586));
#229304=CARTESIAN_POINT('Ctrl Pts',(-148.811860372582,-5.48490703988586,
133.713133334664));
#229305=CARTESIAN_POINT('Ctrl Pts',(-149.090307996395,-0.517493363741682,
136.991230955176));
#229306=CARTESIAN_POINT('Ctrl Pts',(-149.368755620208,4.92547143272535,
134.583896980843));
#229307=CARTESIAN_POINT('Ctrl Pts',(-149.647203244021,5.84216860517359,
128.703353729273));
#229308=CARTESIAN_POINT('Ctrl Pts',(-149.925650867833,1.39019823527075,
124.753533168151));
#229309=CARTESIAN_POINT('Ctrl Pts',(-150.204098491647,-4.33929639788676,
126.364127433687));
#229310=CARTESIAN_POINT('Ctrl Pts',(-150.482546115459,-6.08118962780021,
132.055079077756));
#229311=CARTESIAN_POINT('Ctrl Pts',(-150.760993739272,-2.23476667239474,
136.596681557904));
#229312=CARTESIAN_POINT('Ctrl Pts',(-151.039441363085,3.66529768052036,
135.81542406449));
#229313=CARTESIAN_POINT('Ctrl Pts',(-151.317888986898,6.19713252478332,
130.429244067412));
#229314=CARTESIAN_POINT('Ctrl Pts',(-151.596336610711,3.03410532552526,
125.387777854462));
#229315=CARTESIAN_POINT('Ctrl Pts',(-151.874784234524,-2.91711644360522,
125.323886586026));
#229316=CARTESIAN_POINT('Ctrl Pts',(-152.153231858337,-6.18765071012318,
130.296283216534));
#229317=CARTESIAN_POINT('Ctrl Pts',(-152.431679482149,-3.77203625758034,
135.735578157629));
#229318=CARTESIAN_POINT('Ctrl Pts',(-152.710127105962,2.10989524146327,
136.643325082775));
#229319=CARTESIAN_POINT('Ctrl Pts',(-152.988574729775,6.0529360877152,132.185348913665));
#229320=CARTESIAN_POINT('Ctrl Pts',(-153.267022353588,4.43362437172323,
126.458311965469));
#229321=CARTESIAN_POINT('Ctrl Pts',(-153.545469977401,-1.25997154729018,
124.725081412269));
#229322=CARTESIAN_POINT('Ctrl Pts',(-153.823917601214,-5.79571516737629,
128.578411459437));
#229323=CARTESIAN_POINT('Ctrl Pts',(-154.102365225027,-5.00547968506979,
134.477280039263));
#229324=CARTESIAN_POINT('Ctrl Pts',(-154.38081284884,0.38454709653853,137.000915102638));
#229325=CARTESIAN_POINT('Ctrl Pts',(-154.659260472653,5.4211938825983,133.830219312748));
#229326=CARTESIAN_POINT('Ctrl Pts',(-154.937708096465,5.47602833059452,
127.8789072034));
#229327=CARTESIAN_POINT('Ctrl Pts',(-155.216155720278,0.498660261630971,
124.615943865326));
#229328=CARTESIAN_POINT('Ctrl Pts',(-155.494603344091,-4.93695222686361,
127.039833201595));
#229329=CARTESIAN_POINT('Ctrl Pts',(-155.773050967904,-5.83574680239484,
132.923139325752));
#229330=CARTESIAN_POINT('Ctrl Pts',(-156.051498591717,-1.37177515860606,
136.85939132518));
#229331=CARTESIAN_POINT('Ctrl Pts',(-156.32994621553,4.3527908409998,135.231365909006));
#229332=CARTESIAN_POINT('Ctrl Pts',(-156.608393839343,6.0773547033811,129.535138901228));
#229333=CARTESIAN_POINT('Ctrl Pts',(-156.886841463156,2.21712648863745,
125.005264645838));
#229334=CARTESIAN_POINT('Ctrl Pts',(-157.165289086968,-3.68053265651321,
125.804476286877));
#229335=CARTESIAN_POINT('Ctrl Pts',(-157.443736710782,-6.19596209434481,
131.19833736989));
#229336=CARTESIAN_POINT('Ctrl Pts',(-157.722184334594,-3.0176050570491,
136.230153064351));
#229337=CARTESIAN_POINT('Ctrl Pts',(-158.000631958407,2.93378360947182,
136.275930564914));
#229338=CARTESIAN_POINT('Ctrl Pts',(-158.27907958222,6.18916846218569,131.293602584915));
#229339=CARTESIAN_POINT('Ctrl Pts',(-158.557527206033,3.7570098558391,125.861685137721));
#229340=CARTESIAN_POINT('Ctrl Pts',(-158.835974829846,-2.12765726788813,
124.971844993383));
#229341=CARTESIAN_POINT('Ctrl Pts',(-159.114422453659,-6.05711130426257,
129.44180177344));
#229342=CARTESIAN_POINT('Ctrl Pts',(-159.392870077472,-4.42037595835707,
135.163883566548));
#229343=CARTESIAN_POINT('Ctrl Pts',(-159.671317701285,1.27846894590735,
136.879776744077));
#229344=CARTESIAN_POINT('Ctrl Pts',(-159.949765325097,5.80246334556346,
133.01265930192));
#229345=CARTESIAN_POINT('Ctrl Pts',(-160.22821294891,4.9942773967397,127.116223250229));
#229346=CARTESIAN_POINT('Ctrl Pts',(-160.506660572723,-0.403405495673234,
124.609005263594));
#229347=CARTESIAN_POINT('Ctrl Pts',(-160.785108196536,-5.43037844501628,
127.795016187323));
#229348=CARTESIAN_POINT('Ctrl Pts',(-161.063555820349,-5.46709889212507,
133.746467627798));
#229349=CARTESIAN_POINT('Ctrl Pts',(-161.342003444162,-0.479822539999598,
136.994266455786));
#229350=CARTESIAN_POINT('Ctrl Pts',(-161.620451067975,4.94838728575097,
134.553844212161));
#229351=CARTESIAN_POINT('Ctrl Pts',(-161.898898691787,5.82927093805496,
128.66782971756));
#229352=CARTESIAN_POINT('Ctrl Pts',(-162.177346315601,1.35333937400316,
124.745182744726));
#229353=CARTESIAN_POINT('Ctrl Pts',(-162.455793939413,-4.36624496045326,
126.390624229737));
#229354=CARTESIAN_POINT('Ctrl Pts',(-162.734241563226,-6.07346347917808,
132.092073832152));
#229355=CARTESIAN_POINT('Ctrl Pts',(-163.012689187039,-2.19946576572379,
136.61017789865));
#229356=CARTESIAN_POINT('Ctrl Pts',(-163.291136810852,3.69573353655413,
135.793019513774));
#229357=CARTESIAN_POINT('Ctrl Pts',(-163.569584434665,6.19473426535967,
130.391527312818));
#229358=CARTESIAN_POINT('Ctrl Pts',(-163.848032058478,3.0010768338922,125.369408750896));
#229359=CARTESIAN_POINT('Ctrl Pts',(-164.126479682291,-2.95042359716811,
125.341745442286));
#229360=CARTESIAN_POINT('Ctrl Pts',(-164.404927306104,-6.19062887863655,
130.333958616169));
#229361=CARTESIAN_POINT('Ctrl Pts',(-164.683374929917,-3.74194864967208,
135.758448248921));
#229362=CARTESIAN_POINT('Ctrl Pts',(-164.961822553729,2.14539958398697,
136.630373369092));
#229363=CARTESIAN_POINT('Ctrl Pts',(-165.240270177542,6.06123040855813,
132.148477387157));
#229364=CARTESIAN_POINT('Ctrl Pts',(-165.518717801355,4.40708659523179,
126.431403757722));
#229365=CARTESIAN_POINT('Ctrl Pts',(-165.797165425168,-1.29695450096345,
124.732863851664));
#229366=CARTESIAN_POINT('Ctrl Pts',(-166.075613048981,-5.80915777052276,
128.613732864363));
#229367=CARTESIAN_POINT('Ctrl Pts',(-166.354060672794,-4.98302884210618,
134.50768176414));
#229368=CARTESIAN_POINT('Ctrl Pts',(-166.632508296607,0.422260157714416,
136.998459447511));
#229369=CARTESIAN_POINT('Ctrl Pts',(-166.91095592042,5.43951270115045,133.797162904712));
#229370=CARTESIAN_POINT('Ctrl Pts',(-167.189403544233,5.45811880719792,
127.845627266545));
#229371=CARTESIAN_POINT('Ctrl Pts',(-167.467851168046,0.460980373357943,
124.613023035806));
#229372=CARTESIAN_POINT('Ctrl Pts',(-167.746298791858,-4.95977650345479,
127.069955579048));
#229373=CARTESIAN_POINT('Ctrl Pts',(-168.024746415672,-5.822741072145,132.958623916859));
#229374=CARTESIAN_POINT('Ctrl Pts',(-168.303194039484,-1.33489105224939,
136.867629524233));
#229375=CARTESIAN_POINT('Ctrl Pts',(-168.581641663297,4.37965863161014,
135.204787213532));
#229376=CARTESIAN_POINT('Ctrl Pts',(-168.86008928711,6.06951599123876,129.498167833929));
#229377=CARTESIAN_POINT('Ctrl Pts',(-169.138536910923,2.18178466725943,
124.991875811423));
#229378=CARTESIAN_POINT('Ctrl Pts',(-169.416984534736,-3.71090017982492,
125.826973370093));
#229379=CARTESIAN_POINT('Ctrl Pts',(-169.695432158549,-6.19344904920226,
131.236046650305));
#229380=CARTESIAN_POINT('Ctrl Pts',(-169.973879782361,-2.98452080916978,
136.248421555465));
#229381=CARTESIAN_POINT('Ctrl Pts',(-170.252327406175,2.96703625254325,
136.257970415857));
#229382=CARTESIAN_POINT('Ctrl Pts',(-170.530775029987,6.19203194594742,
131.25591829527));
#229383=CARTESIAN_POINT('Ctrl Pts',(-170.8092226538,3.72685277860365,125.838906728691));
#229384=CARTESIAN_POINT('Ctrl Pts',(-171.087670277614,-2.16312202539704,
124.984904710079));
#229385=CARTESIAN_POINT('Ctrl Pts',(-171.366117901426,-6.06529336244348,
129.478698374222));
#229386=CARTESIAN_POINT('Ctrl Pts',(-171.644565525239,-4.39375640545797,
135.190710877796));
#229387=CARTESIAN_POINT('Ctrl Pts',(-171.923013149052,1.31542804121008,
136.871881777341));
#229388=CARTESIAN_POINT('Ctrl Pts',(-172.201460772865,5.81579838023838,
132.977297145939));
#229389=CARTESIAN_POINT('Ctrl Pts',(-172.479908396678,4.97173412537368,
127.085889998814));
#229390=CARTESIAN_POINT('Ctrl Pts',(-172.75835602049,-0.441110907994683,
124.611575692932));
#229391=CARTESIAN_POINT('Ctrl Pts',(-173.036803644304,-5.4485965663818,
127.828128198426));
#229392=CARTESIAN_POINT('Ctrl Pts',(-173.315251268116,-5.44908815900415,
133.779692900072));
#229393=CARTESIAN_POINT('Ctrl Pts',(-173.593698891929,-0.442133936257506,
136.997072587158));
#229394=CARTESIAN_POINT('Ctrl Pts',(-173.872146515742,4.97111977446672,
134.523652504987));
#229395=CARTESIAN_POINT('Ctrl Pts',(-174.150594139555,5.81615726515733,
128.632384875785));
#229396=CARTESIAN_POINT('Ctrl Pts',(-174.429041763368,1.31643036424716,
124.737056846366));
#229397=CARTESIAN_POINT('Ctrl Pts',(-174.707489387181,-4.39303173020782,
126.417284578411));
#229398=CARTESIAN_POINT('Ctrl Pts',(-174.985937010994,-6.06551227613263,
132.129020869861));
#229399=CARTESIAN_POINT('Ctrl Pts',(-175.264384634806,-2.16408335703982,
136.623459102702));
#229400=CARTESIAN_POINT('Ctrl Pts',(-175.542832258619,3.72603244582337,
135.770430106468));
#229401=CARTESIAN_POINT('Ctrl Pts',(-175.821279882432,6.19210645777918,
130.353825855915));
#229402=CARTESIAN_POINT('Ctrl Pts',(-176.099727506245,2.96793713625374,
125.351241041473));
#229403=CARTESIAN_POINT('Ctrl Pts',(-176.378175130058,-2.98362142169932,
125.359806717758));
#229404=CARTESIAN_POINT('Ctrl Pts',(-176.656622753871,-6.19337765112022,
130.371651446723));
#229405=CARTESIAN_POINT('Ctrl Pts',(-176.935070377684,-3.71172238248064,
135.781134764673));
#229406=CARTESIAN_POINT('Ctrl Pts',(-177.213518001496,2.18082442793968,
136.617205770365));
#229407=CARTESIAN_POINT('Ctrl Pts',(-177.49196562531,6.06930012827989,132.111556053907));
#229408=CARTESIAN_POINT('Ctrl Pts',(-177.770413249122,4.38038551252508,
126.404657591498));
#229409=CARTESIAN_POINT('Ctrl Pts',(-178.048860872936,-1.33388939551094,
124.740871272604));
#229410=CARTESIAN_POINT('Ctrl Pts',(-178.327308496748,-5.82238511319243,
128.649135443807));
#229411=CARTESIAN_POINT('Ctrl Pts',(-178.605756120561,-4.96039335117553,
134.537946261091));
#229412=CARTESIAN_POINT('Ctrl Pts',(-178.884203744374,0.459957571884186,
136.995774267775));
#229413=CARTESIAN_POINT('Ctrl Pts',(-179.162651368187,5.45762995655925,
133.763995597288));
#229414=CARTESIAN_POINT('Ctrl Pts',(-179.441098991999,5.44000703120181,
127.812456966643));
#229415=CARTESIAN_POINT('Ctrl Pts',(-179.719546615813,0.423283403288203,
124.610331628578));
#229416=CARTESIAN_POINT('Ctrl Pts',(-179.997994239625,-4.98241699370369,
127.100216336253));
#229417=CARTESIAN_POINT('Ctrl Pts',(-180.276441863438,-5.80951957808352,
132.994028680947));
#229418=CARTESIAN_POINT('Ctrl Pts',(-180.554889487251,-1.29795748101432,
136.875643046625));
#229419=CARTESIAN_POINT('Ctrl Pts',(-180.833337111064,4.40636413235919,
135.178045458633));
#229420=CARTESIAN_POINT('Ctrl Pts',(-181.111784734877,6.06145237094964,
129.461245168083));
#229421=CARTESIAN_POINT('Ctrl Pts',(-181.39023235869,2.14636199904753,124.97870236077));
#229422=CARTESIAN_POINT('Ctrl Pts',(-181.668679982503,-3.74113019436597,
125.849654892224));
#229423=CARTESIAN_POINT('Ctrl Pts',(-181.947127606316,-6.19070650352801,
131.273739934436));
#229424=CARTESIAN_POINT('Ctrl Pts',(-182.225575230128,-2.95132596877351,
136.266488314898));
#229425=CARTESIAN_POINT('Ctrl Pts',(-182.504022853942,3.00017895099442,
136.239808181284));
#229426=CARTESIAN_POINT('Ctrl Pts',(-182.782470477755,6.19466598168877,
131.218217272988));
#229427=CARTESIAN_POINT('Ctrl Pts',(-183.060918101567,3.6965576014681,125.81631231638));
#229428=CARTESIAN_POINT('Ctrl Pts',(-183.33936572538,-2.19850662762309,
124.998180068855));
#229429=CARTESIAN_POINT('Ctrl Pts',(-183.617813349193,-6.07325066894868,
129.515644097905));
#229430=CARTESIAN_POINT('Ctrl Pts',(-183.896260973006,-4.36697404029963,
135.217375651221));
#229431=CARTESIAN_POINT('Ctrl Pts',(-184.174708596819,1.35233839284232,
136.863761976378));
#229432=CARTESIAN_POINT('Ctrl Pts',(-184.453156220632,5.8289179083658,132.941854470998));
#229433=CARTESIAN_POINT('Ctrl Pts',(-184.731603844444,4.94900662457131,
127.055694536694));
#229434=CARTESIAN_POINT('Ctrl Pts',(-185.010051468258,-0.478799974789776,
124.614375598192));
#229435=CARTESIAN_POINT('Ctrl Pts',(-185.28849909207,-5.46661278799793,
127.861350494915));
#229436=CARTESIAN_POINT('Ctrl Pts',(-185.566946715884,-5.43087550791776,
133.812807920317));
#229437=CARTESIAN_POINT('Ctrl Pts',(-185.845394339696,-0.404428949079144,
136.999649245311));
#229438=CARTESIAN_POINT('Ctrl Pts',(-186.123841963509,4.99366805651034,
134.493322978084));
#229439=CARTESIAN_POINT('Ctrl Pts',(-186.402289587322,5.80282807241402,
128.59702051737));
#229440=CARTESIAN_POINT('Ctrl Pts',(-186.680737211135,1.27947257368013,
124.729155774178));
#229441=CARTESIAN_POINT('Ctrl Pts',(-186.959184834948,-4.41965571455532,
126.444107491802));
#229442=CARTESIAN_POINT('Ctrl Pts',(-187.237632458761,-6.0573363132998,
132.165918821797));
#229443=CARTESIAN_POINT('Ctrl Pts',(-187.516080082574,-2.12862075745111,
136.636524677919));
#229444=CARTESIAN_POINT('Ctrl Pts',(-187.794527706387,3.75619328558978,
135.74765667963));
#229445=CARTESIAN_POINT('Ctrl Pts',(-188.072975330199,6.18924919941703,
130.316141093742));
#229446=CARTESIAN_POINT('Ctrl Pts',(-188.351422954013,2.93468746061294,
125.333275399398));
#229447=CARTESIAN_POINT('Ctrl Pts',(-188.629870577825,-3.01670868704181,
125.378069743179));
#229448=CARTESIAN_POINT('Ctrl Pts',(-188.908318201638,-6.19589692571743,
130.409360311474));
#229449=CARTESIAN_POINT('Ctrl Pts',(-189.186765825451,-3.68135857605119,
135.80363686423));
#229450=CARTESIAN_POINT('Ctrl Pts',(-189.465213449264,2.21616846064164,
136.603822774524));
#229451=CARTESIAN_POINT('Ctrl Pts',(-189.743661073077,6.07714494785282,
132.07458628205));
#229452=CARTESIAN_POINT('Ctrl Pts',(-190.02210869689,4.35352211302309,126.378074457888));
#229453=CARTESIAN_POINT('Ctrl Pts',(-190.300556320702,-1.37077486229612,
124.749103378371));
#229454=CARTESIAN_POINT('Ctrl Pts',(-190.579003944516,-5.83539670523986,
128.684617885911));
#229455=CARTESIAN_POINT('Ctrl Pts',(-190.857451568328,-4.93757405104588,
134.568072408653));
#229456=CARTESIAN_POINT('Ctrl Pts',(-191.135899192141,0.497637942157669,
136.992859662928));
#229457=CARTESIAN_POINT('Ctrl Pts',(-191.414346815954,5.47554497748281,
133.730718619501));
#229458=CARTESIAN_POINT('Ctrl Pts',(-191.692794439767,5.42169367374449,
127.779397532831));
#229459=CARTESIAN_POINT('Ctrl Pts',(-191.97124206358,0.385570748295746,
124.60786974337));
#229460=CARTESIAN_POINT('Ctrl Pts',(-192.249689687393,-5.00487285865859,
127.130614351886));
#229461=CARTESIAN_POINT('Ctrl Pts',(-192.528137311206,-5.79608281013753,
133.029352306079));
#229462=CARTESIAN_POINT('Ctrl Pts',(-192.806584935019,-1.26097581348702,
136.883431595415));
#229463=CARTESIAN_POINT('Ctrl Pts',(-193.085032558831,4.43290635366497,
135.151141635234));
#229464=CARTESIAN_POINT('Ctrl Pts',(-193.363480182644,6.05316414131348,
129.424372271875));
#229465=CARTESIAN_POINT('Ctrl Pts',(-193.641927806457,2.11085979660312,
124.965744782026));
#229466=CARTESIAN_POINT('Ctrl Pts',(-193.92037543027,-3.77122157995168,
125.872520012798));
#229467=CARTESIAN_POINT('Ctrl Pts',(-194.198823054083,-6.1877345589472,
131.311415825543));
#229468=CARTESIAN_POINT('Ctrl Pts',(-194.477270677896,-2.91802176590892,
136.284352673182));
#229469=CARTESIAN_POINT('Ctrl Pts',(-194.755718301709,3.03321047671203,
136.221444534203));
#229470=CARTESIAN_POINT('Ctrl Pts',(-195.034165925522,6.19707047180361,
131.180500915096));
#229471=CARTESIAN_POINT('Ctrl Pts',(-195.312613549334,3.66612544703105,
125.793902738034));
#229472=CARTESIAN_POINT('Ctrl Pts',(-195.591061173148,-2.23380976337827,
125.011670577786));
#229473=CARTESIAN_POINT('Ctrl Pts',(-195.86950879696,-6.08098292891658,
129.552637575454));
#229474=CARTESIAN_POINT('Ctrl Pts',(-196.147956420774,-4.3400298553121,
135.243876898752));
#229475=CARTESIAN_POINT('Ctrl Pts',(-196.426404044586,1.38919863307876,
136.855417642068));
#229476=CARTESIAN_POINT('Ctrl Pts',(-196.704851668399,5.84182144379631,
132.906332590435));
#229477=CARTESIAN_POINT('Ctrl Pts',(-196.983299292212,4.92609573650846,
127.025637982775));
#229478=CARTESIAN_POINT('Ctrl Pts',(-197.261746916025,-0.516471299475173,
124.617404875624));
#229479=CARTESIAN_POINT('Ctrl Pts',(-197.540194539838,-5.48442644226676,
127.894681845726));
#229480=CARTESIAN_POINT('Ctrl Pts',(-197.81864216365,-5.41246161374207,
133.845811461438));
#229481=CARTESIAN_POINT('Ctrl Pts',(-198.097089787464,-0.36670897563802,
137.001996334766));
#229482=CARTESIAN_POINT('Ctrl Pts',(-198.375537411276,5.01603129634849,
134.462856755322));
#229483=CARTESIAN_POINT('Ctrl Pts',(-198.65398503509,5.78928385374183,128.561737952753));
#229484=CARTESIAN_POINT('Ctrl Pts',(-198.932432658902,1.24246737178614,
124.721479820939));
#229485=CARTESIAN_POINT('Ctrl Pts',(-199.210880282716,-4.44611592693577,
126.471091975977));
#229486=CARTESIAN_POINT('Ctrl Pts',(-199.489327906528,-6.04893589364168,
132.202766320694));
#229487=CARTESIAN_POINT('Ctrl Pts',(-199.767775530341,-2.09307928103787,
136.649374140152));
#229488=CARTESIAN_POINT('Ctrl Pts',(-200.046223154153,3.7862149382325,135.724700077139));
#229489=CARTESIAN_POINT('Ctrl Pts',(-200.324670777967,6.18616259614969,
130.278474422724));
#229490=CARTESIAN_POINT('Ctrl Pts',(-200.603118401779,2.90132903904936,
125.315512490399));
#229491=CARTESIAN_POINT('Ctrl Pts',(-200.881566025592,-3.04968416713424,
125.396533841802));
#229492=CARTESIAN_POINT('Ctrl Pts',(-201.160013649405,-6.1981866090755,
130.447083813107));
#229493=CARTESIAN_POINT('Ctrl Pts',(-201.438461273218,-3.65085835552605,
135.825953713766));
#229494=CARTESIAN_POINT('Ctrl Pts',(-201.716908897031,2.2514303724059,136.590224877478));
#229495=CARTESIAN_POINT('Ctrl Pts',(-201.995356520844,6.08476457658541,
132.037569441512));
#229496=CARTESIAN_POINT('Ctrl Pts',(-202.273804144657,4.32649739215744,
126.35165534194));
#229497=CARTESIAN_POINT('Ctrl Pts',(-202.55225176847,-1.40760953451491,
124.757559863922));
#229498=CARTESIAN_POINT('Ctrl Pts',(-202.830699392283,-5.84819206451709,
128.720178875862));
#229499=CARTESIAN_POINT('Ctrl Pts',(-203.109147016096,-4.91457178729319,
134.59805909049));
#229500=CARTESIAN_POINT('Ctrl Pts',(-203.387594639908,0.535299872273523,
136.989715740974));
#229501=CARTESIAN_POINT('Ctrl Pts',(-203.666042263721,5.49325710007376,
133.697333204442));
#229502=CARTESIAN_POINT('Ctrl Pts',(-203.944489887534,5.40317941343439,
127.746450190138));
#229503=CARTESIAN_POINT('Ctrl Pts',(-204.222937511347,0.347843805837959,
124.605637471411));
#229504=CARTESIAN_POINT('Ctrl Pts',(-204.50138513516,-5.0271432662092,127.161148499539));
#229505=CARTESIAN_POINT('Ctrl Pts',(-204.779832758973,-5.78243126621161,
133.064593483327));
#229506=CARTESIAN_POINT('Ctrl Pts',(-205.058280382786,-1.22394742003769,
136.890994881994));
#229507=CARTESIAN_POINT('Ctrl Pts',(-205.336728006599,4.45928431199552,
135.124076740266));
#229508=CARTESIAN_POINT('Ctrl Pts',(-205.615175630412,6.04465160945437,
129.387550511641));
#229509=CARTESIAN_POINT('Ctrl Pts',(-205.893623254225,2.07527937547198,
124.953003555339));
#229510=CARTESIAN_POINT('Ctrl Pts',(-206.172070878037,-3.80117322153507,
125.89556788454));
#229511=CARTESIAN_POINT('Ctrl Pts',(-206.45051850185,-6.18453332558722,
131.349072927534));
#229512=CARTESIAN_POINT('Ctrl Pts',(-206.728966125663,-2.8846094346739,
136.302013968343));
#229513=CARTESIAN_POINT('Ctrl Pts',(-207.007413749476,3.06612960569919,
136.202880155086));
#229514=CARTESIAN_POINT('Ctrl Pts',(-207.285861373289,6.19924532719362,
131.142770619188));
#229515=CARTESIAN_POINT('Ctrl Pts',(-207.564308997102,3.63555744296752,
125.771678824048));
#229516=CARTESIAN_POINT('Ctrl Pts',(-207.842756620915,-2.26903012449045,
125.025375736976));
#229517=CARTESIAN_POINT('Ctrl Pts',(-208.121204244728,-6.08848985582611,
129.58967743606));
#229518=CARTESIAN_POINT('Ctrl Pts',(-208.399651868541,-4.31292484892225,
135.270213638376));
#229519=CARTESIAN_POINT('Ctrl Pts',(-208.678099492353,1.42600739604885,
136.846849083615));
#229520=CARTESIAN_POINT('Ctrl Pts',(-208.956547116166,5.85450850838505,
132.870732820528));
#229521=CARTESIAN_POINT('Ctrl Pts',(-209.234994739979,4.90300231015654,
126.995721450812));
#229522=CARTESIAN_POINT('Ctrl Pts',(-209.513442363792,-0.554123486127181,
124.620663412976));
#229523=CARTESIAN_POINT('Ctrl Pts',(-209.791889987605,-5.50203686909699,
127.928121015754));
#229524=CARTESIAN_POINT('Ctrl Pts',(-210.070337611418,-5.393847158811,133.878702300482));
#229525=CARTESIAN_POINT('Ctrl Pts',(-210.348785235231,-0.328975413660277,
137.004113768549));
#229526=CARTESIAN_POINT('Ctrl Pts',(-210.627232859043,5.03820866530154,
134.432254965643));
#229527=CARTESIAN_POINT('Ctrl Pts',(-210.905680482857,5.77552511102812,
128.526538489345));
#229528=CARTESIAN_POINT('Ctrl Pts',(-211.184128106669,1.20541612980698,
124.714029271085));
#229529=CARTESIAN_POINT('Ctrl Pts',(-211.462575730482,-4.47241138685473,
126.498237031013));
#229530=CARTESIAN_POINT('Ctrl Pts',(-211.741023354295,-6.04031132844015,
132.239562001151));
#229531=CARTESIAN_POINT('Ctrl Pts',(-212.019470978108,-2.05746024480169,
136.66200701326));
#229532=CARTESIAN_POINT('Ctrl Pts',(-212.297918601921,3.81609629128846,
135.701561149659));
#229533=CARTESIAN_POINT('Ctrl Pts',(-212.576366225734,6.1828467623524,130.240827238612));
#229534=CARTESIAN_POINT('Ctrl Pts',(-212.854813849547,2.86786310767097,
125.297952972686));
#229535=CARTESIAN_POINT('Ctrl Pts',(-213.133261473359,-3.0825466400586,
125.415198329437));
#229536=CARTESIAN_POINT('Ctrl Pts',(-213.411709097173,-6.20024661634941,
130.484820553763));
#229537=CARTESIAN_POINT('Ctrl Pts',(-213.690156720985,-3.62022285110177,
135.848084486325));
#229538=CARTESIAN_POINT('Ctrl Pts',(-213.968604344798,2.28660885659016,
136.576412583105));
#229539=CARTESIAN_POINT('Ctrl Pts',(-214.247051968611,6.09215873212836,
132.00050690397));
#229540=CARTESIAN_POINT('Ctrl Pts',(-214.525499592424,4.29931235134063,
126.325401222624));
#229541=CARTESIAN_POINT('Ctrl Pts',(-214.803947216237,-1.44439204724454,
124.766240415898));
#229542=CARTESIAN_POINT('Ctrl Pts',(-215.08239484005,-5.86077071688603,
128.755817095934));
#229543=CARTESIAN_POINT('Ctrl Pts',(-215.360842463863,-4.89138741227638,
134.627905195436));
#229544=CARTESIAN_POINT('Ctrl Pts',(-215.639290087675,0.572941966656434,
136.986342618411));
#229545=CARTESIAN_POINT('Ctrl Pts',(-215.917737711489,5.51076566800256,
133.66384058922));
#229546=CARTESIAN_POINT('Ctrl Pts',(-216.196185335301,5.38446493632399,
127.713616159441));
#229547=CARTESIAN_POINT('Ctrl Pts',(-216.474632959115,0.310103973899474,
124.603634895418));
#229548=CARTESIAN_POINT('Ctrl Pts',(-216.753080582927,-5.04922739111732,
127.191817647757));
#229549=CARTESIAN_POINT('Ctrl Pts',(-217.031528206741,-5.76856545216855,
133.099750906814));
#229550=CARTESIAN_POINT('Ctrl Pts',(-217.309975830553,-1.18687367276612,
136.898332626102));
#229551=CARTESIAN_POINT('Ctrl Pts',(-217.588423454366,4.48549702990607,
135.096851776628));
#229552=CARTESIAN_POINT('Ctrl Pts',(-217.866871078179,6.03591509080661,
129.350781251827));
#229553=CARTESIAN_POINT('Ctrl Pts',(-218.145318701992,2.03962205410111,
124.94047915284));
#229554=CARTESIAN_POINT('Ctrl Pts',(-218.423766325804,-3.83098400924668,
125.9187976534));
#229555=CARTESIAN_POINT('Ctrl Pts',(-218.702213949618,-6.18110292207006,
131.386709845009));
#229556=CARTESIAN_POINT('Ctrl Pts',(-218.98066157343,-2.85109021317626,
136.319471545938));
#229557=CARTESIAN_POINT('Ctrl Pts',(-219.259109197243,3.09893511812703,
136.18411573184));
#229558=CARTESIAN_POINT('Ctrl Pts',(-219.537556821056,6.20119046726778,
131.105027783371));
#229559=CARTESIAN_POINT('Ctrl Pts',(-219.816004444869,3.6048547219858,125.749641397935));
#229560=CARTESIAN_POINT('Ctrl Pts',(-220.094452068682,-2.30416640585769,
125.039295038577));
#229561=CARTESIAN_POINT('Ctrl Pts',(-220.372899692494,-6.09577117150464,
129.626762307198));
#229562=CARTESIAN_POINT('Ctrl Pts',(-220.651347316308,-4.28566002551621,
135.296384894171));
#229563=CARTESIAN_POINT('Ctrl Pts',(-220.929794940121,1.46276331779004,
136.83805661853));
#229564=CARTESIAN_POINT('Ctrl Pts',(-221.208242563933,5.86697863200795,
132.835056480438));
#229565=CARTESIAN_POINT('Ctrl Pts',(-221.486690187747,4.87972720125093,
126.965946049375));
#229566=CARTESIAN_POINT('Ctrl Pts',(-221.765137811559,-0.591755139529082,
124.624151089502));
#229567=CARTESIAN_POINT('Ctrl Pts',(-222.043585435373,-5.51944341592756,
127.961666765899));
#229568=CARTESIAN_POINT('Ctrl Pts',(-222.322033059185,-5.37503283288975,
133.911479218663));
#229569=CARTESIAN_POINT('Ctrl Pts',(-222.600480682998,-0.29122966137826,
137.006001468201));
#229570=CARTESIAN_POINT('Ctrl Pts',(-222.878928306811,5.06019934158045,
134.401518743003));
#229571=CARTESIAN_POINT('Ctrl Pts',(-223.157375930624,5.7615523541068,128.491423431472));
#229572=CARTESIAN_POINT('Ctrl Pts',(-223.435823554437,1.16832022068962,
124.706804400699));
#229573=CARTESIAN_POINT('Ctrl Pts',(-223.71427117825,-4.49854111992577,
126.525541651043));
#229574=CARTESIAN_POINT('Ctrl Pts',(-223.992718802062,-6.03146293728042,
132.276304499695));
#229575=CARTESIAN_POINT('Ctrl Pts',(-224.271166425875,-2.02176496861996,
136.674422829126));
#229576=CARTESIAN_POINT('Ctrl Pts',(-224.549614049688,3.84583623749284,
135.678240754614));
#229577=CARTESIAN_POINT('Ctrl Pts',(-224.828061673501,6.1793018208946,130.203200936436));
#229578=CARTESIAN_POINT('Ctrl Pts',(-225.106509297314,2.83429090657077,
125.280597496933));
#229579=CARTESIAN_POINT('Ctrl Pts',(-225.384956921127,-3.11529488808334,
125.434062514461));
#229580=CARTESIAN_POINT('Ctrl Pts',(-225.66340454494,-6.20207687120481,
130.522569135094));
#229581=CARTESIAN_POINT('Ctrl Pts',(-225.941852168753,-3.5894531979886,
135.87002836184));
#229582=CARTESIAN_POINT('Ctrl Pts',(-226.220299792565,2.32170260964191,
136.562386403224));
#229583=CARTESIAN_POINT('Ctrl Pts',(-226.498747416378,6.09932714048972,
131.963400042786));
#229584=CARTESIAN_POINT('Ctrl Pts',(-226.777195040191,4.27196799792278,
126.299313072794));
#229585=CARTESIAN_POINT('Ctrl Pts',(-227.055642664004,-1.48112103749588,
124.775144712639));
#229586=CARTESIAN_POINT('Ctrl Pts',(-227.334090287817,-5.87313219624144,
128.79153122554));
#229587=CARTESIAN_POINT('Ctrl Pts',(-227.61253791163,-4.8680217850994,134.65760961753));
#229588=CARTESIAN_POINT('Ctrl Pts',(-227.890985535443,0.610562830463375,
136.982740420231));
#229589=CARTESIAN_POINT('Ctrl Pts',(-228.169433159256,5.52807003248314,
133.630242014917));
#229590=CARTESIAN_POINT('Ctrl Pts',(-228.447880783069,5.36555093588535,
127.680896657417));
#229591=CARTESIAN_POINT('Ctrl Pts',(-228.726328406882,0.272352650944771,
124.601862089598));
#229592=CARTESIAN_POINT('Ctrl Pts',(-229.004776030695,-5.07112441504767,
127.222620660081));
#229593=CARTESIAN_POINT('Ctrl Pts',(-229.283223654507,-5.75448588181141,
133.134823273769));
#229594=CARTESIAN_POINT('Ctrl Pts',(-229.561671278321,-1.14975594545406,
136.905444555836));
#229595=CARTESIAN_POINT('Ctrl Pts',(-229.840118902133,4.51154353607471,
135.069467753152));
#229596=CARTESIAN_POINT('Ctrl Pts',(-230.118566525947,6.0269549091058,129.314065854931));
#229597=CARTESIAN_POINT('Ctrl Pts',(-230.397014149759,2.00388915378425,
124.928172038625));
#229598=CARTESIAN_POINT('Ctrl Pts',(-230.675461773572,-3.86065283843716,
125.942208458593));
#229599=CARTESIAN_POINT('Ctrl Pts',(-230.953909397385,-6.17744347551146,
131.424325183319));
#229600=CARTESIAN_POINT('Ctrl Pts',(-231.232357021197,-2.81746534348149,
136.33672475907));
#229601=CARTESIAN_POINT('Ctrl Pts',(-231.510804645011,3.13162579837364,
136.165151959792));
#229602=CARTESIAN_POINT('Ctrl Pts',(-231.789252268823,6.20290581994918,
131.067273806224));
#229603=CARTESIAN_POINT('Ctrl Pts',(-232.067699892636,3.57401842178686,
125.727791276302));
#229604=CARTESIAN_POINT('Ctrl Pts',(-232.346147516449,-2.33921730549066,
125.053427966802));
#229605=CARTESIAN_POINT('Ctrl Pts',(-232.624595140262,-6.10282660614105,
129.663890814674));
#229606=CARTESIAN_POINT('Ctrl Pts',(-232.903042764075,-4.25823639540172,
135.322389696357));
#229607=CARTESIAN_POINT('Ctrl Pts',(-233.181490387888,1.499465036299,136.829040572621));
#229608=CARTESIAN_POINT('Ctrl Pts',(-233.459938011701,5.87923135258013,
132.799304892167));
#229609=CARTESIAN_POINT('Ctrl Pts',(-233.738385635514,4.85627127225937,
126.9363128818));
#229610=CARTESIAN_POINT('Ctrl Pts',(-234.016833259326,-0.629364865227224,
124.627867775965));
#229611=CARTESIAN_POINT('Ctrl Pts',(-234.29528088314,-5.53664543775268,
127.99531785311));
#229612=CARTESIAN_POINT('Ctrl Pts',(-234.573728506952,-5.35601933315035,
133.944141001422));
#229613=CARTESIAN_POINT('Ctrl Pts',(-234.852176130765,-0.253473117473377,
137.007659363768));
#229614=CARTESIAN_POINT('Ctrl Pts',(-235.130623754578,5.08200251031112,
134.370649226346));
#229615=CARTESIAN_POINT('Ctrl Pts',(-235.409071378391,5.74736610074488,
128.456394080338));
#229616=CARTESIAN_POINT('Ctrl Pts',(-235.687519002204,1.13118101903705,
124.699805477501));
#229617=CARTESIAN_POINT('Ctrl Pts',(-235.965966626017,-4.52450415790052,
126.553004824284));
#229618=CARTESIAN_POINT('Ctrl Pts',(-236.24441424983,-6.0223910480441,132.312992454817));
#229619=CARTESIAN_POINT('Ctrl Pts',(-236.522861873642,-1.98599477519336,
136.686621127679));
#229620=CARTESIAN_POINT('Ctrl Pts',(-236.801309497456,3.87543367482126,
135.654739756147));
#229621=CARTESIAN_POINT('Ctrl Pts',(-237.079757121268,6.1755279031354,130.165596910454));
#229622=CARTESIAN_POINT('Ctrl Pts',(-237.358204745081,2.80061367977841,
125.263446706254));
#229623=CARTESIAN_POINT('Ctrl Pts',(-237.636652368894,-3.14792769771062,
125.453125697856));
#229624=CARTESIAN_POINT('Ctrl Pts',(-237.915099992707,-6.20367730582095,
130.560328158313));
#229625=CARTESIAN_POINT('Ctrl Pts',(-238.19354761652,-3.55855053636696,
135.891784527174));
#229626=CARTESIAN_POINT('Ctrl Pts',(-238.471995240333,2.35671033115007,
136.54814685758));
#229627=CARTESIAN_POINT('Ctrl Pts',(-238.750442864146,6.10626953604027,
131.92625023297));
#229628=CARTESIAN_POINT('Ctrl Pts',(-239.028890487959,4.24446534516054,
126.273391859158));
#229629=CARTESIAN_POINT('Ctrl Pts',(-239.307338111771,-1.51779514426229,
124.784272424193));
#229630=CARTESIAN_POINT('Ctrl Pts',(-239.585785735585,-5.88527604452282,
128.827319941278));
#229631=CARTESIAN_POINT('Ctrl Pts',(-239.864233359397,-4.84447577158576,
134.687171256065));
#229632=CARTESIAN_POINT('Ctrl Pts',(-240.14268098321,0.648161069640796,
136.978909279916));
#229633=CARTESIAN_POINT('Ctrl Pts',(-240.421128607023,5.54516955229552,
133.596538726537));
#229634=CARTESIAN_POINT('Ctrl Pts',(-240.699576230836,5.34643811298351,
127.648292896498));
#229635=CARTESIAN_POINT('Ctrl Pts',(-240.978023854649,0.234591235861842,
124.600319119639));
#229636=CARTESIAN_POINT('Ctrl Pts',(-241.256471478461,-5.09283352659785,
127.253556395099));
#229637=CARTESIAN_POINT('Ctrl Pts',(-241.534919102275,-5.74019307686353,
133.169809284574));
#229638=CARTESIAN_POINT('Ctrl Pts',(-241.813366726087,-1.11259561351327,
136.912330407661));
#229639=CARTESIAN_POINT('Ctrl Pts',(-242.0918143499,4.53742286533832,135.041925684563));
#229640=CARTESIAN_POINT('Ctrl Pts',(-242.370261973713,6.01777139637409,
129.277405681456));
#229641=CARTESIAN_POINT('Ctrl Pts',(-242.648709597526,1.96808199861856,
124.916082668738));
#229642=CARTESIAN_POINT('Ctrl Pts',(-242.927157221339,-3.89017860971679,
125.965799432623));
#229643=CARTESIAN_POINT('Ctrl Pts',(-243.205604845152,-6.1735551215127,
131.461917548614));
#229644=CARTESIAN_POINT('Ctrl Pts',(-243.484052468965,-2.78373607157309,
136.353772968415));
#229645=CARTESIAN_POINT('Ctrl Pts',(-243.762500092778,3.16420043507544,
136.145989541648));
#229646=CARTESIAN_POINT('Ctrl Pts',(-244.040947716591,6.20439132167383,
131.029510086731));
#229647=CARTESIAN_POINT('Ctrl Pts',(-244.319395340403,3.54304968502077,
125.706129268813));
#229648=CARTESIAN_POINT('Ctrl Pts',(-244.597842964216,-2.37418152456686,
125.067773997952));
#229649=CARTESIAN_POINT('Ctrl Pts',(-244.876290588029,-6.10965589829292,
129.701061582678));
#229650=CARTESIAN_POINT('Ctrl Pts',(-245.154738211842,-4.23065497477177,
135.348227081313));
#229651=CARTESIAN_POINT('Ctrl Pts',(-245.433185835655,1.53611119157916,
136.819801279981));
#229652=CARTESIAN_POINT('Ctrl Pts',(-245.711633459468,5.89126621607239,
132.763479380503));
#229653=CARTESIAN_POINT('Ctrl Pts',(-245.990081083281,4.83263539234992,
126.906823046158));
#229654=CARTESIAN_POINT('Ctrl Pts',(-246.268528707094,-0.666951269578287,
124.631813334641));
#229655=CARTESIAN_POINT('Ctrl Pts',(-246.546976330906,-5.55364229714491,
128.029073030433));
#229656=CARTESIAN_POINT('Ctrl Pts',(-246.825423954719,-5.33680736414475,
133.976686438464));
#229657=CARTESIAN_POINT('Ctrl Pts',(-247.103871578532,-0.215707181029578,
137.009087393821));
#229658=CARTESIAN_POINT('Ctrl Pts',(-247.382319202345,5.10361736357064,
134.339647559554));
#229659=CARTESIAN_POINT('Ctrl Pts',(-247.660766826158,5.73296687661779,
128.421451733968));
#229660=CARTESIAN_POINT('Ctrl Pts',(-247.939214449971,1.09399990105564,
124.693032760838));
#229661=CARTESIAN_POINT('Ctrl Pts',(-248.217662073784,-4.55029953871062,
126.580625533077));
#229662=CARTESIAN_POINT('Ctrl Pts',(-248.496109697597,-6.01309599689209,
132.349624507031));
#229663=CARTESIAN_POINT('Ctrl Pts',(-248.77455732141,-1.95015099000055,
136.698601456905));
#229664=CARTESIAN_POINT('Ctrl Pts',(-249.053004945222,3.90488750652966,
135.631059025098));
#229665=CARTESIAN_POINT('Ctrl Pts',(-249.331452569036,6.17152514891849,
130.128016554096));
#229666=CARTESIAN_POINT('Ctrl Pts',(-249.609900192848,2.76683267521693,
125.246501236177));
#229667=CARTESIAN_POINT('Ctrl Pts',(-249.888347816661,-3.18044385971988,
125.472387173231));
#229668=CARTESIAN_POINT('Ctrl Pts',(-250.166795440474,-6.20504786089197,
130.598096224241));
#229669=CARTESIAN_POINT('Ctrl Pts',(-250.445243064287,-3.5275160113489,
135.913352176149));
#229670=CARTESIAN_POINT('Ctrl Pts',(-250.7236906881,2.39163072389511,136.533694473816));
#229671=CARTESIAN_POINT('Ctrl Pts',(-251.002138311913,6.11298566151878,
131.889058851139));
#229672=CARTESIAN_POINT('Ctrl Pts',(-251.280585935725,4.21680541219097,
126.247638542206));
#229673=CARTESIAN_POINT('Ctrl Pts',(-251.559033559539,-1.5544130086051,
124.793623212388));
#229674=CARTESIAN_POINT('Ctrl Pts',(-251.837481183351,-5.89720181167361,
128.863181916876));
#229675=CARTESIAN_POINT('Ctrl Pts',(-252.115928807165,-4.82075024435922,
134.716589015834));
#229676=CARTESIAN_POINT('Ctrl Pts',(-252.394376430977,0.685735291195708,
136.974849339035));
#229677=CARTESIAN_POINT('Ctrl Pts',(-252.67282405479,5.56206359338632,133.562731973716));
#229678=CARTESIAN_POINT('Ctrl Pts',(-252.951271678603,5.32712717665345,
127.615806083426));
#229679=CARTESIAN_POINT('Ctrl Pts',(-253.229719302416,0.196821126400439,
124.599006045371));
#229680=CARTESIAN_POINT('Ctrl Pts',(-253.508166926229,-5.11435391846912,
127.284623701469));
#229681=CARTESIAN_POINT('Ctrl Pts',(-253.786614550041,-5.72568757235024,
133.204707652256));
#229682=CARTESIAN_POINT('Ctrl Pts',(-254.065062173855,-1.07539404373626,
136.918989908584));
#229683=CARTESIAN_POINT('Ctrl Pts',(-254.343509797667,4.56313403947717,
135.014226625117));
#229684=CARTESIAN_POINT('Ctrl Pts',(-254.621957421481,6.00836492926231,
129.240802026269));
#229685=CARTESIAN_POINT('Ctrl Pts',(-254.900405045293,1.9322018468105,124.904211611225));
#229686=CARTESIAN_POINT('Ctrl Pts',(-255.178852669106,-3.91956009939235,
125.989569474605));
#229687=CARTESIAN_POINT('Ctrl Pts',(-255.457300292919,-6.16943824888009,
131.499485975975));
#229688=CARTESIAN_POINT('Ctrl Pts',(-255.735747916732,-2.74990318521692,
136.370614733943));
#229689=CARTESIAN_POINT('Ctrl Pts',(-256.014195540545,3.19665694865877,
136.126630713714));
#229690=CARTESIAN_POINT('Ctrl Pts',(-256.292643164358,6.20564856486739,
130.991735142402));
#229691=CARTESIAN_POINT('Ctrl Pts',(-256.571090788171,3.51194654848645,
125.68466161966));
#229692=CARTESIAN_POINT('Ctrl Pts',(-256.849538411983,-2.40905189372645,
125.082322325773));
#229693=CARTESIAN_POINT('Ctrl Pts',(-257.127986035797,-6.11626988572704,
129.738292634474));
#229694=CARTESIAN_POINT('Ctrl Pts',(-257.406433659609,-4.20289584392431,
135.373859459261));
#229695=CARTESIAN_POINT('Ctrl Pts',(-257.684881283423,1.57266088340656,
136.810408252432));
#229696=CARTESIAN_POINT('Ctrl Pts',(-257.963328907235,5.90315744058412,
132.727450666138));
#229697=CARTESIAN_POINT('Ctrl Pts',(-258.241776531048,4.80867945501638,
126.87772425425));
#229698=CARTESIAN_POINT('Ctrl Pts',(-258.520224154861,-0.704246744852541,
124.635521896935));
#229699=CARTESIAN_POINT('Ctrl Pts',(-258.798671778674,-5.5709361272427,
128.063810879205));
#229700=CARTESIAN_POINT('Ctrl Pts',(-259.077119402487,-5.31644754243966,
134.007449313497));
#229701=CARTESIAN_POINT('Ctrl Pts',(-259.355567026299,-0.179733571114533,
137.013459703814));
#229702=CARTESIAN_POINT('Ctrl Pts',(-259.634014650113,5.12849404027147,
134.30227331953));
#229703=CARTESIAN_POINT('Ctrl Pts',(-259.866054336623,5.61428989304695,
129.384066440553));
#229704=CARTESIAN_POINT('Ctrl Pts',(-260.051696012132,3.39054283699284,
126.521203045511));
#229705=CARTESIAN_POINT('Ctrl Pts',(-260.144521813036,1.754921961264,125.780753115897));
#229706=CARTESIAN_POINT('Ctrl Pts',(-260.190939676638,0.892893391295023,
125.631947563271));
#229707=CARTESIAN_POINT('Ctrl Pts',(210.191733024964,-2.43880115184907,
125.780342085335));
#229708=CARTESIAN_POINT('Ctrl Pts',(210.145323348611,-3.27594855749458,
126.186716565447));
#229709=CARTESIAN_POINT('Ctrl Pts',(210.052505734956,-4.72940422381435,
127.426013481475));
#229710=CARTESIAN_POINT('Ctrl Pts',(209.866872246696,-6.15821517169733,
131.008352419918));
#229711=CARTESIAN_POINT('Ctrl Pts',(209.634832560185,-4.21099667891447,
135.892791108304));
#229712=CARTESIAN_POINT('Ctrl Pts',(209.356384936373,2.01508446636645,137.098708070195));
#229713=CARTESIAN_POINT('Ctrl Pts',(209.07793731256,6.37956871319657,132.510708806665));
#229714=CARTESIAN_POINT('Ctrl Pts',(208.799489688747,4.8866719183268,126.359661034021));
#229715=CARTESIAN_POINT('Ctrl Pts',(208.521042064934,-1.09954563679898,
124.290443595948));
#229716=CARTESIAN_POINT('Ctrl Pts',(208.242594441121,-6.07390144970816,
128.208589139036));
#229717=CARTESIAN_POINT('Ctrl Pts',(207.964146817309,-5.46739734855352,
134.511385201899));
#229718=CARTESIAN_POINT('Ctrl Pts',(207.685699193495,0.163779660617915,
137.407996874876));
#229719=CARTESIAN_POINT('Ctrl Pts',(207.407251569682,5.6442383477931,134.235982835808));
#229720=CARTESIAN_POINT('Ctrl Pts',(207.128803945869,5.93803043711477,127.910585036422));
#229721=CARTESIAN_POINT('Ctrl Pts',(206.850356322057,0.775002953389061,
124.244367681185));
#229722=CARTESIAN_POINT('Ctrl Pts',(206.571908698243,-5.10018277131114,
126.606494049502));
#229723=CARTESIAN_POINT('Ctrl Pts',(206.293461074431,-6.28856642889766,
132.82623846394));
#229724=CARTESIAN_POINT('Ctrl Pts',(206.015013450618,-1.69805588527783,
137.187984519302));
#229725=CARTESIAN_POINT('Ctrl Pts',(205.736565826805,4.45288036648484,135.683487507757));
#229726=CARTESIAN_POINT('Ctrl Pts',(205.458118202992,6.51183958365415,129.695313656966));
#229727=CARTESIAN_POINT('Ctrl Pts',(205.179670579179,2.58673502741873,124.726298504418));
#229728=CARTESIAN_POINT('Ctrl Pts',(204.901222955366,-3.71545195245463,
125.342726181157));
#229729=CARTESIAN_POINT('Ctrl Pts',(204.622775331554,-6.60332046735468,
130.978128730661));
#229730=CARTESIAN_POINT('Ctrl Pts',(204.344327707741,-3.42305986725146,
136.4538470632));
#229731=CARTESIAN_POINT('Ctrl Pts',(204.065880083927,2.90282542147133,136.737963244372));
#229732=CARTESIAN_POINT('Ctrl Pts',(203.787432460115,6.56115601364161,131.569388537382));
#229733=CARTESIAN_POINT('Ctrl Pts',(203.508984836302,4.1901047305044,125.69779051756));
#229734=CARTESIAN_POINT('Ctrl Pts',(203.230537212489,-2.03144808657932,
124.518880964767));
#229735=CARTESIAN_POINT('Ctrl Pts',(202.952089588676,-6.38619936200403,
129.116020142231));
#229736=CARTESIAN_POINT('Ctrl Pts',(202.673641964863,-4.87234540261322,
135.2646617407));
#229737=CARTESIAN_POINT('Ctrl Pts',(202.39519434105,1.1189559521872,137.314504502614));
#229738=CARTESIAN_POINT('Ctrl Pts',(202.116746717238,6.08199145217563,133.381843073553));
#229739=CARTESIAN_POINT('Ctrl Pts',(201.838299093424,5.45597392877388,127.080601183836));
#229740=CARTESIAN_POINT('Ctrl Pts',(201.559851469612,-0.183817095687214,
124.201312298284));
#229741=CARTESIAN_POINT('Ctrl Pts',(201.281403845799,-5.65468918935595,
127.389902241135));
#229742=CARTESIAN_POINT('Ctrl Pts',(201.002956221986,-5.92917816483575,
133.716212626452));
#229743=CARTESIAN_POINT('Ctrl Pts',(200.724508598173,-0.755042063338292,
137.366673267433));
#229744=CARTESIAN_POINT('Ctrl Pts',(200.44606097436,5.11294080853837,134.986689170007));
#229745=CARTESIAN_POINT('Ctrl Pts',(200.167613350547,6.2823808583988,128.763349450982));
#229746=CARTESIAN_POINT('Ctrl Pts',(199.889165726734,1.67861981076543,124.415599285115));
#229747=CARTESIAN_POINT('Ctrl Pts',(199.610718102921,-4.46771083782862,
125.938808675424));
#229748=CARTESIAN_POINT('Ctrl Pts',(199.332270479108,-6.50843348626435,
131.933222605136));
#229749=CARTESIAN_POINT('Ctrl Pts',(199.053822855296,-2.56822371547623,
136.890267516244));
#229750=CARTESIAN_POINT('Ctrl Pts',(198.775375231483,3.73205818513161,136.254661300547));
#229751=CARTESIAN_POINT('Ctrl Pts',(198.49692760767,6.60276093478139,130.610495019181));
#229752=CARTESIAN_POINT('Ctrl Pts',(198.218479983857,3.4058489481713,125.14448175187));
#229753=CARTESIAN_POINT('Ctrl Pts',(197.940032360044,-2.92087183683725,
124.879620661678));
#229754=CARTESIAN_POINT('Ctrl Pts',(197.661584736231,-6.56345409631434,
130.05930615131));
#229755=CARTESIAN_POINT('Ctrl Pts',(197.383137112418,-4.1745426838368,135.923660297497));
#229756=CARTESIAN_POINT('Ctrl Pts',(197.104689488605,2.05056951733907,137.083628129519));
#229757=CARTESIAN_POINT('Ctrl Pts',(196.826241864792,6.39130850797037,132.473255877329));
#229758=CARTESIAN_POINT('Ctrl Pts',(196.54779424098,4.85874721255563,126.329250411482));
#229759=CARTESIAN_POINT('Ctrl Pts',(196.269346617166,-1.13876540820057,
124.297652603739));
#229760=CARTESIAN_POINT('Ctrl Pts',(195.990898993354,-6.0898082506034,128.245401590344));
#229761=CARTESIAN_POINT('Ctrl Pts',(195.712451369541,-5.44461481437399,
134.544708910868));
#229762=CARTESIAN_POINT('Ctrl Pts',(195.434003745728,0.203913652044436,
137.406818876019));
#229763=CARTESIAN_POINT('Ctrl Pts',(195.155556121915,5.66505543396973,134.201592249669));
#229764=CARTESIAN_POINT('Ctrl Pts',(194.877108498102,5.92028802542049,127.874475717408));
#229765=CARTESIAN_POINT('Ctrl Pts',(194.59866087429,0.735065143658737,124.239780275557));
#229766=CARTESIAN_POINT('Ctrl Pts',(194.320213250476,-5.1256466951968,126.637613470433));
#229767=CARTESIAN_POINT('Ctrl Pts',(194.041765626664,-6.2761396229282,132.86448373661));
#229768=CARTESIAN_POINT('Ctrl Pts',(193.763318002851,-1.6591668436545,137.198201498994));
#229769=CARTESIAN_POINT('Ctrl Pts',(193.484870379038,4.48249921013125,135.656291847837));
#229770=CARTESIAN_POINT('Ctrl Pts',(193.206422755225,6.50496747206681,129.655694426079));
#229771=CARTESIAN_POINT('Ctrl Pts',(192.927975131412,2.54968841250072,124.710665118833));
#229772=CARTESIAN_POINT('Ctrl Pts',(192.649527507599,-3.74862973894988,
125.365444281348));
#229773=CARTESIAN_POINT('Ctrl Pts',(192.371079883787,-6.60214029104917,
131.018321851013));
#229774=CARTESIAN_POINT('Ctrl Pts',(192.092632259973,-3.38860644815819,
136.474579499726));
#229775=CARTESIAN_POINT('Ctrl Pts',(191.814184636161,2.93889117796205,136.720183001327));
#229776=CARTESIAN_POINT('Ctrl Pts',(191.535737012347,6.56569138435095,131.529434736241));
#229777=CARTESIAN_POINT('Ctrl Pts',(191.257289388535,4.15894196037717,125.672378777932));
#229778=CARTESIAN_POINT('Ctrl Pts',(190.978841764722,-2.06967194957323,
124.531363418996));
#229779=CARTESIAN_POINT('Ctrl Pts',(190.700394140909,-6.3963584469616,129.154926032595));
#229780=CARTESIAN_POINT('Ctrl Pts',(190.421946517096,-4.84510401107414,
135.294238450423));
#229781=CARTESIAN_POINT('Ctrl Pts',(190.143498893283,1.15856431450073,137.307572482581));
#229782=CARTESIAN_POINT('Ctrl Pts',(189.86505126947,6.09756863406271,133.344772510351));
#229783=CARTESIAN_POINT('Ctrl Pts',(189.586603645657,5.4332052617092,127.047458114672));
#229784=CARTESIAN_POINT('Ctrl Pts',(189.308156021844,-0.224008319322015,
124.202553584261));
#229785=CARTESIAN_POINT('Ctrl Pts',(189.029708398032,-5.67536919831109,
127.424387201254));
#229786=CARTESIAN_POINT('Ctrl Pts',(188.751260774218,-5.91134304125131,
133.752251266956));
#229787=CARTESIAN_POINT('Ctrl Pts',(188.472813150406,-0.71508141444371,
137.371147838333));
#229788=CARTESIAN_POINT('Ctrl Pts',(188.194365526593,5.13830509856852,134.955487759214));
#229789=CARTESIAN_POINT('Ctrl Pts',(187.91591790278,6.26984024615536,128.725144630756));
#229790=CARTESIAN_POINT('Ctrl Pts',(187.637470278967,1.63969850624965,124.405499418827));
#229791=CARTESIAN_POINT('Ctrl Pts',(187.359022655154,-4.49724605717418,
125.966095046791));
#229792=CARTESIAN_POINT('Ctrl Pts',(187.080575031341,-6.5014411967389,131.972820371883));
#229793=CARTESIAN_POINT('Ctrl Pts',(186.802127407528,-2.53112948956026,
136.905788265189));
#229794=CARTESIAN_POINT('Ctrl Pts',(186.523679783716,3.76516656597443,136.231842221641));
#229795=CARTESIAN_POINT('Ctrl Pts',(186.245232159903,6.60145848599114,130.570305731164));
#229796=CARTESIAN_POINT('Ctrl Pts',(185.96678453609,3.3713325565579,125.123854247073));
#229797=CARTESIAN_POINT('Ctrl Pts',(185.688336912277,-2.95688329360047,
124.897510609301));
#229798=CARTESIAN_POINT('Ctrl Pts',(185.409889288464,-6.5678678487195,130.099273563458));
#229799=CARTESIAN_POINT('Ctrl Pts',(185.131441664651,-4.14330270904733,
135.948977074923));
#229800=CARTESIAN_POINT('Ctrl Pts',(184.852994040838,2.08875520864929,137.071029390563));
#229801=CARTESIAN_POINT('Ctrl Pts',(184.574546417025,6.40134913096194,132.434319247607));
#229802=CARTESIAN_POINT('Ctrl Pts',(184.296098793212,4.831415925211,126.299756751549));
#229803=CARTESIAN_POINT('Ctrl Pts',(184.017651169399,-1.17835248801931,
124.304705146227));
#229804=CARTESIAN_POINT('Ctrl Pts',(183.739203545587,-6.10527253047917,
128.282519393244));
#229805=CARTESIAN_POINT('Ctrl Pts',(183.460755921774,-5.42174537657308,
134.577782526619));
#229806=CARTESIAN_POINT('Ctrl Pts',(183.182308297961,0.244100911417136,
137.405455267482));
#229807=CARTESIAN_POINT('Ctrl Pts',(182.903860674148,5.68563038680749,134.167044506474));
#229808=CARTESIAN_POINT('Ctrl Pts',(182.625413050335,5.90234329520773,127.838491527799));
#229809=CARTESIAN_POINT('Ctrl Pts',(182.346965426522,0.695091060812155,
124.23542735186));
#229810=CARTESIAN_POINT('Ctrl Pts',(182.068517802709,-5.15091590138369,
126.668891936874));
#229811=CARTESIAN_POINT('Ctrl Pts',(181.790070178896,-6.263482786439,132.902650210566));
#229812=CARTESIAN_POINT('Ctrl Pts',(181.511622555083,-1.62021497890189,
137.208182855437));
#229813=CARTESIAN_POINT('Ctrl Pts',(181.233174931271,4.51195124234396,135.628915707812));
#229814=CARTESIAN_POINT('Ctrl Pts',(180.954727307458,6.49785469294791,129.61611812487));
#229815=CARTESIAN_POINT('Ctrl Pts',(180.676279683645,2.51254711858197,124.695257343842));
#229816=CARTESIAN_POINT('Ctrl Pts',(180.397832059832,-3.78166851301026,
125.388364025079));
#229817=CARTESIAN_POINT('Ctrl Pts',(180.119384436019,-6.60071552592353,
131.058506988669));
#229818=CARTESIAN_POINT('Ctrl Pts',(179.840936812206,-3.35402743339335,
136.495101852955));
#229819=CARTESIAN_POINT('Ctrl Pts',(179.562489188393,2.97484801707599,136.702183530083));
#229820=CARTESIAN_POINT('Ctrl Pts',(179.28404156458,6.56998346925752,131.489454075275));
#229821=CARTESIAN_POINT('Ctrl Pts',(179.005593940767,4.12762507472721,125.647157201507));
#229822=CARTESIAN_POINT('Ctrl Pts',(178.727146316955,-2.10781911778238,
124.544078323705));
#229823=CARTESIAN_POINT('Ctrl Pts',(178.448698693142,-6.40628051373842,
129.193893042167));
#229824=CARTESIAN_POINT('Ctrl Pts',(178.170251069329,-4.81768308177075,
135.323648786705));
#229825=CARTESIAN_POINT('Ctrl Pts',(177.891803445516,1.19812974544141,137.300399483306));
#229826=CARTESIAN_POINT('Ctrl Pts',(177.613355821703,6.11291986848493,133.307607811431));
#229827=CARTESIAN_POINT('Ctrl Pts',(177.33490819789,5.41023526512845,127.014454258818));
#229828=CARTESIAN_POINT('Ctrl Pts',(177.056460574078,-0.264191242194762,
124.204039502676));
#229829=CARTESIAN_POINT('Ctrl Pts',(176.778012950264,-5.69583890440069,
127.458997407505));
#229830=CARTESIAN_POINT('Ctrl Pts',(176.499565326452,-5.89328887066216,
133.788180672302));
#229831=CARTESIAN_POINT('Ctrl Pts',(176.221117702638,-0.675094267951971,
137.375379074508));
#229832=CARTESIAN_POINT('Ctrl Pts',(175.942670078826,5.16347898681764,134.924132526884));
#229833=CARTESIAN_POINT('Ctrl Pts',(175.664222455013,6.25706730267374,128.687016856641));
#229834=CARTESIAN_POINT('Ctrl Pts',(175.3857748312,1.60071644210391,124.395636664696));
#229835=CARTESIAN_POINT('Ctrl Pts',(175.107327207387,-4.5266146294138,125.993560701866));
#229836=CARTESIAN_POINT('Ctrl Pts',(174.828879583574,-6.49420799391872,
132.012374840923));
#229837=CARTESIAN_POINT('Ctrl Pts',(174.550431959762,-2.49394147171037,
136.92108292349));
#229838=CARTESIAN_POINT('Ctrl Pts',(174.271984335948,3.79813542718566,136.208822025409));
#229839=CARTESIAN_POINT('Ctrl Pts',(173.993536712136,6.59991141772898,130.530125116137));
#229840=CARTESIAN_POINT('Ctrl Pts',(173.715089088322,3.33669123897678,125.103437235529));
#229841=CARTESIAN_POINT('Ctrl Pts',(173.43664146451,-2.99278518196597,124.915619437422));
#229842=CARTESIAN_POINT('Ctrl Pts',(173.158193840697,-6.5720382263662,130.139267102866));
#229843=CARTESIAN_POINT('Ctrl Pts',(172.879746216884,-4.11190920265221,
135.974103216695));
#229844=CARTESIAN_POINT('Ctrl Pts',(172.601298593071,2.12686350036709,137.058198437889));
#229845=CARTESIAN_POINT('Ctrl Pts',(172.322850969258,6.41115254960738,132.395322219168));
#229846=CARTESIAN_POINT('Ctrl Pts',(172.044403345445,4.80390560797255,126.270430011369));
#229847=CARTESIAN_POINT('Ctrl Pts',(171.765955721632,-1.21789590355323,
124.31199853584));
#229848=CARTESIAN_POINT('Ctrl Pts',(171.487508097819,-6.12051057723618,
128.319730643897));
#229849=CARTESIAN_POINT('Ctrl Pts',(171.209060474007,-5.39867503400336,
134.610716316833));
#229850=CARTESIAN_POINT('Ctrl Pts',(170.930612850193,0.284279125540913,
137.403847052956));
#229851=CARTESIAN_POINT('Ctrl Pts',(170.652165226381,5.70599465652041,134.13237215779));
#229852=CARTESIAN_POINT('Ctrl Pts',(170.373717602568,5.88417985149351,127.802617239562));
#229853=CARTESIAN_POINT('Ctrl Pts',(170.095269978755,0.655091221110643,
124.231317842401));
#229854=CARTESIAN_POINT('Ctrl Pts',(169.816822354942,-5.17599423848763,
126.700323644626));
#229855=CARTESIAN_POINT('Ctrl Pts',(169.538374731129,-6.25059385429175,
132.940738931629));
#229856=CARTESIAN_POINT('Ctrl Pts',(169.259927107316,-1.58120307648749,
137.217926915891));
#229857=CARTESIAN_POINT('Ctrl Pts',(168.981479483503,4.54123608254409,135.601360792124));
#229858=CARTESIAN_POINT('Ctrl Pts',(168.703031859691,6.49050113343381,129.576585854424));
#229859=CARTESIAN_POINT('Ctrl Pts',(168.424584235878,2.47531272130571,124.680075943919));
#229860=CARTESIAN_POINT('Ctrl Pts',(168.146136612065,-3.81456715595326,
125.411484460556));
#229861=CARTESIAN_POINT('Ctrl Pts',(167.867688988252,-6.59904616885666,
131.098682708838));
#229862=CARTESIAN_POINT('Ctrl Pts',(167.589241364439,-3.31932413390846,
136.515413333674));
#229863=CARTESIAN_POINT('Ctrl Pts',(167.310793740626,3.01069462210276,136.683965512842));
#229864=CARTESIAN_POINT('Ctrl Pts',(167.032346116813,6.57403210101054,131.449448027918));
#229865=CARTESIAN_POINT('Ctrl Pts',(166.753898493,4.09615523841214,125.622126727152));
#229866=CARTESIAN_POINT('Ctrl Pts',(166.475450869187,-2.14588817997888,
124.557025205477));
#229867=CARTESIAN_POINT('Ctrl Pts',(166.197003245374,-6.41596519343492,
129.232919728208));
#229868=CARTESIAN_POINT('Ctrl Pts',(165.918555621562,-4.79008363144905,
135.352891659104));
#229869=CARTESIAN_POINT('Ctrl Pts',(165.640107997748,1.23765077924384,137.292985770921));
#229870=CARTESIAN_POINT('Ctrl Pts',(165.361660373936,6.12804458641347,133.270350353765));
#229871=CARTESIAN_POINT('Ctrl Pts',(165.083212750123,5.38706479029029,126.981590839339));
#229872=CARTESIAN_POINT('Ctrl Pts',(164.80476512631,-0.304364375363971,
124.205769998417));
#229873=CARTESIAN_POINT('Ctrl Pts',(164.526317502497,-5.71609754908509,
127.493731577419));
#229874=CARTESIAN_POINT('Ctrl Pts',(164.247869878684,-5.8750163220866,133.823999511097));
#229875=CARTESIAN_POINT('Ctrl Pts',(163.969422254871,-0.635082105593798,
137.37936681918));
#229876=CARTESIAN_POINT('Ctrl Pts',(163.690974631059,5.18846154045405,134.892624634889));
#229877=CARTESIAN_POINT('Ctrl Pts',(163.412527007245,6.24406250126218,128.648967541478));
#229878=CARTESIAN_POINT('Ctrl Pts',(163.134079383433,1.56167506282176,124.386011388187));
#229879=CARTESIAN_POINT('Ctrl Pts',(162.85563175962,-4.55581546628373,126.021204622902));
#229880=CARTESIAN_POINT('Ctrl Pts',(162.577184135807,-6.48673414583306,
132.051884546553));
#229881=CARTESIAN_POINT('Ctrl Pts',(162.298736511994,-2.45666103994207,
136.936150924396));
#229882=CARTESIAN_POINT('Ctrl Pts',(162.020288888181,3.83096354709181,136.185601564872));
#229883=CARTESIAN_POINT('Ctrl Pts',(161.741841264368,6.59811978732212,130.489954663008));
#229884=CARTESIAN_POINT('Ctrl Pts',(161.463393640556,3.30192627907479,125.083231473798));
#229885=CARTESIAN_POINT('Ctrl Pts',(161.184946016742,-3.02857617157586,
124.933946475014));
#229886=CARTESIAN_POINT('Ctrl Pts',(160.90649839293,-6.57596507471956,130.179285287561));
#229887=CARTESIAN_POINT('Ctrl Pts',(160.628050769116,-4.08036332794952,
135.999037791754));
#229888=CARTESIAN_POINT('Ctrl Pts',(160.349603145304,2.16489298037573,137.045135746957));
#229889=CARTESIAN_POINT('Ctrl Pts',(160.07115552149,6.42071840063739,132.356266237063));
#229890=CARTESIAN_POINT('Ctrl Pts',(159.792707897678,4.77621728024515,126.241271277656));
#229891=CARTESIAN_POINT('Ctrl Pts',(159.514260273865,-1.25739418950663,
124.319532502318));
#229892=CARTESIAN_POINT('Ctrl Pts',(159.235812650052,-6.13552182622286,
128.357033963427));
#229893=CARTESIAN_POINT('Ctrl Pts',(158.957365026239,-5.37540464154493,
134.643509061136));
#229894=CARTESIAN_POINT('Ctrl Pts',(158.678917402427,0.324446805597038,
137.401994292032));
#229895=CARTESIAN_POINT('Ctrl Pts',(158.400469778613,5.72614748850293,134.097576488416));
#229896=CARTESIAN_POINT('Ctrl Pts',(158.122022154801,5.86579836733105,127.766854182028));
#229897=CARTESIAN_POINT('Ctrl Pts',(157.843574530988,0.615067106763091,
124.22745189946));
#229898=CARTESIAN_POINT('Ctrl Pts',(157.565126907175,-5.20088077722156,
126.731907428977));
#229899=CARTESIAN_POINT('Ctrl Pts',(157.286679283362,-6.23747330409059,
132.978748488409));
#229900=CARTESIAN_POINT('Ctrl Pts',(157.008231659549,-1.54213258201158,
137.227433319288));
#229901=CARTESIAN_POINT('Ctrl Pts',(156.729784035736,4.5703526455712,135.57362812183));
#229902=CARTESIAN_POINT('Ctrl Pts',(156.451336411923,6.48290706601333,129.537099079623));
#229903=CARTESIAN_POINT('Ctrl Pts',(156.172888788111,2.43798660040623,124.665121481617));
#229904=CARTESIAN_POINT('Ctrl Pts',(155.894441164297,-3.84732444870741,
125.434804731043));
#229905=CARTESIAN_POINT('Ctrl Pts',(155.615993540485,-6.59713228170722,
131.138847522794));
#229906=CARTESIAN_POINT('Ctrl Pts',(155.337545916672,-3.28449783564716,
136.535513189234));
#229907=CARTESIAN_POINT('Ctrl Pts',(155.059098292859,3.04642966473303,136.665529624679));
#229908=CARTESIAN_POINT('Ctrl Pts',(154.780650669046,6.57783712958646,131.409418076611));
#229909=CARTESIAN_POINT('Ctrl Pts',(154.502203045233,4.06453361755842,125.597288282381));
#229910=CARTESIAN_POINT('Ctrl Pts',(154.22375542142,-2.18387772549973,124.57020358456));
#229911=CARTESIAN_POINT('Ctrl Pts',(153.945307797607,-6.42541212718171,
129.272004644569));
#229912=CARTESIAN_POINT('Ctrl Pts',(153.666860173794,-4.76230668281685,
135.381965984011));
#229913=CARTESIAN_POINT('Ctrl Pts',(153.388412549982,1.27712595144142,137.285331620145));
#229914=CARTESIAN_POINT('Ctrl Pts',(153.109964926169,6.14294222739622,133.233001517943));
#229915=CARTESIAN_POINT('Ctrl Pts',(152.831517302356,5.36369469578529,126.948869073999));
#229916=CARTESIAN_POINT('Ctrl Pts',(152.553069678543,-0.344526230199219,
124.207745007359));
#229917=CARTESIAN_POINT('Ctrl Pts',(152.27462205473,-5.73614438167267,127.528588423912));
#229918=CARTESIAN_POINT('Ctrl Pts',(151.996174430917,-5.85652607262075,
133.859706456064));
#229919=CARTESIAN_POINT('Ctrl Pts',(151.717726807104,-0.595046410034728,
137.383110924578));
#229920=CARTESIAN_POINT('Ctrl Pts',(151.439279183291,5.21325183374003,134.860965250768));
#229921=CARTESIAN_POINT('Ctrl Pts',(151.160831559478,6.23082632381839,128.610998095198));
#229922=CARTESIAN_POINT('Ctrl Pts',(150.882383935665,1.52257581509584,124.376623945969));
#229923=CARTESIAN_POINT('Ctrl Pts',(150.603936311853,-4.58484748573611,
126.049025785542));
#229924=CARTESIAN_POINT('Ctrl Pts',(150.32548868804,-6.47901992942814,132.091348024725));
#229925=CARTESIAN_POINT('Ctrl Pts',(150.047041064227,-2.41928957569559,
136.950991709558));
#229926=CARTESIAN_POINT('Ctrl Pts',(149.768593440414,3.8636497092349,136.162181700472));
#229927=CARTESIAN_POINT('Ctrl Pts',(149.490145816601,6.59608366116008,130.449795860306));
#229928=CARTESIAN_POINT('Ctrl Pts',(149.211698192788,3.26703896508027,125.06323771061));
#229929=CARTESIAN_POINT('Ctrl Pts',(148.933250568975,-3.06425493618196,
124.95249104296));
#229930=CARTESIAN_POINT('Ctrl Pts',(148.654802945162,-6.57964824826877,
130.219326634649));
#229931=CARTESIAN_POINT('Ctrl Pts',(148.376355321349,-4.04866625388314,
136.02377987614));
#229932=CARTESIAN_POINT('Ctrl Pts',(148.097907697537,2.20284223947883,137.031841801807));
#229933=CARTESIAN_POINT('Ctrl Pts',(147.819460073724,6.43004632958585,132.317152748525));
#229934=CARTESIAN_POINT('Ctrl Pts',(147.541012449911,4.74835196802999,126.212281630895));
#229935=CARTESIAN_POINT('Ctrl Pts',(147.262564826098,-1.29684588225586,
124.327306766486));
#229936=CARTESIAN_POINT('Ctrl Pts',(146.984117202285,-6.15030572119196,
128.394427969547));
#229937=CARTESIAN_POINT('Ctrl Pts',(146.705669578472,-5.35193506149072,
134.676159544383));
#229938=CARTESIAN_POINT('Ctrl Pts',(146.427221954659,0.364602463157475,
137.399897053366));
#229939=CARTESIAN_POINT('Ctrl Pts',(146.148774330846,5.74608813598446,134.062658787717));
#229940=CARTESIAN_POINT('Ctrl Pts',(145.870326707034,5.84719952385297,127.731203680413));
#229941=CARTESIAN_POINT('Ctrl Pts',(145.59187908322,0.575020200877703,124.22382966629));
#229942=CARTESIAN_POINT('Ctrl Pts',(145.313431459408,-5.22557459540567,
126.76364211958));
#229943=CARTESIAN_POINT('Ctrl Pts',(145.034983835595,-6.22412162202233,
133.016677472446));
#229944=CARTESIAN_POINT('Ctrl Pts',(144.756536211782,-1.50300494324566,
137.236701713364));
#229945=CARTESIAN_POINT('Ctrl Pts',(144.478088587969,4.59929985250025,135.545718724575));
#229946=CARTESIAN_POINT('Ctrl Pts',(144.199640964156,6.47507277208744,129.497659263665));
#229947=CARTESIAN_POINT('Ctrl Pts',(143.921193340343,2.40057013901678,124.65039451108));
#229948=CARTESIAN_POINT('Ctrl Pts',(143.64274571653,-3.87993917743928,125.458323972397));
#229949=CARTESIAN_POINT('Ctrl Pts',(143.364298092718,-6.594973935395,131.178999942215));
#229950=CARTESIAN_POINT('Ctrl Pts',(143.085850468904,-3.2495498291107,136.555400674828));
#229951=CARTESIAN_POINT('Ctrl Pts',(142.807402845092,3.08205182079176,136.646876548744));
#229952=CARTESIAN_POINT('Ctrl Pts',(142.528955221279,6.58139841398854,131.369365704677));
#229953=CARTESIAN_POINT('Ctrl Pts',(142.250507597466,4.03276138391676,125.572642787588));
#229954=CARTESIAN_POINT('Ctrl Pts',(141.972059973653,-2.2217863466284,124.583612972623));
#229955=CARTESIAN_POINT('Ctrl Pts',(141.69361234984,-6.43462096491922,129.311146342943));
#229956=CARTESIAN_POINT('Ctrl Pts',(141.415164726027,-4.7343532651591,135.410870684068));
#229957=CARTESIAN_POINT('Ctrl Pts',(141.136717102214,1.31655379926713,137.277437314604));
#229958=CARTESIAN_POINT('Ctrl Pts',(140.858269478402,6.15761223939561,133.195562687939));
#229959=CARTESIAN_POINT('Ctrl Pts',(140.579821854588,5.34012584760095,126.916290175316));
#229960=CARTESIAN_POINT('Ctrl Pts',(140.301374230776,-0.384675318488256,
124.20996445632));
#229961=CARTESIAN_POINT('Ctrl Pts',(140.022926606963,-5.75597865932068,
127.563566655346));
#229962=CARTESIAN_POINT('Ctrl Pts',(139.74447898315,-5.83781880742758,133.895300184066));
#229963=CARTESIAN_POINT('Ctrl Pts',(139.466031359337,-0.554988664812238,
137.386611251964));
#229964=CARTESIAN_POINT('Ctrl Pts',(139.187583735524,5.23784894806212,134.829155547671));
#229965=CARTESIAN_POINT('Ctrl Pts',(138.909136111711,6.21735926081381,128.573109924773));
#229966=CARTESIAN_POINT('Ctrl Pts',(138.630688487898,1.48342014776303,124.367474685896));
#229967=CARTESIAN_POINT('Ctrl Pts',(138.352240864086,-4.61370961197883,
126.077023158863));
#229968=CARTESIAN_POINT('Ctrl Pts',(138.073793240272,-6.47106563055709,
132.130763813104));
#229969=CARTESIAN_POINT('Ctrl Pts',(137.79534561646,-2.38182846378423,136.965604729043));
#229970=CARTESIAN_POINT('Ctrl Pts',(137.516897992647,3.89619270241722,136.138563300043));
#229971=CARTESIAN_POINT('Ctrl Pts',(137.238450368834,6.59380311469226,130.409650196134));
#229972=CARTESIAN_POINT('Ctrl Pts',(136.960002745021,3.23203058975544,125.043456686844));
#229973=CARTESIAN_POINT('Ctrl Pts',(136.681555121208,-3.09982015369448,
124.971252454085));
#229974=CARTESIAN_POINT('Ctrl Pts',(136.403107497395,-6.58308761053252,
130.259389660389));
#229975=CARTESIAN_POINT('Ctrl Pts',(136.124659873582,-4.01681915499975,
136.048328553027));
#229976=CARTESIAN_POINT('Ctrl Pts',(135.846212249769,2.24070987145278,137.018317095051));
#229977=CARTESIAN_POINT('Ctrl Pts',(135.567764625956,6.43913599080291,132.277983202917));
#229978=CARTESIAN_POINT('Ctrl Pts',(135.289317002144,4.72031070388647,126.183462145311));
#229979=CARTESIAN_POINT('Ctrl Pts',(135.010869378331,-1.33624951990408,
124.335321040266));
#229980=CARTESIAN_POINT('Ctrl Pts',(134.732421754518,-6.16486171432077,
128.431911276607));
#229981=CARTESIAN_POINT('Ctrl Pts',(134.453974130705,-5.32826716351462,
134.708666556695));
#229982=CARTESIAN_POINT('Ctrl Pts',(134.175526506892,0.404744610239488,
137.397555414672));
#229983=CARTESIAN_POINT('Ctrl Pts',(133.897078883079,5.76581586005707,134.027620349581));
#229984=CARTESIAN_POINT('Ctrl Pts',(133.618631259266,5.82838401024617,127.695667055759));
#229985=CARTESIAN_POINT('Ctrl Pts',(133.340183635453,0.534951987407334,
124.220451277114));
#229986=CARTESIAN_POINT('Ctrl Pts',(133.06173601164,-5.25007477800144,126.795526540492));
#229987=CARTESIAN_POINT('Ctrl Pts',(132.783288387828,-6.21053930283845,
133.054524478268));
#229988=CARTESIAN_POINT('Ctrl Pts',(132.504840764015,-1.46382161007886,
137.245731754674));
#229989=CARTESIAN_POINT('Ctrl Pts',(132.226393140202,4.62807663068185,135.517633634551));
#229990=CARTESIAN_POINT('Ctrl Pts',(131.947945516389,6.46699854195874,129.458267868007));
#229991=CARTESIAN_POINT('Ctrl Pts',(131.669497892576,2.3630647236181,124.635895578019));
#229992=CARTESIAN_POINT('Ctrl Pts',(131.391050268763,-3.91241013359816,
125.482041313105));
#229993=CARTESIAN_POINT('Ctrl Pts',(131.11260264495,-6.59257120989826,131.219138479237));
#229994=CARTESIAN_POINT('Ctrl Pts',(130.834155021138,-3.2144814093103,136.575075053519));
#229995=CARTESIAN_POINT('Ctrl Pts',(130.555707397324,3.1175597702868,136.628006976231));
#229996=CARTESIAN_POINT('Ctrl Pts',(130.277259773512,6.58471582225214,131.329292396271));
#229997=CARTESIAN_POINT('Ctrl Pts',(129.998812149698,4.0008397148189,125.548191156024));
#229998=CARTESIAN_POINT('Ctrl Pts',(129.720364525886,-2.25961263864694,
124.59725287278));
#229999=CARTESIAN_POINT('Ctrl Pts',(129.441916902073,-6.44359136541048,
129.350343372922));
#230000=CARTESIAN_POINT('Ctrl Pts',(129.16346927826,-4.70622441430021,135.439604688201));
#230001=CARTESIAN_POINT('Ctrl Pts',(128.885021654447,1.35593286170785,137.269303146827));
#230002=CARTESIAN_POINT('Ctrl Pts',(128.606574030634,6.17205407880915,133.158035251063));
#230003=CARTESIAN_POINT('Ctrl Pts',(128.328126406821,5.31635911908928,126.883855350513));
#230004=CARTESIAN_POINT('Ctrl Pts',(128.049678783009,-0.424810152491945,
124.212428263054));
#230005=CARTESIAN_POINT('Ctrl Pts',(127.771231159195,-5.77559964706288,
127.598664975593));
#230006=CARTESIAN_POINT('Ctrl Pts',(127.492783535383,-5.81889521971155,
133.930779376167));
#230007=CARTESIAN_POINT('Ctrl Pts',(127.21433591157,-0.514910354280421,
137.389867671632));
#230008=CARTESIAN_POINT('Ctrl Pts',(126.935888287757,5.26225197196523,134.797196704317));
#230009=CARTESIAN_POINT('Ctrl Pts',(126.657440663944,6.20366181127538,128.535304434163));
#230010=CARTESIAN_POINT('Ctrl Pts',(126.378993040131,1.44420951175126,124.358563947));
#230011=CARTESIAN_POINT('Ctrl Pts',(126.100545416318,-4.64240077551519,
126.105195705413));
#230012=CARTESIAN_POINT('Ctrl Pts',(125.822097792505,-6.46287154396936,
132.170130451126));
#230013=CARTESIAN_POINT('Ctrl Pts',(125.543650168692,-2.34427909234318,
136.979989441362));
#230014=CARTESIAN_POINT('Ctrl Pts',(125.26520254488,3.92859132074607,136.114747238771));
#230015=CARTESIAN_POINT('Ctrl Pts',(124.986754921067,6.59127823242518,130.369519158099));
#230016=CARTESIAN_POINT('Ctrl Pts',(124.708307297254,3.19690245034852,125.023889135492));
#230017=CARTESIAN_POINT('Ctrl Pts',(124.429859673441,-3.13527050623128,
124.990230013179));
#230018=CARTESIAN_POINT('Ctrl Pts',(124.151412049628,-6.58628303406391,
130.299472880227));
#230019=CARTESIAN_POINT('Ctrl Pts',(123.872964425815,-3.98482321140548,
136.072682912751));
#230020=CARTESIAN_POINT('Ctrl Pts',(123.594516802002,2.2784944730983,137.004562127853));
#230021=CARTESIAN_POINT('Ctrl Pts',(123.316069178189,6.44798704746787,132.238759051683));
#230022=CARTESIAN_POINT('Ctrl Pts',(123.037621554376,4.6920945268939,126.154813888819));
#230023=CARTESIAN_POINT('Ctrl Pts',(122.759173930564,-1.37560364233486,
124.343575026687));
#230024=CARTESIAN_POINT('Ctrl Pts',(122.480726306751,-6.17918926623166,
128.46948249565));
#230025=CARTESIAN_POINT('Ctrl Pts',(122.202278682938,-5.30440182463932,
134.741028893516));
#230026=CARTESIAN_POINT('Ctrl Pts',(121.923831059125,0.444871759361186,
137.394969462721));
#230027=CARTESIAN_POINT('Ctrl Pts',(121.645383435312,5.78532992970255,133.992462472369));
#230028=CARTESIAN_POINT('Ctrl Pts',(121.366935811499,5.80935252372653,127.660245624887));
#230029=CARTESIAN_POINT('Ctrl Pts',(121.088488187686,0.494863951094175,
124.21731685712));
#230030=CARTESIAN_POINT('Ctrl Pts',(120.810040563873,-5.27438041714564,
126.827559510225));
#230031=CARTESIAN_POINT('Ctrl Pts',(120.53159294006,-6.19672684983677,133.092288103441));
#230032=CARTESIAN_POINT('Ctrl Pts',(120.253145316248,-1.42458403446405,
137.254523108609));
#230033=CARTESIAN_POINT('Ctrl Pts',(119.974697692435,4.65668191378195,135.489373892464));
#230034=CARTESIAN_POINT('Ctrl Pts',(119.696250068622,6.45868467482089,129.418926352309));
#230035=CARTESIAN_POINT('Ctrl Pts',(119.417802444809,2.32547174398699,124.621625219699));
#230036=CARTESIAN_POINT('Ctrl Pts',(119.139354820996,-3.94473611396066,
125.505955874312));
#230037=CARTESIAN_POINT('Ctrl Pts',(118.860907197183,-6.58992419425096,
131.259261646514));
#230038=CARTESIAN_POINT('Ctrl Pts',(118.58245957337,-3.17929387571916,136.594535596262));
#230039=CARTESIAN_POINT('Ctrl Pts',(118.304011949557,3.15295219745811,136.608921606362));
#230040=CARTESIAN_POINT('Ctrl Pts',(118.025564325744,6.58778923144938,131.289199636326));
#230041=CARTESIAN_POINT('Ctrl Pts',(117.747116701932,3.96876979313418,125.523934293753));
#230042=CARTESIAN_POINT('Ctrl Pts',(117.468669078118,-2.29735519988813,
124.611122779595));
#230043=CARTESIAN_POINT('Ctrl Pts',(117.190221454306,-6.45232299625411,
129.389594282045));
#230044=CARTESIAN_POINT('Ctrl Pts',(116.911773830493,-4.67792117256487,
135.468166931659));
#230045=CARTESIAN_POINT('Ctrl Pts',(116.63332620668,1.39526167955762,137.260929418227));
#230046=CARTESIAN_POINT('Ctrl Pts',(116.354878582867,6.18626721048894,133.120420597908));
#230047=CARTESIAN_POINT('Ctrl Pts',(116.076430959054,5.29239539093549,126.851565801475));
#230048=CARTESIAN_POINT('Ctrl Pts',(115.797983335241,-0.464929244999223,
124.215136336267));
#230049=CARTESIAN_POINT('Ctrl Pts',(115.519535711428,-5.79500661783607,
127.633882084071));
#230050=CARTESIAN_POINT('Ctrl Pts',(115.241088087616,-5.79975601069334,
133.96614271767));
#230051=CARTESIAN_POINT('Ctrl Pts',(114.962640463802,-0.474812963556037,
137.392880062915));
#230052=CARTESIAN_POINT('Ctrl Pts',(114.68419283999,5.28646000118636,134.765089904953));
#230053=CARTESIAN_POINT('Ctrl Pts',(114.405745216177,6.18973448276714,128.497583024264));
#230054=CARTESIAN_POINT('Ctrl Pts',(114.127297592364,1.40494536002493,124.349892059469));
#230055=CARTESIAN_POINT('Ctrl Pts',(113.848849968551,-4.67091991318358,
126.133542381245));
#230056=CARTESIAN_POINT('Ctrl Pts',(113.570402344738,-6.45443797329988,
132.209446480045));
#230057=CARTESIAN_POINT('Ctrl Pts',(113.291954720925,-2.30664285277824,
136.994145313484));
#230058=CARTESIAN_POINT('Ctrl Pts',(113.013507097112,3.96084436367879,136.09073439917));
#230059=CARTESIAN_POINT('Ctrl Pts',(112.735059473299,6.58850910791926,130.329404233275));
#230060=CARTESIAN_POINT('Ctrl Pts',(112.456611849487,3.16165584854565,125.004535781636));
#230061=CARTESIAN_POINT('Ctrl Pts',(112.178164225674,-3.1706046801665,125.00942301702));
#230062=CARTESIAN_POINT('Ctrl Pts',(111.899716601861,-6.58923440045535,
130.339574808866));
#230063=CARTESIAN_POINT('Ctrl Pts',(111.621268978048,-3.9526796087217,136.096842052857));
#230064=CARTESIAN_POINT('Ctrl Pts',(111.342821354235,2.31619464429322,136.990577409908));
#230065=CARTESIAN_POINT('Ctrl Pts',(111.064373730422,6.45659917160154,132.199481748287));
#230066=CARTESIAN_POINT('Ctrl Pts',(110.785926106609,4.66370448261314,126.12633792299));
#230067=CARTESIAN_POINT('Ctrl Pts',(110.507478482796,-1.41490679126679,
124.352068419894));
#230068=CARTESIAN_POINT('Ctrl Pts',(110.229030858983,-6.19328784601188,
128.50714023446));
#230069=CARTESIAN_POINT('Ctrl Pts',(109.950583235171,-5.28033992920373,
134.773245355646));
#230070=CARTESIAN_POINT('Ctrl Pts',(109.672135611358,0.484982423596243,
137.392139293334));
#230071=CARTESIAN_POINT('Ctrl Pts',(109.393687987545,5.80462962181993,133.957186458871));
#230072=CARTESIAN_POINT('Ctrl Pts',(109.115240363732,5.79010576951274,127.624940700352));
#230073=CARTESIAN_POINT('Ctrl Pts',(108.836792739919,0.454757577415474,
124.214426522456));
#230074=CARTESIAN_POINT('Ctrl Pts',(108.558345116106,-5.29849061218381,
126.859739841786));
#230075=CARTESIAN_POINT('Ctrl Pts',(108.279897492293,-6.18268477484283,
133.12996694862));
#230076=CARTESIAN_POINT('Ctrl Pts',(108.00144986848,-1.38529367036394,137.2630754494));
#230077=CARTESIAN_POINT('Ctrl Pts',(107.723002244667,4.68511464182123,135.460940545486));
#230078=CARTESIAN_POINT('Ctrl Pts',(107.444554620855,6.45013147874722,129.379636174388));
#230079=CARTESIAN_POINT('Ctrl Pts',(107.166106997042,2.28779259314522,124.607583964913));
#230080=CARTESIAN_POINT('Ctrl Pts',(106.887659373229,-3.97691592067581,
125.530066769856));
#230081=CARTESIAN_POINT('Ctrl Pts',(106.609211749416,-6.58703298653922,
131.299367957265));
#230082=CARTESIAN_POINT('Ctrl Pts',(106.330764125603,-3.14398853222427,
136.613781581943));
#230083=CARTESIAN_POINT('Ctrl Pts',(106.05231650179,3.18822779082625,136.589621146351));
#230084=CARTESIAN_POINT('Ctrl Pts',(105.773868877977,6.59061852769399,131.249088910493));
#230085=CARTESIAN_POINT('Ctrl Pts',(105.495421254164,3.93655280722527,125.49987309962));
#230086=CARTESIAN_POINT('Ctrl Pts',(105.216973630351,-2.33501263178752,
124.625222179118));
#230087=CARTESIAN_POINT('Ctrl Pts',(104.938526006539,-6.46081553389627,
129.428897615854));
#230088=CARTESIAN_POINT('Ctrl Pts',(104.660078382726,-4.64944458874018,
135.49655635606));
#230089=CARTESIAN_POINT('Ctrl Pts',(104.381630758913,1.43453879547275,137.252316439095));
#230090=CARTESIAN_POINT('Ctrl Pts',(104.1031831351,6.20025110776228,133.082720122298));
#230091=CARTESIAN_POINT('Ctrl Pts',(103.824735511287,5.26823555112421,126.819422724701));
#230092=CARTESIAN_POINT('Ctrl Pts',(103.546287887474,-0.505031109382345,
124.218088575609));
#230093=CARTESIAN_POINT('Ctrl Pts',(103.267840263661,-5.81419885250792,
127.669216675797));
#230094=CARTESIAN_POINT('Ctrl Pts',(102.989392639848,-5.78040188958328,
134.001388898174));
#230095=CARTESIAN_POINT('Ctrl Pts',(102.710945016035,-0.434697978462825,
137.395648314187));
#230096=CARTESIAN_POINT('Ctrl Pts',(102.432497392222,5.31047213868803,134.732836339309));
#230097=CARTESIAN_POINT('Ctrl Pts',(102.15404976841,6.17557779137139,128.459947092858));
#230098=CARTESIAN_POINT('Ctrl Pts',(101.875602144597,1.3656291475316,124.341459344644));
#230099=CARTESIAN_POINT('Ctrl Pts',(101.597154520784,-4.69926596819684,
126.162062135967));
#230100=CARTESIAN_POINT('Ctrl Pts',(101.318706896971,-6.44576523105769,
132.248710442988));
#230101=CARTESIAN_POINT('Ctrl Pts',(101.040259273158,-2.26892113971413,
137.008071820859));
#230102=CARTESIAN_POINT('Ctrl Pts',(100.761811649345,3.99295063606701,136.066525671043));
#230103=CARTESIAN_POINT('Ctrl Pts',(100.483364025532,6.58549584378548,130.289306908136));
#230104=CARTESIAN_POINT('Ctrl Pts',(100.204916401719,3.12629209042249,124.985397342422));
#230105=CARTESIAN_POINT('Ctrl Pts',(99.9264687779064,-3.20582136617937,
125.028830754405));
#230106=CARTESIAN_POINT('Ctrl Pts',(99.6480211540935,-6.5919416003429,130.379693960313));
#230107=CARTESIAN_POINT('Ctrl Pts',(99.3695735302808,-3.92038953804142,
136.120805078117));
#230108=CARTESIAN_POINT('Ctrl Pts',(99.0911259064677,2.35380898804382,136.976363459425));
#230109=CARTESIAN_POINT('Ctrl Pts',(98.812678282655,6.46497204407849,132.160152748165));
#230110=CARTESIAN_POINT('Ctrl Pts',(98.5342306588419,4.63514162304771,126.098035303012));
#230111=CARTESIAN_POINT('Ctrl Pts',(98.2557830350292,-1.45415751030726,
124.36080090516));
#230112=CARTESIAN_POINT('Ctrl Pts',(97.9773354112161,-6.20715693123341,
128.544883097616));
#230113=CARTESIAN_POINT('Ctrl Pts',(97.6988877874034,-5.25608236883021,
134.805314749293));
#230114=CARTESIAN_POINT('Ctrl Pts',(97.4204401635904,0.525075116629235,
137.389065011387));
#230115=CARTESIAN_POINT('Ctrl Pts',(97.1419925397775,5.82371422125203,133.921793616252));
#230116=CARTESIAN_POINT('Ctrl Pts',(96.8635449159648,5.77064446080036,127.589753590393));
#230117=CARTESIAN_POINT('Ctrl Pts',(96.5850972921516,0.414634352527504,
124.211780380221));
#230118=CARTESIAN_POINT('Ctrl Pts',(96.306649668339,-5.32240446970382,126.89206634272));
#230119=CARTESIAN_POINT('Ctrl Pts',(96.0282020445258,-6.16841359819089,
133.1675596176));
#230120=CARTESIAN_POINT('Ctrl Pts',(95.7497544207132,-1.34595197369742,
137.271388460138));
#230121=CARTESIAN_POINT('Ctrl Pts',(95.4713067969001,4.7133737612145,135.432334647225));
#230122=CARTESIAN_POINT('Ctrl Pts',(95.1928591730874,6.44133927067958,129.340398790155));
#230123=CARTESIAN_POINT('Ctrl Pts',(94.9144115492744,2.25002866730758,124.593772333964));
#230124=CARTESIAN_POINT('Ctrl Pts',(94.6359639254615,-4.008948361309,125.554373106298));
#230125=CARTESIAN_POINT('Ctrl Pts',(94.3575163016487,-6.58389769389783,
131.339455925338));
#230126=CARTESIAN_POINT('Ctrl Pts',(94.0790686778357,-3.10856668707799,
136.632812297395));
#230127=CARTESIAN_POINT('Ctrl Pts',(93.8006210540229,3.22338524324122,136.570106311383));
#230128=CARTESIAN_POINT('Ctrl Pts',(93.52217343021,6.59320360614536,131.208961705089));
#230129=CARTESIAN_POINT('Ctrl Pts',(93.2437258063971,3.90418995090443,125.476008465224));
#230130=CARTESIAN_POINT('Ctrl Pts',(92.9652781825842,-2.37258353893516,
124.639550548886));
#230131=CARTESIAN_POINT('Ctrl Pts',(92.6868305587713,-6.46906866364288,
129.468251917951));
#230132=CARTESIAN_POINT('Ctrl Pts',(92.4083829349583,-4.62079571803641,
135.524771909422));
#230133=CARTESIAN_POINT('Ctrl Pts',(92.1299353111456,1.47376275402524,137.24346452859));
#230134=CARTESIAN_POINT('Ctrl Pts',(91.8514876873325,6.21400525245068,133.04493522124));
#230135=CARTESIAN_POINT('Ctrl Pts',(91.5730400635199,5.24388049490719,126.787427311268));
#230136=CARTESIAN_POINT('Ctrl Pts',(91.2945924397067,-0.545114259651984,
124.221284871682));
#230137=CARTESIAN_POINT('Ctrl Pts',(91.016144815894,-5.83317563990314,127.704667441434));
#230138=CARTESIAN_POINT('Ctrl Pts',(90.7376971920811,-5.76083357355547,
134.036516611621));
#230139=CARTESIAN_POINT('Ctrl Pts',(90.4592495682681,-0.394566885476172,
137.398172322869));
#230140=CARTESIAN_POINT('Ctrl Pts',(90.1808019444553,5.33428749469169,134.700437202553));
#230141=CARTESIAN_POINT('Ctrl Pts',(89.9023543206424,6.16119226166949,128.422398034556));
#230142=CARTESIAN_POINT('Ctrl Pts',(89.6239066968295,1.32626233114802,124.333266115003));
#230143=CARTESIAN_POINT('Ctrl Pts',(89.3454590730166,-4.72743789018152,
126.190753912764));
#230144=CARTESIAN_POINT('Ctrl Pts',(89.0670114492037,-6.43685363861442,
132.28792088502));
#230145=CARTESIAN_POINT('Ctrl Pts',(88.7885638253908,-2.23111535094281,
137.021768447433));
#230146=CARTESIAN_POINT('Ctrl Pts',(88.5101162015778,4.02490894820102,136.042121951457));
#230147=CARTESIAN_POINT('Ctrl Pts',(88.2316685777651,6.58223855168135,130.2492286685));
#230148=CARTESIAN_POINT('Ctrl Pts',(87.9532209539521,3.09081248639635,124.966474527032));
#230149=CARTESIAN_POINT('Ctrl Pts',(87.6747733301392,-3.2409192593025,125.048452506173));
#230150=CARTESIAN_POINT('Ctrl Pts',(87.3963257063264,-6.59440453341028,
130.41982884794));
#230151=CARTESIAN_POINT('Ctrl Pts',(87.1178780825135,-3.88795419588509,
136.144571100572));
#230152=CARTESIAN_POINT('Ctrl Pts',(86.8394304587006,2.39133611053674,136.961920803106));
#230153=CARTESIAN_POINT('Ctrl Pts',(86.5609828348878,6.47310535463887,132.120773508667));
#230154=CARTESIAN_POINT('Ctrl Pts',(86.2825352110747,4.60640700660486,126.06990707765));
#230155=CARTESIAN_POINT('Ctrl Pts',(86.004087587262,-1.49335434500641,124.369772158902));
#230156=CARTESIAN_POINT('Ctrl Pts',(85.725639963449,-6.22079600797217,128.582709686544));
#230157=CARTESIAN_POINT('Ctrl Pts',(85.4471923396362,-5.23163004239161,
134.837235886113));
#230158=CARTESIAN_POINT('Ctrl Pts',(85.1687447158232,0.565148352810691,
137.385746730796));
#230159=CARTESIAN_POINT('Ctrl Pts',(84.8902970920103,5.842583020812,133.886285256006));
#230160=CARTESIAN_POINT('Ctrl Pts',(84.6118494681974,5.75096931873532,127.554685598878));
#230161=CARTESIAN_POINT('Ctrl Pts',(84.3334018443846,0.374495763211118,
124.209378528473));
#230162=CARTESIAN_POINT('Ctrl Pts',(84.0549542205716,-5.34612110356891,
126.924537815158));
#230163=CARTESIAN_POINT('Ctrl Pts',(83.7765065967588,-6.15391384870464,
133.205064717373));
#230164=CARTESIAN_POINT('Ctrl Pts',(83.498058972946,-1.30656040228555,137.279461832782));
#230165=CARTESIAN_POINT('Ctrl Pts',(83.2196113491328,4.74145822480973,135.403557257686));
#230166=CARTESIAN_POINT('Ctrl Pts',(82.9411637253203,6.43230837641647,129.301215653567));
#230167=CARTESIAN_POINT('Ctrl Pts',(82.6627161015071,2.21218136583022,124.580190838648));
#230168=CARTESIAN_POINT('Ctrl Pts',(82.3842684776944,-4.04083224888638,
125.578873982957));
#230169=CARTESIAN_POINT('Ctrl Pts',(82.1058208538814,-6.58051843250612,
131.379524065257));
#230170=CARTESIAN_POINT('Ctrl Pts',(81.8273732300686,-3.07302965285007,
136.651627037425));
#230171=CARTESIAN_POINT('Ctrl Pts',(81.5489256062556,3.25842325193051,136.550377824588));
#230172=CARTESIAN_POINT('Ctrl Pts',(81.270477982443,6.59554437101248,131.168819507043));
#230173=CARTESIAN_POINT('Ctrl Pts',(80.9920303586297,3.87168242338918,125.452341274876));
#230174=CARTESIAN_POINT('Ctrl Pts',(80.713582734817,-2.41006652912724,124.654107357959));
#230175=CARTESIAN_POINT('Ctrl Pts',(80.435135111004,-6.47708207967116,129.507655730047));
#230176=CARTESIAN_POINT('Ctrl Pts',(80.1566874871913,-4.59197562204804,
135.552812546207));
#230177=CARTESIAN_POINT('Ctrl Pts',(79.8782398633782,1.51293210175691,137.234374014721));
#230178=CARTESIAN_POINT('Ctrl Pts',(79.5997922395654,6.22752913488936,133.007067294864));
#230179=CARTESIAN_POINT('Ctrl Pts',(79.3213446157525,5.2193311247699,126.755580746775));
#230180=CARTESIAN_POINT('Ctrl Pts',(79.0428969919396,-0.585177210512381,
124.224725106049));
#230181=CARTESIAN_POINT('Ctrl Pts',(78.7644493681267,-5.85193627682986,
127.740233067343));
#230182=CARTESIAN_POINT('Ctrl Pts',(78.4860017443139,-5.74105178772106,
134.071524556339));
#230183=CARTESIAN_POINT('Ctrl Pts',(78.2075541205009,-0.354421171668466,
137.400451995434));
#230184=CARTESIAN_POINT('Ctrl Pts',(77.9291064966881,5.35790518671055,134.667893695246));
#230185=CARTESIAN_POINT('Ctrl Pts',(77.6506588728751,6.14657842672258,128.384937240753));
#230186=CARTESIAN_POINT('Ctrl Pts',(77.3722112490624,1.28684636962602,124.325312674148));
#230187=CARTESIAN_POINT('Ctrl Pts',(77.0937636252493,-4.75543463521666,
126.219616648455));
#230188=CARTESIAN_POINT('Ctrl Pts',(76.8153160014366,-6.42770352619243,
132.327076353179));
#230189=CARTESIAN_POINT('Ctrl Pts',(76.5368683776235,-2.19322688737167,
137.035234685673));
#230190=CARTESIAN_POINT('Ctrl Pts',(76.2584207538107,4.05671811585379,136.017524144697));
#230191=CARTESIAN_POINT('Ctrl Pts',(75.9799731299978,6.57873735230709,130.209170999483));
#230192=CARTESIAN_POINT('Ctrl Pts',(75.7015255061849,3.05521835117689,124.947768036657));
#230193=CARTESIAN_POINT('Ctrl Pts',(75.423077882372,-3.27589705897064,125.068287545233));
#230194=CARTESIAN_POINT('Ctrl Pts',(75.1446302585591,-6.5966231083926,130.459977984534));
#230195=CARTESIAN_POINT('Ctrl Pts',(74.8661826347462,-3.85537478415624,
136.168139239563));
#230196=CARTESIAN_POINT('Ctrl Pts',(74.5877350109334,2.42877462119068,136.94724997613));
#230197=CARTESIAN_POINT('Ctrl Pts',(74.3092873871204,6.48099880189986,132.081345489005));
#230198=CARTESIAN_POINT('Ctrl Pts',(74.0308397633076,4.57750169805637,126.041954289206));
#230199=CARTESIAN_POINT('Ctrl Pts',(73.7523921394947,-1.53249584291112,
124.378981848686));
#230200=CARTESIAN_POINT('Ctrl Pts',(73.4739445156818,-6.23420457082727,
128.620618599563));
#230201=CARTESIAN_POINT('Ctrl Pts',(73.1954968918689,-5.20698385597775,
134.869007583256));
#230202=CARTESIAN_POINT('Ctrl Pts',(72.917049268056,0.605200647212208,137.382184574524));
#230203=CARTESIAN_POINT('Ctrl Pts',(72.6386016442432,5.86123532130951,133.850662693911));
#230204=CARTESIAN_POINT('Ctrl Pts',(72.3601540204302,5.73108107238729,127.519738025268));
#230205=CARTESIAN_POINT('Ctrl Pts',(72.0817063966174,0.334343296816498,
124.207221056211));
#230206=CARTESIAN_POINT('Ctrl Pts',(71.8032587728044,-5.36963963495047,
126.957153055855));
#230207=CARTESIAN_POINT('Ctrl Pts',(71.5248111489915,-6.13918606367764,
133.242480858172));
#230208=CARTESIAN_POINT('Ctrl Pts',(71.2463635251787,-1.26712041579749,
137.287295268168));
#230209=CARTESIAN_POINT('Ctrl Pts',(70.9679159013657,4.76936699192676,135.374609443224));
#230210=CARTESIAN_POINT('Ctrl Pts',(70.689468277553,6.423039130601,129.262088216567));
#230211=CARTESIAN_POINT('Ctrl Pts',(70.4110206537399,2.17425209115883,124.566839982233));
#230212=CARTESIAN_POINT('Ctrl Pts',(70.1325730299272,-4.07256640193864,
125.603568491945));
#230213=CARTESIAN_POINT('Ctrl Pts',(69.8541254061142,-6.57689532758393,
131.419570892283));
#230214=CARTESIAN_POINT('Ctrl Pts',(69.5756777823013,-3.03737874637841,
136.670225104848));
#230215=CARTESIAN_POINT('Ctrl Pts',(69.2972301584884,3.2933405185478,136.530436417012));
#230216=CARTESIAN_POINT('Ctrl Pts',(69.0187825346755,6.5976407355574,131.128663803839));
#230217=CARTESIAN_POINT('Ctrl Pts',(68.7403349108627,3.83903142925813,125.428872405572));
#230218=CARTESIAN_POINT('Ctrl Pts',(68.4618872870498,-2.44746021341752,
124.668892066929));
#230219=CARTESIAN_POINT('Ctrl Pts',(68.1834396632368,-6.48485548504104,
129.547107592018));
#230220=CARTESIAN_POINT('Ctrl Pts',(67.904992039424,-4.56298536871445,135.580677227361));
#230221=CARTESIAN_POINT('Ctrl Pts',(67.6265444156111,1.55204538723279,137.225045234339));
#230222=CARTESIAN_POINT('Ctrl Pts',(67.3480967917982,6.2408222539455,132.969117746385));
#230223=CARTESIAN_POINT('Ctrl Pts',(67.0696491679854,5.19458835039884,126.723884211309));
#230224=CARTESIAN_POINT('Ctrl Pts',(66.7912015441724,-0.625218477415679,
124.228409151229));
#230225=CARTESIAN_POINT('Ctrl Pts',(66.5127539203596,-5.87048006810572,
127.775912235624));
#230226=CARTESIAN_POINT('Ctrl Pts',(66.2343062965465,-5.72105726510147,
134.106411435094));
#230227=CARTESIAN_POINT('Ctrl Pts',(65.9558586727338,-0.314262324654327,
137.402487247406));
#230228=CARTESIAN_POINT('Ctrl Pts',(65.6774110489208,5.3813243395822,134.6352070233));
#230229=CARTESIAN_POINT('Ctrl Pts',(65.398963425108,6.13173682805169,128.347566099575));
#230230=CARTESIAN_POINT('Ctrl Pts',(65.120515801295,1.24738272353907,124.317599316798));
#230231=CARTESIAN_POINT('Ctrl Pts',(64.8420681774823,-4.78325516587229,
126.248649273519));
#230232=CARTESIAN_POINT('Ctrl Pts',(64.5636205536692,-6.41831523285262,
132.366175396547));
#230233=CARTESIAN_POINT('Ctrl Pts',(64.2851729298565,-2.15525715297185,
137.048470036584));
#230234=CARTESIAN_POINT('Ctrl Pts',(64.0067253060435,4.08837696032456,135.992733162246));
#230235=CARTESIAN_POINT('Ctrl Pts',(63.7282776822307,6.57499237540094,130.169135385437));
#230236=CARTESIAN_POINT('Ctrl Pts',(63.4498300584178,3.01951100371835,124.929278564476));
#230237=CARTESIAN_POINT('Ctrl Pts',(63.1713824346048,-3.31075346906837,
125.088335136589));
#230238=CARTESIAN_POINT('Ctrl Pts',(62.892934810792,-6.59859724307971,130.500139882352));
#230239=CARTESIAN_POINT('Ctrl Pts',(62.614487186979,-3.82265251009718,136.191508621766));
#230240=CARTESIAN_POINT('Ctrl Pts',(62.3360395631662,2.46612313270748,136.932351522132));
#230241=CARTESIAN_POINT('Ctrl Pts',(62.0575919393533,6.48865209336687,132.041870150199));
#230242=CARTESIAN_POINT('Ctrl Pts',(61.7791443155403,4.5484267684992,126.014177973478));
#230243=CARTESIAN_POINT('Ctrl Pts',(61.5006966917276,-1.57158055361859,
124.388429633243));
#230244=CARTESIAN_POINT('Ctrl Pts',(61.2222490679146,-6.24738212293903,
128.658608431946));
#230245=CARTESIAN_POINT('Ctrl Pts',(60.9438014441017,-5.18214472286266,
134.900628663412));
#230246=CARTESIAN_POINT('Ctrl Pts',(60.6653538202889,0.645230515680748,
137.378378674564));
#230247=CARTESIAN_POINT('Ctrl Pts',(60.3869061964759,5.87967043157647,133.814927249971));
#230248=CARTESIAN_POINT('Ctrl Pts',(60.108458572663,5.71098045872276,127.484912164554));
#230249=CARTESIAN_POINT('Ctrl Pts',(59.8300109488502,0.294178441208572,
124.205308043382));
#230250=CARTESIAN_POINT('Ctrl Pts',(59.5515633250373,-5.39295919236059,
126.989910856244));
#230251=CARTESIAN_POINT('Ctrl Pts',(59.2731157012244,-6.12423078885343,
133.27980665353));
#230252=CARTESIAN_POINT('Ctrl Pts',(58.9946680774115,-1.2276334756968,137.294888476026));
#230253=CARTESIAN_POINT('Ctrl Pts',(58.7162204535986,4.79709902839574,135.345492276511));
#230254=CARTESIAN_POINT('Ctrl Pts',(58.4377728297857,6.41353187670863,129.223017929039));
#230255=CARTESIAN_POINT('Ctrl Pts',(58.1593252059728,2.13624224877676,124.553720259438));
#230256=CARTESIAN_POINT('Ctrl Pts',(57.8808775821599,-4.10414964454526,
125.628455718198));
#230257=CARTESIAN_POINT('Ctrl Pts',(57.602429958347,-6.57302851338661,131.459594922466));
#230258=CARTESIAN_POINT('Ctrl Pts',(57.3239823345341,-3.00161528872044,
136.688605810505));
#230259=CARTESIAN_POINT('Ctrl Pts',(57.0455347107212,3.32813574922106,136.510282827592));
#230260=CARTESIAN_POINT('Ctrl Pts',(56.7670870869083,6.59949262209846,131.088496083461));
#230261=CARTESIAN_POINT('Ctrl Pts',(56.4886394630955,3.80623817840574,125.405602726962));
#230262=CARTESIAN_POINT('Ctrl Pts',(56.2101918392826,-2.48476320616966,
124.683904127941));
#230263=CARTESIAN_POINT('Ctrl Pts',(55.9317442154696,-6.49238859170611,
129.586606041964));
#230264=CARTESIAN_POINT('Ctrl Pts',(55.6532965916568,-4.53382603227983,
135.608364920346));
#230265=CARTESIAN_POINT('Ctrl Pts',(55.3748489678439,1.59110116109648,137.215478533129));
#230266=CARTESIAN_POINT('Ctrl Pts',(55.096401344031,6.25388411703813,132.931087982032));
#230267=CARTESIAN_POINT('Ctrl Pts',(54.8179537202181,5.1696530886458,126.692338879397));
#230268=CARTESIAN_POINT('Ctrl Pts',(54.5395060964052,-0.665236576618623,
124.23233687071));
#230269=CARTESIAN_POINT('Ctrl Pts',(54.2610584725923,-5.88880632658389,
127.811703624173));
#230270=CARTESIAN_POINT('Ctrl Pts',(53.9826108487795,-5.70085074660091,
134.141175955143));
#230271=CARTESIAN_POINT('Ctrl Pts',(53.7041632249665,-0.274091832533765,
137.40427800337));
#230272=CARTESIAN_POINT('Ctrl Pts',(53.4257156011537,5.40454408550164,134.602378397932));
#230273=CARTESIAN_POINT('Ctrl Pts',(53.1472679773408,6.11666801561766,128.310285995821));
#230274=CARTESIAN_POINT('Ctrl Pts',(52.8688203535278,1.20787285522606,124.310126328773));
#230275=CARTESIAN_POINT('Ctrl Pts',(52.590372729715,-4.81089845124901,126.277850712144));
#230276=CARTESIAN_POINT('Ctrl Pts',(52.3119251059021,-6.40868910648141,
132.405216566294));
#230277=CARTESIAN_POINT('Ctrl Pts',(52.0334774820892,-2.11720755472543,
137.061474009724));
#230278=CARTESIAN_POINT('Ctrl Pts',(51.7550298582764,4.11988430848393,135.967749922743));
#230279=CARTESIAN_POINT('Ctrl Pts',(51.4765822344634,6.57100375973434,130.129123309894));
#230280=CARTESIAN_POINT('Ctrl Pts',(51.1981346106506,2.98369176716867,124.91100679562));
#230281=CARTESIAN_POINT('Ctrl Pts',(50.9196869868376,-3.34548719797895,
125.108594537373));
#230282=CARTESIAN_POINT('Ctrl Pts',(50.6412393630248,-6.60032686431936,
130.540313053181));
#230283=CARTESIAN_POINT('Ctrl Pts',(50.3627917392119,-3.78978858624336,
136.214678381218));
#230284=CARTESIAN_POINT('Ctrl Pts',(50.0843441153989,2.50338026112505,136.917225993175));
#230285=CARTESIAN_POINT('Ctrl Pts',(49.8058964915862,6.49606494544435,132.002348955022));
#230286=CARTESIAN_POINT('Ctrl Pts',(49.5274488677731,4.51918329531533,125.986579159731));
#230287=CARTESIAN_POINT('Ctrl Pts',(49.2490012439603,-1.6106070288309,124.39811516248));
#230288=CARTESIAN_POINT('Ctrl Pts',(48.9705536201474,-6.26032817600901,
128.696677775965));
#230289=CARTESIAN_POINT('Ctrl Pts',(48.6921059963345,-5.15711356346882,
134.932097954848));
#230290=CARTESIAN_POINT('Ctrl Pts',(48.4136583725217,0.685236474895564,
137.374329171949));
#230291=CARTESIAN_POINT('Ctrl Pts',(48.1352107487087,5.89788766849362,133.779080248378));
#230292=CARTESIAN_POINT('Ctrl Pts',(47.8567631248959,5.69066822257687,127.450209307224));
#230293=CARTESIAN_POINT('Ctrl Pts',(47.578315501083,0.254002684709825,124.203639560873));
#230294=CARTESIAN_POINT('Ctrl Pts',(47.29986787727,-5.41607891168467,127.022810002472));
#230295=CARTESIAN_POINT('Ctrl Pts',(47.0214202534572,-6.10904857840509,
133.317040720324));
#230296=CARTESIAN_POINT('Ctrl Pts',(46.7429726296443,-1.18810104518584,
137.302241174989));
#230297=CARTESIAN_POINT('Ctrl Pts',(46.4645250058313,4.82465330659632,135.316206836494));
#230298=CARTESIAN_POINT('Ctrl Pts',(46.1860773820186,6.40378696703385,129.184006238746));
#230299=CARTESIAN_POINT('Ctrl Pts',(45.9076297582056,2.09815324715241,124.54083215642));
#230300=CARTESIAN_POINT('Ctrl Pts',(45.6291821343927,-4.13558080637756,
125.653534739511));
#230301=CARTESIAN_POINT('Ctrl Pts',(45.3507345105798,-6.56891813320061,
131.499594672701));
#230302=CARTESIAN_POINT('Ctrl Pts',(45.072286886767,-2.96574060510383,136.706768473292));
#230303=CARTESIAN_POINT('Ctrl Pts',(44.793839262954,3.36280765460034,136.489917803126));
#230304=CARTESIAN_POINT('Ctrl Pts',(44.5153916391412,6.60109996201359,131.048317834339));
#230305=CARTESIAN_POINT('Ctrl Pts',(44.2369440153282,3.77330388599763,125.38253310131));
#230306=CARTESIAN_POINT('Ctrl Pts',(43.9584963915154,-2.52197412510756,
124.699142984721));
#230307=CARTESIAN_POINT('Ctrl Pts',(43.6800487677024,-6.49968112052436,
129.626149616253));
#230308=CARTESIAN_POINT('Ctrl Pts',(43.4016011438896,-4.50449869325427,
135.635874599185));
#230309=CARTESIAN_POINT('Ctrl Pts',(43.1231535200766,1.6300979761215,137.205674265588));
#230310=CARTESIAN_POINT('Ctrl Pts',(42.8447058962639,6.26671424015497,132.892979411015));
#230311=CARTESIAN_POINT('Ctrl Pts',(42.5662582724509,5.14452626349642,126.660945919963));
#230312=CARTESIAN_POINT('Ctrl Pts',(42.287810648638,-0.705230025235587,
124.236508118946));
#230313=CARTESIAN_POINT('Ctrl Pts',(42.0093630248251,-5.90691437317801,
127.847605906729));
#230314=CARTESIAN_POINT('Ctrl Pts',(41.7309154010123,-5.68043298097947,
134.175816828272));
#230315=CARTESIAN_POINT('Ctrl Pts',(41.4524677771993,-0.233911183839542,
137.405824196969));
#230316=CARTESIAN_POINT('Ctrl Pts',(41.1740201533865,5.42756356405245,134.569409035618));
#230317=CARTESIAN_POINT('Ctrl Pts',(40.8955725295735,6.10137254780096,128.273098310918));
#230318=CARTESIAN_POINT('Ctrl Pts',(40.6171249057607,1.1683182287399,124.302893986988));
#230319=CARTESIAN_POINT('Ctrl Pts',(40.3386772819477,-4.83836346701448,
126.307219882257));
#230320=CARTESIAN_POINT('Ctrl Pts',(40.060229658135,-6.39882550377857,132.444198415735));
#230321=CARTESIAN_POINT('Ctrl Pts',(39.781782034322,-2.07907950257448,137.074246123225));
#230322=CARTESIAN_POINT('Ctrl Pts',(39.5033344105091,4.15123899281517,135.94257535195));
#230323=CARTESIAN_POINT('Ctrl Pts',(39.2248867866962,6.56677165310695,130.089136255519));
#230324=CARTESIAN_POINT('Ctrl Pts',(38.9464391628834,2.94776196882331,124.892953407157));
#230325=CARTESIAN_POINT('Ctrl Pts',(38.6679915390704,-3.38009695863112,
125.129064996863));
#230326=CARTESIAN_POINT('Ctrl Pts',(38.3895439152575,-6.6018119080198,130.58049600839));
#230327=CARTESIAN_POINT('Ctrl Pts',(38.1110962914447,-3.75678423037978,
136.237647659355));
#230328=CARTESIAN_POINT('Ctrl Pts',(37.8326486676317,2.54054462586645,136.901873949744));
#230329=CARTESIAN_POINT('Ctrl Pts',(37.5542010438189,6.50323708344635,131.962783367948));
#230330=CARTESIAN_POINT('Ctrl Pts',(37.275753420006,4.48977236213255,125.959158870647));
#230331=CARTESIAN_POINT('Ctrl Pts',(36.9973057961931,-1.64957382240749,
124.4080380775));
#230332=CARTESIAN_POINT('Ctrl Pts',(36.7188581723802,-6.27304225031618,
128.734825220947));
#230333=CARTESIAN_POINT('Ctrl Pts',(36.4404105485673,-5.13189130533538,
134.96341429146));
#230334=CARTESIAN_POINT('Ctrl Pts',(36.1619629247544,0.725217042420823,
137.370036216732));
#230335=CARTESIAN_POINT('Ctrl Pts',(35.8835153009416,5.91588635701427,133.743123017455));
#230336=CARTESIAN_POINT('Ctrl Pts',(35.6050676771286,5.67014511662727,127.415630739204));
#230337=CARTESIAN_POINT('Ctrl Pts',(35.3266200533158,0.213817516048174,
124.202215670509));
#230338=CARTESIAN_POINT('Ctrl Pts',(35.0481724295028,-5.43899793621292,
127.055849275448));
#230339=CARTESIAN_POINT('Ctrl Pts',(34.76972480569,-6.09363999491508,133.354181678833));
#230340=CARTESIAN_POINT('Ctrl Pts',(34.4912771818771,-1.14852458915375,
137.309353092597));
#230341=CARTESIAN_POINT('Ctrl Pts',(34.2128295580642,4.85202880549439,135.286754208357));
#230342=CARTESIAN_POINT('Ctrl Pts',(33.9343819342512,6.393804762678,129.145054591279));
#230343=CARTESIAN_POINT('Ctrl Pts',(33.6559343104384,2.05998649768791,124.528176150753));
#230344=CARTESIAN_POINT('Ctrl Pts',(33.3774866866255,-4.16685872274224,
125.678804626571));
#230345=CARTESIAN_POINT('Ctrl Pts',(33.0990390628127,-6.56456433933747,
131.539568660782));
#230346=CARTESIAN_POINT('Ctrl Pts',(32.8205914389997,-2.92975602487846,
136.724712420187));
#230347=CARTESIAN_POINT('Ctrl Pts',(32.5421438151868,3.39735494990529,136.469342098247));
#230348=CARTESIAN_POINT('Ctrl Pts',(32.263696191374,6.60246269574222,131.008130545292));
#230349=CARTESIAN_POINT('Ctrl Pts',(31.985248567561,3.74022977242616,125.359664383471));
#230350=CARTESIAN_POINT('Ctrl Pts',(31.7068009437482,-2.55909159136699,
124.714608072585));
#230351=CARTESIAN_POINT('Ctrl Pts',(31.4283533199352,-6.50673280126843,
129.665736849585));
#230352=CARTESIAN_POINT('Ctrl Pts',(31.1499056961224,-4.47500443837311,
135.663205244496));
#230353=CARTESIAN_POINT('Ctrl Pts',(30.8714580723094,1.66903438726656,137.195632795014));
#230354=CARTESIAN_POINT('Ctrl Pts',(30.5930104484966,6.27931214787105,132.854793445461));
#230355=CARTESIAN_POINT('Ctrl Pts',(30.3145628246837,5.11920880603445,126.629706496284));
#230356=CARTESIAN_POINT('Ctrl Pts',(30.0361152008708,-0.745197341294603,
124.240922741373));
#230357=CARTESIAN_POINT('Ctrl Pts',(29.7576675770579,-5.9248035368878,127.883617752917));
#230358=CARTESIAN_POINT('Ctrl Pts',(29.4792199532451,-5.65980472482494,
134.210332770852));
#230359=CARTESIAN_POINT('Ctrl Pts',(29.2007723294321,-0.193721867480399,
137.407125770907));
#230360=CARTESIAN_POINT('Ctrl Pts',(28.9223247056193,5.45038192223944,134.536300158051));
#230361=CARTESIAN_POINT('Ctrl Pts',(28.6438770818064,6.08585099138068,128.236004422871));
#230362=CARTESIAN_POINT('Ctrl Pts',(28.3654294579935,1.12872030979243,124.29590255944));
#230363=CARTESIAN_POINT('Ctrl Pts',(28.0869818341806,-4.86564919544231,
126.336755695574));
#230364=CARTESIAN_POINT('Ctrl Pts',(27.8085342103677,-6.38872479024353,
132.483119500384));
#230365=CARTESIAN_POINT('Ctrl Pts',(27.5300865865548,-2.04087440936798,
137.086785903815));
#230366=CARTESIAN_POINT('Ctrl Pts',(27.2516389627419,4.18243985145892,135.91721038272));
#230367=CARTESIAN_POINT('Ctrl Pts',(26.973191338929,6.56229621234102,130.049175704046));
#230368=CARTESIAN_POINT('Ctrl Pts',(26.6947437151162,2.91172294007416,124.875119068062));
#230369=CARTESIAN_POINT('Ctrl Pts',(26.4162960913032,-3.41458146854746,
125.149745756519));
#230370=CARTESIAN_POINT('Ctrl Pts',(26.1378484674903,-6.60305231915217,
130.620687258984));
#230371=CARTESIAN_POINT('Ctrl Pts',(25.8594008436774,-3.72364066549499,
136.260415605043));
#230372=CARTESIAN_POINT('Ctrl Pts',(25.5809532198646,2.57761484979243,136.886295960714));
#230373=CARTESIAN_POINT('Ctrl Pts',(25.3025055960517,6.51016824160669,131.92317485509));
#230374=CARTESIAN_POINT('Ctrl Pts',(25.0240579722387,4.46019505878377,125.931918122295));
#230375=CARTESIAN_POINT('Ctrl Pts',(24.7456103484259,-1.68847949041943,
124.418198010604));
#230376=CARTESIAN_POINT('Ctrl Pts',(24.467162724613,-6.28552387473587,128.773049353324));
#230377=CARTESIAN_POINT('Ctrl Pts',(24.1887151008001,-5.10647888308236,
134.994576512808));
#230378=CARTESIAN_POINT('Ctrl Pts',(23.9102674769872,0.765170736761864,
137.365499967992));
#230379=CARTESIAN_POINT('Ctrl Pts',(23.6318198531744,5.93366583019039,133.707056889611));
#230380=CARTESIAN_POINT('Ctrl Pts',(23.3533722293614,5.64941190136517,127.381177741815));
#230381=CARTESIAN_POINT('Ctrl Pts',(23.0749246055485,0.173624424299845,
124.201036425055));
#230382=CARTESIAN_POINT('Ctrl Pts',(22.7964769817356,-5.46171541667246,
127.08902745089));
#230383=CARTESIAN_POINT('Ctrl Pts',(22.5180293579228,-6.07800560935413,
133.391228152785));
#230384=CARTESIAN_POINT('Ctrl Pts',(22.2395817341099,-1.10890557412062,
137.316223965318));
#230385=CARTESIAN_POINT('Ctrl Pts',(21.9611341102969,4.87922451068073,135.257135483476));
#230386=CARTESIAN_POINT('Ctrl Pts',(21.6826864864842,6.38358563353538,129.106164430008));
#230387=CARTESIAN_POINT('Ctrl Pts',(21.4042388626712,2.02174341466617,124.515752711409));
#230388=CARTESIAN_POINT('Ctrl Pts',(21.1257912388583,-4.19798223462457,
125.704264442993));
#230389=CARTESIAN_POINT('Ctrl Pts',(20.8473436150454,-6.55996729312864,
131.579515405459));
#230390=CARTESIAN_POINT('Ctrl Pts',(20.5688959912325,-2.89366288146616,
136.742436986267));
#230391=CARTESIAN_POINT('Ctrl Pts',(20.2904483674196,3.43177635497322,136.448556475397));
#230392=CARTESIAN_POINT('Ctrl Pts',(20.0120007436067,6.60358077278748,130.967935705476));
#230393=CARTESIAN_POINT('Ctrl Pts',(19.7335531197938,3.70701706326526,125.336997420853));
#230394=CARTESIAN_POINT('Ctrl Pts',(19.455105495981,-2.59611422954622,124.730298818468));
#230395=CARTESIAN_POINT('Ctrl Pts',(19.176657872168,-6.51354337263571,129.705366275038));
#230396=CARTESIAN_POINT('Ctrl Pts',(18.8982102483552,-4.4453443605568,135.690355843533));
#230397=CARTESIAN_POINT('Ctrl Pts',(18.6197626245423,1.70790895172861,137.1853544935));
#230398=CARTESIAN_POINT('Ctrl Pts',(18.3413150007294,6.29167737336628,132.816531500364));
#230399=CARTESIAN_POINT('Ctrl Pts',(18.0628673769165,5.09370165440758,126.598621765949));
#230400=CARTESIAN_POINT('Ctrl Pts',(17.7844197531036,-0.785137043792105,
124.245580574404));
#230401=CARTESIAN_POINT('Ctrl Pts',(17.5059721292907,-5.94247315482366,
127.919737828307));
#230402=CARTESIAN_POINT('Ctrl Pts',(17.2275245054778,-5.63896674252494,
134.244722503881));
#230403=CARTESIAN_POINT('Ctrl Pts',(16.949076881665,-0.15352537268619,137.408182676953));
#230404=CARTESIAN_POINT('Ctrl Pts',(16.6706292578521,5.47299831451989,134.503052992091));
#230405=CARTESIAN_POINT('Ctrl Pts',(16.3921816340391,6.07010392151387,128.199005706208));
#230406=CARTESIAN_POINT('Ctrl Pts',(16.1137340102263,1.08908056569879,124.289152305198));
#230407=CARTESIAN_POINT('Ctrl Pts',(15.8352863864134,-4.89275462544986,
126.366457057635));
#230408=CARTESIAN_POINT('Ctrl Pts',(15.5568387626005,-6.37838734016194,
132.521978378005));
#230409=CARTESIAN_POINT('Ctrl Pts',(15.2783911387876,-2.00259369080969,
137.099092886824));
#230410=CARTESIAN_POINT('Ctrl Pts',(14.9999435149747,4.21348572825588,135.891655954962));
#230411=CARTESIAN_POINT('Ctrl Pts',(14.7214958911618,6.55757760327567,130.009243136227));
#230412=CARTESIAN_POINT('Ctrl Pts',(14.4430482673489,2.87557601636067,124.857504439193));
#230413=CARTESIAN_POINT('Ctrl Pts',(14.164600643536,-3.44893944989177,125.170636050008));
#230414=CARTESIAN_POINT('Ctrl Pts',(13.8861530197231,-6.60404805175259,
130.660885315664));
#230415=CARTESIAN_POINT('Ctrl Pts',(13.6077053959103,-3.69035911973598,
136.282981374608));
#230416=CARTESIAN_POINT('Ctrl Pts',(13.3292577720973,2.61458955925225,136.870492603333));
#230417=CARTESIAN_POINT('Ctrl Pts',(13.0508101482845,6.5168581630887,131.883524884162));
#230418=CARTESIAN_POINT('Ctrl Pts',(12.7723625244716,4.43045248126686,125.904857924092));
#230419=CARTESIAN_POINT('Ctrl Pts',(12.4939149006587,-1.72732259120293,
124.428594585312));
#230420=CARTESIAN_POINT('Ctrl Pts',(12.2154672768458,-6.29777258675688,
128.811348756686));
#230421=CARTESIAN_POINT('Ctrl Pts',(11.9370196530329,-5.08087723837641,
135.025583464166));
#230422=CARTESIAN_POINT('Ctrl Pts',(11.65857202922,0.805096077419857,137.36072059382));
#230423=CARTESIAN_POINT('Ctrl Pts',(11.3801244054071,5.95122542919731,133.670883201288));
#230424=CARTESIAN_POINT('Ctrl Pts',(11.1016767815943,5.62846934506734,127.346851591727));
#230425=CARTESIAN_POINT('Ctrl Pts',(10.8232291577813,0.13342489883439,124.200101868207));
#230426=CARTESIAN_POINT('Ctrl Pts',(10.5447815339684,-5.4842305112587,127.12234329937));
#230427=CARTESIAN_POINT('Ctrl Pts',(10.2663339101556,-6.06214600106014,
133.428178769409));
#230428=CARTESIAN_POINT('Ctrl Pts',(9.98788628634267,-1.06924546818365,
137.322853538546));
#230429=CARTESIAN_POINT('Ctrl Pts',(9.70943866252976,4.90623941440849,135.227351759386));
#230430=CARTESIAN_POINT('Ctrl Pts',(9.43099103871685,6.37312995827954,129.067337196021));
#230431=CARTESIAN_POINT('Ctrl Pts',(9.15254341490403,1.98342541519871,124.503562298745));
#230432=CARTESIAN_POINT('Ctrl Pts',(8.87409579109107,-4.22895018873139,
125.729913245354));
#230433=CARTESIAN_POINT('Ctrl Pts',(8.59564816727821,-6.55512716491932,
131.61943342649));
#230434=CARTESIAN_POINT('Ctrl Pts',(8.31720054346528,-2.85746251231165,
136.759941514744));
#230435=CARTESIAN_POINT('Ctrl Pts',(8.03875291965246,3.46607059430627,136.427561704794));
#230436=CARTESIAN_POINT('Ctrl Pts',(7.76030529583951,6.60445415171875,130.927734804324));
#230437=CARTESIAN_POINT('Ctrl Pts',(7.48185767202662,3.67366698922382,125.314533053388));
#230438=CARTESIAN_POINT('Ctrl Pts',(7.20341004821377,-2.63304066775796,
124.746214640945));
#230439=CARTESIAN_POINT('Ctrl Pts',(6.92496242440086,-6.52011258225796,
129.745036424131));
#230440=CARTESIAN_POINT('Ctrl Pts',(6.64651480058794,-4.41551955887045,
135.71732539022));
#230441=CARTESIAN_POINT('Ctrl Pts',(6.36806717677509,1.74672022899638,137.174839741911));
#230442=CARTESIAN_POINT('Ctrl Pts',(6.08961955296221,6.30380945844269,132.778194993536));
#230443=CARTESIAN_POINT('Ctrl Pts',(5.81117192914928,5.06800575379271,126.567692880813));
#230444=CARTESIAN_POINT('Ctrl Pts',(5.53272430533639,-0.825047652747706,
124.250481445441));
#230445=CARTESIAN_POINT('Ctrl Pts',(5.25427668152353,-5.95992257223146,
127.955964794454));
#230446=CARTESIAN_POINT('Ctrl Pts',(4.97582905771062,-5.61791980623858,
134.278984753035));
#230447=CARTESIAN_POINT('Ctrl Pts',(4.69738143389771,-0.113323188952861,
137.408994875945));
#230448=CARTESIAN_POINT('Ctrl Pts',(4.41893381008486,5.49541190283514,134.469668769726));
#230449=CARTESIAN_POINT('Ctrl Pts',(4.14048618627195,6.05413192171396,128.162103531929));
#230450=CARTESIAN_POINT('Ctrl Pts',(3.86203856245905,1.0494004653243,124.282643474398));
#230451=CARTESIAN_POINT('Ctrl Pts',(3.58359093864613,-4.91967875263547,
126.396322867843));
#230452=CARTESIAN_POINT('Ctrl Pts',(3.30514331483329,-6.36781353659179,
132.560773608667));
#230453=CARTESIAN_POINT('Ctrl Pts',(3.02669569102039,-1.96423876540577,
137.111166616214));
#230454=CARTESIAN_POINT('Ctrl Pts',(2.74824806720748,4.24437547278969,135.865913015604));
#230455=CARTESIAN_POINT('Ctrl Pts',(2.46980044339459,6.55261600076067,129.969340031779));
#230456=CARTESIAN_POINT('Ctrl Pts',(2.19135281958173,2.83932253712042,124.840110173268));
#230457=CARTESIAN_POINT('Ctrl Pts',(1.91290519576881,-3.48316962951642,
125.191735103234));
#230458=CARTESIAN_POINT('Ctrl Pts',(1.6344575719559,-6.60479906892382,130.701088688872));
#230459=CARTESIAN_POINT('Ctrl Pts',(1.35600994814304,-3.65694082636265,
136.305344131865));
#230460=CARTESIAN_POINT('Ctrl Pts',(1.07756232433016,2.65146738413444,136.854464463202));
#230461=CARTESIAN_POINT('Ctrl Pts',(0.799114700517227,6.52330659999492,
131.843834924404));
#230462=CARTESIAN_POINT('Ctrl Pts',(0.520667076704378,4.40054573170394,
125.877979278764));
#230463=CARTESIAN_POINT('Ctrl Pts',(0.242219452891471,-1.76610168541259,
124.439227416375));
#230464=CARTESIAN_POINT('Ctrl Pts',(-0.03622817092143,-6.30978793249869,
128.849722011837));
#230465=CARTESIAN_POINT('Ctrl Pts',(-0.314675794734322,-5.05508731989592,
135.056433996558));
#230466=CARTESIAN_POINT('Ctrl Pts',(-0.593123418547181,0.844991584946641,
137.355698271319));
#230467=CARTESIAN_POINT('Ctrl Pts',(-0.871571042360099,5.96856450335716,
133.634603292916));
#230468=CARTESIAN_POINT('Ctrl Pts',(-1.15001866617301,5.60731822376822,
127.312653560908));
#230469=CARTESIAN_POINT('Ctrl Pts',(-1.42846628998586,0.0932204292604712,
124.199412034595));
#230470=CARTESIAN_POINT('Ctrl Pts',(-1.70691391379876,-5.50654238566651,
127.155795586355));
#230471=CARTESIAN_POINT('Ctrl Pts',(-1.98536153761166,-6.04606175771675,
133.465032159487));
#230472=CARTESIAN_POINT('Ctrl Pts',(-2.26380916142456,-1.02954574096264,
137.329241566624));
#230473=CARTESIAN_POINT('Ctrl Pts',(-2.5422567852374,4.9330725156305,135.197404139731));
#230474=CARTESIAN_POINT('Ctrl Pts',(-2.82070440905033,6.36243812434939,
129.028574328076));
#230475=CARTESIAN_POINT('Ctrl Pts',(-3.09915203286324,1.94503391917308,
124.491605364478));
#230476=CARTESIAN_POINT('Ctrl Pts',(-3.3775996566761,-4.25976143753379,
125.755750083229));
#230477=CARTESIAN_POINT('Ctrl Pts',(-3.65604728048899,-6.55004413406227,
131.659321244699));
#230478=CARTESIAN_POINT('Ctrl Pts',(-3.9344949043019,-2.82115625883292,
136.777225356981));
#230479=CARTESIAN_POINT('Ctrl Pts',(-4.2129425281148,3.50023639711881,136.406358564405));
#230480=CARTESIAN_POINT('Ctrl Pts',(-4.49139015192765,6.60508280017262,
130.887529331496));
#230481=CARTESIAN_POINT('Ctrl Pts',(-4.76983777574057,3.64018078610111,
125.292272113504));
#230482=CARTESIAN_POINT('Ctrl Pts',(-5.04828539955349,-2.66986953767946,
124.762354950249));
#230483=CARTESIAN_POINT('Ctrl Pts',(-5.32673302336633,-6.52644018671072,
129.784745826872));
#230484=CARTESIAN_POINT('Ctrl Pts',(-5.60518064717923,-4.38553113848304,
135.74411288519));
#230485=CARTESIAN_POINT('Ctrl Pts',(-5.88362827099213,1.7854667809037,137.164088929876));
#230486=CARTESIAN_POINT('Ctrl Pts',(-6.16207589480503,6.31570795354138,
132.739785345549));
#230487=CARTESIAN_POINT('Ctrl Pts',(-6.44052351861788,5.04212205636089,
126.536920986959));
#230488=CARTESIAN_POINT('Ctrl Pts',(-6.71897114243081,-0.864927689259141,
124.255625172881));
#230489=CARTESIAN_POINT('Ctrl Pts',(-6.99741876624371,-5.97715114251656,
127.992297308957));
#230490=CARTESIAN_POINT('Ctrl Pts',(-7.27586639005655,-5.59666469586782,
134.313118248714));
#230491=CARTESIAN_POINT('Ctrl Pts',(-7.55431401386947,-0.0731168059870705,
137.409562337785));
#230492=CARTESIAN_POINT('Ctrl Pts',(-7.83276163768236,5.51762185664139,
134.436148728019));
#230493=CARTESIAN_POINT('Ctrl Pts',(-8.11120926149529,6.03793558382929,
128.125299267457));
#230494=CARTESIAN_POINT('Ctrl Pts',(-8.38965688530811,1.00968147902963,
124.276376308223));
#230495=CARTESIAN_POINT('Ctrl Pts',(-8.66810450912106,-4.94642057931569,
126.426352019512));
#230496=CARTESIAN_POINT('Ctrl Pts',(-8.94655213293394,-6.3570037713493,
132.599503754801));
#230497=CARTESIAN_POINT('Ctrl Pts',(-9.22499975674682,-1.92581105441205,
137.123006644589));
#230498=CARTESIAN_POINT('Ctrl Pts',(-9.50344738055969,4.27510794042973,
135.839982518561));
#230499=CARTESIAN_POINT('Ctrl Pts',(-9.78189500437264,6.54741158865002,
129.929467869325));
#230500=CARTESIAN_POINT('Ctrl Pts',(-10.0603426281855,2.80296384573913,
124.822936914835));
#230501=CARTESIAN_POINT('Ctrl Pts',(-10.3387902519984,-3.51727073900952,
125.213042134361));
#230502=CARTESIAN_POINT('Ctrl Pts',(-10.6172378758113,-6.60530534283666,
130.74129588886));
#230503=CARTESIAN_POINT('Ctrl Pts',(-10.8956854996242,-3.62338702370218,
136.327503048155));
#230504=CARTESIAN_POINT('Ctrl Pts',(-11.174133123437,2.68824695791763,136.838212134247));
#230505=CARTESIAN_POINT('Ctrl Pts',(-11.4525807472499,6.52951331337615,
131.804106446543));
#230506=CARTESIAN_POINT('Ctrl Pts',(-11.7310283710628,4.37047591830066,
125.851283182307));
#230507=CARTESIAN_POINT('Ctrl Pts',(-12.0094759948757,-1.80481533607482,
124.450096109789));
#230508=CARTESIAN_POINT('Ctrl Pts',(-12.2879236186886,-6.32156946672825,
128.88816769684));
#230509=CARTESIAN_POINT('Ctrl Pts',(-12.5663712425015,-5.02911008329581,
135.087126966809));
#230510=CARTESIAN_POINT('Ctrl Pts',(-12.8448188663144,0.884855780999501,
137.350433186591));
#230511=CARTESIAN_POINT('Ctrl Pts',(-13.1232664901273,5.98568241016441,
133.598218508862));
#230512=CARTESIAN_POINT('Ctrl Pts',(-13.4017141139402,5.58595932123025,
127.278584916578));
#230513=CARTESIAN_POINT('Ctrl Pts',(-13.6801617377531,0.0530125053692662,
124.198966949783));
#230514=CARTESIAN_POINT('Ctrl Pts',(-13.958609361566,-5.5286502131212,127.189383072259));
#230515=CARTESIAN_POINT('Ctrl Pts',(-14.2370569853788,-6.02975347533148,
133.501786957402));
#230516=CARTESIAN_POINT('Ctrl Pts',(-14.5155046091917,-0.989807863545592,
137.335387812837));
#230517=CARTESIAN_POINT('Ctrl Pts',(-14.7939522330047,4.95972282003631,
135.167293734234));
#230518=CARTESIAN_POINT('Ctrl Pts',(-15.0723998568175,6.35151052793477,
128.989877262545));
#230519=CARTESIAN_POINT('Ctrl Pts',(-15.3508474806304,1.9065703492003,124.479882351679));
#230520=CARTESIAN_POINT('Ctrl Pts',(-15.6292951044433,-4.29041483930959,
125.781773999224));
#230521=CARTESIAN_POINT('Ctrl Pts',(-15.9077427282562,-6.54471838891106,
131.699177382027));
#230522=CARTESIAN_POINT('Ctrl Pts',(-16.186190352069,-2.78474546637155,
136.794287872519));
#230523=CARTESIAN_POINT('Ctrl Pts',(-16.464637975882,3.53427249738445,136.384947839923));
#230524=CARTESIAN_POINT('Ctrl Pts',(-16.7430855996949,6.60546669485434,
130.847320776822));
#230525=CARTESIAN_POINT('Ctrl Pts',(-17.0215332235078,3.6065596947407,125.270215426085));
#230526=CARTESIAN_POINT('Ctrl Pts',(-17.2999808473206,-2.7065994746034,
124.778719148295));
#230527=CARTESIAN_POINT('Ctrl Pts',(-17.5784284711336,-6.53252595152224,
129.824493011814));
#230528=CARTESIAN_POINT('Ctrl Pts',(-17.8568760949464,-4.35538021062653,
135.770717335825));
#230529=CARTESIAN_POINT('Ctrl Pts',(-18.1353237187593,1.82414717168286,
137.153102455769));
#230530=CARTESIAN_POINT('Ctrl Pts',(-18.4137713425722,6.32737241775927,
132.701303979686));
#230531=CARTESIAN_POINT('Ctrl Pts',(-18.6922189663851,5.01605152124203,
126.506307224649));
#230532=CARTESIAN_POINT('Ctrl Pts',(-18.9706665901979,-0.904775675556959,
124.261011566121));
#230533=CARTESIAN_POINT('Ctrl Pts',(-19.2491142140109,-5.99415822726801,
128.028734025499));
#230534=CARTESIAN_POINT('Ctrl Pts',(-19.5275618378238,-5.57520219902858,
134.347121726088));
#230535=CARTESIAN_POINT('Ctrl Pts',(-19.8060094616367,-0.0329077136511566,
137.409885041447));
#230536=CARTESIAN_POINT('Ctrl Pts',(-20.0844570854496,5.53962735294063,
134.402494109067));
#230537=CARTESIAN_POINT('Ctrl Pts',(-20.3629047092624,6.02151550802112,
128.08859427659));
#230538=CARTESIAN_POINT('Ctrl Pts',(-20.6413523330754,0.969925078616457,
124.270351038909));
#230539=CARTESIAN_POINT('Ctrl Pts',(-20.9197999568882,-4.9729791145623,
126.456543399899));
#230540=CARTESIAN_POINT('Ctrl Pts',(-21.1982475807011,-6.34595844499429,
132.638167381246));
#230541=CARTESIAN_POINT('Ctrl Pts',(-21.476695204514,-1.88731198178147,
137.134612533211));
#230542=CARTESIAN_POINT('Ctrl Pts',(-21.7551428283269,4.30568199237261,
135.813865424697));
#230543=CARTESIAN_POINT('Ctrl Pts',(-22.0335904521398,6.54196455979519,
129.889628126344));
#230544=CARTESIAN_POINT('Ctrl Pts',(-22.3120380759527,2.766501289502,124.805985300257));
#230545=CARTESIAN_POINT('Ctrl Pts',(-22.5904856997656,-3.5512415147419,
125.234556353852));
#230546=CARTESIAN_POINT('Ctrl Pts',(-22.8689333235784,-6.60556685473091,
130.781505425734));
#230547=CARTESIAN_POINT('Ctrl Pts',(-23.1473809473914,-3.58969895510304,
136.349457302372));
#230548=CARTESIAN_POINT('Ctrl Pts',(-23.4258285712042,2.7249269177212,136.821736218705));
#230549=CARTESIAN_POINT('Ctrl Pts',(-23.7042761950172,6.53547807324032,
131.764340922733));
#230550=CARTESIAN_POINT('Ctrl Pts',(-23.98272381883,4.34024415530499,125.824770623956));
#230551=CARTESIAN_POINT('Ctrl Pts',(-24.2611714426429,-1.84346210864104,
124.461200262812));
#230552=CARTESIAN_POINT('Ctrl Pts',(-24.5396190664558,-6.33311675287646,
128.926684387076));
#230553=CARTESIAN_POINT('Ctrl Pts',(-24.8180666902687,-5.00294649117208,
135.117661237576));
#230554=CARTESIAN_POINT('Ctrl Pts',(-25.0965143140816,0.924687188395989,
137.344925534737));
#230555=CARTESIAN_POINT('Ctrl Pts',(-25.3749619378945,6.00257851530871,
133.561730197376));
#230556=CARTESIAN_POINT('Ctrl Pts',(-25.6534095617074,5.56439342891538,
127.244646921163));
#230557=CARTESIAN_POINT('Ctrl Pts',(-25.9318571855203,0.0128026170801758,
124.198766630261));
#230558=CARTESIAN_POINT('Ctrl Pts',(-26.2103048093331,-5.5505531744091,
127.223104512485));
#230559=CARTESIAN_POINT('Ctrl Pts',(-26.4887524331461,-6.01322175821376,
133.538441801192));
#230560=CARTESIAN_POINT('Ctrl Pts',(-26.7672000569589,-0.950033308434149,
137.341292049436));
#230561=CARTESIAN_POINT('Ctrl Pts',(-27.0456476807718,4.98618934008908,
135.137021658645));
#230562=CARTESIAN_POINT('Ctrl Pts',(-27.3240953045847,6.34034757396176,
128.951247433362));
#230563=CARTESIAN_POINT('Ctrl Pts',(-27.6025429283976,1.86803613056208,
124.468393694749));
#230564=CARTESIAN_POINT('Ctrl Pts',(-27.8809905522105,-4.32090925818572,
125.807984029013));
#230565=CARTESIAN_POINT('Ctrl Pts',(-28.1594381760234,-6.53915012681315,
131.739000361591));
#230566=CARTESIAN_POINT('Ctrl Pts',(-28.4378857998363,-2.74823148414282,
136.811128429099));
#230567=CARTESIAN_POINT('Ctrl Pts',(-28.7163334236492,3.56817763388296,
136.36333032473));
#230568=CARTESIAN_POINT('Ctrl Pts',(-28.994781047462,6.60560582153853,130.807110630244));
#230569=CARTESIAN_POINT('Ctrl Pts',(-29.273228671275,3.5728049609845,125.248363808452));
#230570=CARTESIAN_POINT('Ctrl Pts',(-29.5516762950878,-2.74322911748845,
124.795306628702));
#230571=CARTESIAN_POINT('Ctrl Pts',(-29.8301239189007,-6.53836965118233,
129.86427650611));
#230572=CARTESIAN_POINT('Ctrl Pts',(-30.1085715427137,-4.32506789255462,
135.797137756284));
#230573=CARTESIAN_POINT('Ctrl Pts',(-30.3870191665265,1.862759968018,137.141880726698));
#230574=CARTESIAN_POINT('Ctrl Pts',(-30.6654667903394,6.33880241886542,
132.662752321889));
#230575=CARTESIAN_POINT('Ctrl Pts',(-30.9439144141524,4.98979511448915,
126.475852728289));
#230576=CARTESIAN_POINT('Ctrl Pts',(-31.2223620379652,-0.944590135059391,
124.266640425567));
#230577=CARTESIAN_POINT('Ctrl Pts',(-31.5008096617781,-6.01094319628198,
128.065273593905));
#230578=CARTESIAN_POINT('Ctrl Pts',(-31.7792572855909,-5.55353311102158,
134.380993925146));
#230579=CARTESIAN_POINT('Ctrl Pts',(-32.0577049094039,0.00730259809219468,
137.409962974972));
#230580=CARTESIAN_POINT('Ctrl Pts',(-32.3361525332168,5.56142757631112,
134.368706159956));
#230581=CARTESIAN_POINT('Ctrl Pts',(-32.6146001570296,6.0048723027414,128.051989919443));
#230582=CARTESIAN_POINT('Ctrl Pts',(-32.8930477808425,0.930132737272799,
124.264567889721));
#230583=CARTESIAN_POINT('Ctrl Pts',(-33.1714954046555,-4.99935337423901,
126.486895890252));
#230584=CARTESIAN_POINT('Ctrl Pts',(-33.4499430284683,-6.33467796681538,
132.676763055306));
#230585=CARTESIAN_POINT('Ctrl Pts',(-33.7283906522812,-1.84874297411136,
137.145983852021));
#230586=CARTESIAN_POINT('Ctrl Pts',(-34.0068382760941,4.33609649568588,
135.787562701789));
#230587=CARTESIAN_POINT('Ctrl Pts',(-34.285285899907,6.53627511603778,129.849822279112));
#230588=CARTESIAN_POINT('Ctrl Pts',(-34.5637335237199,2.72993621954223,
124.789255957683));
#230589=CARTESIAN_POINT('Ctrl Pts',(-34.8421811475328,-3.58508069791401,
125.256276964487));
#230590=CARTESIAN_POINT('Ctrl Pts',(-35.1206287713457,-6.60558359491616,
130.821715809516));
#230591=CARTESIAN_POINT('Ctrl Pts',(-35.3990763951586,-3.55587786888901,
136.37120608099));
#230592=CARTESIAN_POINT('Ctrl Pts',(-35.6775240189714,2.76150590435573,
136.805037327097));
#230593=CARTESIAN_POINT('Ctrl Pts',(-35.9559716427844,6.54120065856107,
131.724539826499));
#230594=CARTESIAN_POINT('Ctrl Pts',(-36.2344192665972,4.30985156296601,
125.798442586144));
#230595=CARTESIAN_POINT('Ctrl Pts',(-36.5128668904101,-1.8820405710409,
124.472539463974));
#230596=CARTESIAN_POINT('Ctrl Pts',(-36.791314514223,-6.3444293630544,128.965270655295));
#230597=CARTESIAN_POINT('Ctrl Pts',(-37.0697621380359,-4.9765975130263,
135.148035677403));
#230598=CARTESIAN_POINT('Ctrl Pts',(-37.3482097618488,0.964484331168655,
137.339175519844));
#230599=CARTESIAN_POINT('Ctrl Pts',(-37.6266573856617,6.0192521926987,133.525139710547));
#230600=CARTESIAN_POINT('Ctrl Pts',(-37.9051050094746,5.54262134595571,
127.210840832248));
#230601=CARTESIAN_POINT('Ctrl Pts',(-38.1835526332875,-0.0274077456145885,
124.198811083455));
#230602=CARTESIAN_POINT('Ctrl Pts',(-38.4620002571004,-5.5722504579079,
127.256958657474));
#230603=CARTESIAN_POINT('Ctrl Pts',(-38.7404478809132,-5.99646721895241,
133.574995332598));
#230604=CARTESIAN_POINT('Ctrl Pts',(-39.0188955047262,-0.910223549489097,
137.346954057637));
#230605=CARTESIAN_POINT('Ctrl Pts',(-39.297343128539,5.0124710950622,135.106589034709));
#230606=CARTESIAN_POINT('Ctrl Pts',(-39.5757907523519,6.32894967607775,
128.912686271968));
#230607=CARTESIAN_POINT('Ctrl Pts',(-39.8542383761648,1.82943269115809,
124.457139819403));
#230608=CARTESIAN_POINT('Ctrl Pts',(-40.1326859999777,-4.35124356418029,
125.834379201373));
#230609=CARTESIAN_POINT('Ctrl Pts',(-40.4111336237906,-6.53333955410249,
131.778788707735));
#230610=CARTESIAN_POINT('Ctrl Pts',(-40.6895812476035,-2.7116156651858,
136.827746402689));
#230611=CARTESIAN_POINT('Ctrl Pts',(-40.9680288714165,3.60195055024708,
136.34150681987));
#230612=CARTESIAN_POINT('Ctrl Pts',(-41.2464764952292,6.60550017506977,
130.766900381762));
#230613=CARTESIAN_POINT('Ctrl Pts',(-41.5249241190422,3.53891783562657,
125.226718070324));
#230614=CARTESIAN_POINT('Ctrl Pts',(-41.803371742855,-2.77975710900975,
124.812116776814));
#230615=CARTESIAN_POINT('Ctrl Pts',(-42.081819366668,-6.5439710691505,129.904094835568));
#230616=CARTESIAN_POINT('Ctrl Pts',(-42.3602669904808,-4.2945953075014,
135.82337316755));
#230617=CARTESIAN_POINT('Ctrl Pts',(-42.6387146142937,1.90130373909722,
137.130424158489));
#230618=CARTESIAN_POINT('Ctrl Pts',(-42.9171622381066,6.34999753331677,
132.624131800705));
#230619=CARTESIAN_POINT('Ctrl Pts',(-43.1956098619195,4.96335380904355,
126.44555862638));
#230620=CARTESIAN_POINT('Ctrl Pts',(-43.4740574857324,-0.984369592426984,
124.272511542639));
#230621=CARTESIAN_POINT('Ctrl Pts',(-43.7525051095453,-6.02750542758532,
128.101914660188));
#230622=CARTESIAN_POINT('Ctrl Pts',(-44.0309527333582,-5.53165823480283,
134.414733590743));
#230623=CARTESIAN_POINT('Ctrl Pts',(-44.3094003571711,0.0475126392350714,
137.409796135472));
#230624=CARTESIAN_POINT('Ctrl Pts',(-44.5878479809839,5.58302171893757,
134.334786132711));
#230625=CARTESIAN_POINT('Ctrl Pts',(-44.8662956047969,5.98800658471021,
128.015487552405));
#230626=CARTESIAN_POINT('Ctrl Pts',(-45.1447432286098,0.890305929518511,
124.259027074959));
#230627=CARTESIAN_POINT('Ctrl Pts',(-45.4231908524226,-5.02554238103793,
126.517408365848));
#230628=CARTESIAN_POINT('Ctrl Pts',(-45.7016384762356,-6.32316275481482,
132.715289346806));
#230629=CARTESIAN_POINT('Ctrl Pts',(-45.9800861000484,-1.81010546059046,
137.15712017965));
#230630=CARTESIAN_POINT('Ctrl Pts',(-46.2585337238614,4.36635032334889,
135.761075324496));
#230631=CARTESIAN_POINT('Ctrl Pts',(-46.5369813476741,6.53034346820225,
129.810051802649));
#230632=CARTESIAN_POINT('Ctrl Pts',(-46.8154289714873,2.6932699907919,124.772749507024));
#230633=CARTESIAN_POINT('Ctrl Pts',(-47.0938765952999,-3.61878703460243,
125.278203161403));
#230634=CARTESIAN_POINT('Ctrl Pts',(-47.3723242191129,-6.60535556277213,
130.861925550195));
#230635=CARTESIAN_POINT('Ctrl Pts',(-47.6507718429257,-3.52192501831287,
136.392748578105));
#230636=CARTESIAN_POINT('Ctrl Pts',(-47.9292194667387,2.79798256237344,
136.788116078208));
#230637=CARTESIAN_POINT('Ctrl Pts',(-48.2076670905515,6.54668085728591,
131.684704632686));
#230638=CARTESIAN_POINT('Ctrl Pts',(-48.4861147143645,4.27929926749242,
125.772300044465));
#230639=CARTESIAN_POINT('Ctrl Pts',(-48.7645623381774,-1.92054929373528,
124.484113293097));
#230640=CARTESIAN_POINT('Ctrl Pts',(-49.0430099619902,-6.35550687806913,
129.003925071669));
#230641=CARTESIAN_POINT('Ctrl Pts',(-49.3214575858032,-4.95006412522954,
135.178249160753));
#230642=CARTESIAN_POINT('Ctrl Pts',(-49.5999052096159,1.00424573461974,
137.333183354982));
#230643=CARTESIAN_POINT('Ctrl Pts',(-49.878352833429,6.03570282448511,133.488448404247));
#230644=CARTESIAN_POINT('Ctrl Pts',(-50.1568004572417,5.52064387912377,
127.17716790253));
#230645=CARTESIAN_POINT('Ctrl Pts',(-50.4352480810547,-0.0676170927052693,
124.199100307716));
#230646=CARTESIAN_POINT('Ctrl Pts',(-50.7136957048675,-5.5937412596168,
127.290944252747));
#230647=CARTESIAN_POINT('Ctrl Pts',(-50.9921433286805,-5.97949047839309,
133.611446197116));
#230648=CARTESIAN_POINT('Ctrl Pts',(-51.2705909524933,-0.870380061875472,
137.352373627632));
#230649=CARTESIAN_POINT('Ctrl Pts',(-51.5490385763063,5.03856711107574,
135.075996990117));
#230650=CARTESIAN_POINT('Ctrl Pts',(-51.8274862001192,6.31731725663583,
128.874195207264));
#230651=CARTESIAN_POINT('Ctrl Pts',(-52.105933823932,1.79076146145295,124.446121142656));
#230652=CARTESIAN_POINT('Ctrl Pts',(-52.3843814477449,-4.38141663324442,
125.860958538224));
#230653=CARTESIAN_POINT('Ctrl Pts',(-52.6628290715579,-6.52728688609205,
131.818540946088));
#230654=CARTESIAN_POINT('Ctrl Pts',(-52.9412766953706,-2.67489936631311,
136.844141177504));
#230655=CARTESIAN_POINT('Ctrl Pts',(-53.2197243191836,3.63558999500893,
136.319478134021));
#230656=CARTESIAN_POINT('Ctrl Pts',(-53.4981719429964,6.60514975936288,
130.726691521383));
#230657=CARTESIAN_POINT('Ctrl Pts',(-53.7766195668094,3.50489957436681,
125.205279013792));
#230658=CARTESIAN_POINT('Ctrl Pts',(-54.0550671906223,-2.8161820956091,
124.829148969725));
#230659=CARTESIAN_POINT('Ctrl Pts',(-54.3335148144351,-6.54932999786417,
129.943946524707));
#230660=CARTESIAN_POINT('Ctrl Pts',(-54.6119624382481,-4.26396358463975,
135.849422597461));
#230661=CARTESIAN_POINT('Ctrl Pts',(-54.890410062061,1.93977705666721,137.11873317567));
#230662=CARTESIAN_POINT('Ctrl Pts',(-55.1688576858738,6.3609573462743,132.58544384723));
#230663=CARTESIAN_POINT('Ctrl Pts',(-55.4473053096868,4.93672858469731,
126.415426041482));
#230664=CARTESIAN_POINT('Ctrl Pts',(-55.7257529334997,-1.02411257361735,
124.278624699781));
#230665=CARTESIAN_POINT('Ctrl Pts',(-56.0042005573125,-6.0438443074584,
128.138655866601));
#230666=CARTESIAN_POINT('Ctrl Pts',(-56.2826481811254,-5.50957838095395,
134.448339472641));
#230667=CARTESIAN_POINT('Ctrl Pts',(-56.5610958049383,0.0877209197796484,
137.40938452913));
#230668=CARTESIAN_POINT('Ctrl Pts',(-56.8395434287512,5.60440898064107,
134.300735284249));
#230669=CARTESIAN_POINT('Ctrl Pts',(-57.117991052564,5.97091897889293,127.979088528083));
#230670=CARTESIAN_POINT('Ctrl Pts',(-57.396438676377,0.850446131150592,
124.253728799937));
#230671=CARTESIAN_POINT('Ctrl Pts',(-57.6748863001899,-5.05154516451579,
126.548079696037));
#230672=CARTESIAN_POINT('Ctrl Pts',(-57.9533339240027,-6.31141323569307,
132.753744828139));
#230673=CARTESIAN_POINT('Ctrl Pts',(-58.2317815478157,-1.77140087294607,
137.168021103437));
#230674=CARTESIAN_POINT('Ctrl Pts',(-58.5102291716285,4.39644235429495,
135.734404274317));
#230675=CARTESIAN_POINT('Ctrl Pts',(-58.7886767954414,6.52416983608798,
129.770318170665));
#230676=CARTESIAN_POINT('Ctrl Pts',(-59.0671244192543,2.65650396193163,
124.756466559932));
#230677=CARTESIAN_POINT('Ctrl Pts',(-59.3455720430672,-3.6523592758065,
125.300334132115));
#230678=CARTESIAN_POINT('Ctrl Pts',(-59.62401966688,-6.60488276674858,130.902133157784));
#230679=CARTESIAN_POINT('Ctrl Pts',(-59.902467290693,-3.48784166150989,
136.414083995446));
#230680=CARTESIAN_POINT('Ctrl Pts',(-60.1809149145059,2.83435554011865,
136.770973099059));
#230681=CARTESIAN_POINT('Ctrl Pts',(-60.4593625383188,6.55191846634393,
131.644836817403));
#230682=CARTESIAN_POINT('Ctrl Pts',(-60.7378101621316,4.24858840101079,
125.746343967642));
#230683=CARTESIAN_POINT('Ctrl Pts',(-61.0162577859445,-1.95898684976931,
124.49592132131));
#230684=CARTESIAN_POINT('Ctrl Pts',(-61.2947054097575,-6.36634888743926,
129.042646203845));
#230685=CARTESIAN_POINT('Ctrl Pts',(-61.5731530335703,-4.92334731098624,
135.208300568055));
#230686=CARTESIAN_POINT('Ctrl Pts',(-61.8516006573832,1.04396992537583,
137.326949262193));
#230687=CARTESIAN_POINT('Ctrl Pts',(-62.1300482811962,6.05192980108374,
133.451657638088));
#230688=CARTESIAN_POINT('Ctrl Pts',(-62.408495905009,5.49846184280268,127.143629379772));
#230689=CARTESIAN_POINT('Ctrl Pts',(-62.6869435288219,-0.107823934219708,
124.199634292325));
#230690=CARTESIAN_POINT('Ctrl Pts',(-62.9653911526347,-5.61502478318622,
127.325060038955));
#230691=CARTESIAN_POINT('Ctrl Pts',(-63.2438387764477,-5.96229216561512,
133.647793044045));
#230692=CARTESIAN_POINT('Ctrl Pts',(-63.5222864002605,-0.830504322008783,
137.357550558596));
#230693=CARTESIAN_POINT('Ctrl Pts',(-63.8007340240734,5.06447642113188,
135.045246658467));
#230694=CARTESIAN_POINT('Ctrl Pts',(-64.0791816478864,6.30545074667997,
128.835775665549));
#230695=CARTESIAN_POINT('Ctrl Pts',(-64.3576292716992,1.75202387442331,
124.435338072814));
#230696=CARTESIAN_POINT('Ctrl Pts',(-64.6360768955121,-4.41142734730395,
125.887721054655));
#230697=CARTESIAN_POINT('Ctrl Pts',(-64.914524519325,-6.52099234706562,
131.858255603616));
#230698=CARTESIAN_POINT('Ctrl Pts',(-65.1929721431379,-2.63808394806071,
136.860312146029));
#230699=CARTESIAN_POINT('Ctrl Pts',(-65.4714197669508,3.66909472164654,
136.297245083462));
#230700=CARTESIAN_POINT('Ctrl Pts',(-65.7498673907637,6.60455458740261,
130.686485539062));
#230701=CARTESIAN_POINT('Ctrl Pts',(-66.0283150145766,3.4707514377644,125.184047433287));
#230702=CARTESIAN_POINT('Ctrl Pts',(-66.3067626383895,-2.85250272754526,
124.846402576302));
#230703=CARTESIAN_POINT('Ctrl Pts',(-66.5852102622024,-6.55444623874626,
129.983830096806));
#230704=CARTESIAN_POINT('Ctrl Pts',(-66.8636578860152,-4.23317385903938,
135.875285080744));
#230705=CARTESIAN_POINT('Ctrl Pts',(-67.1421055098281,1.978178495085,137.106808211453));
#230706=CARTESIAN_POINT('Ctrl Pts',(-67.4205531336411,6.37168145161813,
132.546689895061));
#230707=CARTESIAN_POINT('Ctrl Pts',(-67.6990007574539,4.90992042805787,
126.385456090168));
#230708=CARTESIAN_POINT('Ctrl Pts',(-67.9774483812669,-1.06381760593968,
124.284979670466));
#230709=CARTESIAN_POINT('Ctrl Pts',(-68.2558960050797,-6.05995923045808,
128.175495851683));
#230710=CARTESIAN_POINT('Ctrl Pts',(-68.5343436288926,-5.48729436765201,
134.481810325563));
#230711=CARTESIAN_POINT('Ctrl Pts',(-68.8127912527054,0.12792594979327,
137.408728171199));
#230712=CARTESIAN_POINT('Ctrl Pts',(-69.0912388765185,5.62558856890878,
134.266554876337));
#230713=CARTESIAN_POINT('Ctrl Pts',(-69.3696865003312,5.9536101184771,127.942794195258));
#230714=CARTESIAN_POINT('Ctrl Pts',(-69.6481341241442,0.810554819188534,
124.248673260987));
#230715=CARTESIAN_POINT('Ctrl Pts',(-69.9265817479571,-5.07736076112986,
126.578908744281));
#230716=CARTESIAN_POINT('Ctrl Pts',(-70.2050293717699,-6.29942984483285,
132.792128074323));
#230717=CARTESIAN_POINT('Ctrl Pts',(-70.4834769955829,-1.73263064539088,
137.178686219444));
#230718=CARTESIAN_POINT('Ctrl Pts',(-70.7619246193956,4.42637147345276,
135.707550539556));
#230719=CARTESIAN_POINT('Ctrl Pts',(-71.0403722432087,6.51775444846118,
129.730622855503));
#230720=CARTESIAN_POINT('Ctrl Pts',(-71.3188198670216,2.6196394953401,124.740407719779));
#230721=CARTESIAN_POINT('Ctrl Pts',(-71.5972674908343,-3.68579617749442,
125.322669056552));
#230722=CARTESIAN_POINT('Ctrl Pts',(-71.8757151146474,-6.6041652243652,
130.942337142376));
#230723=CARTESIAN_POINT('Ctrl Pts',(-72.1541627384602,-3.45362906145158,
136.435211542427));
#230724=CARTESIAN_POINT('Ctrl Pts',(-72.4326103622731,2.87062348977667,
136.753609024891));
#230725=CARTESIAN_POINT('Ctrl Pts',(-72.711057986086,6.55691329165398,131.604937857965));
#230726=CARTESIAN_POINT('Ctrl Pts',(-72.9895056098989,4.21772010152317,
125.720575317484));
#230727=CARTESIAN_POINT('Ctrl Pts',(-73.2679532337117,-1.99735181482566,
124.50796311106));
#230728=CARTESIAN_POINT('Ctrl Pts',(-73.5464008575247,-6.37695498941029,
129.081432616995));
#230729=CARTESIAN_POINT('Ctrl Pts',(-73.8248484813376,-4.89644806029751,
135.238188785743));
#230730=CARTESIAN_POINT('Ctrl Pts',(-74.1032961051504,1.08365543144292,
137.320473472483));
#230731=CARTESIAN_POINT('Ctrl Pts',(-74.3817437289633,6.06793252119795,
133.414768775364));
#230732=CARTESIAN_POINT('Ctrl Pts',(-74.6601913527762,5.47607605895596,
127.110226506756));
#230733=CARTESIAN_POINT('Ctrl Pts',(-74.9386389765891,-0.148026780279403,
124.200413017498));
#230734=CARTESIAN_POINT('Ctrl Pts',(-75.217086600402,-5.63610023994771,
127.359304751927));
#230735=CARTESIAN_POINT('Ctrl Pts',(-75.4955342242149,-5.94487291790794,
133.684034526541));
#230736=CARTESIAN_POINT('Ctrl Pts',(-75.7739818480278,-0.790597807498519,
137.362484658699));
#230737=CARTESIAN_POINT('Ctrl Pts',(-76.0524294718406,5.09019806515201,
135.014339179226));
#230738=CARTESIAN_POINT('Ctrl Pts',(-76.3308770956536,6.29335058592772,
128.797429070474));
#230739=CARTESIAN_POINT('Ctrl Pts',(-76.6093247194664,1.71322136550425,
124.424791009442));
#230740=CARTESIAN_POINT('Ctrl Pts',(-76.8877723432794,-4.44127459430165,
125.914665758975));
#230741=CARTESIAN_POINT('Ctrl Pts',(-77.1662199670922,-6.51445617026952,
131.89793120868));
#230742=CARTESIAN_POINT('Ctrl Pts',(-77.4446675909052,-2.60117077463652,
136.876258709042));
#230743=CARTESIAN_POINT('Ctrl Pts',(-77.7231152147181,3.7024634886308,136.274808492052));
#230744=CARTESIAN_POINT('Ctrl Pts',(-78.0015628385308,6.60371468124315,
130.646283924643));
#230745=CARTESIAN_POINT('Ctrl Pts',(-78.2800104623438,3.43647469119047,
125.163024115555));
#230746=CARTESIAN_POINT('Ctrl Pts',(-78.5584580861567,-2.88871765894464,
124.863876957204));
#230747=CARTESIAN_POINT('Ctrl Pts',(-78.8369057099696,-6.55931960221255,
130.023744073965));
#230748=CARTESIAN_POINT('Ctrl Pts',(-79.1153533337825,-4.20222727162433,
135.900959659057));
#230749=CARTESIAN_POINT('Ctrl Pts',(-79.3938009575953,2.01650663137172,
137.094649707722));
#230750=CARTESIAN_POINT('Ctrl Pts',(-79.6722485814083,6.38216945196263,
132.507871380239));
#230751=CARTESIAN_POINT('Ctrl Pts',(-79.9506962052212,4.88293033251105,
126.355649882987));
#230752=CARTESIAN_POINT('Ctrl Pts',(-80.229143829034,-1.10348321810992,
124.29157621921));
#230753=CARTESIAN_POINT('Ctrl Pts',(-80.507591452847,-6.07584959944043,
128.212433250316));
#230754=CARTESIAN_POINT('Ctrl Pts',(-80.7860390766598,-5.46480702063872,
134.515144909234));
#230755=CARTESIAN_POINT('Ctrl Pts',(-81.0644867004727,0.168126239464741,
137.407827085998));
#230756=CARTESIAN_POINT('Ctrl Pts',(-81.3429343242857,5.64655969892388,
134.232246175545));
#230757=CARTESIAN_POINT('Ctrl Pts',(-81.6213819480984,5.93608064484842,
127.906605898828));
#230758=CARTESIAN_POINT('Ctrl Pts',(-81.8998295719115,0.770633471818905,
124.243860645443));
#230759=CARTESIAN_POINT('Ctrl Pts',(-82.1782771957242,-5.10298821427442,
126.609894368197));
#230760=CARTESIAN_POINT('Ctrl Pts',(-82.4567248195372,-6.28721302628274,
132.830437663053));
#230761=CARTESIAN_POINT('Ctrl Pts',(-82.7351724433501,-1.69379621456928,
137.189115132473));
#230762=CARTESIAN_POINT('Ctrl Pts',(-83.0136200671628,4.45613657178832,
135.680515115291));
#230763=CARTESIAN_POINT('Ctrl Pts',(-83.2920676909759,6.51109754304618,
129.690967328089));
#230764=CARTESIAN_POINT('Ctrl Pts',(-83.5705153147887,2.58267795704331,
124.724573581631));
#230765=CARTESIAN_POINT('Ctrl Pts',(-83.8489629386017,-3.71909650065006,
125.345207107088));
#230766=CARTESIAN_POINT('Ctrl Pts',(-84.1274105624144,-6.60320296221082,
130.982536014198));
#230767=CARTESIAN_POINT('Ctrl Pts',(-84.4058581862275,-3.41928848589759,
136.456130436155));
#230768=CARTESIAN_POINT('Ctrl Pts',(-84.6843058100402,2.90678506742617,
136.736024499134));
#230769=CARTESIAN_POINT('Ctrl Pts',(-84.9627534338533,6.56166514813073,
131.565009232842));
#230770=CARTESIAN_POINT('Ctrl Pts',(-85.241201057666,4.1866955128661,125.694995048862));
#230771=CARTESIAN_POINT('Ctrl Pts',(-85.519648681479,-2.03564276727566,
124.520238216135));
#230772=CARTESIAN_POINT('Ctrl Pts',(-85.7980963052919,-6.38732479096924,
129.120282873878));
#230773=CARTESIAN_POINT('Ctrl Pts',(-86.0765439291047,-4.8693673699251,
135.267912706297));
#230774=CARTESIAN_POINT('Ctrl Pts',(-86.3549915529177,1.12330078225909,
137.313756225814));
#230775=CARTESIAN_POINT('Ctrl Pts',(-86.6334391767305,6.08371039184151,
133.377783183006));
#230776=CARTESIAN_POINT('Ctrl Pts',(-86.9118868005434,5.45348735709659,
127.076960521238));
#230777=CARTESIAN_POINT('Ctrl Pts',(-87.1903344243564,-0.188224141151809,
124.201436454379));
#230778=CARTESIAN_POINT('Ctrl Pts',(-87.4687820481692,-5.65696684894189,
127.39367712271));
#230779=CARTESIAN_POINT('Ctrl Pts',(-87.7472296719821,-5.92723338074904,
133.720169301662));
#230780=CARTESIAN_POINT('Ctrl Pts',(-88.0256772957949,-0.750661997095914,
137.367175745102));
#230781=CARTESIAN_POINT('Ctrl Pts',(-88.3041249196079,5.11573109001074,
134.983275697681));
#230782=CARTESIAN_POINT('Ctrl Pts',(-88.5825725434208,6.28101722275544,
128.759156842984));
#230783=CARTESIAN_POINT('Ctrl Pts',(-88.8610201672337,1.67435537253749,
124.414480343369));
#230784=CARTESIAN_POINT('Ctrl Pts',(-89.1394677910466,-4.47095726823472,
125.941791652735));
#230785=CARTESIAN_POINT('Ctrl Pts',(-89.4179154148595,-6.50767859790483,
131.93756629108));
#230786=CARTESIAN_POINT('Ctrl Pts',(-89.6963630386723,-2.56416121387375,
136.891980275641));
#230787=CARTESIAN_POINT('Ctrl Pts',(-89.9748106624853,3.73569505946763,
136.252169191183));
#230788=CARTESIAN_POINT('Ctrl Pts',(-90.253258286298,6.60263007200808,130.606088167816));
#230789=CARTESIAN_POINT('Ctrl Pts',(-90.5317059101111,3.40207060478355,
125.142209839621));
#230790=CARTESIAN_POINT('Ctrl Pts',(-90.8101535339238,-2.9248255478482,
124.881571464914));
#230791=CARTESIAN_POINT('Ctrl Pts',(-91.0886011577368,-6.56394990767886,
130.063686977158));
#230792=CARTESIAN_POINT('Ctrl Pts',(-91.3670487815497,-4.17112496913288,
135.926445381018));
#230793=CARTESIAN_POINT('Ctrl Pts',(-91.6454964053626,2.05476004526333,
137.082258115016));
#230794=CARTESIAN_POINT('Ctrl Pts',(-91.9239440291755,6.39242095867105,
132.468989741201));
#230795=CARTESIAN_POINT('Ctrl Pts',(-92.2023916529884,4.85575929818535,
126.326008524418));
#230796=CARTESIAN_POINT('Ctrl Pts',(-92.4808392768012,-1.14310794030347,
124.298414101576));
#230797=CARTESIAN_POINT('Ctrl Pts',(-92.7592869006141,-6.09151482558059,
128.249466693771));
#230798=CARTESIAN_POINT('Ctrl Pts',(-93.0377345244271,-5.44211717319261,
134.548341988427));
#230799=CARTESIAN_POINT('Ctrl Pts',(-93.3161821482399,0.208320299155509,
137.406681306919));
#230800=CARTESIAN_POINT('Ctrl Pts',(-93.5946297720528,5.6673215935918,134.197810453193));
#230801=CARTESIAN_POINT('Ctrl Pts',(-93.8730773958657,5.91833120756931,
127.870524979765));
#230802=CARTESIAN_POINT('Ctrl Pts',(-94.1515250196785,0.730683568342929,
124.239291131637));
#230803=CARTESIAN_POINT('Ctrl Pts',(-94.4299726434915,-5.12842657431339,
126.641035419604));
#230804=CARTESIAN_POINT('Ctrl Pts',(-94.7084202673044,-6.27476323274215,
132.868672174754));
#230805=CARTESIAN_POINT('Ctrl Pts',(-94.9868678911172,-1.6548990195065,
137.199307456074));
#230806=CARTESIAN_POINT('Ctrl Pts',(-95.2653155149302,4.48573654634406,
135.653299003326));
#230807=CARTESIAN_POINT('Ctrl Pts',(-95.543763138743,6.50419936651746,129.651353057874));
#230808=CARTESIAN_POINT('Ctrl Pts',(-95.822210762556,2.54562071666526,124.708964732227));
#230809=CARTESIAN_POINT('Ctrl Pts',(-96.1006583863688,-3.75225901131679,
125.367947448562));
#230810=CARTESIAN_POINT('Ctrl Pts',(-96.3791060101818,-6.60199601594203,
131.022728283664));
#230811=CARTESIAN_POINT('Ctrl Pts',(-96.6575536339946,-3.38482120735248,
136.476839901474));
#230812=CARTESIAN_POINT('Ctrl Pts',(-96.9360012578075,2.94283893308538,
136.718220173391));
#230813=CARTESIAN_POINT('Ctrl Pts',(-97.2144488816204,6.5661738596919,131.525052421605));
#230814=CARTESIAN_POINT('Ctrl Pts',(-97.4928965054334,4.15551578466796,
125.669604109659));
#230815=CARTESIAN_POINT('Ctrl Pts',(-97.771344129246,-2.07385828823457,
124.532746181678));
#230816=CARTESIAN_POINT('Ctrl Pts',(-98.0497917530593,-6.39745790785863,
129.15919553488));
#230817=CARTESIAN_POINT('Ctrl Pts',(-98.3282393768718,-4.84210624335443,
135.297471228287));
#230818=CARTESIAN_POINT('Ctrl Pts',(-98.606687000685,1.16290450875192,137.306797771098));
#230819=CARTESIAN_POINT('Ctrl Pts',(-98.8851346244975,6.09926282835875,
133.340702231527));
#230820=CARTESIAN_POINT('Ctrl Pts',(-99.1635822483109,5.43069657425812,
127.043832655902));
#230821=CARTESIAN_POINT('Ctrl Pts',(-99.4420298721233,-0.228414527308866,
124.202704565042));
#230822=CARTESIAN_POINT('Ctrl Pts',(-99.7204774959365,-5.67762383694899,
127.428175877623));
#230823=CARTESIAN_POINT('Ctrl Pts',(-99.9989251197493,-5.90937420777732,
133.756196030418));
#230824=CARTESIAN_POINT('Ctrl Pts',(-100.277372743562,-0.710698370637635,
137.371623643978));
#230825=CARTESIAN_POINT('Ctrl Pts',(-100.555820367375,5.14107454957247,
134.9520573649));
#230826=CARTESIAN_POINT('Ctrl Pts',(-100.834267991188,6.26845111417983,
128.720960401273));
#230827=CARTESIAN_POINT('Ctrl Pts',(-101.112715615001,1.63542733571746,
124.404406456659));
#230828=CARTESIAN_POINT('Ctrl Pts',(-101.391163238814,-4.50047426920288,
125.969097730777));
#230829=CARTESIAN_POINT('Ctrl Pts',(-101.669610862627,-6.50065988111587,
131.977159382129));
#230830=CARTESIAN_POINT('Ctrl Pts',(-101.94805848644,-2.52705663717401,
136.907476263252));
#230831=CARTESIAN_POINT('Ctrl Pts',(-102.226506110253,3.76878820275105,
136.229328019765));
#230832=CARTESIAN_POINT('Ctrl Pts',(-102.504953734065,6.60130079988703,
130.565899758046));
#230833=CARTESIAN_POINT('Ctrl Pts',(-102.783401357878,3.36754045339959,
125.121605376767));
#230834=CARTESIAN_POINT('Ctrl Pts',(-103.061848981691,-2.96082505626518,
124.899485443752));
#230835=CARTESIAN_POINT('Ctrl Pts',(-103.340296605504,-6.56833698356739,
130.103657326284));
#230836=CARTESIAN_POINT('Ctrl Pts',(-103.618744229317,-4.13986810407194,
135.951741302244));
#230837=CARTESIAN_POINT('Ctrl Pts',(-103.89719185313,2.0929373192654,137.06963389251));
#230838=CARTESIAN_POINT('Ctrl Pts',(-104.175639476943,6.40243559186997,
132.430046418718));
#230839=CARTESIAN_POINT('Ctrl Pts',(-104.454087100755,4.82840833191319,
126.296533112833));
#230840=CARTESIAN_POINT('Ctrl Pts',(-104.732534724569,-1.18269030421136,
124.305493064181));
#230841=CARTESIAN_POINT('Ctrl Pts',(-105.010982348381,-6.10695432839948,
128.286594809759));
#230842=CARTESIAN_POINT('Ctrl Pts',(-105.289429972194,-5.41922566609253,
134.581400333014));
#230843=CARTESIAN_POINT('Ctrl Pts',(-105.567877596007,0.248506639461218,
137.40529087642));
#230844=CARTESIAN_POINT('Ctrl Pts',(-105.84632521982,5.68787348357469,134.163248985309));
#230845=CARTESIAN_POINT('Ctrl Pts',(-106.124772843633,5.90036246435008,
127.834552775061));
#230846=CARTESIAN_POINT('Ctrl Pts',(-106.403220467446,0.690706589119241,
124.234964888896));
#230847=CARTESIAN_POINT('Ctrl Pts',(-106.681668091259,-5.1536748986197,
126.672330744555));
#230848=CARTESIAN_POINT('Ctrl Pts',(-106.960115715072,-6.26208092554253,
132.906830192629));
#230849=CARTESIAN_POINT('Ctrl Pts',(-107.238563338885,-1.61594050155245,
137.209262812568));
#230850=CARTESIAN_POINT('Ctrl Pts',(-107.517010962697,4.51517030028232,
135.625903212168));
#230851=CARTESIAN_POINT('Ctrl Pts',(-107.79545858651,6.49706017448951,129.611781512777));
#230852=CARTESIAN_POINT('Ctrl Pts',(-108.073906210323,2.50846914737518,
124.69358174996));
#230853=CARTESIAN_POINT('Ctrl Pts',(-108.352353834136,-3.78528248064593,
125.390889238328));
#230854=CARTESIAN_POINT('Ctrl Pts',(-108.630801457949,-6.60054443028347,
131.062912461436));
#230855=CARTESIAN_POINT('Ctrl Pts',(-108.909249081762,-3.35022850301195,
136.497339170987));
#230856=CARTESIAN_POINT('Ctrl Pts',(-109.187696705575,2.97878375076591,
136.700196707408));
#230857=CARTESIAN_POINT('Ctrl Pts',(-109.466144329388,6.57043925926657,
131.485068904869));
#230858=CARTESIAN_POINT('Ctrl Pts',(-109.7445919532,4.12418207230337,125.644403440746));
#230859=CARTESIAN_POINT('Ctrl Pts',(-110.023039577014,-2.11199696161116,
124.5454865442));
#230860=CARTESIAN_POINT('Ctrl Pts',(-110.301487200826,-6.40735396459295,
129.198169158078));
#230861=CARTESIAN_POINT('Ctrl Pts',(-110.579934824639,-4.81466569075636,
135.326863256411));
#230862=CARTESIAN_POINT('Ctrl Pts',(-110.858382448452,1.20246514338981,
137.299598366182));
#230863=CARTESIAN_POINT('Ctrl Pts',(-111.136830072265,6.11458925444912,
133.303527294979));
#230864=CARTESIAN_POINT('Ctrl Pts',(-111.415277696078,5.407704554961,127.010844138312));
#230865=CARTESIAN_POINT('Ctrl Pts',(-111.693725319891,-0.268596449482207,
124.204217302498));
#230866=CARTESIAN_POINT('Ctrl Pts',(-111.972172943703,-5.69807043851701,
127.462799738304));
#230867=CARTESIAN_POINT('Ctrl Pts',(-112.250620567517,-5.89129606077132,
133.792113377828));
#230868=CARTESIAN_POINT('Ctrl Pts',(-112.529068191329,-0.670708408989202,
137.375828190507));
#230869=CARTESIAN_POINT('Ctrl Pts',(-112.807515815142,5.16622750472631,
134.920685337692));
#230870=CARTESIAN_POINT('Ctrl Pts',(-113.085963438955,6.25565272584325,
128.682841160722));
#230871=CARTESIAN_POINT('Ctrl Pts',(-113.364411062768,1.5964386975353,124.394569722605));
#230872=CARTESIAN_POINT('Ctrl Pts',(-113.642858686581,-4.52982450344111,
125.996582981263));
#230873=CARTESIAN_POINT('Ctrl Pts',(-113.921306310394,-6.49340027998504,
132.016709014688));
#230874=CARTESIAN_POINT('Ctrl Pts',(-114.199753934207,-2.48985841946147,
136.922746097669));
#230875=CARTESIAN_POINT('Ctrl Pts',(-114.47820155802,3.80174169220082,136.206285824184));
#230876=CARTESIAN_POINT('Ctrl Pts',(-114.756649181833,6.59972691413776,
130.525720184532));
#230877=CARTESIAN_POINT('Ctrl Pts',(-115.035096805645,3.3328855165654,125.101211490497));
#230878=CARTESIAN_POINT('Ctrl Pts',(-115.313544429458,-2.99671485022117,
124.917618229914));
#230879=CARTESIAN_POINT('Ctrl Pts',(-115.591992053271,-6.57248066731354,
130.143653640229));
#230880=CARTESIAN_POINT('Ctrl Pts',(-115.870439677084,-4.10845783467579,
135.976846485386));
#230881=CARTESIAN_POINT('Ctrl Pts',(-116.148887300897,2.13103703870585,
137.056777507999));
#230882=CARTESIAN_POINT('Ctrl Pts',(-116.42733492471,6.41221298046361,132.391042855849));
#230883=CARTESIAN_POINT('Ctrl Pts',(-116.705782548523,4.8008784471946,126.267224740454));
#230884=CARTESIAN_POINT('Ctrl Pts',(-116.984230172336,-1.22222884309565,
124.312812844714));
#230885=CARTESIAN_POINT('Ctrl Pts',(-117.262677796149,-6.12216753577917,
128.323816222486));
#230886=CARTESIAN_POINT('Ctrl Pts',(-117.541125419961,-5.39613334759327,
134.614318718005));
#230887=CARTESIAN_POINT('Ctrl Pts',(-117.819573043774,0.288683771261777,
137.403655846021));
#230888=CARTESIAN_POINT('Ctrl Pts',(-118.098020667587,5.70821460731317,
134.128563052582));
#230889=CARTESIAN_POINT('Ctrl Pts',(-118.3764682914,5.88217508103065,127.79869061768));
#230890=CARTESIAN_POINT('Ctrl Pts',(-118.654915915213,0.650704015508265,
124.230882077529));
#230891=CARTESIAN_POINT('Ctrl Pts',(-118.933363539026,-5.17873225160735,
126.703779183394));
#230892=CARTESIAN_POINT('Ctrl Pts',(-119.211811162839,-6.24916657463125,
132.944910302722));
#230893=CARTESIAN_POINT('Ctrl Pts',(-119.490258786652,-1.57692210432836,
137.218980833058));
#230894=CARTESIAN_POINT('Ctrl Pts',(-119.768706410464,4.54443674292479,
135.598328756974));
#230895=CARTESIAN_POINT('Ctrl Pts',(-120.047154034278,6.48968023150711,
129.572254159139));
#230896=CARTESIAN_POINT('Ctrl Pts',(-120.32560165809,2.47122462583917,124.67842520485));
#230897=CARTESIAN_POINT('Ctrl Pts',(-120.604049281903,-3.81816568494053,
125.414031626265));
#230898=CARTESIAN_POINT('Ctrl Pts',(-120.882496905716,-6.59884825902321,
131.103087058474));
#230899=CARTESIAN_POINT('Ctrl Pts',(-121.160944529529,-3.31551165472302,
136.517627485086));
#230900=CARTESIAN_POINT('Ctrl Pts',(-121.439392153342,3.0146181885189,136.68195476905));
#230901=CARTESIAN_POINT('Ctrl Pts',(-121.717839777155,6.57446118879764,
131.445060164237));
#230902=CARTESIAN_POINT('Ctrl Pts',(-121.996287400968,4.0926955368563,125.619393975946));
#230903=CARTESIAN_POINT('Ctrl Pts',(-122.274735024781,-2.15005737416446,
124.5584588316));
#230904=CARTESIAN_POINT('Ctrl Pts',(-122.553182648593,-6.41701259446945,
129.237202299292));
#230905=CARTESIAN_POINT('Ctrl Pts',(-122.831630272406,-4.7870467289504,
135.356087701536));
#230906=CARTESIAN_POINT('Ctrl Pts',(-123.110077896219,1.24198122024032,
137.292158277842));
#230907=CARTESIAN_POINT('Ctrl Pts',(-123.388525520032,6.1296891021858,133.266259750888));
#230908=CARTESIAN_POINT('Ctrl Pts',(-123.666973143845,5.38451215118288,
126.97799619087));
#230909=CARTESIAN_POINT('Ctrl Pts',(-123.945420767658,-0.30876841871475,
124.20597461069));
#230910=CARTESIAN_POINT('Ctrl Pts',(-124.223868391471,-5.71830589598935,
127.497547421752));
#230911=CARTESIAN_POINT('Ctrl Pts',(-124.502316015284,-5.87299960962311,
133.827920012961));
#230912=CARTESIAN_POINT('Ctrl Pts',(-124.780763639097,-0.630693593994696,
137.379789228888));
#230913=CARTESIAN_POINT('Ctrl Pts',(-125.059211262909,5.19118902341993,
134.889160778557));
#230914=CARTESIAN_POINT('Ctrl Pts',(-125.337658886723,6.24262253199412,
128.644800533857));
#230915=CARTESIAN_POINT('Ctrl Pts',(-125.616106510535,1.55739090273089,
124.384970505708));
#230916=CARTESIAN_POINT('Ctrl Pts',(-125.894554134348,-4.55900688336737,
126.024246385717));
#230917=CARTESIAN_POINT('Ctrl Pts',(-126.173001758161,-6.48590006351826,
132.056213723232));
#230918=CARTESIAN_POINT('Ctrl Pts',(-126.451449381974,-2.45256793912933,
136.937789213063));
#230919=CARTESIAN_POINT('Ctrl Pts',(-126.729897005787,3.83455430671493,
136.183043458277));
#230920=CARTESIAN_POINT('Ctrl Pts',(-127.0083446296,6.5979084730801,130.485550936142));
#230921=CARTESIAN_POINT('Ctrl Pts',(-127.286792253413,3.29810707843306,
125.081028936517));
#230922=CARTESIAN_POINT('Ctrl Pts',(-127.565239877225,-3.03249359980603,
124.935969151478));
#230923=CARTESIAN_POINT('Ctrl Pts',(-127.843687501038,-6.57638080537151,
130.183674436914));
#230924=CARTESIAN_POINT('Ctrl Pts',(-128.122135124851,-4.07689532486387,
136.001760000162));
#230925=CARTESIAN_POINT('Ctrl Pts',(-128.400582748664,2.1690577917847,137.043689437881));
#230926=CARTESIAN_POINT('Ctrl Pts',(-128.679030372477,6.42175276214748,
132.351980497887));
#230927=CARTESIAN_POINT('Ctrl Pts',(-128.95747799629,4.77317066415926,126.238084493312));
#230928=CARTESIAN_POINT('Ctrl Pts',(-129.235925620103,-1.26172209184052,
124.320373171937));
#230929=CARTESIAN_POINT('Ctrl Pts',(-129.514373243916,-6.13715388399014,
128.361129552696));
#230930=CARTESIAN_POINT('Ctrl Pts',(-129.792820867728,-5.37284107338758,
134.647095923599));
#230931=CARTESIAN_POINT('Ctrl Pts',(-130.071268491542,0.328850205779251,
137.401776276312));
#230932=CARTESIAN_POINT('Ctrl Pts',(-130.349716115354,5.72834421106097,
134.093753940311));
#230933=CARTESIAN_POINT('Ctrl Pts',(-130.628163739167,5.86376973154965,
127.762939836503));
#230934=CARTESIAN_POINT('Ctrl Pts',(-130.90661136298,0.610677329821333,
124.227042848828));
#230935=CARTESIAN_POINT('Ctrl Pts',(-131.185058986793,-5.20359770476699,
126.735379570785));
#230936=CARTESIAN_POINT('Ctrl Pts',(-131.463506610606,-6.23602065855449,
132.982911093959));
#230937=CARTESIAN_POINT('Ctrl Pts',(-131.741954234419,-1.53784527367628,
137.228461157434));
#230938=CARTESIAN_POINT('Ctrl Pts',(-132.020401858232,4.57353478979242,
135.57057665953));
#230939=CARTESIAN_POINT('Ctrl Pts',(-132.298849482045,6.48205981103755,
129.532772461657));
#230940=CARTESIAN_POINT('Ctrl Pts',(-132.577297105858,2.43388853216508,
124.66349565853));
#230941=CARTESIAN_POINT('Ctrl Pts',(-132.85574472967,-3.85090740570176,
125.437373754826));
#230942=CARTESIAN_POINT('Ctrl Pts',(-133.134192353483,-6.59690756501448,
131.143250586095));
#230943=CARTESIAN_POINT('Ctrl Pts',(-133.412639977296,-3.28067194892964,
136.53770409198));
#230944=CARTESIAN_POINT('Ctrl Pts',(-133.691087601109,3.0503409184865,136.663495034279));
#230945=CARTESIAN_POINT('Ctrl Pts',(-133.969535224922,6.5782394992522,131.405027682246));
#230946=CARTESIAN_POINT('Ctrl Pts',(-134.247982848735,4.06105734507014,
125.59457664199));
#230947=CARTESIAN_POINT('Ctrl Pts',(-134.526430472548,-2.18803811555026,
124.57166256319));
#230948=CARTESIAN_POINT('Ctrl Pts',(-134.804878096361,-6.42643343958478,
129.276293512134));
#230949=CARTESIAN_POINT('Ctrl Pts',(-135.083325720174,-4.75925038136761,
135.385143480741));
#230950=CARTESIAN_POINT('Ctrl Pts',(-135.361773343986,1.28145127501926,
137.284477781773));
#230951=CARTESIAN_POINT('Ctrl Pts',(-135.640220967799,6.14456181203885,
133.228900980221));
#230952=CARTESIAN_POINT('Ctrl Pts',(-135.918668591612,5.36112022232688,
126.945290030769));
#230953=CARTESIAN_POINT('Ctrl Pts',(-136.197116215425,-0.348928946420584,
124.207976424505));
#230954=CARTESIAN_POINT('Ctrl Pts',(-136.475563839238,-5.73832945953392,
127.53241764038));
#230955=CARTESIAN_POINT('Ctrl Pts',(-136.754011463051,-5.85448553231475,
133.863614608987));
#230956=CARTESIAN_POINT('Ctrl Pts',(-137.032459086864,-0.590655408416443,
137.383506612345));
#230957=CARTESIAN_POINT('Ctrl Pts',(-137.310906710677,5.21595818069537,
134.857484855651));
#230958=CARTESIAN_POINT('Ctrl Pts',(-137.58935433449,6.22936101547165,128.606839930282));
#230959=CARTESIAN_POINT('Ctrl Pts',(-137.867801958302,1.51828539823306,
124.375609161675));
#230960=CARTESIAN_POINT('Ctrl Pts',(-138.146249582115,-4.58802032761614,
126.052086919061));
#230961=CARTESIAN_POINT('Ctrl Pts',(-138.424697205928,-6.47815950964009,
132.095672043897));
#230962=CARTESIAN_POINT('Ctrl Pts',(-138.703144829741,-2.41518657799051,
136.952605052004));
#230963=CARTESIAN_POINT('Ctrl Pts',(-138.981592453554,3.86722483040823,
136.159601783301));
#230964=CARTESIAN_POINT('Ctrl Pts',(-139.260040077367,6.59584554409815,
130.445393501362));
#230965=CARTESIAN_POINT('Ctrl Pts',(-139.53848770118,3.26320642772972,125.061058462695));
#230966=CARTESIAN_POINT('Ctrl Pts',(-139.816935324993,-3.06815997922566,
124.954537528447));
#230967=CARTESIAN_POINT('Ctrl Pts',(-140.095382948806,-6.58003725322031,
130.223718233352));
#230968=CARTESIAN_POINT('Ctrl Pts',(-140.373830572619,-4.04518174419624,
136.026480923393));
#230969=CARTESIAN_POINT('Ctrl Pts',(-140.652278196431,2.20699816962987,
137.030370167137));
#230970=CARTESIAN_POINT('Ctrl Pts',(-140.930725820244,6.43105458342049,
132.312860792301));
#230971=CARTESIAN_POINT('Ctrl Pts',(-141.209173444057,4.74528600953044,
126.209113451214));
#230972=CARTESIAN_POINT('Ctrl Pts',(-141.48762106787,-1.30116858700904,
124.328173765698));
#230973=CARTESIAN_POINT('Ctrl Pts',(-141.766068691683,-6.15191281770628,
128.398533417733));
#230974=CARTESIAN_POINT('Ctrl Pts',(-142.044516315496,-5.34934970658085,
134.679730735221));
#230975=CARTESIAN_POINT('Ctrl Pts',(-142.322963939309,0.369004454631186,
137.399652236939));
#230976=CARTESIAN_POINT('Ctrl Pts',(-142.601411563122,5.74826154890666,
134.058822938361));
#230977=CARTESIAN_POINT('Ctrl Pts',(-142.879859186934,5.84514709792562,
127.727301756295));
#230978=CARTESIAN_POINT('Ctrl Pts',(-143.158306810748,0.570628015260733,
124.223447345055));
#230979=CARTESIAN_POINT('Ctrl Pts',(-143.43675443456,-5.22827033670001,
126.767130735766));
#230980=CARTESIAN_POINT('Ctrl Pts',(-143.715202058373,-6.22264366443886,
133.020831158207));
#230981=CARTESIAN_POINT('Ctrl Pts',(-143.993649682186,-1.49871145760156,
137.237703434405));
#230982=CARTESIAN_POINT('Ctrl Pts',(-144.272097305999,4.60246336264661,
135.542647948195));
#230983=CARTESIAN_POINT('Ctrl Pts',(-144.550544929812,6.47419919545755,
129.493337883343));
#230984=CARTESIAN_POINT('Ctrl Pts',(-144.828992553625,2.39646224985712,
124.648793664219));
#230985=CARTESIAN_POINT('Ctrl Pts',(-145.107440177438,-3.8835064296727,
125.460914759058));
#230986=CARTESIAN_POINT('Ctrl Pts',(-145.38588780125,-6.59472242016944,
131.183401556022));
#230987=CARTESIAN_POINT('Ctrl Pts',(-145.664335425064,-3.24571067663155,
136.557568247724));
#230988=CARTESIAN_POINT('Ctrl Pts',(-145.942783048876,3.08595061694992,
136.644818187128));
#230989=CARTESIAN_POINT('Ctrl Pts',(-146.221230672689,6.58177405062243,
131.364972942318));
#230990=CARTESIAN_POINT('Ctrl Pts',(-146.499678296502,4.02926866931097,
125.569952358496));
#230991=CARTESIAN_POINT('Ctrl Pts',(-146.778125920315,-2.22593777837984,
124.585097249699));
#230992=CARTESIAN_POINT('Ctrl Pts',(-147.056573544128,-6.43561615084533,
129.315441348065));
#230993=CARTESIAN_POINT('Ctrl Pts',(-147.335021167941,-4.73127767801157,
135.414029517352));
#230994=CARTESIAN_POINT('Ctrl Pts',(-147.613468791753,1.32087384515067,
137.276557162581));
#230995=CARTESIAN_POINT('Ctrl Pts',(-147.891916415567,6.15920683289404,
133.191452367319));
#230996=CARTESIAN_POINT('Ctrl Pts',(-148.170364039379,5.33752963518947,
126.91272686995));
#230997=CARTESIAN_POINT('Ctrl Pts',(-148.448811663193,-0.389076544435395,
124.210222669761));
#230998=CARTESIAN_POINT('Ctrl Pts',(-148.727259287005,-5.75814038716998,
127.567409102056));
#230999=CARTESIAN_POINT('Ctrl Pts',(-149.005706910818,-5.83575451489182,
133.899195843233));
#231000=CARTESIAN_POINT('Ctrl Pts',(-149.284154534631,-0.550595335885521,
137.386980203127));
#231001=CARTESIAN_POINT('Ctrl Pts',(-149.562602158444,5.24053405872261,
134.825658742734));
#231002=CARTESIAN_POINT('Ctrl Pts',(-149.841049782257,6.21586866768539,
128.568960756646));
#231003=CARTESIAN_POINT('Ctrl Pts',(-150.119497406069,1.47912363311174,
124.366486037389));
#231004=CARTESIAN_POINT('Ctrl Pts',(-150.397945029883,-4.61686376108527,
126.080103549656));
#231005=CARTESIAN_POINT('Ctrl Pts',(-150.676392653695,-6.4701789051783,
132.135082514543));
#231006=CARTESIAN_POINT('Ctrl Pts',(-150.954840277509,-2.37771572122463,
136.967193065487));
#231007=CARTESIAN_POINT('Ctrl Pts',(-151.233287901321,3.89975205266408,
136.135961667893));
#231008=CARTESIAN_POINT('Ctrl Pts',(-151.511735525134,6.59353820363339,
130.405249368239));
#231009=CARTESIAN_POINT('Ctrl Pts',(-151.790183148947,3.22818485771248,
125.041300809049));
#231010=CARTESIAN_POINT('Ctrl Pts',(-152.06863077276,-3.10371266684865,
124.97332267276));
#231011=CARTESIAN_POINT('Ctrl Pts',(-152.347078396573,-6.58344987536885,
130.263783545709));
#231012=CARTESIAN_POINT('Ctrl Pts',(-152.625526020386,-4.01331826783166,
136.051008339035));
#231013=CARTESIAN_POINT('Ctrl Pts',(-152.903973644199,2.24485676634579,
137.016820189321));
#231014=CARTESIAN_POINT('Ctrl Pts',(-153.182421268012,6.44011809960154,
132.273685188686));
#231015=CARTESIAN_POINT('Ctrl Pts',(-153.460868891824,4.71722551658265,
126.180312687687));
#231016=CARTESIAN_POINT('Ctrl Pts',(-153.739316515637,-1.34056686689732,
124.336214336947));
#231017=CARTESIAN_POINT('Ctrl Pts',(-154.01776413945,-6.16644379003131,
128.436026431582));
#231018=CARTESIAN_POINT('Ctrl Pts',(-154.296211763263,-5.32566011765276,
134.712221943579));
#231019=CARTESIAN_POINT('Ctrl Pts',(-154.574659387076,0.409145029887599,
137.397283806609));
#231020=CARTESIAN_POINT('Ctrl Pts',(-154.853107010889,5.7679658828075,134.023771341112));
#231021=CARTESIAN_POINT('Ctrl Pts',(-155.131554634702,5.82630787022557,
127.691777697632));
#231022=CARTESIAN_POINT('Ctrl Pts',(-155.410002258515,0.530557555869813,
124.220095699443));
#231023=CARTESIAN_POINT('Ctrl Pts',(-155.688449882327,-5.25274923315307,
126.799031501784));
#231024=CARTESIAN_POINT('Ctrl Pts',(-155.96689750614,-6.20903608797397,
133.058669090323));
#231025=CARTESIAN_POINT('Ctrl Pts',(-156.245345129953,-1.4595221062231,
137.246707321489));
#231026=CARTESIAN_POINT('Ctrl Pts',(-156.523792753766,4.63122138952822,
135.514543657883));
#231027=CARTESIAN_POINT('Ctrl Pts',(-156.802240377579,6.46609867604585,
129.453951885458));
#231028=CARTESIAN_POINT('Ctrl Pts',(-157.080688001392,2.35894716575843,
124.634319766706));
#231029=CARTESIAN_POINT('Ctrl Pts',(-157.359135625205,-3.9159615488849,
125.484653766641));
#231030=CARTESIAN_POINT('Ctrl Pts',(-157.637583249018,-6.59229290546042,
131.223538480449));
#231031=CARTESIAN_POINT('Ctrl Pts',(-157.916030872831,-3.21062913332988,
136.577219216243));
#231032=CARTESIAN_POINT('Ctrl Pts',(-158.194478496644,3.12144596437753,
136.625924919674));
#231033=CARTESIAN_POINT('Ctrl Pts',(-158.472926120456,6.58506471193526,
131.324897428694));
#231034=CARTESIAN_POINT('Ctrl Pts',(-158.751373744269,3.99733068751967,
125.545522037924));
#231035=CARTESIAN_POINT('Ctrl Pts',(-159.029821368082,-2.26375495826568,
124.598762393297));
#231036=CARTESIAN_POINT('Ctrl Pts',(-159.308268991895,-6.44456038798308,
129.354644356446));
#231037=CARTESIAN_POINT('Ctrl Pts',(-159.586716615708,-4.7031296554214,
135.442744740987));
#231038=CARTESIAN_POINT('Ctrl Pts',(-159.865164239521,1.36024746981527,
137.268396713766));
#231039=CARTESIAN_POINT('Ctrl Pts',(-160.143611863334,6.17362362207528,
133.153915299856));
#231040=CARTESIAN_POINT('Ctrl Pts',(-160.422059487147,5.31374126392856,
126.880307915048));
#231041=CARTESIAN_POINT('Ctrl Pts',(-160.70050711096,-0.429209725076344,
124.212713263223));
#231042=CARTESIAN_POINT('Ctrl Pts',(-160.978954734773,-5.77773794479658,
127.602520510164));
#231043=CARTESIAN_POINT('Ctrl Pts',(-161.257402358585,-5.81680725143943,
133.934662397221));
#231044=CARTESIAN_POINT('Ctrl Pts',(-161.535849982398,-0.51051486084124,
137.390209872519));
#231045=CARTESIAN_POINT('Ctrl Pts',(-161.814297606211,5.26491574683228,
134.793683619137));
#231046=CARTESIAN_POINT('Ctrl Pts',(-162.092745230024,6.20214598860049,
128.531164416574));
#231047=CARTESIAN_POINT('Ctrl Pts',(-162.371192853837,1.43990705852047,
124.357601470914));
#231048=CARTESIAN_POINT('Ctrl Pts',(-162.64964047765,-4.64553611496906,
126.108295239334));
#231049=CARTESIAN_POINT('Ctrl Pts',(-162.928088101462,-6.46195854585841,
132.1744436748));
#231050=CARTESIAN_POINT('Ctrl Pts',(-163.206535725276,-2.34015675732853,
136.981552712947));
#231051=CARTESIAN_POINT('Ctrl Pts',(-163.484983349088,3.93213476817268,
136.112123988049));
#231052=CARTESIAN_POINT('Ctrl Pts',(-163.763430972902,6.5909865371863,130.365120024332));
#231053=CARTESIAN_POINT('Ctrl Pts',(-164.041878596714,3.19304366611785,
125.021756707701));
#231054=CARTESIAN_POINT('Ctrl Pts',(-164.320326220527,-3.13915034525769,
124.99232388833));
#231055=CARTESIAN_POINT('Ctrl Pts',(-164.59877384434,-6.58661854536123,
130.303868889347));
#231056=CARTESIAN_POINT('Ctrl Pts',(-164.877221468153,-3.98130607648258,
136.075341338217));
#231057=CARTESIAN_POINT('Ctrl Pts',(-165.155669091966,2.28263217906914,
137.003040006531));
#231058=CARTESIAN_POINT('Ctrl Pts',(-165.434116715779,6.44894297483741,
132.23445513871));
#231059=CARTESIAN_POINT('Ctrl Pts',(-165.712564339591,4.6889902251094,126.151683269957));
#231060=CARTESIAN_POINT('Ctrl Pts',(-165.991011963405,-1.37991547158711,
124.344494587733));
#231061=CARTESIAN_POINT('Ctrl Pts',(-166.269459587217,-6.18074626251326,
128.473607204924));
#231062=CARTESIAN_POINT('Ctrl Pts',(-166.54790721103,-5.3017731844313,134.744568344699));
#231063=CARTESIAN_POINT('Ctrl Pts',(-166.826354834843,0.449270444124704,
137.394671073086));
#231064=CARTESIAN_POINT('Ctrl Pts',(-167.104802458656,5.78745648261092,
133.988600447415));
#231065=CARTESIAN_POINT('Ctrl Pts',(-167.383250082469,5.8072527465451,127.656368976875));
#231066=CARTESIAN_POINT('Ctrl Pts',(-167.661697706282,0.490467436472931,
124.216988036188));
#231067=CARTESIAN_POINT('Ctrl Pts',(-167.940145330095,-5.27703348705155,
126.831080686747));
#231068=CARTESIAN_POINT('Ctrl Pts',(-168.218592953908,-6.19519843339338,
133.096423488211));
#231069=CARTESIAN_POINT('Ctrl Pts',(-168.49704057772,-1.42027867171577,
137.255472485049));
#231070=CARTESIAN_POINT('Ctrl Pts',(-168.775488201534,4.65980780479824,
135.486264830004));
#231071=CARTESIAN_POINT('Ctrl Pts',(-169.053935825346,6.45775855296945,
129.414615927465));
#231072=CARTESIAN_POINT('Ctrl Pts',(-169.332383449159,2.32134467000579,
124.620074502325));
#231073=CARTESIAN_POINT('Ctrl Pts',(-169.610831072972,-3.94827156070164,
125.508589897919));
#231074=CARTESIAN_POINT('Ctrl Pts',(-169.889278696785,-6.58961911091297,
131.263659872085));
#231075=CARTESIAN_POINT('Ctrl Pts',(-170.167726320598,-3.17542861898582,
136.596656269364));
#231076=CARTESIAN_POINT('Ctrl Pts',(-170.446173944411,3.15682564547787,
136.606815932013));
#231077=CARTESIAN_POINT('Ctrl Pts',(-170.724621568223,6.58811136125304,
131.284802626386));
#231078=CARTESIAN_POINT('Ctrl Pts',(-171.003069192037,3.96524458316956,
125.521286585549));
#231079=CARTESIAN_POINT('Ctrl Pts',(-171.28151681585,-2.30148825387982,
124.612657487621));
#231080=CARTESIAN_POINT('Ctrl Pts',(-171.559964439662,-6.45326581956532,
129.393901084596));
#231081=CARTESIAN_POINT('Ctrl Pts',(-171.838412063475,-4.67480735663214,
135.471288087592));
#231082=CARTESIAN_POINT('Ctrl Pts',(-172.116859687288,1.39957069001038,
137.259996737715));
#231083=CARTESIAN_POINT('Ctrl Pts',(-172.395307311101,6.18781164536257,
133.116291168777));
#231084=CARTESIAN_POINT('Ctrl Pts',(-172.673754934914,5.289755990031,126.848034367363));
#231085=CARTESIAN_POINT('Ctrl Pts',(-172.952202558727,-0.469327001192524,
124.215448112602));
#231086=CARTESIAN_POINT('Ctrl Pts',(-173.23065018254,-5.79712140621875,
127.637750563632));
#231087=CARTESIAN_POINT('Ctrl Pts',(-173.509097806352,-5.79764444405506,
133.970012956726));
#231088=CARTESIAN_POINT('Ctrl Pts',(-173.787545430165,-0.470415468481743,
137.393195500846));
#231089=CARTESIAN_POINT('Ctrl Pts',(-174.065993053978,5.28910234155359,
134.76156066971));
#231090=CARTESIAN_POINT('Ctrl Pts',(-174.344440677791,6.18819348671444,
128.493452310623));
#231091=CARTESIAN_POINT('Ctrl Pts',(-174.622888301604,1.40063712764339,
124.34895579147));
#231092=CARTESIAN_POINT('Ctrl Pts',(-174.901335925417,-4.67403632680454,
126.13666094344));
#231093=CARTESIAN_POINT('Ctrl Pts',(-175.17978354923,-6.45349873628761,
132.213754066126));
#231094=CARTESIAN_POINT('Ctrl Pts',(-175.458231173043,-2.30251107806296,
136.995683462282));
#231095=CARTESIAN_POINT('Ctrl Pts',(-175.736678796856,3.96437177698222,
136.088089627079));
#231096=CARTESIAN_POINT('Ctrl Pts',(-176.015126420669,6.58819063930867,
130.325006956645));
#231097=CARTESIAN_POINT('Ctrl Pts',(-176.293574044481,3.15778415511627,
125.002426882869));
#231098=CARTESIAN_POINT('Ctrl Pts',(-176.572021668294,-3.17447170129595,
125.011540471058));
#231099=CARTESIAN_POINT('Ctrl Pts',(-176.850469292107,-6.58954314578118,
130.343972778891));
#231100=CARTESIAN_POINT('Ctrl Pts',(-177.12891691592,-3.94914635637289,
136.099479019269));
#231101=CARTESIAN_POINT('Ctrl Pts',(-177.407364539733,2.32032300801719,
136.989030129397));
#231102=CARTESIAN_POINT('Ctrl Pts',(-177.685812163546,6.45752888212044,
132.195172096054));
#231103=CARTESIAN_POINT('Ctrl Pts',(-177.964259787359,4.66058118137817,
126.123226258898));
#231104=CARTESIAN_POINT('Ctrl Pts',(-178.242707411172,-1.41921294300185,
124.353014211231));
#231105=CARTESIAN_POINT('Ctrl Pts',(-178.521155034985,-6.19481970517025,
128.511274345191));
#231106=CARTESIAN_POINT('Ctrl Pts',(-178.799602658797,-5.27768979205393,
134.776768739972));
#231107=CARTESIAN_POINT('Ctrl Pts',(-179.078050282611,0.489379210479558,
137.391814133187));
#231108=CARTESIAN_POINT('Ctrl Pts',(-179.356497906423,5.80673262608622,
133.95331156054));
#231109=CARTESIAN_POINT('Ctrl Pts',(-179.634945530236,5.7879824329786,127.621076906106));
#231110=CARTESIAN_POINT('Ctrl Pts',(-179.913393154049,0.450359142625426,
124.214124470449));
#231111=CARTESIAN_POINT('Ctrl Pts',(-180.191840777862,-5.30112219853358,
126.863277103057));
#231112=CARTESIAN_POINT('Ctrl Pts',(-180.470288401675,-6.18113121345664,
133.134092952866));
#231113=CARTESIAN_POINT('Ctrl Pts',(-180.748736025488,-1.38098260826046,
137.263998600285));
#231114=CARTESIAN_POINT('Ctrl Pts',(-181.0271836493,4.68822154917632,135.457812512445));
#231115=CARTESIAN_POINT('Ctrl Pts',(-181.305631273113,6.44917913527537,
129.375331466973));
#231116=CARTESIAN_POINT('Ctrl Pts',(-181.584078896926,2.28365615597197,
124.606058398942));
#231117=CARTESIAN_POINT('Ctrl Pts',(-181.862526520739,-3.98043526786393,
125.532722265928));
#231118=CARTESIAN_POINT('Ctrl Pts',(-182.140974144552,-6.58670113560653,
131.303764244219));
#231119=CARTESIAN_POINT('Ctrl Pts',(-182.419421768365,-3.14011043796568,
136.615878686839));
#231120=CARTESIAN_POINT('Ctrl Pts',(-182.697869392178,3.19208834924215,
136.587491932238));
#231121=CARTESIAN_POINT('Ctrl Pts',(-182.976317015991,6.59091388568205,
131.244690021124));
#231122=CARTESIAN_POINT('Ctrl Pts',(-183.254764639804,3.93301154522339,
125.497246899427));
#231123=CARTESIAN_POINT('Ctrl Pts',(-183.533212263617,-2.33913626699958,
124.626782017781));
#231124=CARTESIAN_POINT('Ctrl Pts',(-183.811659887429,-6.46173212300977,
129.433210077844));
#231125=CARTESIAN_POINT('Ctrl Pts',(-184.090107511242,-4.64631183113728,
135.499658499484));
#231126=CARTESIAN_POINT('Ctrl Pts',(-184.368555135055,1.43884204859816,
137.251357545694));
#231127=CARTESIAN_POINT('Ctrl Pts',(-184.647002758868,6.20177037701405,
133.078581368264));
#231128=CARTESIAN_POINT('Ctrl Pts',(-184.925450382681,5.26557470227994,
126.815907422802));
#231129=CARTESIAN_POINT('Ctrl Pts',(-185.203898006494,-0.50942688622466,
124.218427116558));
#231130=CARTESIAN_POINT('Ctrl Pts',(-185.482345630307,-5.81629005317544,
127.673097957001));
#231131=CARTESIAN_POINT('Ctrl Pts',(-185.76079325412,-5.77826680282389,
134.005246211819));
#231132=CARTESIAN_POINT('Ctrl Pts',(-186.039240877932,-0.430298644703365,
137.395936977472));
#231133=CARTESIAN_POINT('Ctrl Pts',(-186.317688501746,5.31309294664177,
134.729291084778));
#231134=CARTESIAN_POINT('Ctrl Pts',(-186.596136125558,6.17401167904375,
128.455825836229));
#231135=CARTESIAN_POINT('Ctrl Pts',(-186.874583749371,1.36131529564269,
124.340549319425));
#231136=CARTESIAN_POINT('Ctrl Pts',(-187.153031373184,-4.70236334050424,
126.165199610876));
#231137=CARTESIAN_POINT('Ctrl Pts',(-187.431478996997,-6.44479978994851,
132.253012231859));
#231138=CARTESIAN_POINT('Ctrl Pts',(-187.70992662081,-2.26478007840253,
137.009584789872));
#231139=CARTESIAN_POINT('Ctrl Pts',(-187.988374244623,3.99646188453734,
136.063859475589));
#231140=CARTESIAN_POINT('Ctrl Pts',(-188.266821868436,6.58515061360439,
130.284911651585));
#231141=CARTESIAN_POINT('Ctrl Pts',(-188.545269492249,3.12240763126122,
124.983312050825));
#231142=CARTESIAN_POINT('Ctrl Pts',(-188.823717116061,-3.20967542611822,
125.030971708867));
#231143=CARTESIAN_POINT('Ctrl Pts',(-189.102164739874,-6.59222356825658,
130.384093728275));
#231144=CARTESIAN_POINT('Ctrl Pts',(-189.380612363687,-3.91684029919248,
136.123420487763));
#231145=CARTESIAN_POINT('Ctrl Pts',(-189.6590599875,2.35792785654334,136.974791077059));
#231146=CARTESIAN_POINT('Ctrl Pts',(-189.937507611313,6.46587550329532,
132.155837516369));
#231147=CARTESIAN_POINT('Ctrl Pts',(-190.215955235126,4.63199943809816,
126.094942708994));
#231148=CARTESIAN_POINT('Ctrl Pts',(-190.494402858939,-1.45845782495887,
124.361772891742));
#231149=CARTESIAN_POINT('Ctrl Pts',(-190.772850482752,-6.2086635965042,
128.549026456613));
#231150=CARTESIAN_POINT('Ctrl Pts',(-191.051298106565,-5.25341083294129,
134.808821936201));
#231151=CARTESIAN_POINT('Ctrl Pts',(-191.329745730377,0.529469842708527,
137.388713092773));
#231152=CARTESIAN_POINT('Ctrl Pts',(-191.60819335419,5.82579359894846,133.91790598813));
#231153=CARTESIAN_POINT('Ctrl Pts',(-191.886640978003,5.76849764359442,
127.585902793086));
#231154=CARTESIAN_POINT('Ctrl Pts',(-192.165088601816,0.410234160553658,
124.211505108333));
#231155=CARTESIAN_POINT('Ctrl Pts',(-192.443536225629,-5.32501447498302,
126.895619557667));
#231156=CARTESIAN_POINT('Ctrl Pts',(-192.721983849442,-6.16683494942961,
133.171676088433));
#231157=CARTESIAN_POINT('Ctrl Pts',(-193.000431473255,-1.34163537198624,
137.272285351261));
#231158=CARTESIAN_POINT('Ctrl Pts',(-193.278879097068,4.71646156978089,
135.429187759513));
#231159=CARTESIAN_POINT('Ctrl Pts',(-193.557326720881,6.44036074087642,
129.336099959682));
#231160=CARTESIAN_POINT('Ctrl Pts',(-193.835774344694,2.24588302022023,
124.592271975924));
#231161=CARTESIAN_POINT('Ctrl Pts',(-194.114221968506,-4.01245147853337,
125.557049976435));
#231162=CARTESIAN_POINT('Ctrl Pts',(-194.392669592319,-6.58353908766677,
131.343850110767));
#231163=CARTESIAN_POINT('Ctrl Pts',(-194.671117216133,-3.10467589899933,
136.634885756375));
#231164=CARTESIAN_POINT('Ctrl Pts',(-194.949564839945,3.22723276899961,
136.567953636405));
#231165=CARTESIAN_POINT('Ctrl Pts',(-195.228012463758,6.59347218137276,
131.204561099293));
#231166=CARTESIAN_POINT('Ctrl Pts',(-195.506460087571,3.90063276808784,
125.473403870355));
#231167=CARTESIAN_POINT('Ctrl Pts',(-195.784907711384,-2.3766976025655,
124.641135460387));
#231168=CARTESIAN_POINT('Ctrl Pts',(-196.063355335197,-6.46995898459376,
129.472569879579));
#231169=CARTESIAN_POINT('Ctrl Pts',(-196.34180295901,-4.61764413484867,
135.527854925386));
#231170=CARTESIAN_POINT('Ctrl Pts',(-196.620250582823,1.47806009036541,
137.242479457832));
#231171=CARTESIAN_POINT('Ctrl Pts',(-196.898698206635,6.21549929978325,
133.040787295662));
#231172=CARTESIAN_POINT('Ctrl Pts',(-197.177145830448,5.24119829672186,
126.783928271841));
#231173=CARTESIAN_POINT('Ctrl Pts',(-197.455593454261,-0.5495078942556,
124.2216501647));
#231174=CARTESIAN_POINT('Ctrl Pts',(-197.734041078074,-5.83524317536515,
127.708561380459));
#231175=CARTESIAN_POINT('Ctrl Pts',(-198.012488701887,-5.75867504579123,
134.040360856918));
#231176=CARTESIAN_POINT('Ctrl Pts',(-198.2909363257,-0.390165876051177,
137.398434200813));
#231177=CARTESIAN_POINT('Ctrl Pts',(-198.569383949513,5.33688667311775,
134.696876060105));
#231178=CARTESIAN_POINT('Ctrl Pts',(-198.847831573325,6.15960109109908,
128.418286387655));
#231179=CARTESIAN_POINT('Ctrl Pts',(-199.126279197139,1.32194301960288,
124.332382366286));
#231180=CARTESIAN_POINT('Ctrl Pts',(-199.404726820951,-4.73051610640191,
126.193910184127));
#231181=CARTESIAN_POINT('Ctrl Pts',(-199.683174444764,-6.43586202918244,
132.292216717274));
#231182=CARTESIAN_POINT('Ctrl Pts',(-199.961622068577,-2.22696515648391,
137.023256180599));
#231183=CARTESIAN_POINT('Ctrl Pts',(-200.24006969239,4.02840390172748,136.039434431435));
#231184=CARTESIAN_POINT('Ctrl Pts',(-200.518517316203,6.58186657272242,
130.244835594899));
#231185=CARTESIAN_POINT('Ctrl Pts',(-200.796964940016,3.08691540544346,
124.964412919876));
#231186=CARTESIAN_POINT('Ctrl Pts',(-201.075412563829,-3.24476021523692,
125.050616881724));
#231187=CARTESIAN_POINT('Ctrl Pts',(-201.353860187642,-6.59465971346335,
130.424230250803));
#231188=CARTESIAN_POINT('Ctrl Pts',(-201.632307811455,-3.88438910205457,
136.147164856536));
#231189=CARTESIAN_POINT('Ctrl Pts',(-201.910755435267,2.39544533118521,
136.960323377152));
#231190=CARTESIAN_POINT('Ctrl Pts',(-202.18920305908,6.47398252907625,132.116452857208));
#231191=CARTESIAN_POINT('Ctrl Pts',(-202.467650682893,4.60324605437475,
126.066833668302));
#231192=CARTESIAN_POINT('Ctrl Pts',(-202.746098306706,-1.49764866322506,
124.370770304711));
#231193=CARTESIAN_POINT('Ctrl Pts',(-203.024545930519,-6.22227742352606,
128.586862140274));
#231194=CARTESIAN_POINT('Ctrl Pts',(-203.302993554332,-5.22893720675747,
134.840726745644));
#231195=CARTESIAN_POINT('Ctrl Pts',(-203.581441178145,0.569540855237039,
137.385368066758));
#231196=CARTESIAN_POINT('Ctrl Pts',(-203.859888801958,5.84463869488665,
133.882385042152));
#231197=CARTESIAN_POINT('Ctrl Pts',(-204.138336425771,5.7487991004088,127.550847941203));
#231198=CARTESIAN_POINT('Ctrl Pts',(-204.416784049583,0.370093977104817,
124.209130046901));
#231199=CARTESIAN_POINT('Ctrl Pts',(-204.695231673396,-5.34870943106288,
126.928106852114));
#231200=CARTESIAN_POINT('Ctrl Pts',(-204.973679297209,-6.15231017106575,
133.209171502253));
#231201=CARTESIAN_POINT('Ctrl Pts',(-205.252126921022,-1.30223842092043,
137.280332430907));
#231202=CARTESIAN_POINT('Ctrl Pts',(-205.530574544835,4.74452682016742,
135.400391631911));
#231203=CARTESIAN_POINT('Ctrl Pts',(-205.809022168648,6.43130369654214,
129.296922859329));
#231204=CARTESIAN_POINT('Ctrl Pts',(-206.087469792461,2.20802666244648,
124.578715744137));
#231205=CARTESIAN_POINT('Ctrl Pts',(-206.365917416273,-4.04431900633787,
125.581572127967));
#231206=CARTESIAN_POINT('Ctrl Pts',(-206.644365040087,-6.58013308426553,
131.383915986335));
#231207=CARTESIAN_POINT('Ctrl Pts',(-206.922812663899,-3.06912631512495,
136.653676773657));
#231208=CARTESIAN_POINT('Ctrl Pts',(-207.201260287713,3.26225760245914,
136.548201768512));
#231209=CARTESIAN_POINT('Ctrl Pts',(-207.479707911525,6.59578615352751,
131.164417347887));
#231210=CARTESIAN_POINT('Ctrl Pts',(-207.758155535338,3.86810945157081,
125.449758381845));
#231211=CARTESIAN_POINT('Ctrl Pts',(-208.036603159151,-2.41417086872696,
124.655717283569));
#231212=CARTESIAN_POINT('Ctrl Pts',(-208.315050782964,-6.47794609946865,
129.511979031309));
#231213=CARTESIAN_POINT('Ctrl Pts',(-208.593498406777,-4.58880533005852,
135.555876320469));
#231214=CARTESIAN_POINT('Ctrl Pts',(-208.87194603059,1.51722336207232,137.233362803106));
#231215=CARTESIAN_POINT('Ctrl Pts',(-209.150393654402,6.22899790494034,
133.00291035145));
#231216=CARTESIAN_POINT('Ctrl Pts',(-209.428841278216,5.21662767663345,
126.752098099478));
#231217=CARTESIAN_POINT('Ctrl Pts',(-209.707288902028,-0.589568540070009,
124.225117137599));
#231218=CARTESIAN_POINT('Ctrl Pts',(-209.985736525842,-5.85398007047323,
127.744139519898));
#231219=CARTESIAN_POINT('Ctrl Pts',(-210.264184149654,-5.73886989893714,
134.07535559084));
#231220=CARTESIAN_POINT('Ctrl Pts',(-210.542631773467,-0.350018649658268,
137.400687078332));
#231221=CARTESIAN_POINT('Ctrl Pts',(-210.82107939728,5.36048263929459,134.664316796842));
#231222=CARTESIAN_POINT('Ctrl Pts',(-211.099527021093,6.14496225687153,
128.38083535594));
#231223=CARTESIAN_POINT('Ctrl Pts',(-211.377974644906,1.28252175847855,
124.324455234681));
#231224=CARTESIAN_POINT('Ctrl Pts',(-211.656422268719,-4.75849358128477,
126.222791599316));
#231225=CARTESIAN_POINT('Ctrl Pts',(-211.934869892531,-6.4266857851828,
132.331366069634));
#231226=CARTESIAN_POINT('Ctrl Pts',(-212.213317516344,-2.18906771355195,
137.036697127864));
#231227=CARTESIAN_POINT('Ctrl Pts',(-212.491765140157,4.06019664492976,
136.014815399695));
#231228=CARTESIAN_POINT('Ctrl Pts',(-212.770212763971,6.57833863835413,
130.204780271616));
#231229=CARTESIAN_POINT('Ctrl Pts',(-213.048660387783,3.05130879283982,
124.945730190337));
#231230=CARTESIAN_POINT('Ctrl Pts',(-213.327108011596,-3.27972476857289,
125.070475261673));
#231231=CARTESIAN_POINT('Ctrl Pts',(-213.605555635409,-6.59685149112928,
130.464380859201));
#231232=CARTESIAN_POINT('Ctrl Pts',(-213.884003259222,-3.85179396744981,
136.170711245733));
#231233=CARTESIAN_POINT('Ctrl Pts',(-214.162450883035,2.43287404171984,
136.94562756578));
#231234=CARTESIAN_POINT('Ctrl Pts',(-214.440898506847,6.48184965905313,
132.077019577989));
#231235=CARTESIAN_POINT('Ctrl Pts',(-214.71934613066,4.57432209567675,126.038900178414));
#231236=CARTESIAN_POINT('Ctrl Pts',(-214.997793754473,-1.53678400556905,
124.380006116735));
#231237=CARTESIAN_POINT('Ctrl Pts',(-215.276241378286,-6.23566068176903,
128.624779994154));
#231238=CARTESIAN_POINT('Ctrl Pts',(-215.554689002099,-5.20426982038336,
134.872481986055));
#231239=CARTESIAN_POINT('Ctrl Pts',(-215.833136625912,0.609590763220439,
137.381779179092));
#231240=CARTESIAN_POINT('Ctrl Pts',(-216.111584249725,5.86326721558844,
133.846750038845));
#231241=CARTESIAN_POINT('Ctrl Pts',(-216.390031873537,5.72888753335829,
127.51591364943));
#231242=CARTESIAN_POINT('Ctrl Pts',(-216.668479497351,0.329940079686948,
124.206999374164));
#231243=CARTESIAN_POINT('Ctrl Pts',(-216.946927121163,-5.37220618874772,
126.960737782571));
#231244=CARTESIAN_POINT('Ctrl Pts',(-217.225374744977,-6.13755741658593,
133.246577804923));
#231245=CARTESIAN_POINT('Ctrl Pts',(-217.503822368789,-1.26279321493052,
137.288139541036));
#231246=CARTESIAN_POINT('Ctrl Pts',(-217.782269992602,4.77241626036792,
135.37142519669));
#231247=CARTESIAN_POINT('Ctrl Pts',(-218.060717616415,6.4220083378839,129.257801617636));
#231248=CARTESIAN_POINT('Ctrl Pts',(-218.339165240228,2.17008848543354,
124.565390205911));
#231249=CARTESIAN_POINT('Ctrl Pts',(-218.617612864041,-4.07603667041411,
125.606287811847));
#231250=CARTESIAN_POINT('Ctrl Pts',(-218.896060487854,-6.57648325161253,
131.423960386264));
#231251=CARTESIAN_POINT('Ctrl Pts',(-219.174508111666,-3.03346300364714,
136.672251042379));
#231252=CARTESIAN_POINT('Ctrl Pts',(-219.45295573548,3.29716155176439,136.528237060474));
#231253=CARTESIAN_POINT('Ctrl Pts',(-219.731403359293,6.59785571640026,
131.124260254445));
#231254=CARTESIAN_POINT('Ctrl Pts',(-220.009850983105,3.83544280083539,
125.426311310091));
#231255=CARTESIAN_POINT('Ctrl Pts',(-220.288298606918,-2.45155467689987,
124.67052694699));
#231256=CARTESIAN_POINT('Ctrl Pts',(-220.566746230731,-6.48569317166813,
129.551436072715));
#231257=CARTESIAN_POINT('Ctrl Pts',(-220.845193854544,-4.55979648539947,
135.58372164639));
#231258=CARTESIAN_POINT('Ctrl Pts',(-221.123641478357,1.55633041250914,
137.224007919343));
#231259=CARTESIAN_POINT('Ctrl Pts',(-221.40208910217,6.24226569228925,132.964951939167));
#231260=CARTESIAN_POINT('Ctrl Pts',(-221.680536725983,5.19186375248807,
126.720418085194));
#231261=CARTESIAN_POINT('Ctrl Pts',(-221.958984349796,-0.629607339204784,
124.228827906785));
#231262=CARTESIAN_POINT('Ctrl Pts',(-222.237431973609,-5.87250004419688,
127.779831056953));
#231263=CARTESIAN_POINT('Ctrl Pts',(-222.515879597421,-5.71885209614835,
134.110229116839));
#231264=CARTESIAN_POINT('Ctrl Pts',(-222.794327221234,-0.309858453196267,
137.402695526548));
#231265=CARTESIAN_POINT('Ctrl Pts',(-223.072774845047,5.38387997081673,
134.631614501482));
#231266=CARTESIAN_POINT('Ctrl Pts',(-223.35122246886,6.13009571880702,128.343474128844));
#231267=CARTESIAN_POINT('Ctrl Pts',(-223.629670092673,1.24305297303857,
124.316768218352));
#231268=CARTESIAN_POINT('Ctrl Pts',(-223.908117716486,-4.78629472843886,
126.25184278623));
#231269=CARTESIAN_POINT('Ctrl Pts',(-224.186565340298,-6.41727139797729,
132.370458838244));
#231270=CARTESIAN_POINT('Ctrl Pts',(-224.465012964112,-2.15108915391133,
137.049907133607));
#231271=CARTESIAN_POINT('Ctrl Pts',(-224.743460587925,4.09183893605206,
135.990003292637));
#231272=CARTESIAN_POINT('Ctrl Pts',(-225.021908211737,6.57456694122844,
130.164747166004));
#231273=CARTESIAN_POINT('Ctrl Pts',(-225.300355835551,3.01558911286705,
124.927264554503));
#231274=CARTESIAN_POINT('Ctrl Pts',(-225.578803459363,-3.31456779050113,
125.090546112851));
#231275=CARTESIAN_POINT('Ctrl Pts',(-225.857251083176,-6.5987988200372,
130.504544065675));
#231276=CARTESIAN_POINT('Ctrl Pts',(-226.135698706989,-3.8190561032033,
136.194058782834));
#231277=CARTESIAN_POINT('Ctrl Pts',(-226.414146330802,2.47021260121173,
136.930704187504));
#231278=CARTESIAN_POINT('Ctrl Pts',(-226.692593954615,6.48947660170784,
132.037539139922));
#231279=CARTESIAN_POINT('Ctrl Pts',(-226.971041578427,4.54522863379049,
126.011143274415));
#231280=CARTESIAN_POINT('Ctrl Pts',(-227.24948920224,-1.57586240181677,
124.389479985577));
#231281=CARTESIAN_POINT('Ctrl Pts',(-227.527936826054,-6.24881287531301,
128.662778613197));
#231282=CARTESIAN_POINT('Ctrl Pts',(-227.806384449866,-5.17940958787633,
134.904086480733));
#231283=CARTESIAN_POINT('Ctrl Pts',(-228.084832073679,0.649618082593193,
137.377946562762));
#231284=CARTESIAN_POINT('Ctrl Pts',(-228.363279697492,5.88167847076755,
133.811002298682));
#231285=CARTESIAN_POINT('Ctrl Pts',(-228.641727321305,5.70876368027354,
127.481101212267));
#231286=CARTESIAN_POINT('Ctrl Pts',(-228.920174945118,0.289773956218704,
124.205113169075));
#231287=CARTESIAN_POINT('Ctrl Pts',(-229.198622568931,-5.39550387735667,
126.993511139885));
#231288=CARTESIAN_POINT('Ctrl Pts',(-229.477070192744,-6.12257723265909,
133.283893610337));
#231289=CARTESIAN_POINT('Ctrl Pts',(-229.755517816557,-1.22330121567356,
137.295706392352));
#231290=CARTESIAN_POINT('Ctrl Pts',(-230.033965440369,4.80012885692891,
135.34228952721));
#231291=CARTESIAN_POINT('Ctrl Pts',(-230.312413064183,6.41247500934538,
129.218737684256));
#231292=CARTESIAN_POINT('Ctrl Pts',(-230.590860687995,2.13206989499296,
124.552295855027));
#231293=CARTESIAN_POINT('Ctrl Pts',(-230.869308311808,-4.10760329545278,
125.631196112227));
#231294=CARTESIAN_POINT('Ctrl Pts',(-231.147755935621,-6.5725897249546,
131.463981826697));
#231295=CARTESIAN_POINT('Ctrl Pts',(-231.426203559434,-2.99768728608136,
136.690607874263));
#231296=CARTESIAN_POINT('Ctrl Pts',(-231.704651183247,3.33194332353496,
136.508060252089));
#231297=CARTESIAN_POINT('Ctrl Pts',(-231.98309880706,6.59968079330357,131.084091307006));
#231298=CARTESIAN_POINT('Ctrl Pts',(-232.261546430872,3.80263402635669,
125.403063523931));
#231299=CARTESIAN_POINT('Ctrl Pts',(-232.539994054686,-2.48884764181187,
124.685563901874));
#231300=CARTESIAN_POINT('Ctrl Pts',(-232.818441678498,-6.49319991412244,
129.5909395417));
#231301=CARTESIAN_POINT('Ctrl Pts',(-233.096889302311,-4.53061867580467,
135.611389871331));
#231302=CARTESIAN_POINT('Ctrl Pts',(-233.375336926124,1.59537979255065,
137.214415153187));
#231303=CARTESIAN_POINT('Ctrl Pts',(-233.653784549937,6.25530217018742,
132.926913465378));
#231304=CARTESIAN_POINT('Ctrl Pts',(-233.93223217375,5.16690744192206,126.688889402902));
#231305=CARTESIAN_POINT('Ctrl Pts',(-234.210679797563,-0.669622808008655,
124.232782334755));
#231306=CARTESIAN_POINT('Ctrl Pts',(-234.489127421376,-5.89080241027189,
127.815634669064));
#231307=CARTESIAN_POINT('Ctrl Pts',(-234.767575045188,-5.69862237919218,
134.144980142666));
#231308=CARTESIAN_POINT('Ctrl Pts',(-235.046022669002,-0.269686774814632,
137.404459471037));
#231309=CARTESIAN_POINT('Ctrl Pts',(-235.324470292814,5.40707780068583,
134.598770385822));
#231310=CARTESIAN_POINT('Ctrl Pts',(-235.602917916627,6.11500202779203,
128.306204090801));
#231311=CARTESIAN_POINT('Ctrl Pts',(-235.88136554044,1.20353812581378,124.309321602146));
#231312=CARTESIAN_POINT('Ctrl Pts',(-236.159813164253,-4.81391851768082,
126.281062668365));
#231313=CARTESIAN_POINT('Ctrl Pts',(-236.438260788066,-6.40761921642086,
132.40949357451));
#231314=CARTESIAN_POINT('Ctrl Pts',(-236.716708411879,-2.11303088487057,
137.062885708328));
#231315=CARTESIAN_POINT('Ctrl Pts',(-236.995156035692,4.12332960257798,
135.964999029683));
#231316=CARTESIAN_POINT('Ctrl Pts',(-237.273603659505,6.57055162110693,
130.124737761504));
#231317=CARTESIAN_POINT('Ctrl Pts',(-237.552051283318,2.97975768913041,
124.909016696624));
#231318=CARTESIAN_POINT('Ctrl Pts',(-237.83049890713,-3.34928798990126,
125.110828691528));
#231319=CARTESIAN_POINT('Ctrl Pts',(-238.108946530943,-6.60050162802816,
130.544718381962));
#231320=CARTESIAN_POINT('Ctrl Pts',(-238.387394154756,-3.7861767224282,
136.217206602688));
#231321=CARTESIAN_POINT('Ctrl Pts',(-238.665841778569,2.5074596260677,136.915553795314));
#231322=CARTESIAN_POINT('Ctrl Pts',(-238.944289402382,6.49686307441993,
131.998013005973));
#231323=CARTESIAN_POINT('Ctrl Pts',(-239.222737026195,4.51596674678651,
125.983563984846));
#231324=CARTESIAN_POINT('Ctrl Pts',(-239.501184650008,-1.61488240390346,
124.399191560181));
#231325=CARTESIAN_POINT('Ctrl Pts',(-239.77963227382,-6.26173351679718,
128.700856589348));
#231326=CARTESIAN_POINT('Ctrl Pts',(-240.058079897633,-5.15435743044315,
134.935539058562));
#231327=CARTESIAN_POINT('Ctrl Pts',(-240.336527521446,0.689621330129741,
137.373870359787));
#231328=CARTESIAN_POINT('Ctrl Pts',(-240.614975145259,5.89987177818775,
133.775143146303));
#231329=CARTESIAN_POINT('Ctrl Pts',(-240.893422769072,5.68842828685113,
127.446411919705));
#231330=CARTESIAN_POINT('Ctrl Pts',(-241.171870392886,0.249597095069331,
124.203471501526));
#231331=CARTESIAN_POINT('Ctrl Pts',(-241.450318016698,-5.41860163358522,
127.026425709627));
#231332=CARTESIAN_POINT('Ctrl Pts',(-241.728765640511,-6.10737017438111,
133.321117535742));
#231333=CARTESIAN_POINT('Ctrl Pts',(-242.007213264324,-1.18376388654087,
137.303032704464));
#231334=CARTESIAN_POINT('Ctrl Pts',(-242.285660888137,4.82766358294966,
135.312985703106));
#231335=CARTESIAN_POINT('Ctrl Pts',(-242.56410851195,6.40270406418687,129.179732506718));
#231336=CARTESIAN_POINT('Ctrl Pts',(-242.842556135762,2.09397229991911,
124.539433176702));
#231337=CARTESIAN_POINT('Ctrl Pts',(-243.121003759575,-4.13901771174057,
125.65629610612));
#231338=CARTESIAN_POINT('Ctrl Pts',(-243.399451383388,-6.56845264856689,
131.503978824623));
#231339=CARTESIAN_POINT('Ctrl Pts',(-243.677899007202,-2.9618004881116,
136.70874658909));
#231340=CARTESIAN_POINT('Ctrl Pts',(-243.956346631013,3.36660162892119,
136.487672091016));
#231341=CARTESIAN_POINT('Ctrl Pts',(-244.234794254827,6.60126131660758,
131.043911994042));
#231342=CARTESIAN_POINT('Ctrl Pts',(-244.513241878639,3.76968434387551,
125.380015884821));
#231343=CARTESIAN_POINT('Ctrl Pts',(-244.791689502453,-2.52604838156001,
124.70082759102));
#231344=CARTESIAN_POINT('Ctrl Pts',(-245.070137126265,-6.50046604866569,
129.630487974449));
#231345=CARTESIAN_POINT('Ctrl Pts',(-245.348584750079,-4.50127298246883,
135.638879970036));
#231346=CARTESIAN_POINT('Ctrl Pts',(-245.627032373891,1.63437005520677,
137.204584860103));
#231347=CARTESIAN_POINT('Ctrl Pts',(-245.905479997704,6.26810685556324,
132.888796339615));
#231348=CARTESIAN_POINT('Ctrl Pts',(-246.183927621517,5.14175966970064,
126.65751322091));
#231349=CARTESIAN_POINT('Ctrl Pts',(-246.46237524533,-0.709613463692526,
124.236980274974));
#231350=CARTESIAN_POINT('Ctrl Pts',(-246.740822869143,-5.90888649049716,
127.851549029514));
#231351=CARTESIAN_POINT('Ctrl Pts',(-247.019270492956,-5.67818149768794,
134.179607380607));
#231352=CARTESIAN_POINT('Ctrl Pts',(-247.297718116769,-0.229505103091092,
137.405978846438));
#231353=CARTESIAN_POINT('Ctrl Pts',(-247.576165740581,5.43007526929941,
134.565785666913));
#231354=CARTESIAN_POINT('Ctrl Pts',(-247.854613364394,6.09968174312738,
128.269026622868));
#231355=CARTESIAN_POINT('Ctrl Pts',(-248.133060988207,1.16397868104094,
124.302115661998));
#231356=CARTESIAN_POINT('Ctrl Pts',(-248.41150861202,-4.84136392540264,
126.31045016297));
#231357=CARTESIAN_POINT('Ctrl Pts',(-248.689956235833,-6.39772959817725,
132.448468831983));
#231358=CARTESIAN_POINT('Ctrl Pts',(-248.968403859646,-2.07489431669385,
137.075632371099));
#231359=CARTESIAN_POINT('Ctrl Pts',(-249.246851483459,4.15466747760909,
135.939803537374));
#231360=CARTESIAN_POINT('Ctrl Pts',(-249.525299107272,6.56629282677857,
130.08475354068));
#231361=CARTESIAN_POINT('Ctrl Pts',(-249.803746731085,2.94381584937754,
124.890987292882));
#231362=CARTESIAN_POINT('Ctrl Pts',(-250.082194354898,-3.38388408020374,
125.131322246124));
#231363=CARTESIAN_POINT('Ctrl Pts',(-250.36064197871,-6.60195985200274,
130.584902319384));
#231364=CARTESIAN_POINT('Ctrl Pts',(-250.639089602524,-3.75315704348482,
136.240153847548));
#231365=CARTESIAN_POINT('Ctrl Pts',(-250.917537226336,2.54461373609029,
136.900176950603));
#231366=CARTESIAN_POINT('Ctrl Pts',(-251.19598485015,6.50400880347224,131.958442640812));
#231367=CARTESIAN_POINT('Ctrl Pts',(-251.474432473962,4.48653751899202,
125.956163331638));
#231368=CARTESIAN_POINT('Ctrl Pts',(-251.752880097775,-1.65384256596459,
124.409140480742));
#231369=CARTESIAN_POINT('Ctrl Pts',(-252.031327721588,-6.27442212737671,
128.739012511497));
#231370=CARTESIAN_POINT('Ctrl Pts',(-252.309775345401,-5.12911427652582,
134.966838554275));
#231371=CARTESIAN_POINT('Ctrl Pts',(-252.588222969213,0.729599023732927,
137.369550720794));
#231372=CARTESIAN_POINT('Ctrl Pts',(-252.866670593027,5.91784646323776,
133.739173911277));
#231373=CARTESIAN_POINT('Ctrl Pts',(-253.145118216839,5.66788210748017,
127.411847055674));
#231374=CARTESIAN_POINT('Ctrl Pts',(-253.423565840652,0.209410983396998,
124.20207443517));
#231375=CARTESIAN_POINT('Ctrl Pts',(-253.702013464465,-5.44149859849489,
127.059480266814));
#231376=CARTESIAN_POINT('Ctrl Pts',(-253.980461088278,-6.0919368110008,
133.358248211846));
#231377=CARTESIAN_POINT('Ctrl Pts',(-254.258908712091,-1.1441826817532,
137.310118186916));
#231378=CARTESIAN_POINT('Ctrl Pts',(-254.537356335904,4.85501939763767,
135.283514846073));
#231379=CARTESIAN_POINT('Ctrl Pts',(-254.815803959717,6.39269590315201,
129.140787462715));
#231380=CARTESIAN_POINT('Ctrl Pts',(-255.09425158353,2.05579703890082,124.526802775315));
#231381=CARTESIAN_POINT('Ctrl Pts',(-255.372699207342,-4.17027861730954,
125.681586622223));
#231382=CARTESIAN_POINT('Ctrl Pts',(-255.651146831155,-6.5640724361261,
131.5439503534));
#231383=CARTESIAN_POINT('Ctrl Pts',(-255.929594454968,-2.925803447894,136.726665654721));
#231384=CARTESIAN_POINT('Ctrl Pts',(-256.208042078781,3.40113425532747,
136.467074956607));
#231385=CARTESIAN_POINT('Ctrl Pts',(-256.486489702594,6.60259898059897,
131.003720738236));
#231386=CARTESIAN_POINT('Ctrl Pts',(-256.764937326407,3.73659166461274,
125.357175036369));
#231387=CARTESIAN_POINT('Ctrl Pts',(-257.04338495022,-2.56314926818932,
124.716306516944));
#231388=CARTESIAN_POINT('Ctrl Pts',(-257.321832574033,-6.5075031063131,
129.670100547101));
#231389=CARTESIAN_POINT('Ctrl Pts',(-257.600280197845,-4.47173821150659,
135.666151948257));
#231390=CARTESIAN_POINT('Ctrl Pts',(-257.878727821659,1.67325768403046,
137.194590998305));
#231391=CARTESIAN_POINT('Ctrl Pts',(-258.157175445471,6.28075871394982,
132.850463013089));
#231392=CARTESIAN_POINT('Ctrl Pts',(-258.435623069284,5.1162713672671,126.626553096149));
#231393=CARTESIAN_POINT('Ctrl Pts',(-258.714070693097,-0.749294580734974,
124.240926059104));
#231394=CARTESIAN_POINT('Ctrl Pts',(-258.99251831691,-5.92728653745133,
127.888508918958));
#231395=CARTESIAN_POINT('Ctrl Pts',(-259.270965940723,-5.656519339957,134.212338033208));
#231396=CARTESIAN_POINT('Ctrl Pts',(-259.549413564536,-0.191230405826049,
137.41063083554));
#231397=CARTESIAN_POINT('Ctrl Pts',(-259.827861188349,5.45654320709978,
134.526020746857));
#231398=CARTESIAN_POINT('Ctrl Pts',(-260.059900874859,5.97341346954355,
129.293215926205));
#231399=CARTESIAN_POINT('Ctrl Pts',(-260.245542550368,3.60742224527213,
126.247226657536));
#231400=CARTESIAN_POINT('Ctrl Pts',(-260.338368351272,1.86717727106152,
125.459413119698));
#231401=CARTESIAN_POINT('Ctrl Pts',(-260.384786214875,0.950008195528324,
125.301089073499));
#231402=CARTESIAN_POINT('Ctrl Pts',(209.997886486728,-2.58542267678463,
125.478296443779));
#231403=CARTESIAN_POINT('Ctrl Pts',(209.951476810375,-3.47289965896197,
125.909102290886));
#231404=CARTESIAN_POINT('Ctrl Pts',(209.85865919672,-5.01373755653622,127.222906143875));
#231405=CARTESIAN_POINT('Ctrl Pts',(209.67302570846,-6.52844908712303,131.020616473957));
#231406=CARTESIAN_POINT('Ctrl Pts',(209.440986021949,-4.4641631800594,136.198709217918));
#231407=CARTESIAN_POINT('Ctrl Pts',(209.162538398136,2.13623200523086,137.47712630299));
#231408=CARTESIAN_POINT('Ctrl Pts',(208.884090774324,6.76311047611758,132.61329501932));
#231409=CARTESIAN_POINT('Ctrl Pts',(208.60564315051,5.180460236421,126.09244423763));
#231410=CARTESIAN_POINT('Ctrl Pts',(208.327195526698,-1.16565068102074,
123.898824768668));
#231411=CARTESIAN_POINT('Ctrl Pts',(208.048747902884,-6.43906639651766,
128.052530506575));
#231412=CARTESIAN_POINT('Ctrl Pts',(207.770300279072,-5.79609906993421,
134.734252735451));
#231413=CARTESIAN_POINT('Ctrl Pts',(207.491852655259,0.173626147510206,
137.805009652024));
#231414=CARTESIAN_POINT('Ctrl Pts',(207.213405031446,5.98357180802623,134.442293088818));
#231415=CARTESIAN_POINT('Ctrl Pts',(206.934957407633,6.29502677410122,127.736610299611));
#231416=CARTESIAN_POINT('Ctrl Pts',(206.65650978382,0.821596385081328,123.849978754804));
#231417=CARTESIAN_POINT('Ctrl Pts',(206.378062160007,-5.40680743188727,
126.354116934927));
#231418=CARTESIAN_POINT('Ctrl Pts',(206.099614536195,-6.66663710465116,
132.947794423038));
#231419=CARTESIAN_POINT('Ctrl Pts',(205.821166912381,-1.80014356190772,
137.571770081489));
#231420=CARTESIAN_POINT('Ctrl Pts',(205.542719288569,4.72058899422897,135.976822216287));
#231421=CARTESIAN_POINT('Ctrl Pts',(205.264271664756,6.90333351468265,129.628637390042));
#231422=CARTESIAN_POINT('Ctrl Pts',(204.985824040943,2.74225038547515,124.360883417158));
#231423=CARTESIAN_POINT('Ctrl Pts',(204.70737641713,-3.93882614214087,125.014370927945));
#231424=CARTESIAN_POINT('Ctrl Pts',(204.428928793317,-7.00031425910704,
130.988575726592));
#231425=CARTESIAN_POINT('Ctrl Pts',(204.150481169504,-3.62885534891233,
136.793496040797));
#231426=CARTESIAN_POINT('Ctrl Pts',(203.872033545692,3.07734423765085,137.09469337995));
#231427=CARTESIAN_POINT('Ctrl Pts',(203.593585921878,6.95561486460971,131.615382266785));
#231428=CARTESIAN_POINT('Ctrl Pts',(203.315138298066,4.44201520086038,125.390781848689));
#231429=CARTESIAN_POINT('Ctrl Pts',(203.036690674253,-2.15357941165663,
124.140995867004));
#231430=CARTESIAN_POINT('Ctrl Pts',(202.75824305044,-6.77013976170558,129.014516559232));
#231431=CARTESIAN_POINT('Ctrl Pts',(202.479795426627,-5.16527240588502,
135.532816506767));
#231432=CARTESIAN_POINT('Ctrl Pts',(202.201347802814,1.18622795093483,137.705896487686));
#231433=CARTESIAN_POINT('Ctrl Pts',(201.922900179001,6.44764277258624,133.536802163981));
#231434=CARTESIAN_POINT('Ctrl Pts',(201.644452555188,5.78398887041165,126.856727545651));
#231435=CARTESIAN_POINT('Ctrl Pts',(201.366004931376,-0.194868239746226,
123.804334868162));
#231436=CARTESIAN_POINT('Ctrl Pts',(201.087557307562,-5.99465095761073,
127.184623883922));
#231437=CARTESIAN_POINT('Ctrl Pts',(200.80910968375,-6.2856423003101,133.891274124028));
#231438=CARTESIAN_POINT('Ctrl Pts',(200.530662059936,-0.80043543977546,
137.76120165575));
#231439=CARTESIAN_POINT('Ctrl Pts',(200.252214436124,5.42033248649604,135.238132133988));
#231440=CARTESIAN_POINT('Ctrl Pts',(199.973766812311,6.66007965562565,128.640643190398));
#231441=CARTESIAN_POINT('Ctrl Pts',(199.695319188498,1.77953898422249,124.031504858911));
#231442=CARTESIAN_POINT('Ctrl Pts',(199.416871564685,-4.73631107837294,
125.646290097223));
#231443=CARTESIAN_POINT('Ctrl Pts',(199.138423940872,-6.89972264160091,
132.00109015798));
#231444=CARTESIAN_POINT('Ctrl Pts',(198.859976317059,-2.72262616738874,
137.256154234582));
#231445=CARTESIAN_POINT('Ctrl Pts',(198.581528693247,3.95643074697165,136.582335164788));
#231446=CARTESIAN_POINT('Ctrl Pts',(198.303081069434,6.999721087252,130.598839755845));
#231447=CARTESIAN_POINT('Ctrl Pts',(198.024633445621,3.61060970373355,124.804207978572));
#231448=CARTESIAN_POINT('Ctrl Pts',(197.746185821808,-3.09647560942607,
124.523423352781));
#231449=CARTESIAN_POINT('Ctrl Pts',(197.467738197995,-6.9580511087663,130.014513232485));
#231450=CARTESIAN_POINT('Ctrl Pts',(197.189290574182,-4.4255175588443,136.231434272887));
#231451=CARTESIAN_POINT('Ctrl Pts',(196.910842950369,2.17385042910367,137.461139751337));
#231452=CARTESIAN_POINT('Ctrl Pts',(196.632395326556,6.77555607120273,132.573590407591));
#231453=CARTESIAN_POINT('Ctrl Pts',(196.353947702743,5.15085668818228,126.060205318492));
#231454=CARTESIAN_POINT('Ctrl Pts',(196.07550007893,-1.20722835793932,123.90646718437));
#231455=CARTESIAN_POINT('Ctrl Pts',(195.797052455118,-6.45592951949867,
128.091556134528));
#231456=CARTESIAN_POINT('Ctrl Pts',(195.518604831305,-5.77194684232935,
134.769579876729));
#231457=CARTESIAN_POINT('Ctrl Pts',(195.240157207492,0.216173007661386,
137.80376083149));
#231458=CARTESIAN_POINT('Ctrl Pts',(194.961709583679,6.00564042424985,134.405834929363));
#231459=CARTESIAN_POINT('Ctrl Pts',(194.683261959866,6.2762176827981,127.698330076496));
#231460=CARTESIAN_POINT('Ctrl Pts',(194.404814336053,0.779257501134259,
123.845115552844));
#231461=CARTESIAN_POINT('Ctrl Pts',(194.12636671224,-5.43380225522669,126.387107265649));
#231462=CARTESIAN_POINT('Ctrl Pts',(193.847919088427,-6.65346319503207,
132.988339014042));
#231463=CARTESIAN_POINT('Ctrl Pts',(193.569471464615,-1.75891649835014,
137.58260130935));
#231464=CARTESIAN_POINT('Ctrl Pts',(193.291023840801,4.75198853246758,135.947991544374));
#231465=CARTESIAN_POINT('Ctrl Pts',(193.012576216989,6.89604824949333,129.586636238002));
#231466=CARTESIAN_POINT('Ctrl Pts',(192.734128593176,2.70297651592057,124.344310147306));
#231467=CARTESIAN_POINT('Ctrl Pts',(192.455680969363,-3.97399858803937,
125.038454847768));
#231468=CARTESIAN_POINT('Ctrl Pts',(192.17723334555,-6.99906313021511,131.031185270517));
#231469=CARTESIAN_POINT('Ctrl Pts',(191.898785721737,-3.59233057896577,
136.815474918205));
#231470=CARTESIAN_POINT('Ctrl Pts',(191.620338097924,3.11557827924791,137.075844182864));
#231471=CARTESIAN_POINT('Ctrl Pts',(191.341890474111,6.96042290329331,131.573026430018));
#231472=CARTESIAN_POINT('Ctrl Pts',(191.063442850298,4.40897891477476,125.363842346942));
#231473=CARTESIAN_POINT('Ctrl Pts',(190.784995226486,-2.19410130582752,
124.154228770475));
#231474=CARTESIAN_POINT('Ctrl Pts',(190.506547602672,-6.78090961418206,
129.055761484483));
#231475=CARTESIAN_POINT('Ctrl Pts',(190.22809997886,-5.13639325295408,135.564171377977));
#231476=CARTESIAN_POINT('Ctrl Pts',(189.949652355047,1.22821758097839,137.698547712335));
#231477=CARTESIAN_POINT('Ctrl Pts',(189.671204731234,6.46415645975623,133.497502906364));
#231478=CARTESIAN_POINT('Ctrl Pts',(189.392757107421,5.75985134361714,126.821591904301));
#231479=CARTESIAN_POINT('Ctrl Pts',(189.114309483608,-0.237475772924818,
123.80565078066));
#231480=CARTESIAN_POINT('Ctrl Pts',(188.835861859795,-6.01657425548534,
127.221182091151));
#231481=CARTESIAN_POINT('Ctrl Pts',(188.557414235982,-6.2667349232476,133.929479419415));
#231482=CARTESIAN_POINT('Ctrl Pts',(188.278966612169,-0.758072343566082,
137.76594523932));
#231483=CARTESIAN_POINT('Ctrl Pts',(188.000518988357,5.44722168595988,135.205054884148));
#231484=CARTESIAN_POINT('Ctrl Pts',(187.722071364544,6.64678509766207,128.600141483854));
#231485=CARTESIAN_POINT('Ctrl Pts',(187.443623740731,1.73827771811677,124.02079778535));
#231486=CARTESIAN_POINT('Ctrl Pts',(187.165176116918,-4.76762196479028,
125.675216934184));
#231487=CARTESIAN_POINT('Ctrl Pts',(186.886728493105,-6.89230997333645,
132.043068555446));
#231488=CARTESIAN_POINT('Ctrl Pts',(186.608280869292,-2.68330182444739,
137.272608096043));
#231489=CARTESIAN_POINT('Ctrl Pts',(186.329833245479,3.99152961452714,136.558144195375));
#231490=CARTESIAN_POINT('Ctrl Pts',(186.051385621667,6.99834033481346,130.556234274655));
#231491=CARTESIAN_POINT('Ctrl Pts',(185.772937997853,3.5740181753383,124.782340341422));
#231492=CARTESIAN_POINT('Ctrl Pts',(185.494490374041,-3.13465208677821,
124.542388849921));
#231493=CARTESIAN_POINT('Ctrl Pts',(185.216042750227,-6.96273021741339,
130.056883498557));
#231494=CARTESIAN_POINT('Ctrl Pts',(184.937595126415,-4.39239942652681,
136.258273103275));
#231495=CARTESIAN_POINT('Ctrl Pts',(184.659147502602,2.21433185669671,137.447783572063));
#231496=CARTESIAN_POINT('Ctrl Pts',(184.380699878789,6.78620033974098,132.532312894923));
#231497=CARTESIAN_POINT('Ctrl Pts',(184.102252254976,5.12188223488049,126.028938490053));
#231498=CARTESIAN_POINT('Ctrl Pts',(183.823804631163,-1.24919542597752,
123.913943728027));
#231499=CARTESIAN_POINT('Ctrl Pts',(183.54535700735,-6.47232351695142,128.130905471908));
#231500=CARTESIAN_POINT('Ctrl Pts',(183.266909383538,-5.74770248642891,
134.804641889104));
#231501=CARTESIAN_POINT('Ctrl Pts',(182.988461759724,0.258776338245136,
137.80231524236));
#231502=CARTESIAN_POINT('Ctrl Pts',(182.710014135912,6.02745234999885,134.369210164519));
#231503=CARTESIAN_POINT('Ctrl Pts',(182.431566512099,6.25719410952084,127.66018250561));
#231504=CARTESIAN_POINT('Ctrl Pts',(182.153118888286,0.73688016331929,123.840500929948));
#231505=CARTESIAN_POINT('Ctrl Pts',(181.874671264473,-5.46059065437546,
126.420266203747));
#231506=CARTESIAN_POINT('Ctrl Pts',(181.59622364066,-6.64004542538295,133.028800068927));
#231507=CARTESIAN_POINT('Ctrl Pts',(181.317776016847,-1.71762283471616,
137.593182748215));
#231508=CARTESIAN_POINT('Ctrl Pts',(181.039328393035,4.78321123051439,135.918969541833));
#231509=CARTESIAN_POINT('Ctrl Pts',(180.760880769221,6.88850784776155,129.544680596588));
#231510=CARTESIAN_POINT('Ctrl Pts',(180.482433145409,2.66360227523266,124.32797605183));
#231511=CARTESIAN_POINT('Ctrl Pts',(180.203985521595,-4.00902366402984,
125.062752534008));
#231512=CARTESIAN_POINT('Ctrl Pts',(179.925537897783,-6.99755270774298,
131.073786351827));
#231513=CARTESIAN_POINT('Ctrl Pts',(179.64709027397,-3.5556726624947,136.837231082039));
#231514=CARTESIAN_POINT('Ctrl Pts',(179.368642650157,3.15369685531979,137.056762577506));
#231515=CARTESIAN_POINT('Ctrl Pts',(179.090195026344,6.96497302975191,131.530642118605));
#231516=CARTESIAN_POINT('Ctrl Pts',(178.811747402531,4.37577924769062,125.337104441072));
#231517=CARTESIAN_POINT('Ctrl Pts',(178.533299778718,-2.23454189429802,
124.167708099424));
#231518=CARTESIAN_POINT('Ctrl Pts',(178.254852154906,-6.79142819886702,
129.097071203448));
#231519=CARTESIAN_POINT('Ctrl Pts',(177.976404531092,-5.10732376838957,
135.595349873321));
#231520=CARTESIAN_POINT('Ctrl Pts',(177.69795690728,1.27016169860089,137.690943469992));
#231521=CARTESIAN_POINT('Ctrl Pts',(177.419509283467,6.48043061542571,133.458103853558));
#231522=CARTESIAN_POINT('Ctrl Pts',(177.141061659654,5.73550038331004,126.786603845811));
#231523=CARTESIAN_POINT('Ctrl Pts',(176.862614035841,-0.280074506296806,
123.807226032976));
#231524=CARTESIAN_POINT('Ctrl Pts',(176.584166412028,-6.0382746070172,127.257873074351));
#231525=CARTESIAN_POINT('Ctrl Pts',(176.305718788215,-6.24759533000263,
133.967568912391));
#231526=CARTESIAN_POINT('Ctrl Pts',(176.027271164402,-0.71568115671533,
137.770430858802));
#231527=CARTESIAN_POINT('Ctrl Pts',(175.748823540589,5.4739090366252,135.171814564968));
#231528=CARTESIAN_POINT('Ctrl Pts',(175.470375916777,6.63324424063007,128.559721455457));
#231529=CARTESIAN_POINT('Ctrl Pts',(175.191928292964,1.69695203949225,124.010342079205));
#231530=CARTESIAN_POINT('Ctrl Pts',(174.913480669151,-4.79875618522306,
125.704333833448));
#231531=CARTESIAN_POINT('Ctrl Pts',(174.635033045338,-6.88464190799096,
132.085001052137));
#231532=CARTESIAN_POINT('Ctrl Pts',(174.356585421525,-2.64387805077028,
137.288822274217));
#231533=CARTESIAN_POINT('Ctrl Pts',(174.078137797712,4.02648057448505,136.533740017397));
#231534=CARTESIAN_POINT('Ctrl Pts',(173.799690173899,6.99670025630013,130.513637987877));
#231535=CARTESIAN_POINT('Ctrl Pts',(173.521242550086,3.53729421038521,124.76069585245));
#231536=CARTESIAN_POINT('Ctrl Pts',(173.242794926273,-3.17271240844464,
124.561586386726));
#231537=CARTESIAN_POINT('Ctrl Pts',(172.96434730246,-6.96715131953175,130.099281462668));
#231538=CARTESIAN_POINT('Ctrl Pts',(172.685899678648,-4.35911853223319,
136.284909836929));
#231539=CARTESIAN_POINT('Ctrl Pts',(172.407452054835,2.25473123140845,137.434181218309));
#231540=CARTESIAN_POINT('Ctrl Pts',(172.129004431022,6.79659314313001,132.490971352347));
#231541=CARTESIAN_POINT('Ctrl Pts',(171.850556807209,5.09271798834896,125.997848616637));
#231542=CARTESIAN_POINT('Ctrl Pts',(171.572109183396,-1.29111620461978,
123.921675598615));
#231543=CARTESIAN_POINT('Ctrl Pts',(171.293661559583,-6.48847768007612,
128.170353875152));
#231544=CARTESIAN_POINT('Ctrl Pts',(171.01521393577,-5.72324514729908,134.839555669585));
#231545=CARTESIAN_POINT('Ctrl Pts',(170.736766311957,0.301370079776633,
137.800610341449));
#231546=CARTESIAN_POINT('Ctrl Pts',(170.458318688145,6.04904092628448,134.332453302864));
#231547=CARTESIAN_POINT('Ctrl Pts',(170.179871064331,6.23793867361471,127.6221514434));
#231548=CARTESIAN_POINT('Ctrl Pts',(169.901423440519,0.694475520138818,
123.836144355433));
#231549=CARTESIAN_POINT('Ctrl Pts',(169.622975816706,-5.4871767093294,126.453587596077));
#231550=CARTESIAN_POINT('Ctrl Pts',(169.344528192893,-6.62638160640872,
133.06917869639));
#231551=CARTESIAN_POINT('Ctrl Pts',(169.06608056908,-1.67626552393645,137.603512624779));
#231552=CARTESIAN_POINT('Ctrl Pts',(168.787632945267,4.81425668490999,135.88975801558));
#231553=CARTESIAN_POINT('Ctrl Pts',(168.509185321454,6.88071218983824,129.50277163308));
#231554=CARTESIAN_POINT('Ctrl Pts',(168.230737697641,2.62412933378287,124.311881941165));
#231555=CARTESIAN_POINT('Ctrl Pts',(167.952290073828,-4.0439001841742,125.087262977647));
#231556=CARTESIAN_POINT('Ctrl Pts',(167.673842450016,-6.99578298838191,
131.116377449467));
#231557=CARTESIAN_POINT('Ctrl Pts',(167.395394826203,-3.51888298926545,
136.858763695638));
#231558=CARTESIAN_POINT('Ctrl Pts',(167.11694720239,3.19169856999505,137.037449287095));
#231559=CARTESIAN_POINT('Ctrl Pts',(166.838499578577,6.96926506657354,131.488230894564));
#231560=CARTESIAN_POINT('Ctrl Pts',(166.560051954764,4.34241743449723,125.310569126392));
#231561=CARTESIAN_POINT('Ctrl Pts',(166.281604330951,-2.27489968099678,
124.181433351974));
#231562=CARTESIAN_POINT('Ctrl Pts',(166.003156707138,-6.80169512468258,
129.13844418665));
#231563=CARTESIAN_POINT('Ctrl Pts',(165.724709083325,-5.0780650300646,135.626350836796));
#231564=CARTESIAN_POINT('Ctrl Pts',(165.446261459512,1.31205874991464,137.683084042787));
#231565=CARTESIAN_POINT('Ctrl Pts',(165.1678138357,6.49646463635559,133.418606465321));
#231566=CARTESIAN_POINT('Ctrl Pts',(164.889366211887,5.71093689192698,126.751764666776));
#231567=CARTESIAN_POINT('Ctrl Pts',(164.610918588074,-0.322662861405092,
123.809060566689));
#231568=CARTESIAN_POINT('Ctrl Pts',(164.332470964261,-6.05975120806294,
127.29469547395));
#231569=CARTESIAN_POINT('Ctrl Pts',(164.054023340448,-6.22822422981513,
134.00554119152));
#231570=CARTESIAN_POINT('Ctrl Pts',(163.775575716635,-0.673263450036036,
137.774658347991));
#231571=CARTESIAN_POINT('Ctrl Pts',(163.497128092822,5.50039354957815,135.138412408175));
#231572=CARTESIAN_POINT('Ctrl Pts',(163.218680469009,6.61945758629338,128.51938460299));
#231573=CARTESIAN_POINT('Ctrl Pts',(162.940232845196,1.65556347968583,124.000138127916));
#231574=CARTESIAN_POINT('Ctrl Pts',(162.661785221384,-4.82971258598073,
125.733639716082));
#231575=CARTESIAN_POINT('Ctrl Pts',(162.383337597571,-6.87671872970774,
132.126886094224));
#231576=CARTESIAN_POINT('Ctrl Pts',(162.104889973758,-2.60435630721971,
137.304796168278));
#231577=CARTESIAN_POINT('Ctrl Pts',(161.826442349945,4.06128233172446,136.509123535159));
#231578=CARTESIAN_POINT('Ctrl Pts',(161.547994726132,6.99480091248578,130.471052473933));
#231579=CARTESIAN_POINT('Ctrl Pts',(161.269547102319,3.50043916969439,124.739275313697));
#231580=CARTESIAN_POINT('Ctrl Pts',(160.991099478506,-3.21065516408591,
124.581015251828));
#231581=CARTESIAN_POINT('Ctrl Pts',(160.712651854693,-6.97131425129578,
130.141705553748));
#231582=CARTESIAN_POINT('Ctrl Pts',(160.434204230881,-4.32567610919938,
136.311343486817));
#231583=CARTESIAN_POINT('Ctrl Pts',(160.155756607067,2.29504705622523,137.420333194114));
#231584=CARTESIAN_POINT('Ctrl Pts',(159.877308983254,6.80673409626067,132.449567311792));
#231585=CARTESIAN_POINT('Ctrl Pts',(159.598861359442,5.06336502927952,125.966936850291));
#231586=CARTESIAN_POINT('Ctrl Pts',(159.320413735629,-1.33298914047637,
123.929662509627));
#231587=CARTESIAN_POINT('Ctrl Pts',(159.041966111816,-6.50439141027418,
128.209899882485));
#231588=CARTESIAN_POINT('Ctrl Pts',(158.763518488003,-5.69857573121565,
134.874319924428));
#231589=CARTESIAN_POINT('Ctrl Pts',(158.48507086419,0.343952653928878,137.798646191931));
#231590=CARTESIAN_POINT('Ctrl Pts',(158.206623240377,6.07040535313402,134.295565706438));
#231591=CARTESIAN_POINT('Ctrl Pts',(157.928175616564,6.2184520885971,127.584238299121));
#231592=CARTESIAN_POINT('Ctrl Pts',(157.649727992752,0.652045142912632,
123.832045990734));
#231593=CARTESIAN_POINT('Ctrl Pts',(157.371280368939,-5.51355943493244,
126.487070207899));
#231594=CARTESIAN_POINT('Ctrl Pts',(157.092832745126,-6.61247224442723,
133.109473400187));
#231595=CARTESIAN_POINT('Ctrl Pts',(156.814385121313,-1.63484609852131,
137.613590556265));
#231596=CARTESIAN_POINT('Ctrl Pts',(156.5359374975,4.84512374525377,135.860358048054));
#231597=CARTESIAN_POINT('Ctrl Pts',(156.257489873687,6.87266156459436,129.46091090043));
#231598=CARTESIAN_POINT('Ctrl Pts',(155.979042249874,2.58455915425555,124.296028411687));
#231599=CARTESIAN_POINT('Ctrl Pts',(155.700594626061,-4.07862685611001,
125.111985270442));
#231600=CARTESIAN_POINT('Ctrl Pts',(155.422147002248,-6.99375403770952,
131.158956985208));
#231601=CARTESIAN_POINT('Ctrl Pts',(155.143699378435,-3.48196292253304,
136.880071961106));
#231602=CARTESIAN_POINT('Ctrl Pts',(154.865251754623,3.22958201510593,137.017905027291));
#231603=CARTESIAN_POINT('Ctrl Pts',(154.58680413081,6.97329885471516,131.445794329457));
#231604=CARTESIAN_POINT('Ctrl Pts',(154.308356506997,4.30889471142897,125.284237386175));
#231605=CARTESIAN_POINT('Ctrl Pts',(154.029908883184,-2.31517317045128,
124.195404019528));
#231606=CARTESIAN_POINT('Ctrl Pts',(153.751461259371,-6.81171001118396,
129.179878900999));
#231607=CARTESIAN_POINT('Ctrl Pts',(153.473013635558,-5.04861812217248,
135.65717311965));
#231608=CARTESIAN_POINT('Ctrl Pts',(153.194566011745,1.3539071824088,137.674969721956));
#231609=CARTESIAN_POINT('Ctrl Pts',(152.916118387933,6.51225792839928,133.379012205241));
#231610=CARTESIAN_POINT('Ctrl Pts',(152.637670764119,5.68616177967723,126.717075658174));
#231611=CARTESIAN_POINT('Ctrl Pts',(152.359223140307,-0.365239260122265,
123.811154313817));
#231612=CARTESIAN_POINT('Ctrl Pts',(152.080775516494,-6.08100326279917,
127.331647925483));
#231613=CARTESIAN_POINT('Ctrl Pts',(151.802327892681,-6.20862234048841,
134.043394849727));
#231614=CARTESIAN_POINT('Ctrl Pts',(151.523880268868,-0.630820795332096,
137.778627550233));
#231615=CARTESIAN_POINT('Ctrl Pts',(151.245432645055,5.52667424342534,135.104849651499));
#231616=CARTESIAN_POINT('Ctrl Pts',(150.966985021242,6.60542564552152,128.479132421149));
#231617=CARTESIAN_POINT('Ctrl Pts',(150.688537397429,1.61411357236584,123.990186309594));
#231618=CARTESIAN_POINT('Ctrl Pts',(150.410089773616,-4.86049001996232,
125.763133496143));
#231619=CARTESIAN_POINT('Ctrl Pts',(150.131642149803,-6.8685407320831,132.168722129643));
#231620=CARTESIAN_POINT('Ctrl Pts',(149.853194525991,-2.56473805828847,
137.32052918631));
#231621=CARTESIAN_POINT('Ctrl Pts',(149.574746902178,4.09593359665354,136.484295660832));
#231622=CARTESIAN_POINT('Ctrl Pts',(149.296299278365,6.99264237375128,130.428479310845));
#231623=CARTESIAN_POINT('Ctrl Pts',(149.017851654552,3.46345441894284,124.718079518912));
#231624=CARTESIAN_POINT('Ctrl Pts',(148.739404030739,-3.24847894771935,
124.600674725279));
#231625=CARTESIAN_POINT('Ctrl Pts',(148.460956406926,-6.97521885844655,
130.184154199754));
#231626=CARTESIAN_POINT('Ctrl Pts',(148.182508783113,-4.29207339664657,
136.337573073429));
#231627=CARTESIAN_POINT('Ctrl Pts',(147.9040611593,2.33527783722936,137.406240012622));
#231628=CARTESIAN_POINT('Ctrl Pts',(147.625613535487,6.81662282335624,132.408102307496));
#231629=CARTESIAN_POINT('Ctrl Pts',(147.347165911675,5.03382444535687,125.936204336462));
#231630=CARTESIAN_POINT('Ctrl Pts',(147.068718287862,-1.37481268193005,
123.937904165105));
#231631=CARTESIAN_POINT('Ctrl Pts',(146.790270664049,-6.52006411785656,
128.249542028514));
#231632=CARTESIAN_POINT('Ctrl Pts',(146.511823040236,-5.67369515231286,
134.908933365434));
#231633=CARTESIAN_POINT('Ctrl Pts',(146.233375416423,0.386522482789046,
137.796422866589));
#231634=CARTESIAN_POINT('Ctrl Pts',(145.95492779261,6.09154483888081,134.258548742122));
#231635=CARTESIAN_POINT('Ctrl Pts',(145.676480168797,6.19873507655051,127.546444477659));
#231636=CARTESIAN_POINT('Ctrl Pts',(145.398032544984,0.609590603913882,
123.828205987717));
#231637=CARTESIAN_POINT('Ctrl Pts',(145.119584921171,-5.53973785356302,
126.520712798507));
#231638=CARTESIAN_POINT('Ctrl Pts',(144.841137297358,-6.59831785485502,
133.149682687181));
#231639=CARTESIAN_POINT('Ctrl Pts',(144.562689673546,-1.59336609328267,
137.623416169231));
#231640=CARTESIAN_POINT('Ctrl Pts',(144.284242049733,4.87581126775532,135.830770728684));
#231641=CARTESIAN_POINT('Ctrl Pts',(144.00579442592,6.86435627034879,129.419099949804));
#231642=CARTESIAN_POINT('Ctrl Pts',(143.727346802107,2.54489320293839,124.280416050852));
#231643=CARTESIAN_POINT('Ctrl Pts',(143.448899178294,-4.11320239302776,
125.136918496298));
#231644=CARTESIAN_POINT('Ctrl Pts',(143.170451554481,-6.99146593090932,
131.201523381251));
#231645=CARTESIAN_POINT('Ctrl Pts',(142.892003930668,-3.44491383038404,
136.901155088855));
#231646=CARTESIAN_POINT('Ctrl Pts',(142.613556306855,3.26734578686757,136.998130522314));
#231647=CARTESIAN_POINT('Ctrl Pts',(142.335108683042,6.97707424470332,131.403333995789));
#231648=CARTESIAN_POINT('Ctrl Pts',(142.05666105923,4.27521232068256,125.258110196154));
#231649=CARTESIAN_POINT('Ctrl Pts',(141.778213435417,-2.35536087031262,
124.209619584399));
#231650=CARTESIAN_POINT('Ctrl Pts',(141.499765811604,-6.8214724872659,129.221373811115));
#231651=CARTESIAN_POINT('Ctrl Pts',(141.221318187791,-5.01898413587917,
135.687815579753));
#231652=CARTESIAN_POINT('Ctrl Pts',(140.942870563978,1.39570544537436,137.666600808179));
#231653=CARTESIAN_POINT('Ctrl Pts',(140.664422940165,6.52780990633047,133.339322540502));
#231654=CARTESIAN_POINT('Ctrl Pts',(140.385975316352,5.66117596461176,126.68253810542));
#231655=CARTESIAN_POINT('Ctrl Pts',(140.10752769254,-0.407802124764288,
123.813507196776));
#231656=CARTESIAN_POINT('Ctrl Pts',(139.829080068726,-6.10202998372316,
127.368729059661));
#231657=CARTESIAN_POINT('Ctrl Pts',(139.550632444914,-6.18879038837768,
134.081128484328));
#231658=CARTESIAN_POINT('Ctrl Pts',(139.272184821101,-0.588354765331746,
137.78233831845));
#231659=CARTESIAN_POINT('Ctrl Pts',(138.993737197288,5.55275014432601,135.071127538621));
#231660=CARTESIAN_POINT('Ctrl Pts',(138.715289573475,6.59114893827324,128.438966401494));
#231661=CARTESIAN_POINT('Ctrl Pts',(138.436841949662,1.57260385347371,123.980486993006));
#231662=CARTESIAN_POINT('Ctrl Pts',(138.158394325849,-4.8910873466988,125.792814080728));
#231663=CARTESIAN_POINT('Ctrl Pts',(137.879946702036,-6.86010821815569,
132.210507608145));
#231664=CARTESIAN_POINT('Ctrl Pts',(137.601499078223,-2.52502477204539,
137.336020745319));
#231665=CARTESIAN_POINT('Ctrl Pts',(137.32305145441,4.13043308525698,136.459257314423));
#231666=CARTESIAN_POINT('Ctrl Pts',(137.044603830598,6.99022472008204,130.385920076178));
#231667=CARTESIAN_POINT('Ctrl Pts',(136.766156206785,3.42634132861412,124.69710925351));
#231668=CARTESIAN_POINT('Ctrl Pts',(136.487708582972,-3.28618235777073,
124.620564078594));
#231669=CARTESIAN_POINT('Ctrl Pts',(136.209260959159,-6.97886499629743,
130.226625827737));
#231670=CARTESIAN_POINT('Ctrl Pts',(135.930813335346,-4.25831163973555,
136.363597624819));
#231671=CARTESIAN_POINT('Ctrl Pts',(135.652365711533,2.37542208365453,137.391902196061));
#231672=CARTESIAN_POINT('Ctrl Pts',(135.37391808772,6.82625895798624,132.366577875963));
#231673=CARTESIAN_POINT('Ctrl Pts',(135.095470463907,5.00409733121823,125.905652213954));
#231674=CARTESIAN_POINT('Ctrl Pts',(134.817022840094,-1.4165852791943,123.946400259653));
#231675=CARTESIAN_POINT('Ctrl Pts',(134.538575216282,-6.53549522206528,
128.289278844285));
#231676=CARTESIAN_POINT('Ctrl Pts',(134.260127592469,-5.64860433254967,
134.943394709987));
#231677=CARTESIAN_POINT('Ctrl Pts',(133.981679968656,0.429077988916399,
137.793940447809));
#231678=CARTESIAN_POINT('Ctrl Pts',(133.703232344843,6.1124586001935,134.221403781595));
#231679=CARTESIAN_POINT('Ctrl Pts',(133.42478472103,6.17878836809604,127.508771379477));
#231680=CARTESIAN_POINT('Ctrl Pts',(133.146337097217,0.567113476311158,
123.824624488677));
#231681=CARTESIAN_POINT('Ctrl Pts',(132.867889473404,-5.5657109951702,126.554514121259));
#231682=CARTESIAN_POINT('Ctrl Pts',(132.589441849591,-6.58391896218814,
133.189805067404));
#231683=CARTESIAN_POINT('Ctrl Pts',(132.310994225778,-1.55182704527753,
137.632989099587));
#231684=CARTESIAN_POINT('Ctrl Pts',(132.032546601965,4.90631811527725,135.800997153839));
#231685=CARTESIAN_POINT('Ctrl Pts',(131.754098978153,6.85579661485726,129.377340330521));
#231686=CARTESIAN_POINT('Ctrl Pts',(131.47565135434,2.50513294966777,124.265045437181));
#231687=CARTESIAN_POINT('Ctrl Pts',(131.197203730527,-4.14762551371829,
125.162061731307));
#231688=CARTESIAN_POINT('Ctrl Pts',(130.918756106714,-6.98891875276791,
131.244075060281));
#231689=CARTESIAN_POINT('Ctrl Pts',(130.640308482901,-3.4077370856862,136.922012297644));
#231690=CARTESIAN_POINT('Ctrl Pts',(130.361860859088,3.30498848592948,136.978126504915));
#231691=CARTESIAN_POINT('Ctrl Pts',(130.083413235275,6.98059109663955,131.360851466943));
#231692=CARTESIAN_POINT('Ctrl Pts',(129.804965611462,4.24137151037132,125.232188524482));
#231693=CARTESIAN_POINT('Ctrl Pts',(129.526517987649,-2.39546129141071,
124.224079519825));
#231694=CARTESIAN_POINT('Ctrl Pts',(129.248070363836,-6.83098219117618,
129.262927379388));
#231695=CARTESIAN_POINT('Ctrl Pts',(128.969622740024,-4.98916416928312,
135.718277081636));
#231696=CARTESIAN_POINT('Ctrl Pts',(128.691175116211,1.43745198996158,137.657977611568));
#231697=CARTESIAN_POINT('Ctrl Pts',(128.412727492398,6.54311999386511,133.299538941816));
#231698=CARTESIAN_POINT('Ctrl Pts',(128.134279868585,5.63598037258881,126.648153288314));
#231699=CARTESIAN_POINT('Ctrl Pts',(127.855832244772,-0.450349878148651,
123.81611912838));
#231700=CARTESIAN_POINT('Ctrl Pts',(127.577384620959,-6.12283059168226,
127.40593750243));
#231701=CARTESIAN_POINT('Ctrl Pts',(127.298936997146,-6.16872910836309,
134.118740697091));
#231702=CARTESIAN_POINT('Ctrl Pts',(127.020489373333,-0.545866933628919,
137.785790515136));
#231703=CARTESIAN_POINT('Ctrl Pts',(126.742041749521,5.57862028602806,135.037247319125));
#231704=CARTESIAN_POINT('Ctrl Pts',(126.463594125708,6.57662799357718,128.398888032392));
#231705=CARTESIAN_POINT('Ctrl Pts',(126.185146501895,1.53103586116759,123.971040537565));
#231706=CARTESIAN_POINT('Ctrl Pts',(125.906698878082,-4.92150343239493,
125.822680370014));
#231707=CARTESIAN_POINT('Ctrl Pts',(125.628251254269,-6.85142150039552,
132.252240981353));
#231708=CARTESIAN_POINT('Ctrl Pts',(125.349803630456,-2.48521792008072,
137.351270271259));
#231709=CARTESIAN_POINT('Ctrl Pts',(125.071356006643,4.16477951914341,136.434009423738));
#231710=CARTESIAN_POINT('Ctrl Pts',(124.79290838283,6.98754804106521,130.343376346978));
#231711=CARTESIAN_POINT('Ctrl Pts',(124.514460759018,3.38910127394743,124.676365294554));
#231712=CARTESIAN_POINT('Ctrl Pts',(124.236013135205,-3.32376399712637,
124.640682574762));
#231713=CARTESIAN_POINT('Ctrl Pts',(123.957565511392,-6.98225252973936,
130.269118863895));
#231714=CARTESIAN_POINT('Ctrl Pts',(123.679117887579,-4.22439208952083,
136.389416176637));
#231715=CARTESIAN_POINT('Ctrl Pts',(123.400670263766,2.41547830794073,137.377320275725));
#231716=CARTESIAN_POINT('Ctrl Pts',(123.122222639953,6.83564214308024,132.324995555895));
#231717=CARTESIAN_POINT('Ctrl Pts',(122.84377501614,4.97418478841272,125.875281614887));
#231718=CARTESIAN_POINT('Ctrl Pts',(122.565327392328,-1.45830538437,123.955150478444));
#231719=CARTESIAN_POINT('Ctrl Pts',(122.286879768514,-6.55068415109515,
128.329108857337));
#231720=CARTESIAN_POINT('Ctrl Pts',(122.008432144702,-5.62330420167569,
134.977702681109));
#231721=CARTESIAN_POINT('Ctrl Pts',(121.729984520888,0.471617595401148,
137.791199027578));
#231722=CARTESIAN_POINT('Ctrl Pts',(121.451536897076,6.13314586210485,134.184132201278));
#231723=CARTESIAN_POINT('Ctrl Pts',(121.173089273263,6.15861270236637,127.471220400567));
#231724=CARTESIAN_POINT('Ctrl Pts',(120.89464164945,0.52461533410983,123.821301626325));
#231725=CARTESIAN_POINT('Ctrl Pts',(120.616194025637,-5.5914778973097,126.588472923636));
#231726=CARTESIAN_POINT('Ctrl Pts',(120.337746401824,-6.56927609998288,
133.229839054105));
#231727=CARTESIAN_POINT('Ctrl Pts',(120.059298778011,-1.51023049375061,
137.642308992603));
#231728=CARTESIAN_POINT('Ctrl Pts',(119.780851154198,4.93664315737715,135.77103842679));
#231729=CARTESIAN_POINT('Ctrl Pts',(119.502403530385,6.84698291530094,129.33563359));
#231730=CARTESIAN_POINT('Ctrl Pts',(119.223955906573,2.46527986777437,124.249917140239));
#231731=CARTESIAN_POINT('Ctrl Pts',(118.94550828276,-4.18189494262004,125.187414043775));
#231732=CARTESIAN_POINT('Ctrl Pts',(118.667060658947,-6.98611259767199,
131.28661044553));
#231733=CARTESIAN_POINT('Ctrl Pts',(118.388613035134,-3.37043406603744,
136.942642814599));
#231734=CARTESIAN_POINT('Ctrl Pts',(118.110165411321,3.34250871742766,136.95789371635));
#231735=CARTESIAN_POINT('Ctrl Pts',(117.831717787508,6.98384928020556,131.318348317123));
#231736=CARTESIAN_POINT('Ctrl Pts',(117.553270163695,4.20737353447909,125.206473331696));
#231737=CARTESIAN_POINT('Ctrl Pts',(117.274822539882,-2.43547294780967,
124.238783289987));
#231738=CARTESIAN_POINT('Ctrl Pts',(116.99637491607,-6.84023877052931,129.304538066038));
#231739=CARTESIAN_POINT('Ctrl Pts',(116.717927292256,-4.95915932737393,
135.748556496538));
#231740=CARTESIAN_POINT('Ctrl Pts',(116.439479668444,1.47914526923655,137.649100451659));
#231741=CARTESIAN_POINT('Ctrl Pts',(116.161032044631,6.55818762368211,133.259662883379));
#231742=CARTESIAN_POINT('Ctrl Pts',(115.882584420818,5.61057593724064,126.613922481));
#231743=CARTESIAN_POINT('Ctrl Pts',(115.604136797005,-0.49288094365267,
123.818990011842));
#231744=CARTESIAN_POINT('Ctrl Pts',(115.325689173192,-6.14340431590201,
127.443271875017));
#231745=CARTESIAN_POINT('Ctrl Pts',(115.047241549379,-6.14843924382291,
134.156230094282));
#231746=CARTESIAN_POINT('Ctrl Pts',(114.768793925566,-0.5033588746261,137.78898401237));
#231747=CARTESIAN_POINT('Ctrl Pts',(114.490346301753,5.60428370990391,135.003210248456));
#231748=CARTESIAN_POINT('Ctrl Pts',(114.211898677941,6.56186334951224,128.358898798961));
#231749=CARTESIAN_POINT('Ctrl Pts',(113.933451054127,1.48941113576461,123.961847293312));
#231750=CARTESIAN_POINT('Ctrl Pts',(113.655003430315,-4.95173714997151,
125.852731257293));
#231751=CARTESIAN_POINT('Ctrl Pts',(113.376555806502,-6.84248090069202,
132.293920702821));
#231752=CARTESIAN_POINT('Ctrl Pts',(113.098108182689,-2.4453189774521,137.366277199056));
#231753=CARTESIAN_POINT('Ctrl Pts',(112.819660558876,4.19897162559319,136.408552924347));
#231754=CARTESIAN_POINT('Ctrl Pts',(112.541212935063,6.98461243588604,130.300849699721));
#231755=CARTESIAN_POINT('Ctrl Pts',(112.26276531125,3.35173563488669,124.655848410718));
#231756=CARTESIAN_POINT('Ctrl Pts',(111.984317687437,-3.3612224731848,124.661029468288));
#231757=CARTESIAN_POINT('Ctrl Pts',(111.705870063624,-6.98538133324609,
130.311631733633));
#231758=CARTESIAN_POINT('Ctrl Pts',(111.427422439812,-4.1903160029037,136.415027772168));
#231759=CARTESIAN_POINT('Ctrl Pts',(111.148974815999,2.45544502578993,137.362494791951));
#231760=CARTESIAN_POINT('Ctrl Pts',(110.870527192186,6.84477203094083,132.28335688814));
#231761=CARTESIAN_POINT('Ctrl Pts',(110.592079568373,4.94408792536061,125.845093664656));
#231762=CARTESIAN_POINT('Ctrl Pts',(110.31363194456,-1.49997145150339,123.964154497236));
#231763=CARTESIAN_POINT('Ctrl Pts',(110.035184320747,-6.56563034211481,
128.369030591753));
#231764=CARTESIAN_POINT('Ctrl Pts',(109.756736696934,-5.59779569719655,
135.011856007506));
#231765=CARTESIAN_POINT('Ctrl Pts',(109.478289073121,0.514139725922464,
137.788198707481));
#231766=CARTESIAN_POINT('Ctrl Pts',(109.199841449309,6.15360585804082,134.146735382281));
#231767=CARTESIAN_POINT('Ctrl Pts',(108.921393825496,6.13820882697821,127.433792932393));
#231768=CARTESIAN_POINT('Ctrl Pts',(108.642946201683,0.482097752094529,
123.818237523792));
#231769=CARTESIAN_POINT('Ctrl Pts',(108.36449857787,-5.61703760517944,126.622587947283));
#231770=CARTESIAN_POINT('Ctrl Pts',(108.086050954057,-6.5543898108359,133.26978316381));
#231771=CARTESIAN_POINT('Ctrl Pts',(107.807603330244,-1.46857798007734,
137.651375502926));
#231772=CARTESIAN_POINT('Ctrl Pts',(107.529155706431,4.96678527034939,135.740895657668));
#231773=CARTESIAN_POINT('Ctrl Pts',(107.250708082618,6.83791549827476,129.2939812737));
#231774=CARTESIAN_POINT('Ctrl Pts',(106.972260458805,2.42533543402888,124.23503172061));
#231775=CARTESIAN_POINT('Ctrl Pts',(106.693812834992,-4.21600940986681,
125.212974494265));
#231776=CARTESIAN_POINT('Ctrl Pts',(106.415365211179,-6.98304756960462,
131.329127960835));
#231777=CARTESIAN_POINT('Ctrl Pts',(106.136917587367,-3.33300615371489,
136.96304587525));
#231778=CARTESIAN_POINT('Ctrl Pts',(105.858469963554,3.37990509103613,136.937432906355));
#231779=CARTESIAN_POINT('Ctrl Pts',(105.580022339741,6.98684867466819,131.275826121299));
#231780=CARTESIAN_POINT('Ctrl Pts',(105.301574715928,4.1732196528133,125.180965570684));
#231781=CARTESIAN_POINT('Ctrl Pts',(105.023127092115,-2.4753943568629,124.253730350031));
#231782=CARTESIAN_POINT('Ctrl Pts',(104.744679468302,-6.84924188231931,
129.346204329164));
#231783=CARTESIAN_POINT('Ctrl Pts',(104.466231844489,-4.92897072199215,
135.778652702442));
#231784=CARTESIAN_POINT('Ctrl Pts',(104.187784220676,1.52078373823962,137.639969657397));
#231785=CARTESIAN_POINT('Ctrl Pts',(103.909336596864,6.57301223744494,133.219695842813));
#231786=CARTESIAN_POINT('Ctrl Pts',(103.63088897305,5.58496359993783,126.579846951912));
#231787=CARTESIAN_POINT('Ctrl Pts',(103.352441349238,-0.535393745272065,
123.82211974078));
#231788=CARTESIAN_POINT('Ctrl Pts',(103.073993725425,-6.1637503940156,127.480730793984));
#231789=CARTESIAN_POINT('Ctrl Pts',(102.795546101612,-6.12792154660547,
134.193595286717));
#231790=CARTESIAN_POINT('Ctrl Pts',(102.517098477799,-0.460832163475232,
137.791918691816));
#231791=CARTESIAN_POINT('Ctrl Pts',(102.238650853986,5.6297394649859,134.96901758787));
#231792=CARTESIAN_POINT('Ctrl Pts',(101.960203230173,6.54685555318778,128.319000183017));
#231793=CARTESIAN_POINT('Ctrl Pts',(101.68175560636,1.44773121968427,123.952907600908));
#231794=CARTESIAN_POINT('Ctrl Pts',(101.403307982548,-4.981787379107,125.882965629019));
#231795=CARTESIAN_POINT('Ctrl Pts',(101.124860358735,-6.83328675034245,
132.335545228093));
#231796=CARTESIAN_POINT('Ctrl Pts',(100.846412734922,-2.4053294226295,137.38104097262));
#231797=CARTESIAN_POINT('Ctrl Pts',(100.567965111109,4.23300813760519,136.382888759548));
#231798=CARTESIAN_POINT('Ctrl Pts',(100.289517487296,6.98141801332452,130.258341710245));
#231799=CARTESIAN_POINT('Ctrl Pts',(100.011069863483,3.31424579602927,124.635559362262));
#231800=CARTESIAN_POINT('Ctrl Pts',(99.7326222396699,-3.39855639790849,
124.681604005209));
#231801=CARTESIAN_POINT('Ctrl Pts',(99.4541746158571,-6.98825129087862,
130.354162861621));
#231802=CARTESIAN_POINT('Ctrl Pts',(99.1757269920442,-4.15608464258612,
136.440431462363));
#231803=CARTESIAN_POINT('Ctrl Pts',(98.8972793682313,2.49532075622072,137.347426294104));
#231804=CARTESIAN_POINT('Ctrl Pts',(98.6188317444184,6.85364828325664,132.241663415635));
#231805=CARTESIAN_POINT('Ctrl Pts',(98.3403841206056,4.91380785731226,125.815089481885));
#231806=CARTESIAN_POINT('Ctrl Pts',(98.0619364967926,-1.54158193664305,
123.97341198238));
#231807=CARTESIAN_POINT('Ctrl Pts',(97.7834888729798,-6.58033324128762,
128.409042568218));
#231808=CARTESIAN_POINT('Ctrl Pts',(97.5050412491668,-5.57207976433927,
135.045853423614));
#231809=CARTESIAN_POINT('Ctrl Pts',(97.226593625354,0.55664280480716,137.784939598694));
#231810=CARTESIAN_POINT('Ctrl Pts',(96.948146001541,6.17383782984873,134.109214710358));
#231811=CARTESIAN_POINT('Ctrl Pts',(96.6696983777281,6.11757749800464,127.396490361844));
#231812=CARTESIAN_POINT('Ctrl Pts',(96.3912507539153,0.43956230576973,123.815432294619));
#231813=CARTESIAN_POINT('Ctrl Pts',(96.1128031301024,-5.64238917165504,
126.656857928054));
#231814=CARTESIAN_POINT('Ctrl Pts',(95.8343555062895,-6.53926064636413,
133.309635916377));
#231815=CARTESIAN_POINT('Ctrl Pts',(95.5559078824767,-1.42687104770695,
137.660188294596));
#231816=CARTESIAN_POINT('Ctrl Pts',(95.2774602586637,4.99674333726689,135.710569963425));
#231817=CARTESIAN_POINT('Ctrl Pts',(94.9990126348508,6.82859469977515,129.252384925061));
#231818=CARTESIAN_POINT('Ctrl Pts',(94.720565011038,2.38530112858694,124.22038972988));
#231819=CARTESIAN_POINT('Ctrl Pts',(94.442117387225,-4.24996765133445,125.238742135624));
#231820=CARTESIAN_POINT('Ctrl Pts',(94.1636697634123,-6.97972378214161,
131.371626030693));
#231821=CARTESIAN_POINT('Ctrl Pts',(93.885222139599,-3.29545473562348,136.983220723554));
#231822=CARTESIAN_POINT('Ctrl Pts',(93.6067745157866,3.41717622101856,136.91674483311));
#231823=CARTESIAN_POINT('Ctrl Pts',(93.3283268919733,6.98958916888377,131.233286455149));
#231824=CARTESIAN_POINT('Ctrl Pts',(93.0498792681607,4.13891113095855,125.155666186642));
#231825=CARTESIAN_POINT('Ctrl Pts',(92.7714316443476,-2.51522403926791,
124.268920146089));
#231826=CARTESIAN_POINT('Ctrl Pts',(92.4929840205349,-6.85799119293255,
129.387924624807));
#231827=CARTESIAN_POINT('Ctrl Pts',(92.2145363967218,-4.89859947178764,
135.808564584124));
#231828=CARTESIAN_POINT('Ctrl Pts',(91.9360887729091,1.562365854042,137.63058556713));
#231829=CARTESIAN_POINT('Ctrl Pts',(91.6576411490961,6.58759328582208,133.179639301113));
#231830=CARTESIAN_POINT('Ctrl Pts',(91.3791935252832,5.55914430975498,126.545927963732));
#231831=CARTESIAN_POINT('Ctrl Pts',(91.1007459014705,-0.57788670767935,
123.825508199223));
#231832=CARTESIAN_POINT('Ctrl Pts',(90.8222982776573,-6.18386807209161,
127.518312871276));
#231833=CARTESIAN_POINT('Ctrl Pts',(90.5438506538447,-6.10717677700159,
134.230834889814));
#231834=CARTESIAN_POINT('Ctrl Pts',(90.2654030300316,-0.41828837601907,
137.794594444728));
#231835=CARTESIAN_POINT('Ctrl Pts',(89.9869554062187,5.65498660800168,134.934670604388));
#231836=CARTESIAN_POINT('Ctrl Pts',(89.708507782406,6.53160516072318,128.279193663018));
#231837=CARTESIAN_POINT('Ctrl Pts',(89.430060158593,1.40599765739116,123.944221791613));
#231838=CARTESIAN_POINT('Ctrl Pts',(89.1516125347801,-5.01165300627911,
125.913382364846));
#231839=CARTESIAN_POINT('Ctrl Pts',(88.8731649109673,-6.82383939003939,
132.377113014756));
#231840=CARTESIAN_POINT('Ctrl Pts',(88.5947172871542,-2.36525073744058,
137.395561044874));
#231841=CARTESIAN_POINT('Ctrl Pts',(88.3162696633415,4.26688779394398,136.357017880338));
#231842=CARTESIAN_POINT('Ctrl Pts',(88.0378220395285,6.97796489175107,130.2158539537));
#231843=CARTESIAN_POINT('Ctrl Pts',(87.7593744157156,3.2766331465752,124.615498901007));
#231844=CARTESIAN_POINT('Ctrl Pts',(87.4809267919028,-3.43576438787495,
124.702405423128));
#231845=CARTESIAN_POINT('Ctrl Pts',(87.2024791680898,-6.99086229628967,
130.396710671853));
#231846=CARTESIAN_POINT('Ctrl Pts',(86.924031544277,-4.1216992770237,136.465626305881));
#231847=CARTESIAN_POINT('Ctrl Pts',(86.6455839204641,2.53510402162323,137.332115340552));
#231848=CARTESIAN_POINT('Ctrl Pts',(86.3671362966513,6.8622705711149,132.199916683345));
#231849=CARTESIAN_POINT('Ctrl Pts',(86.0886886728382,4.88334570630671,125.785270178391));
#231850=CARTESIAN_POINT('Ctrl Pts',(85.8102410490255,-1.58313529789712,
123.982922590838));
#231851=CARTESIAN_POINT('Ctrl Pts',(85.5317934252125,-6.59479230379227,
128.449143304076));
#231852=CARTESIAN_POINT('Ctrl Pts',(85.2533458013996,-5.5461573560172,135.079693669646));
#231853=CARTESIAN_POINT('Ctrl Pts',(84.9748981775869,0.599125257088023,
137.781421821987));
#231854=CARTESIAN_POINT('Ctrl Pts',(84.6964505537737,6.19384102782544,134.071571575853));
#231855=CARTESIAN_POINT('Ctrl Pts',(84.418002929961,6.09671947994716,127.359314071181));
#231856=CARTESIAN_POINT('Ctrl Pts',(84.1395553061481,0.397010571302045,
123.812886042756));
#231857=CARTESIAN_POINT('Ctrl Pts',(83.8611076823352,-5.66753165732491,
126.691281596061));
#231858=CARTESIAN_POINT('Ctrl Pts',(83.5826600585222,-6.52388916718428,
133.349395835046));
#231859=CARTESIAN_POINT('Ctrl Pts',(83.3042124347095,-1.38511124210516,
137.66874704105));
#231860=CARTESIAN_POINT('Ctrl Pts',(83.0257648108964,5.02651624802251,135.68006246779));
#231861=CARTESIAN_POINT('Ctrl Pts',(82.7473171870836,6.81902086518772,129.210846085452));
#231862=CARTESIAN_POINT('Ctrl Pts',(82.4688695632707,2.34517843493451,124.205991710613));
#231863=CARTESIAN_POINT('Ctrl Pts',(82.1904219394578,-4.28376840868787,
125.264716013022));
#231864=CARTESIAN_POINT('Ctrl Pts',(81.9119743156449,-6.97614135844701,
131.414103080323));
#231865=CARTESIAN_POINT('Ctrl Pts',(81.6335266918322,-3.25778120324508,
137.003166611925));
#231866=CARTESIAN_POINT('Ctrl Pts',(81.355079068019,3.45432072627939,136.895830263219));
#231867=CARTESIAN_POINT('Ctrl Pts',(81.0766314442065,6.99207066130227,131.190730894994));
#231868=CARTESIAN_POINT('Ctrl Pts',(80.7981838203932,4.10444924022979,125.130576117049));
#231869=CARTESIAN_POINT('Ctrl Pts',(80.5197361965806,-2.55496051912119,
124.284352115297));
#231870=CARTESIAN_POINT('Ctrl Pts',(80.2412885727675,-6.86648637816013,
129.429697407007));
#231871=CARTESIAN_POINT('Ctrl Pts',(79.9628409489547,-4.86804670217826,
135.838291033188));
#231872=CARTESIAN_POINT('Ctrl Pts',(79.6843933251418,1.6038900758031,137.620948528586));
#231873=CARTESIAN_POINT('Ctrl Pts',(79.405945701329,6.60193022850756,133.139494742587));
#231874=CARTESIAN_POINT('Ctrl Pts',(79.1274980775159,5.53311902343524,126.512166773338));
#231875=CARTESIAN_POINT('Ctrl Pts',(78.8490504537032,-0.620358256282274,
123.829155261608));
#231876=CARTESIAN_POINT('Ctrl Pts',(78.5706028298902,-6.2037566046621,127.556016714277));
#231877=CARTESIAN_POINT('Ctrl Pts',(78.2921552060774,-6.08620570371632,
134.267947523646));
#231878=CARTESIAN_POINT('Ctrl Pts',(78.0137075822645,-0.375729088733312,
137.797011171955));
#231879=CARTESIAN_POINT('Ctrl Pts',(77.7352599584516,5.68002420340909,134.90017057075));
#231880=CARTESIAN_POINT('Ctrl Pts',(77.4568123346387,6.51611273722737,128.23948071401));
#231881=CARTESIAN_POINT('Ctrl Pts',(77.1783647108257,1.36421199533782,123.935790187287));
#231882=CARTESIAN_POINT('Ctrl Pts',(76.8999170870129,-5.04133292480603,
125.94398033767));
#231883=CARTESIAN_POINT('Ctrl Pts',(76.6214694632,-6.81413916985829,132.418622522501));
#231884=CARTESIAN_POINT('Ctrl Pts',(76.3430218393871,-2.32508440701577,
137.409836877774));
#231885=CARTESIAN_POINT('Ctrl Pts',(76.0645742155741,4.30060933918641,136.33094124537));
#231886=CARTESIAN_POINT('Ctrl Pts',(75.7861265917614,6.97425319912241,130.173388004487));
#231887=CARTESIAN_POINT('Ctrl Pts',(75.5076789679483,3.23889908027492,124.595667770297));
#231888=CARTESIAN_POINT('Ctrl Pts',(75.2292313441357,-3.47284506432852,
124.72343295124));
#231889=CARTESIAN_POINT('Ctrl Pts',(74.9507837203226,-6.99321425272744,
130.439273587703));
#231890=CARTESIAN_POINT('Ctrl Pts',(74.6723360965098,-4.08716118037883,
136.490611369118));
#231891=CARTESIAN_POINT('Ctrl Pts',(74.3938884726969,2.57479334781394,137.316562498648));
#231892=CARTESIAN_POINT('Ctrl Pts',(74.1154408488841,6.87063857501356,132.158118238212));
#231893=CARTESIAN_POINT('Ctrl Pts',(73.836993225071,4.85270260113016,125.755636859138));
#231894=CARTESIAN_POINT('Ctrl Pts',(73.5585456012583,-1.62462999549052,
123.992685970191));
#231895=CARTESIAN_POINT('Ctrl Pts',(73.2800979774453,-6.60900699384299,
128.489331313375));
#231896=CARTESIAN_POINT('Ctrl Pts',(73.0016503536324,-5.52002943279461,
135.113375491641));
#231897=CARTESIAN_POINT('Ctrl Pts',(72.7232027298196,0.641585508562261,
137.777645507711));
#231898=CARTESIAN_POINT('Ctrl Pts',(72.4447551060067,6.21361471074508,134.033807373642));
#231899=CARTESIAN_POINT('Ctrl Pts',(72.1663074821937,6.07563554570727,127.322265437984));
#231900=CARTESIAN_POINT('Ctrl Pts',(71.8878598583809,0.354444125461637,
123.810598862555));
#231901=CARTESIAN_POINT('Ctrl Pts',(71.609412234568,-5.69246413052499,126.725857675724));
#231902=CARTESIAN_POINT('Ctrl Pts',(71.330964610755,-6.5082759428922,133.3890614465));
#231903=CARTESIAN_POINT('Ctrl Pts',(71.0525169869423,-1.34330011069692,
137.677051425141));
#231904=CARTESIAN_POINT('Ctrl Pts',(70.7740693631292,5.05610289937005,135.649374301231));
#231905=CARTESIAN_POINT('Ctrl Pts',(70.4956217393166,6.80919434927445,129.16936629411));
#231906=CARTESIAN_POINT('Ctrl Pts',(70.2171741155033,2.30496883983272,124.191838196331));
#231907=CARTESIAN_POINT('Ctrl Pts',(69.9387264916908,-4.31741042942741,
125.290895163988));
#231908=CARTESIAN_POINT('Ctrl Pts',(69.6602788678776,-6.97230043126892,
131.456557535721));
#231909=CARTESIAN_POINT('Ctrl Pts',(69.3818312440649,-3.21998695258627,
137.02288280126));
#231910=CARTESIAN_POINT('Ctrl Pts',(69.1033836202519,3.49133723041524,136.874689971681));
#231911=CARTESIAN_POINT('Ctrl Pts',(68.8249359964391,6.9942930599711,131.148161017746));
#231912=CARTESIAN_POINT('Ctrl Pts',(68.5464883726262,4.0698352576252,125.105696291628));
#231913=CARTESIAN_POINT('Ctrl Pts',(68.2680407488133,-2.59460232397255,
124.300025685817));
#231914=CARTESIAN_POINT('Ctrl Pts',(67.9895931250004,-6.87472712320984,
129.471521127857));
#231915=CARTESIAN_POINT('Ctrl Pts',(67.7111455011875,-4.83731354530826,
135.867830948109));
#231916=CARTESIAN_POINT('Ctrl Pts',(67.4326978773747,1.64535486482719,137.61105889887));
#231917=CARTESIAN_POINT('Ctrl Pts',(67.1542502535617,6.61602253424027,133.099263654809));
#231918=CARTESIAN_POINT('Ctrl Pts',(66.8758026297489,5.50688870535577,126.478564631767));
#231919=CARTESIAN_POINT('Ctrl Pts',(66.5973550059358,-0.662806817281494,
123.833060792792));
#231920=CARTESIAN_POINT('Ctrl Pts',(66.3189073821232,-6.22341525475008,
127.593840925854));
#231921=CARTESIAN_POINT('Ctrl Pts',(66.0404597583101,-6.0650091038406,134.304931812993));
#231922=CARTESIAN_POINT('Ctrl Pts',(65.7620121344974,-0.333155878668442,
137.799168783944));
#231923=CARTESIAN_POINT('Ctrl Pts',(65.4835645106842,5.70485132343066,134.865518765369));
#231924=CARTESIAN_POINT('Ctrl Pts',(65.2051168868716,6.50037885677781,128.199862807569));
#231925=CARTESIAN_POINT('Ctrl Pts',(64.9266692630585,1.32237578190785,123.927613100363));
#231926=CARTESIAN_POINT('Ctrl Pts',(64.6482216392459,-5.07082603488719,
125.974758413674));
#231927=CARTESIAN_POINT('Ctrl Pts',(64.3697740154327,-6.80418644924447,
132.460072213177));
#231928=CARTESIAN_POINT('Ctrl Pts',(64.09132639162,-2.28483191973344,137.423867942321));
#231929=CARTESIAN_POINT('Ctrl Pts',(63.812878767807,4.33417152376786,136.304659820925));
#231930=CARTESIAN_POINT('Ctrl Pts',(63.5344311439942,6.97028307297671,130.130945436197));
#231931=CARTESIAN_POINT('Ctrl Pts',(63.2559835201813,3.20104499537862,124.576066704985));
#231932=CARTESIAN_POINT('Ctrl Pts',(62.9775358963684,-3.5097970532309,124.744685810362));
#231933=CARTESIAN_POINT('Ctrl Pts',(62.6990882725555,-6.9953070730393,130.481850031987));
#231934=CARTESIAN_POINT('Ctrl Pts',(62.4206406487427,-4.05247163247362,
136.51538572624));
#231935=CARTESIAN_POINT('Ctrl Pts',(62.1421930249296,2.61438726408988,137.300768344709));
#231936=CARTESIAN_POINT('Ctrl Pts',(61.8637454011169,6.87875198487314,132.116269629093));
#231937=CARTESIAN_POINT('Ctrl Pts',(61.5852977773038,4.82187967727427,125.726190622201));
#231938=CARTESIAN_POINT('Ctrl Pts',(61.3068501534911,-1.66606449182178,
124.002701758653));
#231939=CARTESIAN_POINT('Ctrl Pts',(61.0284025296781,-6.62297678470872,
128.529605106938));
#231940=CARTESIAN_POINT('Ctrl Pts',(60.7499549058653,-5.49369696285183,
135.146897641504));
#231941=CARTESIAN_POINT('Ctrl Pts',(60.4715072820523,0.684021985849089,
137.773610795799));
#231942=CARTESIAN_POINT('Ctrl Pts',(60.1930596582395,6.23315814588628,133.995923503096));
#231943=CARTESIAN_POINT('Ctrl Pts',(59.9146120344266,6.05432647655821,127.285345835106));
#231944=CARTESIAN_POINT('Ctrl Pts',(59.6361644106137,0.311864545564345,
123.808570838767));
#231945=CARTESIAN_POINT('Ctrl Pts',(59.3577167868007,-5.71718566737322,
126.760584885814));
#231946=CARTESIAN_POINT('Ctrl Pts',(59.0792691629879,-6.49242155204172,
133.428631280914));
#231947=CARTESIAN_POINT('Ctrl Pts',(58.800821539175,-1.30143920280946,137.685101139145));
#231948=CARTESIAN_POINT('Ctrl Pts',(58.5223739153621,5.08550219496502,135.618506600908));
#231949=CARTESIAN_POINT('Ctrl Pts',(58.2439262915492,6.79911551616065,129.127947088084));
#231950=CARTESIAN_POINT('Ctrl Pts',(57.9654786677363,2.26467383326308,124.1779297115));
#231951=CARTESIAN_POINT('Ctrl Pts',(57.6870310439234,-4.35089246693584,
125.317278618444));
#231952=CARTESIAN_POINT('Ctrl Pts',(57.4085834201106,-6.96820114293417,
131.498987823723));
#231953=CARTESIAN_POINT('Ctrl Pts',(57.1301357962976,-3.18207338412696,
137.042368560968));
#231954=CARTESIAN_POINT('Ctrl Pts',(56.8516881724848,3.52822436176609,136.853324741857));
#231955=CARTESIAN_POINT('Ctrl Pts',(56.5732405486719,6.9962562825383,131.105578400848));
#231956=CARTESIAN_POINT('Ctrl Pts',(56.294792924859,4.03507046577855,125.081027632309));
#231957=CARTESIAN_POINT('Ctrl Pts',(56.0163453010462,-2.63414798488075,
124.315940276861));
#231958=CARTESIAN_POINT('Ctrl Pts',(55.7378976772331,-6.8827131227178,129.513394237565));
#231959=CARTESIAN_POINT('Ctrl Pts',(55.4594500534204,-4.80640114000575,
135.897183234276));
#231960=CARTESIAN_POINT('Ctrl Pts',(55.1810024296073,1.68675868462211,137.600917044446));
#231961=CARTESIAN_POINT('Ctrl Pts',(54.9025548057946,6.62986968082513,133.058947528554));
#231962=CARTESIAN_POINT('Ctrl Pts',(54.6241071819816,5.4804543274898,126.445122784157));
#231963=CARTESIAN_POINT('Ctrl Pts',(54.3456595581689,-0.705230817730614,
123.837224648055));
#231964=CARTESIAN_POINT('Ctrl Pts',(54.0672119343557,-6.24284329389726,
127.63178410442));
#231965=CARTESIAN_POINT('Ctrl Pts',(53.7887643105431,-6.04358776282204,
134.341786387386));
#231966=CARTESIAN_POINT('Ctrl Pts',(53.51031668673,-0.290570323389535,137.801067200743));
#231967=CARTESIAN_POINT('Ctrl Pts',(53.2318690629172,5.72946704808866,134.830716472279));
#231968=CARTESIAN_POINT('Ctrl Pts',(52.9534214391043,6.48440410239917,128.160341411752));
#231969=CARTESIAN_POINT('Ctrl Pts',(52.6749738152913,1.28049056735643,123.919690833848));
#231970=CARTESIAN_POINT('Ctrl Pts',(52.3965261914786,-5.10013124364513,
126.005715452363));
#231971=CARTESIAN_POINT('Ctrl Pts',(52.1180785676656,-6.79398159699943,
132.501460550851));
#231972=CARTESIAN_POINT('Ctrl Pts',(51.8396309438527,-2.24449476716385,
137.43765371859));
#231973=CARTESIAN_POINT('Ctrl Pts',(51.5611833200399,4.36757310402998,136.278174580871));
#231974=CARTESIAN_POINT('Ctrl Pts',(51.2827356962269,6.96605466042841,130.088527821552));
#231975=CARTESIAN_POINT('Ctrl Pts',(51.0042880724141,3.16307229458231,124.556696431394));
#231976=CARTESIAN_POINT('Ctrl Pts',(50.7258404486012,-3.54661898531293,
124.766163212963));
#231977=CARTESIAN_POINT('Ctrl Pts',(50.4473928247883,-6.99714067967511,
130.52443842702));
#231978=CARTESIAN_POINT('Ctrl Pts',(50.1689452009753,-4.0176319187415,136.539948459229));
#231979=CARTESIAN_POINT('Ctrl Pts',(49.8904975771625,2.65388430328469,137.284733463992));
#231980=CARTESIAN_POINT('Ctrl Pts',(49.6120499533496,6.88661050004828,132.074372406703));
#231981=CARTESIAN_POINT('Ctrl Pts',(49.3336023295367,4.79087807689359,125.696932558722));
#231982=CARTESIAN_POINT('Ctrl Pts',(49.0551547057238,-1.7074372515208,124.012969585086));
#231983=CARTESIAN_POINT('Ctrl Pts',(48.776707081911,-6.63670115873435,128.569963192402));
#231984=CARTESIAN_POINT('Ctrl Pts',(48.498259458098,-5.46716092194746,135.180258877061));
#231985=CARTESIAN_POINT('Ctrl Pts',(48.2198118342852,0.72643311645002,137.769317835757));
#231986=CARTESIAN_POINT('Ctrl Pts',(47.9413642104722,6.25247060906043,133.957921368012));
#231987=CARTESIAN_POINT('Ctrl Pts',(47.6629165866595,6.03279306211481,127.248556630613));
#231988=CARTESIAN_POINT('Ctrl Pts',(47.3844689628464,0.269273409411107,
123.806802046542));
#231989=CARTESIAN_POINT('Ctrl Pts',(47.1060213390337,-5.74169535180415,
126.7954619395));
#231990=CARTESIAN_POINT('Ctrl Pts',(46.8275737152206,-6.47632658212296,
133.468103872012));
#231991=CARTESIAN_POINT('Ctrl Pts',(46.5491260914079,-1.25953006961336,
137.69289588478));
#231992=CARTESIAN_POINT('Ctrl Pts',(46.2706784675948,5.11471304540623,135.587460510634));
#231993=CARTESIAN_POINT('Ctrl Pts',(45.9922308437821,6.78878473932087,129.086590002178));
#231994=CARTESIAN_POINT('Ctrl Pts',(45.7137832199691,2.22429490837156,124.164266771503));
#231995=CARTESIAN_POINT('Ctrl Pts',(45.4353355961562,-4.38421328052394,
125.343865398741));
#231996=CARTESIAN_POINT('Ctrl Pts',(45.1568879723434,-6.96384364534361,
131.541392372057));
#231997=CARTESIAN_POINT('Ctrl Pts',(44.8784403485304,-3.1440419027679,137.061623168999));
#231998=CARTESIAN_POINT('Ctrl Pts',(44.5999927247176,3.56498075346585,136.831735365442));
#231999=CARTESIAN_POINT('Ctrl Pts',(44.3215451009046,6.99796025625624,131.062984622213));
#232000=CARTESIAN_POINT('Ctrl Pts',(44.0430974770918,4.00015615291162,125.056571053198));
#232001=CARTESIAN_POINT('Ctrl Pts',(43.7646498532789,-2.67359603646683,
124.332095298706));
#232002=CARTESIAN_POINT('Ctrl Pts',(43.486202229466,-6.8904440807599,129.555315184507));
#232003=CARTESIAN_POINT('Ctrl Pts',(43.2077546056531,-4.77531063174146,
135.926346804027));
#232004=CARTESIAN_POINT('Ctrl Pts',(42.9293069818402,1.72810000095366,137.590523341125));
#232005=CARTESIAN_POINT('Ctrl Pts',(42.6508593580274,6.64347115515083,133.018547857752));
#232006=CARTESIAN_POINT('Ctrl Pts',(42.3724117342144,5.4538168693733,126.411842469708));
#232007=CARTESIAN_POINT('Ctrl Pts',(42.0939641104015,-0.74762868559244,
123.841646673103));
#232008=CARTESIAN_POINT('Ctrl Pts',(41.8155164865887,-6.26204000219037,
127.669844843974));
#232009=CARTESIAN_POINT('Ctrl Pts',(41.5370688627757,-6.02194247443641,
134.378509881167));
#232010=CARTESIAN_POINT('Ctrl Pts',(41.2586212389629,-0.247974000920424,
137.802706352008));
#232011=CARTESIAN_POINT('Ctrl Pts',(40.9801736151499,5.75387046523817,134.795764981093));
#232012=CARTESIAN_POINT('Ctrl Pts',(40.7017259913371,6.46818906604193,128.120917991039));
#232013=CARTESIAN_POINT('Ctrl Pts',(40.4232783675241,1.23855790375582,123.912023681303));
#232014=CARTESIAN_POINT('Ctrl Pts',(40.1448307437113,-5.12924746516435,
126.036850306614));
#232015=CARTESIAN_POINT('Ctrl Pts',(39.8663831198984,-6.78352499126783,
132.542786001862));
#232016=CARTESIAN_POINT('Ctrl Pts',(39.5879354960856,-2.20407444401526,
137.451193695743));
#232017=CARTESIAN_POINT('Ctrl Pts',(39.3094878722726,4.40081284226458,136.251486506627));
#232018=CARTESIAN_POINT('Ctrl Pts',(39.0310402484598,6.96156811816289,130.046136732356));
#232019=CARTESIAN_POINT('Ctrl Pts',(38.7525926246468,3.12498238497894,124.537557667297));
#232020=CARTESIAN_POINT('Ctrl Pts',(38.474145000834,-3.58330949612422,124.78786436319));
#232021=CARTESIAN_POINT('Ctrl Pts',(38.195697377021,-6.9987150046898,130.567037194673));
#232022=CARTESIAN_POINT('Ctrl Pts',(37.9172497532082,-3.98264333018119,
136.564298657899));
#232023=CARTESIAN_POINT('Ctrl Pts',(37.6388021293952,2.69328300182069,137.268458450676));
#232024=CARTESIAN_POINT('Ctrl Pts',(37.3603545055824,6.89421382933879,132.032428123559));
#232025=CARTESIAN_POINT('Ctrl Pts',(37.0819068817695,4.7596989487639,125.667863752866));
#232026=CARTESIAN_POINT('Ctrl Pts',(36.8034592579566,-1.74874674150458,
124.02348906901));
#232027=CARTESIAN_POINT('Ctrl Pts',(36.5250116341437,-6.65017960735793,
128.610404074285));
#232028=CARTESIAN_POINT('Ctrl Pts',(36.2465640103308,-5.44042229338459,
135.213457962098));
#232029=CARTESIAN_POINT('Ctrl Pts',(35.968116386518,0.768817328804687,137.764766786667));
#232030=CARTESIAN_POINT('Ctrl Pts',(35.689668762705,6.27155138463682,133.919802376575));
#232031=CARTESIAN_POINT('Ctrl Pts',(35.4112211388921,6.01103610030595,127.211899187745));
#232032=CARTESIAN_POINT('Ctrl Pts',(35.1327735150793,0.226672295232647,
123.805292551423));
#232033=CARTESIAN_POINT('Ctrl Pts',(34.8543258912663,-5.76599227560232,
126.830487544402));
#232034=CARTESIAN_POINT('Ctrl Pts',(34.5758782674535,-6.45999162954105,
133.507477757125));
#232035=CARTESIAN_POINT('Ctrl Pts',(34.2974306436406,-1.21757426406734,
137.700435373207));
#232036=CARTESIAN_POINT('Ctrl Pts',(34.0189830198277,5.1437343682746,135.556237180835));
#232037=CARTESIAN_POINT('Ctrl Pts',(33.7405353960148,6.778202401566,129.045296568894));
#232038=CARTESIAN_POINT('Ctrl Pts',(33.4620877722019,2.18383356141425,124.150849882625));
#232039=CARTESIAN_POINT('Ctrl Pts',(33.1836401483891,-4.41737163547663,
125.370654519698));
#232040=CARTESIAN_POINT('Ctrl Pts',(32.9051925245761,-6.95922809996586,
131.58376960941));
#232041=CARTESIAN_POINT('Ctrl Pts',(32.6267449007632,-3.10589391777991,
137.080645911863));
#232042=CARTESIAN_POINT('Ctrl Pts',(32.3482972769504,3.60160504349277,136.80992264244));
#232043=CARTESIAN_POINT('Ctrl Pts',(32.0698496531375,6.99940491798352,131.020381260171));
#232044=CARTESIAN_POINT('Ctrl Pts',(31.7914020293246,3.96509361278713,125.032327460544));
#232045=CARTESIAN_POINT('Ctrl Pts',(31.5129544055117,-2.71294501696876,
124.348490152723));
#232046=CARTESIAN_POINT('Ctrl Pts',(31.2345067816988,-6.89791971086261,
129.597282415287));
#232047=CARTESIAN_POINT('Ctrl Pts',(30.9560591578859,-4.74404317258561,
135.955320576696));
#232048=CARTESIAN_POINT('Ctrl Pts',(30.677611534073,1.76937728190418,137.579878174048));
#232049=CARTESIAN_POINT('Ctrl Pts',(30.3991639102601,6.65682645320975,132.978066139427));
#232050=CARTESIAN_POINT('Ctrl Pts',(30.1207162864473,5.42697731806706,126.378724921634));
#232051=CARTESIAN_POINT('Ctrl Pts',(29.8422686626343,-0.789998849798377,
123.846326704078));
#232052=CARTESIAN_POINT('Ctrl Pts',(29.5638210388214,-6.28100466828836,
127.708021734164));
#232053=CARTESIAN_POINT('Ctrl Pts',(29.2853734150086,-6.00007404075783,
134.415100933532));
#232054=CARTESIAN_POINT('Ctrl Pts',(29.0069257911957,-0.205368489683527,
137.804086176998));
#232055=CARTESIAN_POINT('Ctrl Pts',(28.7284781673828,5.77806067060162,134.760665586949));
#232056=CARTESIAN_POINT('Ctrl Pts',(28.4500305435699,6.45173434856014,128.08159400628));
#232057=CARTESIAN_POINT('Ctrl Pts',(28.171582919757,1.19657934493693,123.904611926838));
#232058=CARTESIAN_POINT('Ctrl Pts',(27.8931352959441,-5.15817362053239,
126.068161822712));
#232059=CARTESIAN_POINT('Ctrl Pts',(27.6146876721312,-6.77281701952304,
132.584047034882));
#232060=CARTESIAN_POINT('Ctrl Pts',(27.3362400483183,-2.16357244807759,
137.464487372053));
#232061=CARTESIAN_POINT('Ctrl Pts',(27.0577924245054,4.4338895067609,136.22459658713));
#232062=CARTESIAN_POINT('Ctrl Pts',(26.7793448006925,6.95682361243065,130.003773739425));
#232063=CARTESIAN_POINT('Ctrl Pts',(26.5008971768797,3.08677667800406,124.518651121888));
#232064=CARTESIAN_POINT('Ctrl Pts',(26.2224495530668,-3.61986722608435,
124.809788456898));
#232065=CARTESIAN_POINT('Ctrl Pts',(25.9440019292538,-7.00002998974624,
130.609644756432));
#232066=CARTESIAN_POINT('Ctrl Pts',(25.665554305441,-3.94750716330764,136.588435419948));
#232067=CARTESIAN_POINT('Ctrl Pts',(25.3871066816281,2.7325818997646,137.251943907838));
#232068=CARTESIAN_POINT('Ctrl Pts',(25.1086590578152,6.90156169100052,131.990438333922));
#232069=CARTESIAN_POINT('Ctrl Pts',(24.8302114340022,4.72834344823931,125.638985281792));
#232070=CARTESIAN_POINT('Ctrl Pts',(24.5517638101894,-1.78999143103474,
124.034259820624));
#232071=CARTESIAN_POINT('Ctrl Pts',(24.2733161863765,-6.66341163113055,
128.650926254035));
#232072=CARTESIAN_POINT('Ctrl Pts',(23.9948685625636,-5.41348206797292,
135.246493666413));
#232073=CARTESIAN_POINT('Ctrl Pts',(23.7164209387507,0.811173052350488,
137.759957817164));
#232074=CARTESIAN_POINT('Ctrl Pts',(23.4379733149379,6.29039976557031,133.881567941299));
#232075=CARTESIAN_POINT('Ctrl Pts',(23.159525691125,5.98905639734383,127.175374864857));
#232076=CARTESIAN_POINT('Ctrl Pts',(22.8810780673121,0.184062781628937,
123.804042409345));
#232077=CARTESIAN_POINT('Ctrl Pts',(22.6026304434992,-5.79007553843628,
126.865660402631));
#232078=CARTESIAN_POINT('Ctrl Pts',(22.3241828196863,-6.44341729959363,
133.546751477239));
#232079=CARTESIAN_POINT('Ctrl Pts',(22.0457351958734,-1.17557334085921,
137.707719325048));
#232080=CARTESIAN_POINT('Ctrl Pts',(21.7672875720605,5.17256508817436,135.524837768503));
#232081=CARTESIAN_POINT('Ctrl Pts',(21.4888399482477,6.76736889502847,129.004068318375));
#232082=CARTESIAN_POINT('Ctrl Pts',(21.2103923244347,2.14329129170119,124.137679542035));
#232083=CARTESIAN_POINT('Ctrl Pts',(20.9319447006219,-4.45036630309889,
125.397644988631));
#232084=CARTESIAN_POINT('Ctrl Pts',(20.6534970768089,-6.95435467783159,
131.626117965476));
#232085=CARTESIAN_POINT('Ctrl Pts',(20.3750494529961,-3.06763084275059,
137.099436084669));
#232086=CARTESIAN_POINT('Ctrl Pts',(20.0966018291831,3.6380958747203,136.787887381128));
#232087=CARTESIAN_POINT('Ctrl Pts',(19.8181542053702,7.00059021418742,130.977769893405));
#232088=CARTESIAN_POINT('Ctrl Pts',(19.5397065815574,3.92988414466092,125.0082977527));
#232089=CARTESIAN_POINT('Ctrl Pts',(19.2612589577445,-2.75219346829522,
124.365124231394));
#232090=CARTESIAN_POINT('Ctrl Pts',(18.9828113339316,-6.90513973601376,
129.639294374793));
#232091=CARTESIAN_POINT('Ctrl Pts',(18.7043637101187,-4.71259992116536,
135.98410347865));
#232092=CARTESIAN_POINT('Ctrl Pts',(18.4259160863058,1.81058899792882,137.568981937677));
#232093=CARTESIAN_POINT('Ctrl Pts',(18.1474684624929,6.6699350801164,132.937503873645));
#232094=CARTESIAN_POINT('Ctrl Pts',(17.86902083868,5.39993666812053,126.345771367118));
#232095=CARTESIAN_POINT('Ctrl Pts',(17.5905732148672,-0.832339740306418,
123.851264567558));
#232096=CARTESIAN_POINT('Ctrl Pts',(17.3121255910542,-6.29973658944851,
127.746313360329));
#232097=CARTESIAN_POINT('Ctrl Pts',(17.0336779672413,-5.97798327212915,
134.451558188587));
#232098=CARTESIAN_POINT('Ctrl Pts',(16.7552303434285,-0.162755368441711,
137.805206624583));
#232099=CARTESIAN_POINT('Ctrl Pts',(16.4767827196156,5.80203676780203,134.72541959047));
#232100=CARTESIAN_POINT('Ctrl Pts',(16.1983350958026,6.43504055968944,128.042370914639));
#232101=CARTESIAN_POINT('Ctrl Pts',(15.9198874719898,1.15455644643036,123.897455845098));
#232102=CARTESIAN_POINT('Ctrl Pts',(15.6414398481769,-5.18690863788001,
126.0996488404));
#232103=CARTESIAN_POINT('Ctrl Pts',(15.362992224364,-6.7618580785529,132.625242120967));
#232104=CARTESIAN_POINT('Ctrl Pts',(15.0845446005511,-2.12299028016722,
137.477534254917));
#232105=CARTESIAN_POINT('Ctrl Pts',(14.8060969767383,4.466801871851,136.197505818795));
#232106=CARTESIAN_POINT('Ctrl Pts',(14.5276493529253,6.95182131904109,129.961440412534));
#232107=CARTESIAN_POINT('Ctrl Pts',(14.2492017291125,3.04845658938423,124.499977495755));
#232108=CARTESIAN_POINT('Ctrl Pts',(13.9707541052995,-3.65629082053323,
124.831934681683));
#232109=CARTESIAN_POINT('Ctrl Pts',(13.6923064814867,-7.00108558611715,
130.652259533458));
#232110=CARTESIAN_POINT('Ctrl Pts',(13.4138588576738,-3.91222472010448,
136.612357850978));
#232111=CARTESIAN_POINT('Ctrl Pts',(13.1354112338608,2.77177954088132,137.23519044743));
#232112=CARTESIAN_POINT('Ctrl Pts',(12.856963610048,6.90865381275575,131.94840459374));
#232113=CARTESIAN_POINT('Ctrl Pts',(12.5785159862351,4.6968127372094,125.6102982156));
#232114=CARTESIAN_POINT('Ctrl Pts',(12.3000683624222,-1.83116979177416,
124.045281440813));
#232115=CARTESIAN_POINT('Ctrl Pts',(12.0216207386093,-6.67639673973472,
128.691528230086));
#232116=CARTESIAN_POINT('Ctrl Pts',(11.7431731147965,-5.38634124399241,
135.279364765853));
#232117=CARTESIAN_POINT('Ctrl Pts',(11.4647254909835,0.853498717580522,
137.75489110545));
#232118=CARTESIAN_POINT('Ctrl Pts',(11.1862778671706,6.30901505342741,133.843219478972));
#232119=CARTESIAN_POINT('Ctrl Pts',(10.9078302433578,5.96685476769427,127.13898501537));
#232120=CARTESIAN_POINT('Ctrl Pts',(10.6293826195448,0.141446447510913,
123.803051666633));
#232121=CARTESIAN_POINT('Ctrl Pts',(10.350934995732,-5.81394424789186,126.900979210845));
#232122=CARTESIAN_POINT('Ctrl Pts',(10.0724873719191,-6.42660420644864,
133.585923577051));
#232123=CARTESIAN_POINT('Ctrl Pts',(9.79403974810624,-1.1335288563486,137.714747470394));
#232124=CARTESIAN_POINT('Ctrl Pts',(9.51559212429333,5.20120413677258,135.493263437154));
#232125=CARTESIAN_POINT('Ctrl Pts',(9.23714450048043,6.75628462114785,128.962906778349));
#232126=CARTESIAN_POINT('Ctrl Pts',(8.95869687666756,2.10266960154115,124.124756237763));
#232127=CARTESIAN_POINT('Ctrl Pts',(8.68024925285465,-4.48319606076117,
125.4248358054));
#232128=CARTESIAN_POINT('Ctrl Pts',(8.40180162904178,-6.94922355952728,
131.66843587102));
#232129=CARTESIAN_POINT('Ctrl Pts',(8.12335400522884,-3.0292540955323,137.117992991138));
#232130=CARTESIAN_POINT('Ctrl Pts',(7.84490638141603,3.67445189496732,136.765630398031));
#232131=CARTESIAN_POINT('Ctrl Pts',(7.56645875760307,7.00151610094645,130.935152100895));
#232132=CARTESIAN_POINT('Ctrl Pts',(7.2880111337902,3.89452905323253,124.984482820099));
#232133=CARTESIAN_POINT('Ctrl Pts',(7.00956350997733,-2.79133993608059,
124.381996918337));
#232134=CARTESIAN_POINT('Ctrl Pts',(6.73111588616443,-6.91210388867261,
129.681349506257));
#232135=CARTESIAN_POINT('Ctrl Pts',(6.45266826235151,-4.68098204262199,
136.012694443327));
#232136=CARTESIAN_POINT('Ctrl Pts',(6.17422063853866,1.85173362191231,137.557835035774));
#232137=CARTESIAN_POINT('Ctrl Pts',(5.89577301472578,6.68279655012581,132.896862563455));
#232138=CARTESIAN_POINT('Ctrl Pts',(5.61732539091285,5.37269592153495,126.312983027266));
#232139=CARTESIAN_POINT('Ctrl Pts',(5.33887776709996,-0.874649788159289,
123.856460080569));
#232140=CARTESIAN_POINT('Ctrl Pts',(5.06043014328709,-6.31823507155263,
127.784718303561));
#232141=CARTESIAN_POINT('Ctrl Pts',(4.7819825194742,-5.95567098713191,134.487880295395));
#232142=CARTESIAN_POINT('Ctrl Pts',(4.50353489566127,-0.120136216239877,
137.806067653244));
#232143=CARTESIAN_POINT('Ctrl Pts',(4.22508727184843,5.82579786839633,134.690028297709));
#232144=CARTESIAN_POINT('Ctrl Pts',(3.94663964803551,6.41810831802433,128.003250169541));
#232145=CARTESIAN_POINT('Ctrl Pts',(3.66819202422262,1.11249076541009,123.890555701254));
#232146=CARTESIAN_POINT('Ctrl Pts',(3.3897444004097,-5.21545145242058,126.131310192911));
#232147=CARTESIAN_POINT('Ctrl Pts',(3.11129677659686,-6.75064857444498,
132.666369733619));
#232148=CARTESIAN_POINT('Ctrl Pts',(2.83284915278395,-2.08232944407128,
137.490333860877));
#232149=CARTESIAN_POINT('Ctrl Pts',(2.55440152897106,4.49954871795507,136.170215205482));
#232150=CARTESIAN_POINT('Ctrl Pts',(2.27595390515816,6.94656142335602,129.919138320362));
#232151=CARTESIAN_POINT('Ctrl Pts',(1.9975062813453,3.01002353908442,124.481537480858));
#232152=CARTESIAN_POINT('Ctrl Pts',(1.71905865753238,-3.69257892978116,
124.854302216906));
#232153=CARTESIAN_POINT('Ctrl Pts',(1.44061103371947,-7.00188175468703,
130.694879946647));
#232154=CARTESIAN_POINT('Ctrl Pts',(1.16216340990662,-3.87679730797559,
136.636065064534));
#232155=CARTESIAN_POINT('Ctrl Pts',(0.883715786093727,2.81087447268782,
137.218198690258));
#232156=CARTESIAN_POINT('Ctrl Pts',(0.605268162280799,6.91548993180329,
131.906328460586));
#232157=CARTESIAN_POINT('Ctrl Pts',(0.326820538467947,4.66510798405627,
125.5818036173));
#232158=CARTESIAN_POINT('Ctrl Pts',(0.0483729146550416,-1.87228029784353,
124.056553521165));
#232159=CARTESIAN_POINT('Ctrl Pts',(-0.23007470915786,-6.68913445200245,
128.732208497919));
#232160=CARTESIAN_POINT('Ctrl Pts',(-0.508522332970751,-5.35900082715629,
135.312070042369));
#232161=CARTESIAN_POINT('Ctrl Pts',(-0.786969956783612,0.895792756101716,
137.749566839272));
#232162=CARTESIAN_POINT('Ctrl Pts',(-1.06541758059653,6.32739655841135,
133.804758410613));
#232163=CARTESIAN_POINT('Ctrl Pts',(-1.34386520440944,5.94443203404716,
127.102730987725));
#232164=CARTESIAN_POINT('Ctrl Pts',(-1.62231282822229,0.0988248720430084,
123.802320359999));
#232165=CARTESIAN_POINT('Ctrl Pts',(-1.90076045203519,-5.83759751950527,
126.936442660293));
#232166=CARTESIAN_POINT('Ctrl Pts',(-2.17920807584809,-6.40955297312139,
133.624992605024));
#232167=CARTESIAN_POINT('Ctrl Pts',(-2.45765569966099,-1.09144236850938,
137.721519548813));
#232168=CARTESIAN_POINT('Ctrl Pts',(-2.73610332347384,5.22965045283876,
135.461515356786));
#232169=CARTESIAN_POINT('Ctrl Pts',(-3.01455094728676,6.74494999065597,
128.921813474073));
#232170=CARTESIAN_POINT('Ctrl Pts',(-3.29299857109967,2.06196999618574,
124.112080448687));
#232171=CARTESIAN_POINT('Ctrl Pts',(-3.57144619491253,-4.51585969194472,
125.452225962441));
#232172=CARTESIAN_POINT('Ctrl Pts',(-3.84989381872542,-6.94383493518842,
131.710721757939));
#232173=CARTESIAN_POINT('Ctrl Pts',(-4.12834144253832,-2.99076509818949,
137.136315943637));
#232174=CARTESIAN_POINT('Ctrl Pts',(-4.40678906635123,3.71067175704807,
136.743152517891));
#232175=CARTESIAN_POINT('Ctrl Pts',(-4.68523669016409,7.00218254395157,
130.892529461858));
#232176=CARTESIAN_POINT('Ctrl Pts',(-4.963684313977,3.85902964859785,124.960883545208));
#232177=CARTESIAN_POINT('Ctrl Pts',(-5.24213193778992,-2.83038296973812,
124.399107588329));
#232178=CARTESIAN_POINT('Ctrl Pts',(-5.52057956160276,-6.91881191077996,
129.723446251312));
#232179=CARTESIAN_POINT('Ctrl Pts',(-5.79902718541567,-4.6491907085676,
136.041092411279));
#232180=CARTESIAN_POINT('Ctrl Pts',(-6.07747480922856,1.89280962922548,
137.546437881394));
#232181=CARTESIAN_POINT('Ctrl Pts',(-6.35592243304147,6.69541038665145,
132.856143714835));
#232182=CARTESIAN_POINT('Ctrl Pts',(-6.63437005685431,5.34525608772619,
126.280361117063));
#232183=CARTESIAN_POINT('Ctrl Pts',(-6.91281768066725,-0.916927425542613,
123.86191305059));
#232184=CARTESIAN_POINT('Ctrl Pts',(-7.19126530448013,-6.33649942913263,
127.823235140749));
#232185=CARTESIAN_POINT('Ctrl Pts',(-7.469712928293,-5.93313801255607,134.524065908027));
#232186=CARTESIAN_POINT('Ctrl Pts',(-7.74816055210589,-0.0775126123463511,
137.806669231077));
#232187=CARTESIAN_POINT('Ctrl Pts',(-8.02660817591882,5.84934309190818,
134.654493020103));
#232188=CARTESIAN_POINT('Ctrl Pts',(-8.3050557997317,6.40093825099524,127.964233220621));
#232189=CARTESIAN_POINT('Ctrl Pts',(-8.58350342354456,1.07038386063539,
123.883911750995));
#232190=CARTESIAN_POINT('Ctrl Pts',(-8.86195104735747,-5.2438010064896,
126.163144707024));
#232191=CARTESIAN_POINT('Ctrl Pts',(-9.14039867117038,-6.73918892257159,
132.707428348838));
#232192=CARTESIAN_POINT('Ctrl Pts',(-9.41884629498326,-2.04159144649203,
137.50288571564));
#232193=CARTESIAN_POINT('Ctrl Pts',(-9.69729391879612,4.53212883162697,
136.142725758454));
#232194=CARTESIAN_POINT('Ctrl Pts',(-9.97574154260907,6.94104412028278,
129.876869030427));
#232195=CARTESIAN_POINT('Ctrl Pts',(-10.254189166422,2.97147895125515,124.463331760497));
#232196=CARTESIAN_POINT('Ctrl Pts',(-10.5326367902348,-3.72873020915888,
124.876890233732));
#232197=CARTESIAN_POINT('Ctrl Pts',(-10.8110844140478,-7.00241846595355,
130.737504416682));
#232198=CARTESIAN_POINT('Ctrl Pts',(-11.0895320378606,-3.84122623969676,
136.659556182137));
#232199=CARTESIAN_POINT('Ctrl Pts',(-11.3679796616735,2.84986524650705,
137.200969265957));
#232200=CARTESIAN_POINT('Ctrl Pts',(-11.6464272854864,6.92206979482823,
131.864211493609));
#232201=CARTESIAN_POINT('Ctrl Pts',(-11.9248749092993,4.6332303636112,125.553502542771));
#232202=CARTESIAN_POINT('Ctrl Pts',(-12.2033225331122,-1.91332142587795,
124.068075643991));
#232203=CARTESIAN_POINT('Ctrl Pts',(-12.4817701569251,-6.70162429593314,
128.77296555011));
#232204=CARTESIAN_POINT('Ctrl Pts',(-12.760217780738,-5.33146183057377,
135.344608284054));
#232205=CARTESIAN_POINT('Ctrl Pts',(-13.0386654045509,0.938053600692905,
137.743985215925));
#232206=CARTESIAN_POINT('Ctrl Pts',(-13.3171130283637,6.34554359938892,
133.766186161411));
#232207=CARTESIAN_POINT('Ctrl Pts',(-13.5955606521767,5.92178902728497,
127.066614125326));
#232208=CARTESIAN_POINT('Ctrl Pts',(-13.8740082759896,0.0561996345831295,
123.801848516541));
#232209=CARTESIAN_POINT('Ctrl Pts',(-14.1524558998025,-5.86103447679583,
126.972049436864));
#232210=CARTESIAN_POINT('Ctrl Pts',(-14.4309035236153,-6.39226423145161,
133.663957113442));
#232211=CARTESIAN_POINT('Ctrl Pts',(-14.7093511474282,-1.04931543687181,
137.728035309365));
#232212=CARTESIAN_POINT('Ctrl Pts',(-14.9877987712411,5.25790298228423,
135.429594703837));
#232213=CARTESIAN_POINT('Ctrl Pts',(-15.266246395054,6.73336542356173,128.880789928272));
#232214=CARTESIAN_POINT('Ctrl Pts',(-15.5446940188669,2.02119398377386,
124.099652644515));
#232215=CARTESIAN_POINT('Ctrl Pts',(-15.8231416426798,-4.54835598628669,
125.479814444798));
#232216=CARTESIAN_POINT('Ctrl Pts',(-16.1015892664927,-6.93818900449243,
131.752974059312));
#232217=CARTESIAN_POINT('Ctrl Pts',(-16.3800368903055,-2.95216527694612,
137.154404263204));
#232218=CARTESIAN_POINT('Ctrl Pts',(-16.6584845141185,3.74675411882228,
136.720454573632));
#232219=CARTESIAN_POINT('Ctrl Pts',(-16.9369321379314,7.00258951850748,
130.849903555692));
#232220=CARTESIAN_POINT('Ctrl Pts',(-17.2153797617442,3.82338724620039,
124.93750080251));
#232221=CARTESIAN_POINT('Ctrl Pts',(-17.4938273855571,-2.86932112251383,
124.416455607327));
#232222=CARTESIAN_POINT('Ctrl Pts',(-17.77227500937,-6.92526355376757,129.765583050046));
#232223=CARTESIAN_POINT('Ctrl Pts',(-18.0507226331829,-4.61722709704176,
136.069296330209));
#232224=CARTESIAN_POINT('Ctrl Pts',(-18.3291702569958,1.93381549778173,
137.534790896862));
#232225=CARTESIAN_POINT('Ctrl Pts',(-18.6076178808087,6.70777612228299,
132.81534883664));
#232226=CARTESIAN_POINT('Ctrl Pts',(-18.8860655046216,5.31761818348739,
126.247906845325));
#232227=CARTESIAN_POINT('Ctrl Pts',(-19.1645131284344,-0.959171085842972,
123.867623275557));
#232228=CARTESIAN_POINT('Ctrl Pts',(-19.4429607522474,-6.35452898539608,
127.861862444637));
#232229=CARTESIAN_POINT('Ctrl Pts',(-19.7214083760603,-5.91038518336925,
134.560113685611));
#232230=CARTESIAN_POINT('Ctrl Pts',(-19.9998559998732,-0.0348861361944895,
137.807011335788));
#232231=CARTESIAN_POINT('Ctrl Pts',(-20.278303623686,5.87267156586067,134.618815074426));
#232232=CARTESIAN_POINT('Ctrl Pts',(-20.5567512474989,6.38353099484532,
127.925321513668));
#232233=CARTESIAN_POINT('Ctrl Pts',(-20.8351988713118,1.02823729239309,
123.877524240513));
#232234=CARTESIAN_POINT('Ctrl Pts',(-21.1136464951247,-5.27195624958391,
126.1951512031));
#232235=CARTESIAN_POINT('Ctrl Pts',(-21.3920941189376,-6.72747954757436,
132.748416445183));
#232236=CARTESIAN_POINT('Ctrl Pts',(-21.6705417427505,-2.00077779699093,
137.515189354092));
#232237=CARTESIAN_POINT('Ctrl Pts',(-21.9489893665634,4.56454100559805,
136.115038496344));
#232238=CARTESIAN_POINT('Ctrl Pts',(-22.2274369903762,6.93526961426714,
129.834634109035));
#232239=CARTESIAN_POINT('Ctrl Pts',(-22.5058846141892,2.93282425418085,
124.445361009293));
#232240=CARTESIAN_POINT('Ctrl Pts',(-22.784332238002,-3.76474331906749,
124.899697895151));
#232241=CARTESIAN_POINT('Ctrl Pts',(-23.062779861815,-7.0026957000287,130.780131364099));
#232242=CARTESIAN_POINT('Ctrl Pts',(-23.3412274856278,-3.80551283336702,
136.682830333316));
#232243=CARTESIAN_POINT('Ctrl Pts',(-23.6196751094408,2.88875041752152,
137.183502812971));
#232244=CARTESIAN_POINT('Ctrl Pts',(-23.8981227332536,6.92839315801137,
131.822055253468));
#232245=CARTESIAN_POINT('Ctrl Pts',(-24.1765703570665,4.60118105711114,
125.525396040718));
#232246=CARTESIAN_POINT('Ctrl Pts',(-24.4550179808794,-1.95429165508329,
124.079847382335));
#232247=CARTESIAN_POINT('Ctrl Pts',(-24.7334656046923,-6.71386580871103,
128.813797876394));
#232248=CARTESIAN_POINT('Ctrl Pts',(-25.0119132285052,-5.30372527471246,
135.376978285193));
#232249=CARTESIAN_POINT('Ctrl Pts',(-25.290360852318,0.980279685362951,
137.738146442235));
#232250=CARTESIAN_POINT('Ctrl Pts',(-25.568808476131,6.36345550391485,133.727504160674));
#232251=CARTESIAN_POINT('Ctrl Pts',(-25.8472560999438,5.89892658645264,
127.030635766497));
#232252=CARTESIAN_POINT('Ctrl Pts',(-26.1257037237567,0.0135723146251221,
123.801636153745));
#232253=CARTESIAN_POINT('Ctrl Pts',(-26.4041513475696,-5.88425425129846,
127.007798221134));
#232254=CARTESIAN_POINT('Ctrl Pts',(-26.6825989713826,-6.37473862207999,
133.70281565846));
#232255=CARTESIAN_POINT('Ctrl Pts',(-26.9610465951954,-1.00714962246484,
137.734294510605));
#232256=CARTESIAN_POINT('Ctrl Pts',(-27.2394942190083,5.28596067820108,
135.397502661138));
#232257=CARTESIAN_POINT('Ctrl Pts',(-27.5179418428212,6.72153134913555,
128.839837661092));
#232258=CARTESIAN_POINT('Ctrl Pts',(-27.7963894666341,1.98034307527561,
124.087473285763));
#232259=CARTESIAN_POINT('Ctrl Pts',(-28.0748370904469,-4.58068373962494,
125.507600230172));
#232260=CARTESIAN_POINT('Ctrl Pts',(-28.3532847142599,-6.93228597665136,
131.795191209466));
#232261=CARTESIAN_POINT('Ctrl Pts',(-28.6317323380727,-2.91345606213275,
137.172257279568));
#232262=CARTESIAN_POINT('Ctrl Pts',(-28.9101799618857,3.78269764324474,
136.697537406337));
#232263=CARTESIAN_POINT('Ctrl Pts',(-29.1886275856985,7.00273700953358,
130.807275961916));
#232264=CARTESIAN_POINT('Ctrl Pts',(-29.4670752095115,3.78760316678249,
124.914335458459));
#232265=CARTESIAN_POINT('Ctrl Pts',(-29.7455228333243,-2.90815295154017,
124.434040332496));
#232266=CARTESIAN_POINT('Ctrl Pts',(-30.0239704571372,-6.93145857856742,
129.807758341064));
#232267=CARTESIAN_POINT('Ctrl Pts',(-30.3024180809501,-4.5850923924679,
136.097305155009));
#232268=CARTESIAN_POINT('Ctrl Pts',(-30.580865704763,1.97474970809384,137.52289451376));
#232269=CARTESIAN_POINT('Ctrl Pts',(-30.8593133285759,6.71989329880362,
132.774479440534));
#232270=CARTESIAN_POINT('Ctrl Pts',(-31.1377609523888,5.28978323295099,
126.215621414657));
#232271=CARTESIAN_POINT('Ctrl Pts',(-31.4162085762017,-1.00137920370602,
123.873590543879));
#232272=CARTESIAN_POINT('Ctrl Pts',(-31.6946562000146,-6.37232307225107,
127.900598783877));
#232273=CARTESIAN_POINT('Ctrl Pts',(-31.9731038238274,-5.88741334268594,
134.596022292384));
#232274=CARTESIAN_POINT('Ctrl Pts',(-32.2515514476404,0.00774163267598956,
137.807093954702));
#232275=CARTESIAN_POINT('Ctrl Pts',(-32.5299990714533,5.89578242580862,
134.582995782735));
#232276=CARTESIAN_POINT('Ctrl Pts',(-32.8084466952661,6.36588719460685,
127.886516490566));
#232277=CARTESIAN_POINT('Ctrl Pts',(-33.086894319079,0.9860526224398,123.8713934065));
#232278=CARTESIAN_POINT('Ctrl Pts',(-33.365341942892,-5.29991613840065,
126.227328495126));
#232279=CARTESIAN_POINT('Ctrl Pts',(-33.6437895667048,-6.71552088334846,
132.789332503824));
#232280=CARTESIAN_POINT('Ctrl Pts',(-33.9222371905177,-1.95989000793276,
137.527244320318));
#232281=CARTESIAN_POINT('Ctrl Pts',(-34.2006848143306,4.59678403882356,
136.08715444511));
#232282=CARTESIAN_POINT('Ctrl Pts',(-34.4791324381435,6.9292381192855,129.792435121214));
#232283=CARTESIAN_POINT('Ctrl Pts',(-34.7575800619564,2.89406088022529,
124.427625893158));
#232284=CARTESIAN_POINT('Ctrl Pts',(-35.0360276857693,-3.80061692502793,
124.922724356021));
#232285=CARTESIAN_POINT('Ctrl Pts',(-35.3144753095821,-7.00271344663942,
130.822759209339));
#232286=CARTESIAN_POINT('Ctrl Pts',(-35.592922933395,-3.76965841235978,
136.705886655638));
#232287=CARTESIAN_POINT('Ctrl Pts',(-35.8713705572079,2.92752854482695,
137.165799978524));
#232288=CARTESIAN_POINT('Ctrl Pts',(-36.1498181810209,6.9344597870381,131.779861302279));
#232289=CARTESIAN_POINT('Ctrl Pts',(-36.4282658048337,4.56896125215494,
125.49748515264));
#232290=CARTESIAN_POINT('Ctrl Pts',(-36.7067134286466,-1.99518946729269,
124.091868299989));
#232291=CARTESIAN_POINT('Ctrl Pts',(-36.9851610524595,-6.72585853672236,
128.854703963711));
#232292=CARTESIAN_POINT('Ctrl Pts',(-37.2636086762724,-5.27579218736066,
135.409178846303));
#232293=CARTESIAN_POINT('Ctrl Pts',(-37.5420563000852,1.02246944540875,
137.732050734562));
#232294=CARTESIAN_POINT('Ctrl Pts',(-37.8205039238982,6.38113160825695,
133.688713841779));
#232295=CARTESIAN_POINT('Ctrl Pts',(-38.0989515477111,5.87584555872632,
126.994797244432));
#232296=CARTESIAN_POINT('Ctrl Pts',(-38.377399171524,-0.0290555082599903,
123.801683279478));
#232297=CARTESIAN_POINT('Ctrl Pts',(-38.6558467953367,-5.90725598259587,
127.04368768842));
#232298=CARTESIAN_POINT('Ctrl Pts',(-38.9342944191497,-6.35697679442443,
133.741566800161));
#232299=CARTESIAN_POINT('Ctrl Pts',(-39.2127420429625,-0.964946487758246,
137.740296920595));
#232300=CARTESIAN_POINT('Ctrl Pts',(-39.4911896667755,5.31382250090111,
135.365240417872));
#232301=CARTESIAN_POINT('Ctrl Pts',(-39.7696372905882,6.70944820589337,
128.798958190032));
#232302=CARTESIAN_POINT('Ctrl Pts',(-40.0480849144012,1.93941878443644,
124.07554282374));
#232303=CARTESIAN_POINT('Ctrl Pts',(-40.3265325382142,-4.61284175404266,
125.535582288951));
#232304=CARTESIAN_POINT('Ctrl Pts',(-40.604980162027,-6.9261260704041,131.837371644027));
#232305=CARTESIAN_POINT('Ctrl Pts',(-40.8834277858398,-2.87463888813357,
137.18987433118));
#232306=CARTESIAN_POINT('Ctrl Pts',(-41.1618754096529,3.81850099841496,
136.674401865208));
#232307=CARTESIAN_POINT('Ctrl Pts',(-41.4403230334656,7.00262501156454,
130.76464826011));
#232308=CARTESIAN_POINT('Ctrl Pts',(-41.7187706572786,3.75167873633635,
124.891388371457));
#232309=CARTESIAN_POINT('Ctrl Pts',(-41.9972182810916,-2.94687701788942,
124.451861112224));
#232310=CARTESIAN_POINT('Ctrl Pts',(-42.2756659049044,-6.93739675562063,
129.849970561546));
#232311=CARTESIAN_POINT('Ctrl Pts',(-42.5541135287174,-4.55278778560923,
136.125117847804));
#232312=CARTESIAN_POINT('Ctrl Pts',(-42.8325611525302,2.01561074332903,
137.510749172913));
#232313=CARTESIAN_POINT('Ctrl Pts',(-43.1110087763431,6.73176146720674,
132.733537040953));
#232314=CARTESIAN_POINT('Ctrl Pts',(-43.389456400156,5.26175226755184,126.183506021407));
#232315=CARTESIAN_POINT('Ctrl Pts',(-43.6679040239687,-1.0435502150944,
123.879814634434));
#232316=CARTESIAN_POINT('Ctrl Pts',(-43.9463516477818,-6.38988103033122,
127.93944272308));
#232317=CARTESIAN_POINT('Ctrl Pts',(-44.2247992715946,-5.86422334173611,
134.631790397739));
#232318=CARTESIAN_POINT('Ctrl Pts',(-44.5032468954075,0.050369114677416,
137.806917084757));
#232319=CARTESIAN_POINT('Ctrl Pts',(-44.7816945192204,5.91867481537061,
134.547036472328));
#232320=CARTESIAN_POINT('Ctrl Pts',(-45.0601421430334,6.34800750407734,
127.847819589252));
#232321=CARTESIAN_POINT('Ctrl Pts',(-45.3385897668461,0.943831413943965,
123.865519476137));
#232322=CARTESIAN_POINT('Ctrl Pts',(-45.6170373906592,-5.32767963687585,
126.25967539076));
#232323=CARTESIAN_POINT('Ctrl Pts',(-45.895485014472,-6.7033133730266,132.830175008601));
#232324=CARTESIAN_POINT('Ctrl Pts',(-46.1739326382849,-1.91892959442962,
137.539050167615));
#232325=CARTESIAN_POINT('Ctrl Pts',(-46.4523802620978,4.62885673652604,
136.059074638009));
#232326=CARTESIAN_POINT('Ctrl Pts',(-46.7308278859106,6.92294985883713,
129.750273630666));
#232327=CARTESIAN_POINT('Ctrl Pts',(-47.0092755097235,2.8551902657795,124.410127069272));
#232328=CARTESIAN_POINT('Ctrl Pts',(-47.2877231335364,-3.83634969773052,
124.945968763085));
#232329=CARTESIAN_POINT('Ctrl Pts',(-47.5661707573492,-7.00247170512816,
130.865386372813));
#232330=CARTESIAN_POINT('Ctrl Pts',(-47.8446183811622,-3.73366430527375,
136.728724294741));
#232331=CARTESIAN_POINT('Ctrl Pts',(-48.123066004975,2.96619819148554,137.147861418602));
#232332=CARTESIAN_POINT('Ctrl Pts',(-48.4015136287881,6.9402694571073,131.737631203552));
#232333=CARTESIAN_POINT('Ctrl Pts',(-48.6799612526008,4.53657214265928,
125.469770912784));
#232334=CARTESIAN_POINT('Ctrl Pts',(-48.9584088764139,-2.03601334702262,
124.104137951514));
#232335=CARTESIAN_POINT('Ctrl Pts',(-49.2368565002267,-6.7376020355722,
128.895682296272));
#232336=CARTESIAN_POINT('Ctrl Pts',(-49.5153041240395,-5.24766360358919,
135.441208774179));
#232337=CARTESIAN_POINT('Ctrl Pts',(-49.7937517478526,1.06462131747325,
137.725698318783));
#232338=CARTESIAN_POINT('Ctrl Pts',(-50.0721993716652,6.39857125742062,
133.649816642113));
#232339=CARTESIAN_POINT('Ctrl Pts',(-50.3506469954783,5.85254679938199,
126.959099887138));
#232340=CARTESIAN_POINT('Ctrl Pts',(-50.6290946192911,-0.0716822544825644,
123.801989891996));
#232341=CARTESIAN_POINT('Ctrl Pts',(-50.907542243104,-5.93003881835047,
127.079716508824));
#232342=CARTESIAN_POINT('Ctrl Pts',(-51.1859898669169,-6.33897940665598,
133.780209102606));
#232343=CARTESIAN_POINT('Ctrl Pts',(-51.4644374907297,-0.922707596604453,
137.746042316915));
#232344=CARTESIAN_POINT('Ctrl Pts',(-51.7428851145428,5.34148741795441,
135.332809169526));
#232345=CARTESIAN_POINT('Ctrl Pts',(-52.0213327383556,6.69711644158035,
128.758153029896));
#232346=CARTESIAN_POINT('Ctrl Pts',(-52.2997803621686,1.89842262772099,
124.063861700536));
#232347=CARTESIAN_POINT('Ctrl Pts',(-52.5782279859813,-4.64482883791282,
125.563759584248));
#232348=CARTESIAN_POINT('Ctrl Pts',(-52.8566756097944,-6.91970951400822,
131.879513799985));
#232349=CARTESIAN_POINT('Ctrl Pts',(-53.135123233607,-2.83571519333325,
137.207254765232));
#232350=CARTESIAN_POINT('Ctrl Pts',(-53.4135708574202,3.85416285762642,
136.651048807542));
#232351=CARTESIAN_POINT('Ctrl Pts',(-53.6920184812329,7.0022535287505,130.72202202986));
#232352=CARTESIAN_POINT('Ctrl Pts',(-53.9704661050458,3.71561528605495,
124.868660391816));
#232353=CARTESIAN_POINT('Ctrl Pts',(-54.2489137288587,-2.98549188662705,
124.469917286158));
#232354=CARTESIAN_POINT('Ctrl Pts',(-54.5273613526715,-6.94307786488582,
129.892218147303));
#232355=CARTESIAN_POINT('Ctrl Pts',(-54.8058089764845,-4.5203144735249,
136.152733377983));
#232356=CARTESIAN_POINT('Ctrl Pts',(-55.0842566002972,2.05639708936689,
137.498355324372));
#232357=CARTESIAN_POINT('Ctrl Pts',(-55.3627042241104,6.74338018771311,
132.69252315503));
#232358=CARTESIAN_POINT('Ctrl Pts',(-55.6411518479232,5.23352632598741,
126.151561855625));
#232359=CARTESIAN_POINT('Ctrl Pts',(-55.919599471736,-1.08568255734582,
123.886295316588));
#232360=CARTESIAN_POINT('Ctrl Pts',(-56.1980470955489,-6.40720220901991,
127.978392822871));
#232361=CARTESIAN_POINT('Ctrl Pts',(-56.4764947193619,-5.8408160398338,
134.667416676276));
#232362=CARTESIAN_POINT('Ctrl Pts',(-56.7549423431748,0.0929947302327828,
137.806480732508));
#232363=CARTESIAN_POINT('Ctrl Pts',(-57.0333899669875,5.94134788626073,
134.510938475691));
#232364=CARTESIAN_POINT('Ctrl Pts',(-57.3118375908005,6.32989258579528,
127.809232243652));
#232365=CARTESIAN_POINT('Ctrl Pts',(-57.5902852146133,0.901575231427987,
123.859902667085));
#232366=CARTESIAN_POINT('Ctrl Pts',(-57.8687328384263,-5.35524571622284,
126.292190691378));
#232367=CARTESIAN_POINT('Ctrl Pts',(-58.1471804622391,-6.69085746896258,
132.870942446081));
#232368=CARTESIAN_POINT('Ctrl Pts',(-58.4256280860521,-1.87789807428466,
137.550606458515));
#232369=CARTESIAN_POINT('Ctrl Pts',(-58.7040757098649,4.6607579102399,136.030800115547));
#232370=CARTESIAN_POINT('Ctrl Pts',(-58.9825233336777,6.91640506593584,
129.708151199698));
#232371=CARTESIAN_POINT('Ctrl Pts',(-59.2609709574908,2.81621385120844,
124.392865186062));
#232372=CARTESIAN_POINT('Ctrl Pts',(-59.5394185813036,-3.87194031308425,
124.969430255013));
#232373=CARTESIAN_POINT('Ctrl Pts',(-59.8178662051166,-7.00197048445272,
130.908011274954));
#232374=CARTESIAN_POINT('Ctrl Pts',(-60.0963138289294,-3.69753184588372,
136.751342404371));
#232375=CARTESIAN_POINT('Ctrl Pts',(-60.3747614527424,3.00475792457964,
137.129687797925));
#232376=CARTESIAN_POINT('Ctrl Pts',(-60.6532090765552,6.94582195293937,
131.695366522141));
#232377=CARTESIAN_POINT('Ctrl Pts',(-60.9316567003681,4.50401492881459,
125.442254348109));
#232378=CARTESIAN_POINT('Ctrl Pts',(-61.210104324181,-2.07676178152925,
124.116655882255));
#232379=CARTESIAN_POINT('Ctrl Pts',(-61.4885519479939,-6.74909587010084,
128.93673135561));
#232380=CARTESIAN_POINT('Ctrl Pts',(-61.7669995718066,-5.21934056571308,
135.473066881942));
#232381=CARTESIAN_POINT('Ctrl Pts',(-62.0454471956197,1.10673373960332,
137.719089430292));
#232382=CARTESIAN_POINT('Ctrl Pts',(-62.3238948194324,6.41577380517329,
133.610814003028));
#232383=CARTESIAN_POINT('Ctrl Pts',(-62.6023424432454,5.82903117176375,
126.923545017394));
#232384=CARTESIAN_POINT('Ctrl Pts',(-62.8807900670583,-0.114306344492842,
123.802555979936));
#232385=CARTESIAN_POINT('Ctrl Pts',(-63.1592376908712,-5.95260191433588,
127.115883347286));
#232386=CARTESIAN_POINT('Ctrl Pts',(-63.4376853146842,-6.32074712567447,
133.818741133891));
#232387=CARTESIAN_POINT('Ctrl Pts',(-63.716132938497,-0.880434514181572,
137.751530486667));
#232388=CARTESIAN_POINT('Ctrl Pts',(-63.99458056231,5.36895440422691,135.300210117855));
#232389=CARTESIAN_POINT('Ctrl Pts',(-64.2730281861228,6.6845365131549,128.717423692735));
#232390=CARTESIAN_POINT('Ctrl Pts',(-64.5514758099358,1.85735612425694,
124.052430348997));
#232391=CARTESIAN_POINT('Ctrl Pts',(-64.8299234337484,-4.67664380594228,
125.592131071942));
#232392=CARTESIAN_POINT('Ctrl Pts',(-65.1083710575615,-6.91303654523158,
131.921616115747));
#232393=CARTESIAN_POINT('Ctrl Pts',(-65.3868186813742,-2.79668642006362,
137.224397937687));
#232394=CARTESIAN_POINT('Ctrl Pts',(-65.6652663051872,3.88968189941585,
136.627479098696));
#232395=CARTESIAN_POINT('Ctrl Pts',(-65.9437139290001,7.00162257485687,
130.679398850698));
#232396=CARTESIAN_POINT('Ctrl Pts',(-66.2221615528129,3.67941415228271,
124.846152361731));
#232397=CARTESIAN_POINT('Ctrl Pts',(-66.500609176626,-3.02399612686491,
124.48820818522));
#232398=CARTESIAN_POINT('Ctrl Pts',(-66.7790568004388,-6.94850169584742,
129.934499532835));
#232399=CARTESIAN_POINT('Ctrl Pts',(-67.0575044242516,-4.48767365952541,
136.180150722241));
#232400=CARTESIAN_POINT('Ctrl Pts',(-67.3359520480646,2.09710723485436,
137.485713427398));
#232401=CARTESIAN_POINT('Ctrl Pts',(-67.6143996718775,6.75474902978674,
132.651439302549));
#232402=CARTESIAN_POINT('Ctrl Pts',(-67.8928472956903,5.20510645418034,
126.119790101011));
#232403=CARTESIAN_POINT('Ctrl Pts',(-68.1712949195033,-1.12777466923081,
123.893032350195));
#232404=CARTESIAN_POINT('Ctrl Pts',(-68.449742543316,-6.42428596647451,
128.017447639935));
#232405=CARTESIAN_POINT('Ctrl Pts',(-68.728190167129,-5.81719230434518,
134.702899807851));
#232406=CARTESIAN_POINT('Ctrl Pts',(-69.0066377909419,0.135616899834216,
137.805784914121));
#232407=CARTESIAN_POINT('Ctrl Pts',(-69.2850854147548,5.96380079832,134.474703130449));
#232408=CARTESIAN_POINT('Ctrl Pts',(-69.5635330385676,6.31154311101565,
127.770755883637));
#232409=CARTESIAN_POINT('Ctrl Pts',(-69.8419806623805,0.859285640710264,
123.854543187474));
#232410=CARTESIAN_POINT('Ctrl Pts',(-70.1204282861936,-5.38261335497044,
126.324873192109));
#232411=CARTESIAN_POINT('Ctrl Pts',(-70.3988759100064,-6.67815363271447,
132.911633305611));
#232412=CARTESIAN_POINT('Ctrl Pts',(-70.6773235338194,-1.83679696793597,
137.561912764793));
#232413=CARTESIAN_POINT('Ctrl Pts',(-70.9557711576322,4.69248637785542,
136.002331925448));
#232414=CARTESIAN_POINT('Ctrl Pts',(-71.2342187814451,6.90960398310133,
129.666069389173));
#232415=CARTESIAN_POINT('Ctrl Pts',(-71.5126664052579,2.77713308079745,
124.375840883174));
#232416=CARTESIAN_POINT('Ctrl Pts',(-71.7911140290708,-3.90738745226578,
124.993107962432));
#232417=CARTESIAN_POINT('Ctrl Pts',(-72.0695616528837,-7.00120980318599,
130.950632336283));
#232418=CARTESIAN_POINT('Ctrl Pts',(-72.3480092766965,-3.66126237309149,
136.773740146404));
#232419=CARTESIAN_POINT('Ctrl Pts',(-72.6264569005095,3.04320631526353,
137.111279789924));
#232420=CARTESIAN_POINT('Ctrl Pts',(-72.9049045243223,6.95111706878496,
131.653068824177));
#232421=CARTESIAN_POINT('Ctrl Pts',(-73.1833521481353,4.47129081703998,
125.414936478256));
#232422=CARTESIAN_POINT('Ctrl Pts',(-73.4617997719481,-2.11743326086482,
124.129421628353));
#232423=CARTESIAN_POINT('Ctrl Pts',(-73.7402473957612,-6.76033961440018,
128.977849620639));
#232424=CARTESIAN_POINT('Ctrl Pts',(-74.018695019574,-5.19082412325261,
135.504751989078));
#232425=CARTESIAN_POINT('Ctrl Pts',(-74.2971426433868,1.14880515130821,
137.712224313981));
#232426=CARTESIAN_POINT('Ctrl Pts',(-74.5755902671998,6.43273861406817,
133.571707369781));
#232427=CARTESIAN_POINT('Ctrl Pts',(-74.8540378910127,5.80529954725181,
126.8881339527));
#232428=CARTESIAN_POINT('Ctrl Pts',(-75.1324855148255,-0.156926198840311,
123.803381522322));
#232429=CARTESIAN_POINT('Ctrl Pts',(-75.4109331386384,-5.97494443446864,
127.15218686363));
#232430=CARTESIAN_POINT('Ctrl Pts',(-75.6893807624512,-6.30228062708332,
133.857161466198));
#232431=CARTESIAN_POINT('Ctrl Pts',(-75.9678283862644,-0.838128806933456,
137.756761226486));
#232432=CARTESIAN_POINT('Ctrl Pts',(-76.2462760100769,5.3962224419198,135.267444470826));
#232433=CARTESIAN_POINT('Ctrl Pts',(-76.52472363389,6.67170888677059,128.676771687789));
#232434=CARTESIAN_POINT('Ctrl Pts',(-76.8031712577027,1.81622079577817,
124.041249192718));
#232435=CARTESIAN_POINT('Ctrl Pts',(-77.0816188815158,-4.70828547921653,
125.620695700721));
#232436=CARTESIAN_POINT('Ctrl Pts',(-77.3600665053286,-6.90610741134329,
131.963677031195));
#232437=CARTESIAN_POINT('Ctrl Pts',(-77.6385141291417,-2.75755401454922,
137.241303213299));
#232438=CARTESIAN_POINT('Ctrl Pts',(-77.9169617529544,3.92505680761298,
136.603693612052));
#232439=CARTESIAN_POINT('Ctrl Pts',(-78.1954093767674,7.00073217326374,
130.636780302039));
#232440=CARTESIAN_POINT('Ctrl Pts',(-78.4738570005803,3.6430766764653,124.823865115242));
#232441=CARTESIAN_POINT('Ctrl Pts',(-78.7523046243931,-3.06238831181505,
124.506733131632));
#232442=CARTESIAN_POINT('Ctrl Pts',(-79.0307522482061,-6.95366804752337,
129.976813151389));
#232443=CARTESIAN_POINT('Ctrl Pts',(-79.3091998720188,-4.45486655312747,
136.207368864621));
#232444=CARTESIAN_POINT('Ctrl Pts',(-79.5876474958318,2.13773967126259,
137.472823950436));
#232445=CARTESIAN_POINT('Ctrl Pts',(-79.8660951196445,6.76586757215105,
132.610287005887));
#232446=CARTESIAN_POINT('Ctrl Pts',(-80.1445427434577,5.17649370523912,
126.08819193488));
#232447=CARTESIAN_POINT('Ctrl Pts',(-80.4229903672703,-1.16982499101125,
123.900025485612));
#232448=CARTESIAN_POINT('Ctrl Pts',(-80.7014379910835,-6.44113166965063,
128.056605727087));
#232449=CARTESIAN_POINT('Ctrl Pts',(-80.9798856148961,-5.7933530106558,
134.738238477622));
#232450=CARTESIAN_POINT('Ctrl Pts',(-81.2583332387092,0.17823404410257,
137.804829655383));
#232451=CARTESIAN_POINT('Ctrl Pts',(-81.5367808625219,5.98603271954817,
134.438331779315));
#232452=CARTESIAN_POINT('Ctrl Pts',(-81.815228486335,6.29295975968447,127.732391934959));
#232453=CARTESIAN_POINT('Ctrl Pts',(-82.0936761101477,0.816964208846405,
123.849441235906));
#232454=CARTESIAN_POINT('Ctrl Pts',(-82.3721237339607,-5.40978153900143,
126.357721681897));
#232455=CARTESIAN_POINT('Ctrl Pts',(-82.6505713577735,-6.66520233502723,
132.952246079378));
#232456=CARTESIAN_POINT('Ctrl Pts',(-82.9290189815866,-1.79562779839943,
137.572968667493));
#232457=CARTESIAN_POINT('Ctrl Pts',(-83.2074666053992,4.72404096366304,
135.97367112261));
#232458=CARTESIAN_POINT('Ctrl Pts',(-83.4859142292123,6.90254686235,129.624029758449));
#232459=CARTESIAN_POINT('Ctrl Pts',(-83.7643618530252,2.73794940269844,
124.359054791448));
#232460=CARTESIAN_POINT('Ctrl Pts',(-84.0428094768383,-3.94268980176888,
125.017001007954));
#232461=CARTESIAN_POINT('Ctrl Pts',(-84.3212571006508,-7.00018968951541,
130.99324797746));
#232462=CARTESIAN_POINT('Ctrl Pts',(-84.5997047244641,-3.62485723087481,
136.795916690882));
#232463=CARTESIAN_POINT('Ctrl Pts',(-84.8781523482765,3.08154193881888,
137.092638076712));
#232464=CARTESIAN_POINT('Ctrl Pts',(-85.1565999720898,6.95615460843127,
131.61073967702));
#232465=CARTESIAN_POINT('Ctrl Pts',(-85.4350475959023,4.4384010199398,125.387818315495));
#232466=CARTESIAN_POINT('Ctrl Pts',(-85.7134952197154,-2.1580262779319,
124.142434716771));
#232467=CARTESIAN_POINT('Ctrl Pts',(-85.9919428435283,-6.7713328518292,
129.019035567703));
#232468=CARTESIAN_POINT('Ctrl Pts',(-86.2703904673411,-5.16211533289519,
135.536262921482));
#232469=CARTESIAN_POINT('Ctrl Pts',(-86.5488380911541,1.19083399361533,
137.70510322424));
#232470=CARTESIAN_POINT('Ctrl Pts',(-86.827285714967,6.4494650554685,133.532498191482));
#232471=CARTESIAN_POINT('Ctrl Pts',(-87.1057333387799,5.78135280522977,
126.852868005224));
#232472=CARTESIAN_POINT('Ctrl Pts',(-87.3841809625928,-0.199540238229241,
123.804466488563));
#232473=CARTESIAN_POINT('Ctrl Pts',(-87.6626285864056,-5.99706555083783,
127.188625712615));
#232474=CARTESIAN_POINT('Ctrl Pts',(-87.9410762102187,-6.28358059516641,
133.895468675847));
#232475=CARTESIAN_POINT('Ctrl Pts',(-88.2195238340314,-0.795792042514341,
137.761734342542));
#232476=CARTESIAN_POINT('Ctrl Pts',(-88.4979714578443,5.42329052060546,
135.234513442586));
#232477=CARTESIAN_POINT('Ctrl Pts',(-88.7764190816572,6.65863403776028,
128.636198521433));
#232478=CARTESIAN_POINT('Ctrl Pts',(-89.0548667054699,1.77501816656995,
124.03031864602));
#232479=CARTESIAN_POINT('Ctrl Pts',(-89.3333143292831,-4.73975268523957,
125.649452412109));
#232480=CARTESIAN_POINT('Ctrl Pts',(-89.6117619530957,-6.8989223691057,
132.005694987746));
#232481=CARTESIAN_POINT('Ctrl Pts',(-89.8902095769088,-2.71831942685781,
137.257969965635));
#232482=CARTESIAN_POINT('Ctrl Pts',(-90.1686572007216,3.9602862713853,136.579693228991));
#232483=CARTESIAN_POINT('Ctrl Pts',(-90.4471048245344,6.99958235696585,
130.59416796313));
#232484=CARTESIAN_POINT('Ctrl Pts',(-90.7255524483476,3.60660420510239,
124.801799478213));
#232485=CARTESIAN_POINT('Ctrl Pts',(-91.0040000721602,-3.10066701883943,
124.525491438947));
#232486=CARTESIAN_POINT('Ctrl Pts',(-91.2824476959735,-6.95857672847263,
130.019157435019));
#232487=CARTESIAN_POINT('Ctrl Pts',(-91.560895319786,-4.4218943700117,136.234386796543));
#232488=CARTESIAN_POINT('Ctrl Pts',(-91.8393429435991,2.17829289294083,
137.459687371113));
#232489=CARTESIAN_POINT('Ctrl Pts',(-92.1177905674117,6.77673540280433,
132.56906778996));
#232490=CARTESIAN_POINT('Ctrl Pts',(-92.3962381912249,5.14768913942031,
126.056768528114));
#232491=CARTESIAN_POINT('Ctrl Pts',(-92.6746858150375,-1.21183196449619,
123.907274463707));
#232492=CARTESIAN_POINT('Ctrl Pts',(-92.9531334388505,-6.45773869432309,
128.095865633305));
#232493=CARTESIAN_POINT('Ctrl Pts',(-93.2315810626634,-5.76929904214118,
134.773431376103));
#232494=CARTESIAN_POINT('Ctrl Pts',(-93.5100286864763,0.220844583841736,
137.803614991691));
#232495=CARTESIAN_POINT('Ctrl Pts',(-93.7884763102892,6.00804282613147,
134.401825770043));
#232496=CARTESIAN_POINT('Ctrl Pts',(-94.0669239341021,6.27414322041607,
127.694141819211));
#232497=CARTESIAN_POINT('Ctrl Pts',(-94.3453715579151,0.774612504073732,
123.844597001431));
#232498=CARTESIAN_POINT('Ctrl Pts',(-94.6238191817278,-5.43674926158731,
126.390734943524));
#232499=CARTESIAN_POINT('Ctrl Pts',(-94.9022668055408,-6.65200405581671,
132.99277926246));
#232500=CARTESIAN_POINT('Ctrl Pts',(-95.1807144293538,-1.75439209121494,
137.583773756932));
#232501=CARTESIAN_POINT('Ctrl Pts',(-95.4591620531666,4.75542049839504,
135.94481876907));
#232502=CARTESIAN_POINT('Ctrl Pts',(-95.7376096769794,6.89523396518648,
129.582033865318));
#232503=CARTESIAN_POINT('Ctrl Pts',(-96.0160573007924,2.69866426887766,
124.342507532899));
#232504=CARTESIAN_POINT('Ctrl Pts',(-96.2945049246052,-3.97784605345104,
125.041108506217));
#232505=CARTESIAN_POINT('Ctrl Pts',(-96.5729525484182,-6.99891018124123,
131.035856619345));
#232506=CARTESIAN_POINT('Ctrl Pts',(-96.8514001722308,-3.58831776824163,
136.817871216047));
#232507=CARTESIAN_POINT('Ctrl Pts',(-97.129847796044,3.11976337470375,137.073763349068));
#232508=CARTESIAN_POINT('Ctrl Pts',(-97.4082954198568,6.96093438520996,
131.56838064919));
#232509=CARTESIAN_POINT('Ctrl Pts',(-97.6867430436697,4.40534675625846,
125.360900864701));
#232510=CARTESIAN_POINT('Ctrl Pts',(-97.9651906674826,-2.1985393285419,
124.155694665303));
#232511=CARTESIAN_POINT('Ctrl Pts',(-98.2436382912955,-6.78207517502872,
129.060287670645));
#232512=CARTESIAN_POINT('Ctrl Pts',(-98.5220859151084,-5.13321525845608,
135.567598511506));
#232513=CARTESIAN_POINT('Ctrl Pts',(-98.8005335389213,1.23281870913114,
137.697726424945));
#232514=CARTESIAN_POINT('Ctrl Pts',(-99.0789811627341,6.4659525095689,133.493187921042));
#232515=CARTESIAN_POINT('Ctrl Pts',(-99.3574287865471,5.7571918330539,126.817748481762));
#232516=CARTESIAN_POINT('Ctrl Pts',(-99.6358764103599,-0.242146883580649,
123.805810838454));
#232517=CARTESIAN_POINT('Ctrl Pts',(-99.9143240341728,-6.01896444373747,
127.225198543987));
#232518=CARTESIAN_POINT('Ctrl Pts',(-100.192771657986,-6.26464772285957,
133.93366134335));
#232519=CARTESIAN_POINT('Ctrl Pts',(-100.471219281798,-0.753425789729175,
137.766449650557));
#232520=CARTESIAN_POINT('Ctrl Pts',(-100.749666905611,5.45015763726631,
135.201418253402));
#232521=CARTESIAN_POINT('Ctrl Pts',(-101.028114529424,6.64531245061667,
128.595705697122));
#232522=CARTESIAN_POINT('Ctrl Pts',(-101.306562153237,1.73374976341167,
124.019639113937));
#232523=CARTESIAN_POINT('Ctrl Pts',(-101.58500977705,-4.77104425798471,
125.678400140516));
#232524=CARTESIAN_POINT('Ctrl Pts',(-101.863457400863,-6.89148168476197,
132.047668428412));
#232525=CARTESIAN_POINT('Ctrl Pts',(-102.141905024676,-2.67898411084018,
137.274397577103));
#232526=CARTESIAN_POINT('Ctrl Pts',(-102.420352648489,3.99536898529432,
136.555478838857));
#232527=CARTESIAN_POINT('Ctrl Pts',(-102.698800272302,6.99817316856906,
130.551563412989));
#232528=CARTESIAN_POINT('Ctrl Pts',(-102.977247896115,3.56999808969468,
124.779956268296));
#232529=CARTESIAN_POINT('Ctrl Pts',(-103.255695519928,-3.13883082950684,
124.544482412068));
#232530=CARTESIAN_POINT('Ctrl Pts',(-103.53414314374,-6.96322755680218,
130.061530814641));
#232531=CARTESIAN_POINT('Ctrl Pts',(-103.812590767553,-4.38875833197407,
136.261203516848));
#232532=CARTESIAN_POINT('Ctrl Pts',(-104.091038391366,2.21876539717438,
137.44630417621));
#232533=CARTESIAN_POINT('Ctrl Pts',(-104.369486015179,6.78735211903507,
132.52778318216));
#232534=CARTESIAN_POINT('Ctrl Pts',(-104.647933638992,5.11869382408742,
126.02552104512));
#232535=CARTESIAN_POINT('Ctrl Pts',(-104.926381262805,-1.25379403310144,
123.914779015865));
#232536=CARTESIAN_POINT('Ctrl Pts',(-105.204828886617,-6.47410642511416,
128.135225903801));
#232537=CARTESIAN_POINT('Ctrl Pts',(-105.483276510431,-5.74503129012806,
134.808477199207));
#232538=CARTESIAN_POINT('Ctrl Pts',(-105.761724134243,0.263446940103889,
137.802140968053));
#232539=CARTESIAN_POINT('Ctrl Pts',(-106.040171758056,6.02983030247923,
134.365186455377));
#232540=CARTESIAN_POINT('Ctrl Pts',(-106.318619381869,6.25509419046252,
127.656006953765));
#232541=CARTESIAN_POINT('Ctrl Pts',(-106.597067005682,0.732232095750508,
123.840010663559));
#232542=CARTESIAN_POINT('Ctrl Pts',(-106.875514629495,-5.46351552342998,
126.423911753675));
#232543=CARTESIAN_POINT('Ctrl Pts',(-107.153962253308,-6.63855928414971,
133.033231352883));
#232544=CARTESIAN_POINT('Ctrl Pts',(-107.432409877121,-1.71309137438684,
137.594327632723));
#232545=CARTESIAN_POINT('Ctrl Pts',(-107.710857500934,4.78662381927155,
135.915775933963));
#232546=CARTESIAN_POINT('Ctrl Pts',(-107.989305124746,6.8876655625929,129.540083265954));
#232547=CARTESIAN_POINT('Ctrl Pts',(-108.26775274856,2.65927913505975,124.326199720693));
#232548=CARTESIAN_POINT('Ctrl Pts',(-108.546200372372,-4.0128549045848,
125.065429563905));
#232549=CARTESIAN_POINT('Ctrl Pts',(-108.824647996185,-6.99737132577695,
131.078456683062));
#232550=CARTESIAN_POINT('Ctrl Pts',(-109.103095619998,-3.5516453391731,
136.839602908365));
#232551=CARTESIAN_POINT('Ctrl Pts',(-109.381543243811,3.1578692066097,137.054656306401));
#232552=CARTESIAN_POINT('Ctrl Pts',(-109.659990867624,6.96545622200577,
131.525993310316));
#232553=CARTESIAN_POINT('Ctrl Pts',(-109.938438491437,4.37212925083209,
125.334185123311));
#232554=CARTESIAN_POINT('Ctrl Pts',(-110.21688611525,-2.23897091146772,
124.169200982596));
#232555=CARTESIAN_POINT('Ctrl Pts',(-110.495333739063,-6.79256618593892,
129.10160440085));
#232556=CARTESIAN_POINT('Ctrl Pts',(-110.773781362875,-5.10412497083799,
135.598757597999));
#232557=CARTESIAN_POINT('Ctrl Pts',(-111.052228986688,1.27475774209554,
137.690094189444));
#232558=CARTESIAN_POINT('Ctrl Pts',(-111.330676610501,6.48220036542147,
133.453778015119));
#232559=CARTESIAN_POINT('Ctrl Pts',(-111.609124234314,5.73281752601749,
126.782776683677));
#232560=CARTESIAN_POINT('Ctrl Pts',(-111.887571858127,-0.284744556090853,
123.807414522182));
#232561=CARTESIAN_POINT('Ctrl Pts',(-112.16601948194,-6.04064030169634,
127.261904002525));
#232562=CARTESIAN_POINT('Ctrl Pts',(-112.444467105753,-6.24548271172772,
133.971738053464));
#232563=CARTESIAN_POINT('Ctrl Pts',(-112.722914729566,-0.71103161847358,
137.770906975801));
#232564=CARTESIAN_POINT('Ctrl Pts',(-113.001362353379,5.47682279633179,
135.16816012963));
#232565=CARTESIAN_POINT('Ctrl Pts',(-113.279809977192,6.63174461897671,
128.55529471533));
#232566=CARTESIAN_POINT('Ctrl Pts',(-113.558257601004,1.69241711551747,
124.009210992206));
#232567=CARTESIAN_POINT('Ctrl Pts',(-113.836705224817,-4.80215903792943,
125.707537813274));
#232568=CARTESIAN_POINT('Ctrl Pts',(-114.11515284863,-6.88378563403075,
132.089595797848));
#232569=CARTESIAN_POINT('Ctrl Pts',(-114.393600472443,-2.63954952408134,
137.290585438973));
#232570=CARTESIAN_POINT('Ctrl Pts',(-114.672048096256,4.03030364933543,
136.531051338922));
#232571=CARTESIAN_POINT('Ctrl Pts',(-114.950495720069,6.99650466029252,
130.508968230339));
#232572=CARTESIAN_POINT('Ctrl Pts',(-115.228943343882,3.53325968669456,
124.758336294896));
#232573=CARTESIAN_POINT('Ctrl Pts',(-115.507390967695,-3.17687832964389,
124.563705347279));
#232574=CARTESIAN_POINT('Ctrl Pts',(-115.785838591507,-6.96762036017394,
130.103931720095));
#232575=CARTESIAN_POINT('Ctrl Pts',(-116.06428621532,-4.35545966688232,
136.287818031834));
#232576=CARTESIAN_POINT('Ctrl Pts',(-116.342733839133,2.25915568424066,
137.432674861647));
#232577=CARTESIAN_POINT('Ctrl Pts',(-116.621181462946,6.79771732743703,
132.486434712303));
#232578=CARTESIAN_POINT('Ctrl Pts',(-116.899629086759,5.08950883367243,
125.994450643782));
#232579=CARTESIAN_POINT('Ctrl Pts',(-117.178076710572,-1.2957096419083,
123.922538864004));
#232580=CARTESIAN_POINT('Ctrl Pts',(-117.456524334385,-6.49023425551004,
128.174685080065));
#232581=CARTESIAN_POINT('Ctrl Pts',(-117.734971958198,-5.7205506538686,
134.843374648297));
#232582=CARTESIAN_POINT('Ctrl Pts',(-118.013419582011,0.306039534242538,
137.800407639092));
#232583=CARTESIAN_POINT('Ctrl Pts',(-118.291867205823,6.05139434124684,
134.328415193001));
#232584=CARTESIAN_POINT('Ctrl Pts',(-118.570314829636,6.23581337569426,
127.617988751722));
#232585=CARTESIAN_POINT('Ctrl Pts',(-118.848762453449,0.689824554297045,
123.835682392233));
#232586=CARTESIAN_POINT('Ctrl Pts',(-119.127210077262,-5.49007933269568,
126.457250882969));
#232587=CARTESIAN_POINT('Ctrl Pts',(-119.405657701075,-6.62486851822702,
133.073600851681));
#232588=CARTESIAN_POINT('Ctrl Pts',(-119.684105324888,-1.67172717832737,
137.60462990379));
#232589=CARTESIAN_POINT('Ctrl Pts',(-119.962552948701,4.81764977004229,
135.886543693482));
#232590=CARTESIAN_POINT('Ctrl Pts',(-120.241000572514,6.87984193501854,
129.498179514853));
#232591=CARTESIAN_POINT('Ctrl Pts',(-120.519448196327,2.61979546067638,
124.310131959122));
#232592=CARTESIAN_POINT('Ctrl Pts',(-120.79789582014,-4.04771505790416,
125.089963279793));
#232593=CARTESIAN_POINT('Ctrl Pts',(-121.076343443952,-6.9955731801444,
131.121046590047));
#232594=CARTESIAN_POINT('Ctrl Pts',(-121.354791067765,-3.51484130258126,
136.86111096256));
#232595=CARTESIAN_POINT('Ctrl Pts',(-121.633238691578,3.19585802251066,
137.035317656727));
#232596=CARTESIAN_POINT('Ctrl Pts',(-121.911686315391,6.96971995125911,
131.483579231079));
#232597=CARTESIAN_POINT('Ctrl Pts',(-122.190133939204,4.3387497345494,125.307672081285));
#232598=CARTESIAN_POINT('Ctrl Pts',(-122.468581563017,-2.2793195285039,
124.182953168171));
#232599=CARTESIAN_POINT('Ctrl Pts',(-122.74702918683,-6.80280549581075,
129.142984227312));
#232600=CARTESIAN_POINT('Ctrl Pts',(-123.025476810643,-5.07484554799192,
135.629739026348));
#232601=CARTESIAN_POINT('Ctrl Pts',(-123.303924434456,1.31664953844379,
137.682206800553));
#232602=CARTESIAN_POINT('Ctrl Pts',(-123.582372058268,6.49820802095541,
133.414269934058));
#232603=CARTESIAN_POINT('Ctrl Pts',(-123.860819682081,5.7082307873194,126.747953906865));
#232604=CARTESIAN_POINT('Ctrl Pts',(-124.139267305894,-0.327331677286216,
123.809277480321));
#232605=CARTESIAN_POINT('Ctrl Pts',(-124.417714929707,-6.06209232150722,
127.298740728095));
#232606=CARTESIAN_POINT('Ctrl Pts',(-124.69616255352,-6.22608627193705,
134.009697395242));
#232607=CARTESIAN_POINT('Ctrl Pts',(-124.974610177333,-0.668611099680587,
137.77510615311));
#232608=CARTESIAN_POINT('Ctrl Pts',(-125.253057801146,5.50328500971429,
135.134740303665));
#232609=CARTESIAN_POINT('Ctrl Pts',(-125.531505424959,6.61793104560076,
128.514967073503));
#232610=CARTESIAN_POINT('Ctrl Pts',(-125.809953048772,1.6510217544855,123.999034667242));
#232611=CARTESIAN_POINT('Ctrl Pts',(-126.088400672584,-4.8330958721059,
125.736864350674));
#232612=CARTESIAN_POINT('Ctrl Pts',(-126.366848296398,-6.87583450209069,
132.131475542423));
#232613=CARTESIAN_POINT('Ctrl Pts',(-126.64529592021,-2.60001712784396,
137.306532951397));
#232614=CARTESIAN_POINT('Ctrl Pts',(-126.923743544023,4.06508896899354,
136.506411634357));
#232615=CARTESIAN_POINT('Ctrl Pts',(-127.202191167836,6.99457689396224,
130.466383993564));
#232616=CARTESIAN_POINT('Ctrl Pts',(-127.480638791649,3.49639035745773,
124.736940359153));
#232617=CARTESIAN_POINT('Ctrl Pts',(-127.759086415462,-3.21480810938582,
124.583159532264));
#232618=CARTESIAN_POINT('Ctrl Pts',(-128.037534039275,-6.97175497581086,
130.146358580199));
#232619=CARTESIAN_POINT('Ctrl Pts',(-128.315981663087,-4.32199960863106,
136.314229355287));
#232620=CARTESIAN_POINT('Ctrl Pts',(-128.594429286901,2.29946225746178,
137.418799932461));
#232621=CARTESIAN_POINT('Ctrl Pts',(-128.872876910713,6.80783064392392,
132.44502391257));
#232622=CARTESIAN_POINT('Ctrl Pts',(-129.151324534526,5.06013524963555,
125.963558475429));
#232623=CARTESIAN_POINT('Ctrl Pts',(-129.429772158339,-1.33757723771771,
123.930553720578));
#232624=CARTESIAN_POINT('Ctrl Pts',(-129.708219782152,-6.50612158788957,
128.214241699924));
#232625=CARTESIAN_POINT('Ctrl Pts',(-129.986667405965,-5.69585804050008,
134.878122430239));
#232626=CARTESIAN_POINT('Ctrl Pts',(-130.265115029778,0.348620787973942,
137.798415069035));
#232627=CARTESIAN_POINT('Ctrl Pts',(-130.543562653591,6.07273414337257,
134.291513345486));
#232628=CARTESIAN_POINT('Ctrl Pts',(-130.822010277403,6.21630149056731,
127.58008862186));
#232629=CARTESIAN_POINT('Ctrl Pts',(-131.100457901217,0.647391451141708,
123.831612347843));
#232630=CARTESIAN_POINT('Ctrl Pts',(-131.378905525029,-5.5164397050528,
126.490751096011));
#232631=CARTESIAN_POINT('Ctrl Pts',(-131.657353148842,-6.61093226536518,
133.113886262947));
#232632=CARTESIAN_POINT('Ctrl Pts',(-131.935800772655,-1.63030103580305,
137.614680188378));
#232633=CARTESIAN_POINT('Ctrl Pts',(-132.214248396468,4.848497201029,135.857123130838));
#232634=CARTESIAN_POINT('Ctrl Pts',(-132.492696020281,6.87176337237162,
129.456324164773));
#232635=CARTESIAN_POINT('Ctrl Pts',(-132.771143644094,2.58021470880796,
124.294304843582));
#232636=CARTESIAN_POINT('Ctrl Pts',(-133.049591267907,-4.08242522165371,
125.114708744776));
#232637=CARTESIAN_POINT('Ctrl Pts',(-133.32803889172,-6.99351581097555,
131.163624762118));
#232638=CARTESIAN_POINT('Ctrl Pts',(-133.606486515532,-3.47790702225152,
136.882394581644));
#232639=CARTESIAN_POINT('Ctrl Pts',(-133.884934139345,3.23372841471757,
137.015748116649));
#232640=CARTESIAN_POINT('Ctrl Pts',(-134.163381763158,6.97372541497715,
131.441139983145));
#232641=CARTESIAN_POINT('Ctrl Pts',(-134.441829386971,4.30520944429882,
125.281362721075));
#232642=CARTESIAN_POINT('Ctrl Pts',(-134.720277010784,-2.31958368451587,
124.196950712432));
#232643=CARTESIAN_POINT('Ctrl Pts',(-134.998724634597,-6.81279272522359,
129.184425616688));
#232644=CARTESIAN_POINT('Ctrl Pts',(-135.27717225841,-5.04537807487797,
135.660541648527));
#232645=CARTESIAN_POINT('Ctrl Pts',(-135.555619882223,1.35849254585843,
137.674064550544));
#232646=CARTESIAN_POINT('Ctrl Pts',(-135.834067506036,6.51397488300169,
133.374665141848));
#232647=CARTESIAN_POINT('Ctrl Pts',(-136.112515129848,5.68343252803032,
126.713281441693));
#232648=CARTESIAN_POINT('Ctrl Pts',(-136.390962753662,-0.369906669086523,
123.811399643837));
#232649=CARTESIAN_POINT('Ctrl Pts',(-136.669410377474,-6.08331970825794,
127.335707355701));
#232650=CARTESIAN_POINT('Ctrl Pts',(-136.947858001288,-6.20645912223011,
134.047537962086));
#232651=CARTESIAN_POINT('Ctrl Pts',(-137.2263056251,-0.626165805256695,
137.779047026878));
#232652=CARTESIAN_POINT('Ctrl Pts',(-137.504753248913,5.52954329684707,
135.101160013885));
#232653=CARTESIAN_POINT('Ctrl Pts',(-137.783200872726,6.60387224235649,
128.474724265995));
#232654=CARTESIAN_POINT('Ctrl Pts',(-138.061648496539,1.60956521423443,
123.989110516135));
#232655=CARTESIAN_POINT('Ctrl Pts',(-138.340096120352,-4.86385361413656,
125.766378666012));
#232656=CARTESIAN_POINT('Ctrl Pts',(-138.618543744165,-6.86762858357524,
132.173306110266));
#232657=CARTESIAN_POINT('Ctrl Pts',(-138.896991367977,-2.56038838701599,
137.322239523433));
#232658=CARTESIAN_POINT('Ctrl Pts',(-139.17543899179,4.09972365528409,136.481560638194));
#232659=CARTESIAN_POINT('Ctrl Pts',(-139.453886615603,6.99238994101352,
130.423812280637));
#232660=CARTESIAN_POINT('Ctrl Pts',(-139.732334239416,3.45939146819007,
124.715769253897));
#232661=CARTESIAN_POINT('Ctrl Pts',(-140.010781863229,-3.25261876323132,
124.602844246145));
#232662=CARTESIAN_POINT('Ctrl Pts',(-140.289229487042,-6.97563125050334,
130.188809822811));
#232663=CARTESIAN_POINT('Ctrl Pts',(-140.567677110855,-4.28837939709471,
136.340436508528));
#232664=CARTESIAN_POINT('Ctrl Pts',(-140.846124734668,2.33968362326381,
137.404679902793));
#232665=CARTESIAN_POINT('Ctrl Pts',(-141.124572358481,6.81769169374202,
132.403552317457));
#232666=CARTESIAN_POINT('Ctrl Pts',(-141.403019982293,5.03057416042698,
125.932845684778));
#232667=CARTESIAN_POINT('Ctrl Pts',(-141.681467606106,-1.37939526911043,
123.938823288595));
#232668=CARTESIAN_POINT('Ctrl Pts',(-141.959915229919,-6.52176783354029,
128.253894297592));
#232669=CARTESIAN_POINT('Ctrl Pts',(-142.238362853732,-5.67095436501806,
134.912719257437));
#232670=CARTESIAN_POINT('Ctrl Pts',(-142.516810477545,0.39118912343359,
137.796163331718));
#232671=CARTESIAN_POINT('Ctrl Pts',(-142.795258101358,6.09384891810056,
134.254482280245));
#232672=CARTESIAN_POINT('Ctrl Pts',(-143.073705725171,6.19655925810344,
127.542307968582));
#232673=CARTESIAN_POINT('Ctrl Pts',(-143.352153348984,0.604934358657401,
123.827800681205));
#232674=CARTESIAN_POINT('Ctrl Pts',(-143.630600972796,-5.54259566370794,
126.524411151443));
#232675=CARTESIAN_POINT('Ctrl Pts',(-143.90904859661,-6.59675104197701,
133.154086093891));
#232676=CARTESIAN_POINT('Ctrl Pts',(-144.187496220422,-1.58881448187379,
137.624478114069));
#232677=CARTESIAN_POINT('Ctrl Pts',(-144.465943844235,4.87916496916901,
135.827515336221));
#232678=CARTESIAN_POINT('Ctrl Pts',(-144.744391468048,6.86343017400547,
129.41451876668));
#232679=CARTESIAN_POINT('Ctrl Pts',(-145.022839091861,2.54053834613545,
124.278718960552));
#232680=CARTESIAN_POINT('Ctrl Pts',(-145.301286715674,-4.11698410963516,
125.139665041902));
#232681=CARTESIAN_POINT('Ctrl Pts',(-145.579734339487,-6.99119929450595,
131.206189621523));
#232682=CARTESIAN_POINT('Ctrl Pts',(-145.8581819633,-3.44084386679896,136.903452976945));
#232683=CARTESIAN_POINT('Ctrl Pts',(-146.136629587113,3.27147897992919,
136.995948411323));
#232684=CARTESIAN_POINT('Ctrl Pts',(-146.415077210925,6.97747246473481,
131.398677139117));
#232685=CARTESIAN_POINT('Ctrl Pts',(-146.693524834738,4.27150962292939,
125.255258017582));
#232686=CARTESIAN_POINT('Ctrl Pts',(-146.971972458551,-2.35976188750221,
124.211193096699));
#232687=CARTESIAN_POINT('Ctrl Pts',(-147.250420082364,-6.82252750409623,
129.225927033352));
#232688=CARTESIAN_POINT('Ctrl Pts',(-147.528867706177,-5.01572364342383,
135.69116432313));
#232689=CARTESIAN_POINT('Ctrl Pts',(-147.80731532999,1.40028521383297,137.665667741127));
#232690=CARTESIAN_POINT('Ctrl Pts',(-148.085762953803,6.52950036731291,
133.334965106058));
#232691=CARTESIAN_POINT('Ctrl Pts',(-148.364210577616,5.65842366705879,
126.678760572968));
#232692=CARTESIAN_POINT('Ctrl Pts',(-148.642658201429,-0.412467953858535,
123.813780934094));
#232693=CARTESIAN_POINT('Ctrl Pts',(-148.921105825242,-6.10432167535963,
127.372802515528));
#232694=CARTESIAN_POINT('Ctrl Pts',(-149.199553449054,-6.18660198989778,
134.085258351801));
#232695=CARTESIAN_POINT('Ctrl Pts',(-149.478001072867,-0.583697308029368,
137.782729451077));
#232696=CARTESIAN_POINT('Ctrl Pts',(-149.75644869668,5.55559668471987,135.067420504625));
#232697=CARTESIAN_POINT('Ctrl Pts',(-150.034896320493,6.58956873019717,
128.434567784019));
#232698=CARTESIAN_POINT('Ctrl Pts',(-150.313343944306,1.56804903095274,
123.979438906626));
#232699=CARTESIAN_POINT('Ctrl Pts',(-150.591791568119,-4.89443112428377,
125.796079665625));
#232700=CARTESIAN_POINT('Ctrl Pts',(-150.870239191931,-6.85916818255639,
132.21508595133));
#232701=CARTESIAN_POINT('Ctrl Pts',(-151.148686815745,-2.52066477005453,
137.33770457307));
#232702=CARTESIAN_POINT('Ctrl Pts',(-151.427134439557,4.13420642480782,
136.456499271296));
#232703=CARTESIAN_POINT('Ctrl Pts',(-151.705582063371,6.98994388248347,
130.381254669068));
#232704=CARTESIAN_POINT('Ctrl Pts',(-151.984029687183,3.42226438989971,
124.694823763634));
#232705=CARTESIAN_POINT('Ctrl Pts',(-152.262477310996,-3.29030889009209,
124.622758759495));
#232706=CARTESIAN_POINT('Ctrl Pts',(-152.540924934809,-6.97924904061452,
130.231283874884));
#232707=CARTESIAN_POINT('Ctrl Pts',(-152.819372558622,-4.25460027808296,
136.366438520441));
#232708=CARTESIAN_POINT('Ctrl Pts',(-153.097820182435,2.37981829122829,
137.390315295868));
#232709=CARTESIAN_POINT('Ctrl Pts',(-153.376267806248,6.82730011148789,
132.362021463707));
#232710=CARTESIAN_POINT('Ctrl Pts',(-153.654715430061,5.00082666144207,
125.902313409905));
#232711=CARTESIAN_POINT('Ctrl Pts',(-153.933163053873,-1.42116218650446,
123.947347261623));
#232712=CARTESIAN_POINT('Ctrl Pts',(-154.211610677687,-6.53717241268631,
128.293641403726));
#232713=CARTESIAN_POINT('Ctrl Pts',(-154.490058301499,-5.64584055023574,
134.947163847896));
#232714=CARTESIAN_POINT('Ctrl Pts',(-154.768505925312,0.433742963236675,
137.79365251058));
#232715=CARTESIAN_POINT('Ctrl Pts',(-155.046953549125,6.11473788301669,
134.217323369476));
#232716=CARTESIAN_POINT('Ctrl Pts',(-155.325401172938,6.17658740985663,
127.504648191865));
#232717=CARTESIAN_POINT('Ctrl Pts',(-155.603848796751,0.562454850108638,
123.824247533559));
#232718=CARTESIAN_POINT('Ctrl Pts',(-155.882296420564,-5.5685462394425,
126.558229801974));
#232719=CARTESIAN_POINT('Ctrl Pts',(-156.160744044376,-6.5823253735531,
133.194198854895));
#232720=CARTESIAN_POINT('Ctrl Pts',(-156.43919166819,-1.54726905384013,
137.634023317798));
#232721=CARTESIAN_POINT('Ctrl Pts',(-156.717639292002,4.90965193805665,
135.79772140676));
#232722=CARTESIAN_POINT('Ctrl Pts',(-156.996086915816,6.8548426487106,129.372764869687));
#232723=CARTESIAN_POINT('Ctrl Pts',(-157.274534539628,2.50076784287941,
124.263374887574));
#232724=CARTESIAN_POINT('Ctrl Pts',(-157.552982163441,-4.15139044125659,
125.164831246407));
#232725=CARTESIAN_POINT('Ctrl Pts',(-157.831429787254,-6.98862371657603,
131.248739591007));
#232726=CARTESIAN_POINT('Ctrl Pts',(-158.109877411067,-3.40365320961064,
136.924285368134));
#232727=CARTESIAN_POINT('Ctrl Pts',(-158.38832503488,3.30910831928323,136.975919274434));
#232728=CARTESIAN_POINT('Ctrl Pts',(-158.666772658693,6.98096096168483,
131.356192272474));
#232729=CARTESIAN_POINT('Ctrl Pts',(-158.945220282506,4.23765151920024,
125.229358938127));
#232730=CARTESIAN_POINT('Ctrl Pts',(-159.223667906319,-2.39985264864321,
124.225679793212));
#232731=CARTESIAN_POINT('Ctrl Pts',(-159.502115530131,-6.8320094717036,
129.267486939452));
#232732=CARTESIAN_POINT('Ctrl Pts',(-159.780563153944,-4.98588335248574,
135.721605915426));
#232733=CARTESIAN_POINT('Ctrl Pts',(-160.059010777757,1.44202599372318,
137.657016683454));
#232734=CARTESIAN_POINT('Ctrl Pts',(-160.33745840157,6.54478389858708,133.295171297791));
#232735=CARTESIAN_POINT('Ctrl Pts',(-160.615906025383,5.63320513111742,
126.644392579866));
#232736=CARTESIAN_POINT('Ctrl Pts',(-160.894353649196,-0.455013954479453,
123.816421262852));
#232737=CARTESIAN_POINT('Ctrl Pts',(-161.172801273009,-6.12509744457689,
127.410024833003));
#232738=CARTESIAN_POINT('Ctrl Pts',(-161.451248896821,-6.16651561075379,
134.122857166646));
#232739=CARTESIAN_POINT('Ctrl Pts',(-161.729696520635,-0.541207181682879,
137.786153289251));
#232740=CARTESIAN_POINT('Ctrl Pts',(-162.008144144447,5.58144420791359,
135.033523026113));
#232741=CARTESIAN_POINT('Ctrl Pts',(-162.286591768261,6.57502103914602,
128.394499115588));
#232742=CARTESIAN_POINT('Ctrl Pts',(-162.565039392073,1.52647474303778,
123.970020197102));
#232743=CARTESIAN_POINT('Ctrl Pts',(-162.843487015886,-4.92482726948487,
125.825966248931));
#232744=CARTESIAN_POINT('Ctrl Pts',(-163.121934639699,-6.85045361253876,
132.256813517449));
#232745=CARTESIAN_POINT('Ctrl Pts',(-163.400382263512,-2.48084774893327,
137.352927527244));
#232746=CARTESIAN_POINT('Ctrl Pts',(-163.678829887325,4.16853599979124,
136.431228462323));
#232747=CARTESIAN_POINT('Ctrl Pts',(-163.957277511138,6.98723880901292,
130.338712735846));
#232748=CARTESIAN_POINT('Ctrl Pts',(-164.23572513495,3.3850104983435,124.674104664506));
#232749=CARTESIAN_POINT('Ctrl Pts',(-164.514172758764,-3.32787709334726,
124.642902334375));
#232750=CARTESIAN_POINT('Ctrl Pts',(-164.792620382576,-6.98260821208591,
130.273779162525));
#232751=CARTESIAN_POINT('Ctrl Pts',(-165.07106800639,-4.22066350329308,
136.392234427513));
#232752=CARTESIAN_POINT('Ctrl Pts',(-165.349515630202,2.4198647741513,137.37570664397));
#232753=CARTESIAN_POINT('Ctrl Pts',(-165.627963254015,6.83665554111671,
132.320432890263));
#232754=CARTESIAN_POINT('Ctrl Pts',(-165.906410877828,4.97089385498702,
125.871962782194));
#232755=CARTESIAN_POINT('Ctrl Pts',(-166.184858501641,-1.46287644221077,
123.956125323802));
#232756=CARTESIAN_POINT('Ctrl Pts',(-166.463306125454,-6.55233475450377,
128.333481545486));
#232757=CARTESIAN_POINT('Ctrl Pts',(-166.741753749267,-5.62051752675643,
134.981454925258));
#232758=CARTESIAN_POINT('Ctrl Pts',(-167.020201373079,0.476280730534997,
137.790882698662));
#232759=CARTESIAN_POINT('Ctrl Pts',(-167.298648996893,6.13540026407138,
134.180037990117));
#232760=CARTESIAN_POINT('Ctrl Pts',(-167.577096620705,6.15638668589229,
127.467110687205));
#232761=CARTESIAN_POINT('Ctrl Pts',(-167.855544244518,0.519954499587912,
123.820953036571));
#232762=CARTESIAN_POINT('Ctrl Pts',(-168.133991868331,-5.5942904706483,
126.592205794446));
#232763=CARTESIAN_POINT('Ctrl Pts',(-168.412439492144,-6.56765579464175,
133.234223059563));
#232764=CARTESIAN_POINT('Ctrl Pts',(-168.690887115956,-1.50566629118217,
137.643315445865));
#232765=CARTESIAN_POINT('Ctrl Pts',(-168.96933473977,4.93995697798634,135.767742446477));
#232766=CARTESIAN_POINT('Ctrl Pts',(-169.247782363582,6.84600111470013,
129.331064021001));
#232767=CARTESIAN_POINT('Ctrl Pts',(-169.526229987396,2.46090467275213,
124.248273193229));
#232768=CARTESIAN_POINT('Ctrl Pts',(-169.804677611208,-4.18564294157836,
125.190206425745));
#232769=CARTESIAN_POINT('Ctrl Pts',(-170.083125235021,-6.98578917262369,
131.291273093865));
#232770=CARTESIAN_POINT('Ctrl Pts',(-170.361572858834,-3.36633642880185,
136.944890983262));
#232771=CARTESIAN_POINT('Ctrl Pts',(-170.640020482647,3.34661503841248,
136.955661448171));
#232772=CARTESIAN_POINT('Ctrl Pts',(-170.91846810646,6.98419077655865,131.313686957504));
#232773=CARTESIAN_POINT('Ctrl Pts',(-171.196915730273,4.20363638773547,
125.203666442409));
#232774=CARTESIAN_POINT('Ctrl Pts',(-171.475363354086,-2.43985448236259,
124.240410265162));
#232775=CARTESIAN_POINT('Ctrl Pts',(-171.753810977898,-6.84123827668714,
129.309103794972));
#232776=CARTESIAN_POINT('Ctrl Pts',(-172.032258601712,-4.9558583078063,
135.751865297389));
#232777=CARTESIAN_POINT('Ctrl Pts',(-172.310706225524,1.48371333881067,
137.648111698089));
#232778=CARTESIAN_POINT('Ctrl Pts',(-172.589153849337,6.55982491048677,
133.255285191615));
#232779=CARTESIAN_POINT('Ctrl Pts',(-172.86760147315,5.60777785468832,126.610178735912));
#232780=CARTESIAN_POINT('Ctrl Pts',(-173.146049096963,-0.497543094390354,
123.819320532272));
#232781=CARTESIAN_POINT('Ctrl Pts',(-173.424496720776,-6.14564624605571,
127.447372928838));
#232782=CARTESIAN_POINT('Ctrl Pts',(-173.702944344589,-6.14620072910595,
134.160333013378));
#232783=CARTESIAN_POINT('Ctrl Pts',(-173.981391968402,-0.498697000705985,
137.789318414533));
#232784=CARTESIAN_POINT('Ctrl Pts',(-174.259839592215,5.60708490864046,
134.999468834432));
#232785=CARTESIAN_POINT('Ctrl Pts',(-174.538287216028,6.56022970827155,
128.354519745462));
#232786=CARTESIAN_POINT('Ctrl Pts',(-174.81673483984,1.48484389103961,123.960854736574));
#232787=CARTESIAN_POINT('Ctrl Pts',(-175.095182463654,-4.95504092340126,
125.85603730847));
#232788=CARTESIAN_POINT('Ctrl Pts',(-175.373630087466,-6.8414851964426,
132.298487262391));
#232789=CARTESIAN_POINT('Ctrl Pts',(-175.652077711279,-2.44093879908611,
137.367907821863));
#232790=CARTESIAN_POINT('Ctrl Pts',(-175.930525335092,4.20271110814107,
136.405749147692));
#232791=CARTESIAN_POINT('Ctrl Pts',(-176.208972958905,6.98427482083815,
130.296188057377));
#232792=CARTESIAN_POINT('Ctrl Pts',(-176.487420582718,3.3476311739788,124.653612724266));
#232793=CARTESIAN_POINT('Ctrl Pts',(-176.765868206531,-3.36532198089259,
124.663274224357));
#232794=CARTESIAN_POINT('Ctrl Pts',(-177.044315830343,-6.98570864044213,
130.316294111058));
#232795=CARTESIAN_POINT('Ctrl Pts',(-177.322763454156,-4.18657033026512,
136.417823273865));
#232796=CARTESIAN_POINT('Ctrl Pts',(-177.601211077969,2.4598215880947,137.360854488428));
#232797=CARTESIAN_POINT('Ctrl Pts',(-177.879658701782,6.84575763596098,
132.278788138201));
#232798=CARTESIAN_POINT('Ctrl Pts',(-178.158106325595,4.94077685023126,
125.841794926299));
#232799=CARTESIAN_POINT('Ctrl Pts',(-178.436553949408,-1.50453649049278,
123.965157149858));
#232800=CARTESIAN_POINT('Ctrl Pts',(-178.715001573221,-6.56725429714808,
128.373413246577));
#232801=CARTESIAN_POINT('Ctrl Pts',(-178.993449197033,-5.59498623293233,
135.015591218853));
#232802=CARTESIAN_POINT('Ctrl Pts',(-179.271896820847,0.518800849074927,
137.787853998597));
#232803=CARTESIAN_POINT('Ctrl Pts',(-179.550344444659,6.15583529561319,
134.142627523792));
#232804=CARTESIAN_POINT('Ctrl Pts',(-179.828792068472,6.13595783475539,
127.429696845569));
#232805=CARTESIAN_POINT('Ctrl Pts',(-180.107239692285,0.477434881962636,
123.81791731232));
#232806=CARTESIAN_POINT('Ctrl Pts',(-180.385687316098,-5.61982740336347,
126.626337869861));
#232807=CARTESIAN_POINT('Ctrl Pts',(-180.664134939911,-6.55274284882976,
133.274157224785));
#232808=CARTESIAN_POINT('Ctrl Pts',(-180.942582563724,-1.4640077355066,
137.652354153945));
#232809=CARTESIAN_POINT('Ctrl Pts',(-181.221030187537,4.97007896599344,
135.737579566256));
#232810=CARTESIAN_POINT('Ctrl Pts',(-181.499477811349,6.83690589960112,
129.289417765863));
#232811=CARTESIAN_POINT('Ctrl Pts',(-181.777925435163,2.42095031289641,
124.233414437113));
#232812=CARTESIAN_POINT('Ctrl Pts',(-182.056373058975,-4.21974034136189,
125.215789639631));
#232813=CARTESIAN_POINT('Ctrl Pts',(-182.334820682789,-6.98269576768506,
131.333788554001));
#232814=CARTESIAN_POINT('Ctrl Pts',(-182.613268306601,-3.32889490715784,
136.965269058779));
#232815=CARTESIAN_POINT('Ctrl Pts',(-182.891715930414,3.38399774748988,
136.935175683191));
#232816=CARTESIAN_POINT('Ctrl Pts',(-183.170163554227,6.98716178967534,
131.27116276926));
#232817=CARTESIAN_POINT('Ctrl Pts',(-183.44861117804,4.16946548897866,125.178181482475));
#232818=CARTESIAN_POINT('Ctrl Pts',(-183.727058801853,-2.47976590637605,
124.255383966707));
#232819=CARTESIAN_POINT('Ctrl Pts',(-184.005506425666,-6.85021357707087,
129.350776057783));
#232820=CARTESIAN_POINT('Ctrl Pts',(-184.283954049479,-4.92564962197493,
135.781941347746));
#232821=CARTESIAN_POINT('Ctrl Pts',(-184.562401673291,1.52534570435398,
137.63895311501));
#232822=CARTESIAN_POINT('Ctrl Pts',(-184.840849297105,6.5746228456623,133.215308265529));
#232823=CARTESIAN_POINT('Ctrl Pts',(-185.119296920917,5.58214277998856,
126.576120308909));
#232824=CARTESIAN_POINT('Ctrl Pts',(-185.39774454473,-0.540053797659538,
123.822478634922));
#232825=CARTESIAN_POINT('Ctrl Pts',(-185.676192168543,-6.16596731835295,
127.484845419088));
#232826=CARTESIAN_POINT('Ctrl Pts',(-185.954639792356,-6.12565809773001,
134.197684503321));
#232827=CARTESIAN_POINT('Ctrl Pts',(-186.233087416169,-0.456168340327589,
137.792224709632));
#232828=CARTESIAN_POINT('Ctrl Pts',(-186.511535039982,5.63251783677319,
134.965259191474));
#232829=CARTESIAN_POINT('Ctrl Pts',(-186.789982663795,6.54519528567348,
128.314631155089));
#232830=CARTESIAN_POINT('Ctrl Pts',(-187.068430287608,1.44315801760525,
123.951942864674));
#232831=CARTESIAN_POINT('Ctrl Pts',(-187.346877911421,-4.98507096645316,
125.886291729948));
#232832=CARTESIAN_POINT('Ctrl Pts',(-187.625325535233,-6.83226326659722,
132.340105641921));
#232833=CARTESIAN_POINT('Ctrl Pts',(-187.903773159046,-2.40093939935397,
137.382644901827));
#232834=CARTESIAN_POINT('Ctrl Pts',(-188.182220782859,4.23673048348491,
136.380062271549));
#232835=CARTESIAN_POINT('Ctrl Pts',(-188.460668406672,6.98105202779173,
130.25368220943));
#232836=CARTESIAN_POINT('Ctrl Pts',(-188.739116030485,3.31012780190951,
124.633348702251));
#232837=CARTESIAN_POINT('Ctrl Pts',(-189.017563654298,-3.40264216519462,
124.683873674555));
#232838=CARTESIAN_POINT('Ctrl Pts',(-189.296011278111,-6.98855021079573,
130.358827145076));
#232839=CARTESIAN_POINT('Ctrl Pts',(-189.574458901924,-4.15232202233378,
136.443204111294));
#232840=CARTESIAN_POINT('Ctrl Pts',(-189.852906525736,2.49968725244504,
137.345759379595));
#232841=CARTESIAN_POINT('Ctrl Pts',(-190.13135414955,6.85460605873784,132.237088750687));
#232842=CARTESIAN_POINT('Ctrl Pts',(-190.409801773362,4.91047676317321,
125.8118109601));
#232843=CARTESIAN_POINT('Ctrl Pts',(-190.688249397175,-1.5461407876216,
123.974442405114));
#232844=CARTESIAN_POINT('Ctrl Pts',(-190.966697020988,-6.58193048776853,
128.413435027317));
#232845=CARTESIAN_POINT('Ctrl Pts',(-191.245144644801,-5.56924761483672,
135.049571463749));
#232846=CARTESIAN_POINT('Ctrl Pts',(-191.523592268614,0.561301743259386,
137.784566522618));
#232847=CARTESIAN_POINT('Ctrl Pts',(-191.802039892427,6.17604222041412,
134.105093356759));
#232848=CARTESIAN_POINT('Ctrl Pts',(-192.08048751624,6.11530161344434,127.39240805334));
#232849=CARTESIAN_POINT('Ctrl Pts',(-192.358935140053,0.43489757281158,
123.815140473294));
#232850=CARTESIAN_POINT('Ctrl Pts',(-192.637382763865,-5.64515609130746,
126.660624763449));
#232851=CARTESIAN_POINT('Ctrl Pts',(-192.915830387678,-6.53758708872167,
133.313999870785));
#232852=CARTESIAN_POINT('Ctrl Pts',(-193.194278011491,-1.42229493048546,
137.661139107108));
#232853=CARTESIAN_POINT('Ctrl Pts',(-193.472725635304,5.00001678589681,
135.707233883791));
#232854=CARTESIAN_POINT('Ctrl Pts',(-193.751173259117,6.82755734043935,
129.247827647489));
#232855=CARTESIAN_POINT('Ctrl Pts',(-194.02962088293,2.38090624383734,124.218799169824));
#232856=CARTESIAN_POINT('Ctrl Pts',(-194.308068506743,-4.25368137711504,
125.241579940071));
#232857=CARTESIAN_POINT('Ctrl Pts',(-194.586516130556,-6.97934361638637,
131.376284395991));
#232858=CARTESIAN_POINT('Ctrl Pts',(-194.864963754369,-3.29133003208973,
136.985418839569));
#232859=CARTESIAN_POINT('Ctrl Pts',(-195.143411378181,3.42125506128717,
136.914462738605));
#232860=CARTESIAN_POINT('Ctrl Pts',(-195.421859001994,6.98987389094189,
131.22862128349));
#232861=CARTESIAN_POINT('Ctrl Pts',(-195.700306625807,4.13514008914463,
125.152905002676));
#232862=CARTESIAN_POINT('Ctrl Pts',(-195.97875424962,-2.51958544175274,
124.270600342989));
#232863=CARTESIAN_POINT('Ctrl Pts',(-196.257201873433,-6.85893504027095,
129.392502183704));
#232864=CARTESIAN_POINT('Ctrl Pts',(-196.535649497246,-4.89525841438522,
135.811832952018));
#232865=CARTESIAN_POINT('Ctrl Pts',(-196.814097121059,1.56692154765205,
137.629541273595));
#232866=CARTESIAN_POINT('Ctrl Pts',(-197.092544744872,6.58917715577019,
133.175242000891));
#232867=CARTESIAN_POINT('Ctrl Pts',(-197.370992368684,5.55630085693524,
126.542218560906));
#232868=CARTESIAN_POINT('Ctrl Pts',(-197.649439992498,-0.582544489036021,
123.825895453776));
#232869=CARTESIAN_POINT('Ctrl Pts',(-197.92788761631,-6.18605990846357,
127.522440915193));
#232870=CARTESIAN_POINT('Ctrl Pts',(-198.206335240123,-6.10488847784037,
134.234910252398));
#232871=CARTESIAN_POINT('Ctrl Pts',(-198.484782863936,-0.413622776464342,
137.79487206686));
#232872=CARTESIAN_POINT('Ctrl Pts',(-198.763230487749,5.657742049887,134.930895364888));
#232873=CARTESIAN_POINT('Ctrl Pts',(-199.041678111562,6.52991832845634,
128.274834822558));
#232874=CARTESIAN_POINT('Ctrl Pts',(-199.320125735375,1.40141866741961,
123.943284911633));
#232875=CARTESIAN_POINT('Ctrl Pts',(-199.598573359188,-5.01491628586802,
125.916728392279));
#232876=CARTESIAN_POINT('Ctrl Pts',(-199.877020983,-6.82278816472322,132.381667113854));
#232877=CARTESIAN_POINT('Ctrl Pts',(-200.155468606814,-2.36085103192995,
137.397138221046));
#232878=CARTESIAN_POINT('Ctrl Pts',(-200.433916230626,4.27059286522247,
136.354168785731));
#232879=CARTESIAN_POINT('Ctrl Pts',(-200.712363854439,6.97757054929515,
130.211196767073));
#232880=CARTESIAN_POINT('Ctrl Pts',(-200.990811478252,3.27250177183757,
124.613313349352));
#232881=CARTESIAN_POINT('Ctrl Pts',(-201.269259102065,-3.43983626333961,
124.704699921646));
#232882=CARTESIAN_POINT('Ctrl Pts',(-201.547706725878,-6.9911328178512,
130.401376688499));
#232883=CARTESIAN_POINT('Ctrl Pts',(-201.826154349691,-4.1179198485831,
136.468375999304));
#232884=CARTESIAN_POINT('Ctrl Pts',(-202.104601973504,2.53946028996452,
137.330421876826));
#232885=CARTESIAN_POINT('Ctrl Pts',(-202.383049597317,6.86320048156709,
132.195336272904));
#232886=CARTESIAN_POINT('Ctrl Pts',(-202.66149722113,4.87999471659204,125.782011994664));
#232887=CARTESIAN_POINT('Ctrl Pts',(-202.939944844942,-1.5876877919352,
123.983980745501));
#232888=CARTESIAN_POINT('Ctrl Pts',(-203.218392468755,-6.59636278253501,
128.453545404684));
#232889=CARTESIAN_POINT('Ctrl Pts',(-203.496840092568,-5.54330262622176,
135.083394400798));
#232890=CARTESIAN_POINT('Ctrl Pts',(-203.775287716381,0.603781838200554,
137.781020392543));
#232891=CARTESIAN_POINT('Ctrl Pts',(-204.053735340194,6.19602028969954,
134.067436879861));
#232892=CARTESIAN_POINT('Ctrl Pts',(-204.332182964007,6.09441878738321,
127.355245692268));
#232893=CARTESIAN_POINT('Ctrl Pts',(-204.61063058782,0.392344148371673,
123.812622622391));
#232894=CARTESIAN_POINT('Ctrl Pts',(-204.889078211633,-5.67027559591653,
126.69506520469));
#232895=CARTESIAN_POINT('Ctrl Pts',(-205.167525835445,-6.5221890759199,
133.353749521179));
#232896=CARTESIAN_POINT('Ctrl Pts',(-205.445973459259,-1.38052942180316,
137.66966997982));
#232897=CARTESIAN_POINT('Ctrl Pts',(-205.724421083071,5.02976932833932,
135.676706523556));
#232898=CARTESIAN_POINT('Ctrl Pts',(-206.002868706884,6.8179557836299,129.206295207017));
#232899=CARTESIAN_POINT('Ctrl Pts',(-206.281316330697,2.340773949421,124.204427932937));
#232900=CARTESIAN_POINT('Ctrl Pts',(-206.55976395451,-4.28746479114066,
125.267576371395));
#232901=CARTESIAN_POINT('Ctrl Pts',(-206.838211578323,-6.97573284294384,
131.418759045136));
#232902=CARTESIAN_POINT('Ctrl Pts',(-207.116659202136,-3.253643195576,137.005339578972));
#232903=CARTESIAN_POINT('Ctrl Pts',(-207.395106825949,3.4583855992191,136.893523381939));
#232904=CARTESIAN_POINT('Ctrl Pts',(-207.673554449762,6.99232697986142,
131.186064076586));
#232905=CARTESIAN_POINT('Ctrl Pts',(-207.952002073574,4.10066146017411,
125.127837939644));
#232906=CARTESIAN_POINT('Ctrl Pts',(-208.230449697387,-2.55931161296347,
124.286058830161));
#232907=CARTESIAN_POINT('Ctrl Pts',(-208.5088973212,-6.86740234311116,129.434280626559));
#232908=CARTESIAN_POINT('Ctrl Pts',(-208.787344945013,-4.86468581119477,
135.841539002563));
#232909=CARTESIAN_POINT('Ctrl Pts',(-209.065792568826,1.60843932809579,
137.619876522599));
#232910=CARTESIAN_POINT('Ctrl Pts',(-209.344240192639,6.60348730149562,
133.135087882371));
#232911=CARTESIAN_POINT('Ctrl Pts',(-209.622687816452,5.53025304311036,
126.508474748144));
#232912=CARTESIAN_POINT('Ctrl Pts',(-209.901135440264,-0.625013594012848,
123.829570862223));
#232913=CARTESIAN_POINT('Ctrl Pts',(-210.179583064078,-6.20592327184948,
127.56015802404));
#232914=CARTESIAN_POINT('Ctrl Pts',(-210.45803068789,-6.08389263906328,
134.272008881199));
#232915=CARTESIAN_POINT('Ctrl Pts',(-210.736478311703,-0.371061885656257,
137.797260388114));
#232916=CARTESIAN_POINT('Ctrl Pts',(-211.014925935516,5.68275661328764,
134.896378628042));
#232917=CARTESIAN_POINT('Ctrl Pts',(-211.293373559329,6.51439940271492,
128.235132222534));
#232918=CARTESIAN_POINT('Ctrl Pts',(-211.571821183142,1.35962738715011,
123.934881198276));
#232919=CARTESIAN_POINT('Ctrl Pts',(-211.850268806955,-5.04457577571481,
125.947346167619));
#232920=CARTESIAN_POINT('Ctrl Pts',(-212.128716430768,-6.81306024192543,
132.423170138115));
#232921=CARTESIAN_POINT('Ctrl Pts',(-212.40716405458,-2.32067518230222,
137.411387242468));
#232922=CARTESIAN_POINT('Ctrl Pts',(-212.685611678394,4.30429699857105,
136.32806964973));
#232923=CARTESIAN_POINT('Ctrl Pts',(-212.964059302206,6.97383051435588,
130.168733304621));
#232924=CARTESIAN_POINT('Ctrl Pts',(-213.24250692602,3.23475447800865,124.593507407987));
#232925=CARTESIAN_POINT('Ctrl Pts',(-213.520954549832,-3.47690289708716,
124.725752193909));
#232926=CARTESIAN_POINT('Ctrl Pts',(-213.799402173646,-6.99345636590915,
130.443941164641));
#232927=CARTESIAN_POINT('Ctrl Pts',(-214.077849797458,-4.08336508379785,
136.49333800514));
#232928=CARTESIAN_POINT('Ctrl Pts',(-214.356297421271,2.57913922684953,
137.314842548456));
#232929=CARTESIAN_POINT('Ctrl Pts',(-214.634745045084,6.87154058597789,
132.153532252007));
#232930=CARTESIAN_POINT('Ctrl Pts',(-214.913192668897,4.84933184001288,
125.752399134204));
#232931=CARTESIAN_POINT('Ctrl Pts',(-215.19164029271,-1.62917596389355,
123.993771817573));
#232932=CARTESIAN_POINT('Ctrl Pts',(-215.470087916522,-6.61055064665203,
128.493742892374));
#232933=CARTESIAN_POINT('Ctrl Pts',(-215.748535540335,-5.51715222849034,
135.117058776675));
#232934=CARTESIAN_POINT('Ctrl Pts',(-216.026983164148,0.646239559784443,
137.777215739773));
#232935=CARTESIAN_POINT('Ctrl Pts',(-216.305430787961,6.21576876317433,
134.029659488472));
#232936=CARTESIAN_POINT('Ctrl Pts',(-216.583878411774,6.0733101303926,127.318211139417));
#232937=CARTESIAN_POINT('Ctrl Pts',(-216.862326035587,0.349776185474419,
123.810363852911));
#232938=CARTESIAN_POINT('Ctrl Pts',(-217.1407736594,-5.69518498637811,126.729657917385));
#232939=CARTESIAN_POINT('Ctrl Pts',(-217.419221283213,-6.50654938100331,
133.393404703032));
#232940=CARTESIAN_POINT('Ctrl Pts',(-217.697668907026,-1.33871275709491,
137.67794645597));
#232941=CARTESIAN_POINT('Ctrl Pts',(-217.976116530838,5.05933549082977,
135.64599861675));
#232942=CARTESIAN_POINT('Ctrl Pts',(-218.254564154652,6.80810158496121,
129.164821983446));
#232943=CARTESIAN_POINT('Ctrl Pts',(-218.533011778464,2.30055491676597,
124.190301258982));
#232944=CARTESIAN_POINT('Ctrl Pts',(-218.811459402277,-4.32108933158155,
125.293777970294));
#232945=CARTESIAN_POINT('Ctrl Pts',(-219.08990702609,-6.97186358115499,
131.461210927519));
#232946=CARTESIAN_POINT('Ctrl Pts',(-219.368354649903,-3.21583579411804,
137.02503053882));
#232947=CARTESIAN_POINT('Ctrl Pts',(-219.646802273716,3.49538798540175,
136.872358389107));
#232948=CARTESIAN_POINT('Ctrl Pts',(-219.925249897529,6.99452096553273,
131.143492725519));
#232949=CARTESIAN_POINT('Ctrl Pts',(-220.203697521342,4.06603087968498,
125.102981222246));
#232950=CARTESIAN_POINT('Ctrl Pts',(-220.482145145155,-2.59894294794204,
124.301758855404));
#232951=CARTESIAN_POINT('Ctrl Pts',(-220.760592768967,-6.87561517183164,
129.476109838232));
#232952=CARTESIAN_POINT('Ctrl Pts',(-221.03904039278,-4.83393294528274,
135.87105839861));
#232953=CARTESIAN_POINT('Ctrl Pts',(-221.317488016593,1.64989750722823,
137.609959220154));
#232954=CARTESIAN_POINT('Ctrl Pts',(-221.595935640406,6.61755275257056,
133.094847397895));
#232955=CARTESIAN_POINT('Ctrl Pts',(-221.874383264219,5.5040003037252,126.474890121013));
#232956=CARTESIAN_POINT('Ctrl Pts',(-222.152830888031,-0.667459538880483,
123.83350472407));
#232957=CARTESIAN_POINT('Ctrl Pts',(-222.431278511845,-6.22555667246622,
127.597995348007));
#232958=CARTESIAN_POINT('Ctrl Pts',(-222.709726135657,-6.06267135940695,
134.308979015016));
#232959=CARTESIAN_POINT('Ctrl Pts',(-222.988173759471,-0.328487245014279,
137.799389584896));
#232960=CARTESIAN_POINT('Ctrl Pts',(-223.266621383283,5.70756060005303,
134.861710259961));
#232961=CARTESIAN_POINT('Ctrl Pts',(-223.545069007096,6.49863908350723,
128.195524826214));
#232962=CARTESIAN_POINT('Ctrl Pts',(-223.823516630909,1.31778572538753,
123.926732036005));
#232963=CARTESIAN_POINT('Ctrl Pts',(-224.101964254722,-5.07404833695195,
125.978143921416));
#232964=CARTESIAN_POINT('Ctrl Pts',(-224.380411878535,-6.80307985867417,
132.464613176793));
#232965=CARTESIAN_POINT('Ctrl Pts',(-224.658859502348,-2.28041333920269,
137.425391438088));
#232966=CARTESIAN_POINT('Ctrl Pts',(-224.937307126161,4.33784163461131,
136.30176583066));
#232967=CARTESIAN_POINT('Ctrl Pts',(-225.215754749974,6.96983206156226,
130.126293395573));
#232968=CARTESIAN_POINT('Ctrl Pts',(-225.494202373786,3.19688731916334,
124.573931612073));
#232969=CARTESIAN_POINT('Ctrl Pts',(-225.7726499976,-3.51384069291894,124.747029711241));
#232970=CARTESIAN_POINT('Ctrl Pts',(-226.051097621412,-6.9955207688696,
130.486518996257));
#232971=CARTESIAN_POINT('Ctrl Pts',(-226.329545245225,-4.04865900841799,
136.518089203828));
#232972=CARTESIAN_POINT('Ctrl Pts',(-226.607992869038,2.61872259278156,
137.299021971784));
#232973=CARTESIAN_POINT('Ctrl Pts',(-226.886440492851,6.87962606292594,
132.111678237058));
#232974=CARTESIAN_POINT('Ctrl Pts',(-227.164888116664,4.81848926965818,
125.722973476035));
#232975=CARTESIAN_POINT('Ctrl Pts',(-227.443335740477,-1.67060376613766,
124.003815258517));
#232976=CARTESIAN_POINT('Ctrl Pts',(-227.72178336429,-6.62449355438458,
128.534026000853));
#232977=CARTESIAN_POINT('Ctrl Pts',(-228.000230988102,-5.49079739065326,
135.150563343936));
#232978=CARTESIAN_POINT('Ctrl Pts',(-228.278678611916,0.688673334723007,
137.773152705292));
#232979=CARTESIAN_POINT('Ctrl Pts',(-228.557126235728,6.23528690905198,
133.991762582447));
#232980=CARTESIAN_POINT('Ctrl Pts',(-228.835573859542,6.05197642466173,
127.281305767118));
#232981=CARTESIAN_POINT('Ctrl Pts',(-229.114021483354,0.307195261492642,
123.808364248553));
#232982=CARTESIAN_POINT('Ctrl Pts',(-229.392469107167,-5.7198833396657,
126.764401619687));
#232983=CARTESIAN_POINT('Ctrl Pts',(-229.670916730979,-6.49066858350677,
133.432963946903));
#232984=CARTESIAN_POINT('Ctrl Pts',(-229.949364354793,-1.29684648589306,
137.685968228869));
#232985=CARTESIAN_POINT('Ctrl Pts',(-230.227811978605,5.0887141777831,135.615111301269));
#232986=CARTESIAN_POINT('Ctrl Pts',(-230.506259602419,6.79799510958498,
129.123409513582));
#232987=CARTESIAN_POINT('Ctrl Pts',(-230.784707226231,2.26025063620168,
124.176419671429));
#232988=CARTESIAN_POINT('Ctrl Pts',(-231.063154850045,-4.35455375246839,
125.32018376586));
#232989=CARTESIAN_POINT('Ctrl Pts',(-231.341602473857,-6.96773597439774,
131.503638470075));
#232990=CARTESIAN_POINT('Ctrl Pts',(-231.62005009767,-3.17790922868121,
137.044490989456));
#232991=CARTESIAN_POINT('Ctrl Pts',(-231.898497721483,3.53226084869627,
136.850968544386));
#232992=CARTESIAN_POINT('Ctrl Pts',(-232.176945345296,6.99645576665798,
131.100908807788));
#232993=CARTESIAN_POINT('Ctrl Pts',(-232.455392969109,4.03124963092651,
125.078335771559));
#232994=CARTESIAN_POINT('Ctrl Pts',(-232.733840592922,-2.63847797813309,
124.317699836946));
#232995=CARTESIAN_POINT('Ctrl Pts',(-233.012288216734,-6.88357322210384,
129.517988268725));
#232996=CARTESIAN_POINT('Ctrl Pts',(-233.290735840548,-4.80300095620762,
135.900390046307));
#232997=CARTESIAN_POINT('Ctrl Pts',(-233.56918346436,1.6912945488023,137.599789733751));
#232998=CARTESIAN_POINT('Ctrl Pts',(-233.847631088173,6.63137298779474,
133.05452203859));
#232999=CARTESIAN_POINT('Ctrl Pts',(-234.126078711986,5.47754361158473,
126.441465924004));
#233000=CARTESIAN_POINT('Ctrl Pts',(-234.404526335799,-0.709880750790079,
123.837696893545));
#233001=CARTESIAN_POINT('Ctrl Pts',(-234.682973959612,-6.24495938279112,
127.635951485018));
#233002=CARTESIAN_POINT('Ctrl Pts',(-234.961421583425,-6.04122542523402,
134.345819283911));
#233003=CARTESIAN_POINT('Ctrl Pts',(-235.239869207238,-0.285900432155891,
137.801259578306));
#233004=CARTESIAN_POINT('Ctrl Pts',(-235.518316831051,5.73215309106056,
134.826891545298));
#233005=CARTESIAN_POINT('Ctrl Pts',(-235.796764454864,6.48263795483918,
128.156014101264));
#233006=CARTESIAN_POINT('Ctrl Pts',(-236.075212078676,1.27589523259052,
123.918837726791));
#233007=CARTESIAN_POINT('Ctrl Pts',(-236.353659702489,-5.10333287746112,
126.009120512446));
#233008=CARTESIAN_POINT('Ctrl Pts',(-236.632107326302,-6.79284738479763,
132.505994694203));
#233009=CARTESIAN_POINT('Ctrl Pts',(-236.910554950115,-2.24006699454776,
137.439150288976));
#233010=CARTESIAN_POINT('Ctrl Pts',(-237.189002573928,4.3712255303347,136.275258303218));
#233011=CARTESIAN_POINT('Ctrl Pts',(-237.467450197741,6.96557533907847,
130.083878612554));
#233012=CARTESIAN_POINT('Ctrl Pts',(-237.745897821554,3.15890169848239,
124.554586686994));
#233013=CARTESIAN_POINT('Ctrl Pts',(-238.024345445366,-3.55064828209192,
124.768531685198));
#233014=CARTESIAN_POINT('Ctrl Pts',(-238.30279306918,-6.99732595023538,
130.529108605612));
#233015=CARTESIAN_POINT('Ctrl Pts',(-238.581240692992,-4.01380290848946,
136.542628678202));
#233016=CARTESIAN_POINT('Ctrl Pts',(-238.859688316805,2.65820892098533,
137.282960733047));
#233017=CARTESIAN_POINT('Ctrl Pts',(-239.138135940618,6.88745661279959,
132.069775778975));
#233018=CARTESIAN_POINT('Ctrl Pts',(-239.416583564431,4.78746814841248,
125.693736110535));
#233019=CARTESIAN_POINT('Ctrl Pts',(-239.695031188244,-1.71196966354462,
124.014110696169));
#233020=CARTESIAN_POINT('Ctrl Pts',(-239.973478812057,-6.63819098907155,
128.574393237416));
#233021=CARTESIAN_POINT('Ctrl Pts',(-240.25192643587,-5.46423908930053,
135.183906861057));
#233022=CARTESIAN_POINT('Ctrl Pts',(-240.530374059683,0.731081590618679,
137.768831439659));
#233023=CARTESIAN_POINT('Ctrl Pts',(-240.808821683496,6.25457400407998,
133.95374756607));
#233024=CARTESIAN_POINT('Ctrl Pts',(-241.087269307308,6.03041846071876,
127.244530942912));
#233025=CARTESIAN_POINT('Ctrl Pts',(-241.365716931122,0.264602954276818,
123.806623883412));
#233026=CARTESIAN_POINT('Ctrl Pts',(-241.644164554934,-5.74436974057257,
126.799295024156));
#233027=CARTESIAN_POINT('Ctrl Pts',(-241.922612178747,-6.47454727189872,
133.472425786911));
#233028=CARTESIAN_POINT('Ctrl Pts',(-242.20105980256,-1.25493215956847,
137.693735001267));
#233029=CARTESIAN_POINT('Ctrl Pts',(-242.479507426373,5.11790430056101,
135.584045721651));
#233030=CARTESIAN_POINT('Ctrl Pts',(-242.757955050186,6.78763673199965,
129.082059331979));
#233031=CARTESIAN_POINT('Ctrl Pts',(-243.036402673998,2.21986260121965,
124.162783684665));
#233032=CARTESIAN_POINT('Ctrl Pts',(-243.314850297812,-4.38785681376436,
125.346792779616));
#233033=CARTESIAN_POINT('Ctrl Pts',(-243.593297921624,-6.96335017562108,
131.54604010063));
#233034=CARTESIAN_POINT('Ctrl Pts',(-243.871745545438,-3.13986490465013,
137.063720209766));
#233035=CARTESIAN_POINT('Ctrl Pts',(-244.15019316925,3.56900282276695,136.829354640385));
#233036=CARTESIAN_POINT('Ctrl Pts',(-244.428640793064,6.99813131154132,
131.058313901354));
#233037=CARTESIAN_POINT('Ctrl Pts',(-244.707088416876,3.99631900273028,
125.053902500829));
#233038=CARTESIAN_POINT('Ctrl Pts',(-244.985536040689,-2.67791523855318,
124.333881184089));
#233039=CARTESIAN_POINT('Ctrl Pts',(-245.263983664501,-6.89127619903846,
129.559914366219));
#233040=CARTESIAN_POINT('Ctrl Pts',(-245.542431288315,-4.7718909901659,
135.929532858758));
#233041=CARTESIAN_POINT('Ctrl Pts',(-245.820878912128,1.73262891883438,
137.589368440225));
#233042=CARTESIAN_POINT('Ctrl Pts',(-246.09932653594,6.6449474950541,133.014113298726));
#233043=CARTESIAN_POINT('Ctrl Pts',(-246.377774159753,5.45088394705135,
126.408203395661));
#233044=CARTESIAN_POINT('Ctrl Pts',(-246.656221783566,-0.752275657806765,
123.842147215306));
#233045=CARTESIAN_POINT('Ctrl Pts',(-246.934669407379,-6.26413068384941,
127.674025028594));
#233046=CARTESIAN_POINT('Ctrl Pts',(-247.213117031192,-6.01955563123113,
134.382528322752));
#233047=CARTESIAN_POINT('Ctrl Pts',(-247.491564655005,-0.243303025152602,
137.802870299053));
#233048=CARTESIAN_POINT('Ctrl Pts',(-247.770012278818,5.75653317502817,
134.791923774272));
#233049=CARTESIAN_POINT('Ctrl Pts',(-248.048459902631,6.46639660963695,
128.116601511768));
#233050=CARTESIAN_POINT('Ctrl Pts',(-248.326907526444,1.23395746102625,
123.91119856316));
#233051=CARTESIAN_POINT('Ctrl Pts',(-248.605355150257,-5.13242831209467,
126.040274792862));
#233052=CARTESIAN_POINT('Ctrl Pts',(-248.883802774069,-6.78236319946242,
132.547313156937));
#233053=CARTESIAN_POINT('Ctrl Pts',(-249.162250397883,-2.19963764338714,
137.452663285294));
#233054=CARTESIAN_POINT('Ctrl Pts',(-249.440698021695,4.40444744868852,
136.24854804965));
#233055=CARTESIAN_POINT('Ctrl Pts',(-249.719145645508,6.96106050463867,
130.041490527264));
#233056=CARTESIAN_POINT('Ctrl Pts',(-249.997593269321,3.12079902353814,
124.535473349588));
#233057=CARTESIAN_POINT('Ctrl Pts',(-250.276040893134,-3.58732430068758,
124.790257319018));
#233058=CARTESIAN_POINT('Ctrl Pts',(-250.554488516946,-6.99887184311352,
130.571708414529));
#233059=CARTESIAN_POINT('Ctrl Pts',(-250.83293614076,-3.97879807562073,
136.566955518948));
#233060=CARTESIAN_POINT('Ctrl Pts',(-251.111383764572,2.69759674828547,
137.26665942739));
#233061=CARTESIAN_POINT('Ctrl Pts',(-251.389831388386,6.89503194542569,
132.027826430486));
#233062=CARTESIAN_POINT('Ctrl Pts',(-251.668279012198,4.75626962579305,
125.66468812107));
#233063=CARTESIAN_POINT('Ctrl Pts',(-251.946726636011,-1.75327212332407,
124.024657749096));
#233064=CARTESIAN_POINT('Ctrl Pts',(-252.225174259824,-6.65164244307981,
128.614843106116));
#233065=CARTESIAN_POINT('Ctrl Pts',(-252.503621883637,-5.43747830869239,
135.217088092717));
#233066=CARTESIAN_POINT('Ctrl Pts',(-252.78206950745,0.773462756270139,
137.764252102553));
#233067=CARTESIAN_POINT('Ctrl Pts',(-253.060517131263,6.2736293330892,133.91561584884));
#233068=CARTESIAN_POINT('Ctrl Pts',(-253.338964755075,6.00863703830687,
127.207888027921));
#233069=CARTESIAN_POINT('Ctrl Pts',(-253.617412378889,0.222000840393564,
123.805142824969));
#233070=CARTESIAN_POINT('Ctrl Pts',(-253.895860002702,-5.76864327852066,
126.83433683216));
#233071=CARTESIAN_POINT('Ctrl Pts',(-254.174307626514,-6.45818604965135,
133.511788771436));
#233072=CARTESIAN_POINT('Ctrl Pts',(-254.452755250327,-1.21297131977014,
137.701246465247));
#233073=CARTESIAN_POINT('Ctrl Pts',(-254.73120287414,5.14690475579816,135.55280306703));
#233074=CARTESIAN_POINT('Ctrl Pts',(-255.009650497953,6.7770268770417,129.040772899161));
#233075=CARTESIAN_POINT('Ctrl Pts',(-255.288098121766,2.17939223099114,
124.149393939406));
#233076=CARTESIAN_POINT('Ctrl Pts',(-255.566545745579,-4.42099713522674,
125.37360376984));
#233077=CARTESIAN_POINT('Ctrl Pts',(-255.844993369392,-6.95870662337211,
131.588414730824));
#233078=CARTESIAN_POINT('Ctrl Pts',(-256.123440993205,-3.10170371057109,
137.082716575498));
#233079=CARTESIAN_POINT('Ctrl Pts',(-256.401888617018,3.60561156199617,
136.807519199501));
#233080=CARTESIAN_POINT('Ctrl Pts',(-256.68033624083,6.99954939633056,131.01570633407));
#233081=CARTESIAN_POINT('Ctrl Pts',(-256.958783864643,3.96123678073902,
125.029688453078));
#233082=CARTESIAN_POINT('Ctrl Pts',(-257.237231488456,-2.71724664265218,
124.350290708114));
#233083=CARTESIAN_POINT('Ctrl Pts',(-257.515679112269,-6.89873632689917,
129.601908459729));
#233084=CARTESIAN_POINT('Ctrl Pts',(-257.794126736082,-4.74058057908887,
135.958444437253));
#233085=CARTESIAN_POINT('Ctrl Pts',(-258.072574359895,1.77385448465437,
137.578773744179));
#233086=CARTESIAN_POINT('Ctrl Pts',(-258.351021983707,6.6583599873155,132.973475360041));
#233087=CARTESIAN_POINT('Ctrl Pts',(-258.629469607521,5.42386327951784,
126.375381938049));
#233088=CARTESIAN_POINT('Ctrl Pts',(-258.907917231333,-0.794342416617398,
123.846330221273));
#233089=CARTESIAN_POINT('Ctrl Pts',(-259.186364855146,-6.28363694765996,
127.713206958712));
#233090=CARTESIAN_POINT('Ctrl Pts',(-259.464812478959,-5.99659113747434,
134.41722675292));
#233091=CARTESIAN_POINT('Ctrl Pts',(-259.743260102772,-0.202727240537578,
137.807801967267));
#233092=CARTESIAN_POINT('Ctrl Pts',(-260.021707726585,5.7845923739281,134.749768174183));
#233093=CARTESIAN_POINT('Ctrl Pts',(-260.253747413096,6.33253704604016,
129.202365411857));
#233094=CARTESIAN_POINT('Ctrl Pts',(-260.439389088604,3.82430165355141,
125.973250269562));
#233095=CARTESIAN_POINT('Ctrl Pts',(-260.532214889509,1.97943258085903,
125.138073123498));
#233096=CARTESIAN_POINT('Ctrl Pts',(-260.578632753112,1.00712299976162,
124.970230583726));
#233097=CARTESIAN_POINT('Ctrl Pts',(207.955458783725,-5.89986192518215,
130.414453211936));
#233098=CARTESIAN_POINT('Ctrl Pts',(207.964054739687,-5.87737129978886,
130.750371489811));
#233099=CARTESIAN_POINT('Ctrl Pts',(207.961523532031,-5.84640950003041,
131.085475744573));
#233100=CARTESIAN_POINT('Ctrl Pts',(207.946544851276,-5.80258759547012,
131.456229395558));
#233101=CARTESIAN_POINT('Ctrl Pts',(207.944935584475,-5.7981622731838,131.492794197297));
#233102=CARTESIAN_POINT('Ctrl Pts',(207.943168852932,-5.79356696020855,
131.52989605424));
#233103=CARTESIAN_POINT('Ctrl Pts',(207.943142385322,-5.79349817258261,
131.53045124226));
#233104=CARTESIAN_POINT('Ctrl Pts',(207.94310533414,-5.79340195614918,131.531227539937));
#233105=CARTESIAN_POINT('Ctrl Pts',(207.94309477597,-5.79337454689547,131.531448653929));
#233106=CARTESIAN_POINT('Ctrl Pts',(207.943077748303,-5.79333035677605,
131.531805092076));
#233107=CARTESIAN_POINT('Ctrl Pts',(207.943071281854,-5.7933135783506,131.531940415657));
#233108=CARTESIAN_POINT('Ctrl Pts',(207.943059016683,-5.79328176025719,
131.532197017465));
#233109=CARTESIAN_POINT('Ctrl Pts',(207.943053218331,-5.79326672089837,
131.53231829545));
#233110=CARTESIAN_POINT('Ctrl Pts',(207.943040063266,-5.79323260617857,
131.53259337706));
#233111=CARTESIAN_POINT('Ctrl Pts',(207.943032705692,-5.7932135301817,131.532747180222));
#233112=CARTESIAN_POINT('Ctrl Pts',(207.943010733002,-5.7931565741522,131.533206352869));
#233113=CARTESIAN_POINT('Ctrl Pts',(207.942996111113,-5.79311868898518,
131.533511720278));
#233114=CARTESIAN_POINT('Ctrl Pts',(207.942874410758,-5.79280350296,131.536051743128));
#233115=CARTESIAN_POINT('Ctrl Pts',(207.942766851691,-5.79252583105091,
131.538286329208));
#233116=CARTESIAN_POINT('Ctrl Pts',(207.941632120879,-5.78960574275957,
131.561753268497));
#233117=CARTESIAN_POINT('Ctrl Pts',(207.940561232304,-5.786929583699,131.582979183399));
#233118=CARTESIAN_POINT('Ctrl Pts',(207.935616314913,-5.77491032228197,
131.677081722506));
#233119=CARTESIAN_POINT('Ctrl Pts',(207.93126593134,-5.76519996462025,131.749881133765));
#233120=CARTESIAN_POINT('Ctrl Pts',(207.908432950335,-5.71778482372917,
132.090906340396));
#233121=CARTESIAN_POINT('Ctrl Pts',(207.883444286136,-5.67508447486567,
132.357688125701));
#233122=CARTESIAN_POINT('Ctrl Pts',(207.851560096185,-5.62714347058168,
132.623000814592));
#233123=CARTESIAN_POINT('Origin',(213.235140564004,0.,130.804360617566));
#233124=CARTESIAN_POINT('',(207.935358922621,4.83993619626808,129.931218342011));
#233125=CARTESIAN_POINT('',(207.344471284167,2.40266844899661,126.515070645963));
#233126=CARTESIAN_POINT('Ctrl Pts',(207.932945971377,4.83234977408945,129.889167346526));
#233127=CARTESIAN_POINT('Ctrl Pts',(207.913056351572,4.7697277774651,129.558514356806));
#233128=CARTESIAN_POINT('Ctrl Pts',(207.882216843952,4.67183438727748,129.22996814172));
#233129=CARTESIAN_POINT('Ctrl Pts',(207.767461666534,4.28964812743425,128.310813320659));
#233130=CARTESIAN_POINT('Ctrl Pts',(207.660120443156,3.9118143497335,127.760719114158));
#233131=CARTESIAN_POINT('Ctrl Pts',(207.486761489502,3.17206573993542,127.02097050436));
#233132=CARTESIAN_POINT('Ctrl Pts',(207.410948455005,2.80990088697428,126.741872036394));
#233133=CARTESIAN_POINT('Ctrl Pts',(207.345096392365,2.41028028844146,126.517201652278));
#233134=CARTESIAN_POINT('',(207.776993964391,4.32587057920753,133.142886646627));
#233135=CARTESIAN_POINT('Ctrl Pts',(207.778436608163,4.32133082450553,133.15282457677));
#233136=CARTESIAN_POINT('Ctrl Pts',(207.80166991443,4.4022999262327,133.003836011816));
#233137=CARTESIAN_POINT('Ctrl Pts',(207.823382325825,4.47588902830909,132.850000075013));
#233138=CARTESIAN_POINT('Ctrl Pts',(207.918593342393,4.79298445822067,132.087388166203));
#233139=CARTESIAN_POINT('Ctrl Pts',(207.96044672069,4.91825,131.426623044073));
#233140=CARTESIAN_POINT('Ctrl Pts',(207.96044672069,4.91825,130.532140837719));
#233141=CARTESIAN_POINT('Ctrl Pts',(207.953011753591,4.89537008512156,130.252332639368));
#233142=CARTESIAN_POINT('Ctrl Pts',(207.93776844465,4.84751183684522,129.97320957585));
#233143=CARTESIAN_POINT('Ctrl Pts',(207.777553167153,4.32872518108459,133.139167112577));
#233144=CARTESIAN_POINT('Ctrl Pts',(207.769784873384,4.39355921696334,133.018964978353));
#233145=CARTESIAN_POINT('Ctrl Pts',(207.762016579614,4.45347444860551,132.895890200518));
#233146=CARTESIAN_POINT('Ctrl Pts',(207.754248285845,4.50820764817201,132.770383726144));
#233147=CARTESIAN_POINT('Ctrl Pts',(207.746488411523,4.5628815266944,132.645013278445));
#233148=CARTESIAN_POINT('Ctrl Pts',(207.7387285372,4.61238439418871,132.517216734316));
#233149=CARTESIAN_POINT('Ctrl Pts',(207.730968662878,4.6564985492191,132.387460211281));
#233150=CARTESIAN_POINT('Ctrl Pts',(207.723215343369,4.70057544075838,132.257813294358));
#233151=CARTESIAN_POINT('Ctrl Pts',(207.715462023859,4.73927255412797,132.126210061989));
#233152=CARTESIAN_POINT('Ctrl Pts',(207.707708704349,4.77242014607768,131.993136884074));
#233153=CARTESIAN_POINT('Ctrl Pts',(207.699619190911,4.80700506034141,131.854293481633));
#233154=CARTESIAN_POINT('Ctrl Pts',(207.691529677474,4.83554820242537,131.71385019373));
#233155=CARTESIAN_POINT('Ctrl Pts',(207.683440164036,4.85791441337539,131.572377944727));
#233156=CARTESIAN_POINT('Ctrl Pts',(207.675693401989,4.87933297154286,131.436899852299));
#233157=CARTESIAN_POINT('Ctrl Pts',(207.667946639943,4.89508723941358,131.30047862999));
#233158=CARTESIAN_POINT('Ctrl Pts',(207.660199877896,4.9051107445793,131.163626043001));
#233159=CARTESIAN_POINT('Ctrl Pts',(207.652453621073,4.91513359603885,131.02678238117));
#233160=CARTESIAN_POINT('Ctrl Pts',(207.644707364249,4.91942639951774,130.889507800467));
#233161=CARTESIAN_POINT('Ctrl Pts',(207.636961107426,4.91797464963016,130.752318249297));
#233162=CARTESIAN_POINT('Ctrl Pts',(207.629213678398,4.91652268005615,130.615107937881));
#233163=CARTESIAN_POINT('Ctrl Pts',(207.62146624937,4.90932443143035,130.47798307252));
#233164=CARTESIAN_POINT('Ctrl Pts',(207.613718820343,4.89641751401577,130.341458261837));
#233165=CARTESIAN_POINT('Ctrl Pts',(207.605968541273,4.88350584854127,130.204883227854));
#233166=CARTESIAN_POINT('Ctrl Pts',(207.598218262203,4.8648813720697,130.068909076728));
#233167=CARTESIAN_POINT('Ctrl Pts',(207.590467983133,4.84063335749527,129.934043571425));
#233168=CARTESIAN_POINT('Ctrl Pts',(207.582708968004,4.81635801073261,129.79902604669));
#233169=CARTESIAN_POINT('Ctrl Pts',(207.574949952875,4.78644654020057,129.665120047497));
#233170=CARTESIAN_POINT('Ctrl Pts',(207.567190937746,4.751039073567,129.532821871031));
#233171=CARTESIAN_POINT('Ctrl Pts',(207.559426780275,4.71560814038174,129.400436013003));
#233172=CARTESIAN_POINT('Ctrl Pts',(207.551662622803,4.67467407196882,129.269660472309));
#233173=CARTESIAN_POINT('Ctrl Pts',(207.543898465331,4.62842600073996,129.140973765936));
#233174=CARTESIAN_POINT('Ctrl Pts',(207.536123292545,4.58211231555991,129.01210448669));
#233175=CARTESIAN_POINT('Ctrl Pts',(207.528348119759,4.53046972426244,128.885330318326));
#233176=CARTESIAN_POINT('Ctrl Pts',(207.520572946973,4.47373451129918,128.761107675586));
#233177=CARTESIAN_POINT('Ctrl Pts',(207.518235425263,4.45667768238356,128.723761479917));
#233178=CARTESIAN_POINT('Ctrl Pts',(207.515897903554,4.43916086859752,128.686645716714));
#233179=CARTESIAN_POINT('Ctrl Pts',(207.513560381844,4.42119126588729,128.649772291936));
#233180=CARTESIAN_POINT('Ctrl Pts',(207.505787242456,4.36143557419401,128.527154277599));
#233181=CARTESIAN_POINT('Ctrl Pts',(207.498014103069,4.29648027204063,128.406829765919));
#233182=CARTESIAN_POINT('Ctrl Pts',(207.490240963681,4.2265243627226,128.289271181023));
#233183=CARTESIAN_POINT('Ctrl Pts',(207.48247687602,4.15664991620944,128.171849491667));
#233184=CARTESIAN_POINT('Ctrl Pts',(207.474712788358,4.08178664354628,128.057187654845));
#233185=CARTESIAN_POINT('Ctrl Pts',(207.466948700697,4.00218085216552,127.94573656235));
#233186=CARTESIAN_POINT('Ctrl Pts',(207.459191971722,3.92265050996814,127.834391101541));
#233187=CARTESIAN_POINT('Ctrl Pts',(207.451435242747,3.83838681773448,127.726250646596));
#233188=CARTESIAN_POINT('Ctrl Pts',(207.443678513772,3.74968088678163,127.621739636393));
#233189=CARTESIAN_POINT('Ctrl Pts',(207.435927455956,3.66103981118161,127.517305037071));
#233190=CARTESIAN_POINT('Ctrl Pts',(207.42817639814,3.56796321247351,127.416494898379));
#233191=CARTESIAN_POINT('Ctrl Pts',(207.420425340323,3.47078398382534,127.319702585546));
#233192=CARTESIAN_POINT('Ctrl Pts',(207.412678122975,3.37365290521867,127.222958231046));
#233193=CARTESIAN_POINT('Ctrl Pts',(207.404930905627,3.27242351943269,127.130228014992));
#233194=CARTESIAN_POINT('Ctrl Pts',(207.39718368828,3.16746701561529,127.041869984024));
#233195=CARTESIAN_POINT('Ctrl Pts',(207.389438629274,3.06253975223555,126.95353656923));
#233196=CARTESIAN_POINT('Ctrl Pts',(207.381693570268,2.95388773802827,126.869573164603));
#233197=CARTESIAN_POINT('Ctrl Pts',(207.373948511262,2.84191651249237,126.790298635169));
#233198=CARTESIAN_POINT('Ctrl Pts',(207.366203026905,2.72993913761875,126.711019752064));
#233199=CARTESIAN_POINT('Ctrl Pts',(207.358457542549,2.61464250564787,126.636430485188));
#233200=CARTESIAN_POINT('Ctrl Pts',(207.350712058193,2.49646231867335,126.566807201508));
#233201=CARTESIAN_POINT('Ctrl Pts',(207.348840169584,2.46790114216212,126.549981006311));
#233202=CARTESIAN_POINT('Ctrl Pts',(207.346968280974,2.43917167189546,126.533444654371));
#233203=CARTESIAN_POINT('Ctrl Pts',(207.345096392365,2.41028028844147,126.517201652278));
#233204=CARTESIAN_POINT('Origin',(210.,0.,130.804360617566));
#233205=CARTESIAN_POINT('',(177.987468637443,-4.44881802408841,134.718337674492));
#233206=CARTESIAN_POINT('Ctrl Pts',(177.987171124066,-4.4381842494261,134.71721777451));
#233207=CARTESIAN_POINT('Ctrl Pts',(177.917908154705,-4.66808213043419,
134.456454574234));
#233208=CARTESIAN_POINT('Ctrl Pts',(177.848867591835,-4.8807856187837,134.168285242348));
#233209=CARTESIAN_POINT('Ctrl Pts',(177.78566632542,-5.06704185329145,133.859359376894));
#233210=CARTESIAN_POINT('',(178.188375192211,-5.91592736650928,130.798890494443));
#233211=CARTESIAN_POINT('Ctrl Pts',(178.188375192211,-5.91592736650928,
130.798890494443));
#233212=CARTESIAN_POINT('Ctrl Pts',(178.121415174441,-5.90292116165263,
132.221415516948));
#233213=CARTESIAN_POINT('Ctrl Pts',(178.054455156671,-5.38193783986145,
133.652419557679));
#233214=CARTESIAN_POINT('Ctrl Pts',(177.987495138901,-4.44976524376727,
134.718437431289));
#233215=CARTESIAN_POINT('',(178.530363299101,-1.97902084214117,125.22872231614));
#233216=CARTESIAN_POINT('Ctrl Pts',(178.531594387824,-1.96435919885661,
125.223211676679));
#233217=CARTESIAN_POINT('Ctrl Pts',(178.524172743157,-2.11222423528786,
125.275254732254));
#233218=CARTESIAN_POINT('Ctrl Pts',(178.516751098491,-2.25823691125162,
125.333254551213));
#233219=CARTESIAN_POINT('Ctrl Pts',(178.509329453824,-2.40188156402355,
125.397060411835));
#233220=CARTESIAN_POINT('Ctrl Pts',(178.501916303098,-2.54536181804821,
125.460793247784));
#233221=CARTESIAN_POINT('Ctrl Pts',(178.494503152372,-2.6864791055858,125.530318748188));
#233222=CARTESIAN_POINT('Ctrl Pts',(178.487090001645,-2.82473377071421,
125.605436720538));
#233223=CARTESIAN_POINT('Ctrl Pts',(178.479683718601,-2.96286035412852,
125.68048510219));
#233224=CARTESIAN_POINT('Ctrl Pts',(178.472277435556,-3.09812926890283,
125.761115464114));
#233225=CARTESIAN_POINT('Ctrl Pts',(178.464871152512,-3.23006177761989,
125.847079964299));
#233226=CARTESIAN_POINT('Ctrl Pts',(178.457470116298,-3.36190082143372,
125.932983564681));
#233227=CARTESIAN_POINT('Ctrl Pts',(178.450069080084,-3.4904078540771,126.024213575878));
#233228=CARTESIAN_POINT('Ctrl Pts',(178.44266804387,-3.61512975619378,126.120476822212));
#233229=CARTESIAN_POINT('Ctrl Pts',(178.434930662265,-3.74551973448816,
126.221114820727));
#233230=CARTESIAN_POINT('Ctrl Pts',(178.427193280659,-3.87177211423748,
126.327254051388));
#233231=CARTESIAN_POINT('Ctrl Pts',(178.419455899053,-3.99340362608919,
126.438509263977));
#233232=CARTESIAN_POINT('Ctrl Pts',(178.412059409808,-4.10967631562484,
126.544862811636));
#233233=CARTESIAN_POINT('Ctrl Pts',(178.404662920563,-4.22172630043844,
126.65589090558));
#233234=CARTESIAN_POINT('Ctrl Pts',(178.397266431318,-4.32916618737662,
126.77121659775));
#233235=CARTESIAN_POINT('Ctrl Pts',(178.389869952312,-4.43660592557766,
126.886542130267));
#233236=CARTESIAN_POINT('Ctrl Pts',(178.382473473307,-4.53943532371603,
127.006164976397));
#233237=CARTESIAN_POINT('Ctrl Pts',(178.375076994301,-4.63730509265252,
127.129672598134));
#233238=CARTESIAN_POINT('Ctrl Pts',(178.367679065145,-4.73519404990068,
127.253204434731));
#233239=CARTESIAN_POINT('Ctrl Pts',(178.360281135988,-4.8281212100497,127.380622270841));
#233240=CARTESIAN_POINT('Ctrl Pts',(178.352883206831,-4.915778785888,127.511482015079));
#233241=CARTESIAN_POINT('Ctrl Pts',(178.345482366543,-5.00347085553144,
127.642393253447));
#233242=CARTESIAN_POINT('Ctrl Pts',(178.338081526255,-5.08588900471472,
127.776748786709));
#233243=CARTESIAN_POINT('Ctrl Pts',(178.330680685967,-5.16276990799104,
127.914077337394));
#233244=CARTESIAN_POINT('Ctrl Pts',(178.323271586729,-5.23973660633535,
128.05155913956));
#233245=CARTESIAN_POINT('Ctrl Pts',(178.31586248749,-5.3111535380145,128.192020258013));
#233246=CARTESIAN_POINT('Ctrl Pts',(178.308453388251,-5.37680400071853,
128.334966096564));
#233247=CARTESIAN_POINT('Ctrl Pts',(178.301039443423,-5.44249739916783,
128.478005422438));
#233248=CARTESIAN_POINT('Ctrl Pts',(178.293625498594,-5.5024166726957,128.623532362135));
#233249=CARTESIAN_POINT('Ctrl Pts',(178.286211553766,-5.55639422987409,
128.771034838277));
#233250=CARTESIAN_POINT('Ctrl Pts',(178.278787443269,-5.6104457986575,128.918739563197));
#233251=CARTESIAN_POINT('Ctrl Pts',(178.271363332772,-5.65853927118603,
129.068424878913));
#233252=CARTESIAN_POINT('Ctrl Pts',(178.263939222275,-5.70055742603375,
129.219565490431));
#233253=CARTESIAN_POINT('Ctrl Pts',(178.261616443294,-5.71370363216299,
129.266852803277));
#233254=CARTESIAN_POINT('Ctrl Pts',(178.259293664312,-5.72625552043617,
129.314282511711));
#233255=CARTESIAN_POINT('Ctrl Pts',(178.256970885331,-5.73821053949377,
129.361838393494));
#233256=CARTESIAN_POINT('Ctrl Pts',(178.247172129819,-5.78864336578615,
129.562455181601));
#233257=CARTESIAN_POINT('Ctrl Pts',(178.237373374307,-5.82857446158499,
129.765810079934));
#233258=CARTESIAN_POINT('Ctrl Pts',(178.227574618795,-5.85776135301491,
129.970956457734));
#233259=CARTESIAN_POINT('Ctrl Pts',(178.217994260587,-5.88629771913931,
130.171530477754));
#233260=CARTESIAN_POINT('Ctrl Pts',(178.20841390238,-5.90456354448122,130.373817290498));
#233261=CARTESIAN_POINT('Ctrl Pts',(178.198833544173,-5.9123765717479,130.576909883677));
#233262=CARTESIAN_POINT('Ctrl Pts',(178.195347434846,-5.91521958310856,
130.650811398412));
#233263=CARTESIAN_POINT('Ctrl Pts',(178.19186132552,-5.91667897563865,130.724819368433));
#233264=CARTESIAN_POINT('Ctrl Pts',(178.188375216193,-5.91674747022219,
130.798889226584));
#233265=CARTESIAN_POINT('Ctrl Pts',(178.183768748222,-3.73415024100118,
126.214801538512));
#233266=CARTESIAN_POINT('Ctrl Pts',(178.294473067275,-3.30324972789069,
125.864212903054));
#233267=CARTESIAN_POINT('Ctrl Pts',(178.40360148388,-2.80660255836622,125.563909715843));
#233268=CARTESIAN_POINT('Ctrl Pts',(178.502989322817,-2.18499290349215,
125.304971384407));
#233269=CARTESIAN_POINT('Ctrl Pts',(178.516732714955,-2.09380460320336,
125.26960931481));
#233270=CARTESIAN_POINT('Ctrl Pts',(178.52971317936,-2.00179946419882,125.236530746994));
#233271=CARTESIAN_POINT('Origin',(213.235140564004,0.,130.804360617566));
#233272=CARTESIAN_POINT('',(206.764859435946,-4.91824826123457,130.808496238813));
#233273=CARTESIAN_POINT('Ctrl Pts',(206.834782106149,-4.76405452823405,
129.582490119308));
#233274=CARTESIAN_POINT('Ctrl Pts',(206.827070043619,-4.79800979989384,
129.714881208167));
#233275=CARTESIAN_POINT('Ctrl Pts',(206.819357981088,-4.82644926951694,
129.84871625431));
#233276=CARTESIAN_POINT('Ctrl Pts',(206.811645918557,-4.84926402357277,
129.983494311653));
#233277=CARTESIAN_POINT('Ctrl Pts',(206.803848171462,-4.8723322600444,130.119769815232));
#233278=CARTESIAN_POINT('Ctrl Pts',(206.796050424368,-4.8896499380063,130.257009012014));
#233279=CARTESIAN_POINT('Ctrl Pts',(206.788252677274,-4.90115795633873,
130.394685441948));
#233280=CARTESIAN_POINT('Ctrl Pts',(206.78045493018,-4.91266597467115,130.532361871882));
#233281=CARTESIAN_POINT('Ctrl Pts',(206.772657183085,-4.9183643194193,130.67047511888));
#233282=CARTESIAN_POINT('Ctrl Pts',(206.764859435991,-4.91824826123525,
130.80849623801));
#233283=CARTESIAN_POINT('Ctrl Pts',(206.764859435946,-4.91824826123457,
130.808496238813));
#233284=CARTESIAN_POINT('Ctrl Pts',(206.755633759936,-4.91811095036783,
130.971791882044));
#233285=CARTESIAN_POINT('Ctrl Pts',(206.746408083927,-4.9098372427412,131.134736331661));
#233286=CARTESIAN_POINT('Ctrl Pts',(206.737182407917,-4.89355472835045,
131.296605661359));
#233287=CARTESIAN_POINT('Ctrl Pts',(206.727886086852,-4.87714753159103,
131.459714495655));
#233288=CARTESIAN_POINT('Ctrl Pts',(206.718589765787,-4.85260850573713,
131.621731650502));
#233289=CARTESIAN_POINT('Ctrl Pts',(206.709293444722,-4.82011683649341,
131.781937594102));
#233290=CARTESIAN_POINT('Ctrl Pts',(206.699922676766,-4.7873649671415,131.94342650053));
#233291=CARTESIAN_POINT('Ctrl Pts',(206.69055190881,-4.74653262850223,132.103075044456));
#233292=CARTESIAN_POINT('Ctrl Pts',(206.681181140855,-4.69785138332069,
132.260168105777));
#233293=CARTESIAN_POINT('Ctrl Pts',(206.680193264038,-4.69271935212153,
132.27672903163));
#233294=CARTESIAN_POINT('Ctrl Pts',(206.679205387222,-4.68750013448521,
132.293261576894));
#233295=CARTESIAN_POINT('Ctrl Pts',(206.678217510405,-4.68219403218519,
132.309764917902));
#233296=CARTESIAN_POINT('Ctrl Pts',(206.670443203729,-4.64043653180415,
132.439641469363));
#233297=CARTESIAN_POINT('Ctrl Pts',(206.662668897052,-4.59320493957362,
132.567985005214));
#233298=CARTESIAN_POINT('Ctrl Pts',(206.654894590376,-4.54062928664211,
132.694299437684));
#233299=CARTESIAN_POINT('Ctrl Pts',(206.647129865258,-4.48811843135327,
132.820458192059));
#233300=CARTESIAN_POINT('Ctrl Pts',(206.639365140141,-4.43027676906317,
132.944592461411));
#233301=CARTESIAN_POINT('Ctrl Pts',(206.631600415024,-4.36728419816986,
133.066220868536));
#233302=CARTESIAN_POINT('Ctrl Pts',(206.623843402325,-4.30435419549641,
133.187728466606));
#233303=CARTESIAN_POINT('Ctrl Pts',(206.616086389625,-4.23628364434482,
133.306734810711));
#233304=CARTESIAN_POINT('Ctrl Pts',(206.608329376926,-4.16330052534937,
133.422778421914));
#233305=CARTESIAN_POINT('Ctrl Pts',(206.600578214196,-4.09037244674563,
133.538734518553));
#233306=CARTESIAN_POINT('Ctrl Pts',(206.592827051467,-4.01253938183014,
133.651732000017));
#233307=CARTESIAN_POINT('Ctrl Pts',(206.585075888737,-3.93007506123518,
133.761334252139));
#233308=CARTESIAN_POINT('Ctrl Pts',(206.577328020864,-3.84764579449751,
133.870889914636));
#233309=CARTESIAN_POINT('Ctrl Pts',(206.569580152991,-3.76058942214285,
133.977052906525));
#233310=CARTESIAN_POINT('Ctrl Pts',(206.561832285118,-3.66922266005811,
134.079416057313));
#233311=CARTESIAN_POINT('Ctrl Pts',(206.554086038175,-3.577875012784,134.181757792739));
#233312=CARTESIAN_POINT('Ctrl Pts',(206.546339791231,-3.48221902964024,
134.280300976796));
#233313=CARTESIAN_POINT('Ctrl Pts',(206.538593544287,-3.38261107228556,
134.374672284095));
#233314=CARTESIAN_POINT('Ctrl Pts',(206.530847240371,-3.28300238233128,
134.469044285479));
#233315=CARTESIAN_POINT('Ctrl Pts',(206.523100936455,-3.17944194398242,
134.559244079983));
#233316=CARTESIAN_POINT('Ctrl Pts',(206.515354632539,-3.07232196606475,
134.644936199342));
#233317=CARTESIAN_POINT('Ctrl Pts',(206.507606594067,-2.96517800179731,
134.730647506916));
#233318=CARTESIAN_POINT('Ctrl Pts',(206.499858555595,-2.85447321715903,
134.811848886652));
#233319=CARTESIAN_POINT('Ctrl Pts',(206.492110517123,-2.74063145552457,
134.888246302485));
#233320=CARTESIAN_POINT('Ctrl Pts',(206.484354244035,-2.62666870285167,
134.964724913502));
#233321=CARTESIAN_POINT('Ctrl Pts',(206.476597970948,-2.50956263835897,
135.036389143314));
#233322=CARTESIAN_POINT('Ctrl Pts',(206.46884169786,-2.38976501336611,135.102989031769));
#233323=CARTESIAN_POINT('Ctrl Pts',(206.461081285113,-2.26990345028647,
135.169624465748));
#233324=CARTESIAN_POINT('Ctrl Pts',(206.453320872367,-2.14734781348686,
135.231189997141));
#233325=CARTESIAN_POINT('Ctrl Pts',(206.44556045962,-2.02257190409865,135.28748296201));
#233326=CARTESIAN_POINT('Ctrl Pts',(206.437787589017,-1.8975956908752,135.343866294457));
#233327=CARTESIAN_POINT('Ctrl Pts',(206.430014718413,-1.77039244561536,
135.394960000609));
#233328=CARTESIAN_POINT('Ctrl Pts',(206.422241847809,-1.64145412060007,
135.440610333928));
#233329=CARTESIAN_POINT('Ctrl Pts',(206.41475119407,-1.5171972796397,135.484603198007));
#233330=CARTESIAN_POINT('Ctrl Pts',(206.407260540331,-1.39132946298595,
135.523541019782));
#233331=CARTESIAN_POINT('Ctrl Pts',(206.399769886592,-1.26429990602564,
135.557331142419));
#233332=CARTESIAN_POINT('Ctrl Pts',(206.391995539368,-1.13245935939483,
135.592400998174));
#233333=CARTESIAN_POINT('Ctrl Pts',(206.384221192143,-0.998949706372701,
135.622036643276));
#233334=CARTESIAN_POINT('Ctrl Pts',(206.376446844919,-0.864258611065781,
135.646079332619));
#233335=CARTESIAN_POINT('Ctrl Pts',(206.368682078737,-0.72973350798047,
135.670092391946));
#233336=CARTESIAN_POINT('Ctrl Pts',(206.360917312556,-0.594030240801939,
135.688526141918));
#233337=CARTESIAN_POINT('Ctrl Pts',(206.353152546374,-0.457651051086741,
135.70127174377));
#233338=CARTESIAN_POINT('Ctrl Pts',(206.345395492141,-0.321407312868765,
135.71400468672));
#233339=CARTESIAN_POINT('Ctrl Pts',(206.337638437907,-0.184489374829276,
135.721060688077));
#233340=CARTESIAN_POINT('Ctrl Pts',(206.329881383673,-0.0474087266159011,
135.722382117635));
#233341=CARTESIAN_POINT('Ctrl Pts',(206.322130178985,0.0895685499512351,
135.723702550711));
#233342=CARTESIAN_POINT('Ctrl Pts',(206.314378974297,0.226707903104169,
135.719297015699));
#233343=CARTESIAN_POINT('Ctrl Pts',(206.306627769608,0.363494034138324,
135.709159813216));
#233344=CARTESIAN_POINT('Ctrl Pts',(206.298879859279,0.500222029349606,
135.699026919171));
#233345=CARTESIAN_POINT('Ctrl Pts',(206.29113194895,0.636596711948773,135.68316723157));
#233346=CARTESIAN_POINT('Ctrl Pts',(206.283384038621,0.772104320862591,
135.661627130761));
#233347=CARTESIAN_POINT('Ctrl Pts',(206.275637748924,0.907583585626675,
135.640091535498));
#233348=CARTESIAN_POINT('Ctrl Pts',(206.267891459227,1.04219575158091,135.612877951706));
#233349=CARTESIAN_POINT('Ctrl Pts',(206.26014516953,1.17543410337159,135.580084408902));
#233350=CARTESIAN_POINT('Ctrl Pts',(206.252398822603,1.30867343952879,135.547290623819));
#233351=CARTESIAN_POINT('Ctrl Pts',(206.244652475676,1.44053856163545,135.508916890901));
#233352=CARTESIAN_POINT('Ctrl Pts',(206.236906128749,1.57053522864704,135.465111861526));
#233353=CARTESIAN_POINT('Ctrl Pts',(206.229158047049,1.70056100805719,135.421297022135));
#233354=CARTESIAN_POINT('Ctrl Pts',(206.221409965348,1.8287171293106,135.372048590765));
#233355=CARTESIAN_POINT('Ctrl Pts',(206.213661883648,1.95452711044093,135.317564228866));
#233356=CARTESIAN_POINT('Ctrl Pts',(206.20590556723,2.08047080333817,135.263021960589));
#233357=CARTESIAN_POINT('Ctrl Pts',(206.198149250812,2.2040630157501,135.203232801142));
#233358=CARTESIAN_POINT('Ctrl Pts',(206.190392934394,2.32484926327892,135.138441715738));
#233359=CARTESIAN_POINT('Ctrl Pts',(206.182632478194,2.44569997811104,135.073616049356));
#233360=CARTESIAN_POINT('Ctrl Pts',(206.174872021993,2.5637414075819,135.003783336419));
#233361=CARTESIAN_POINT('Ctrl Pts',(206.167111565792,2.67854694058481,134.929232657955));
#233362=CARTESIAN_POINT('Ctrl Pts',(206.159338651962,2.79353676750179,134.8545623055));
#233363=CARTESIAN_POINT('Ctrl Pts',(206.151565738131,2.90527999882711,134.775159079624));
#233364=CARTESIAN_POINT('Ctrl Pts',(206.143792824301,3.01338136800174,134.691353773397));
#233365=CARTESIAN_POINT('Ctrl Pts',(206.136302637127,3.1175507318328,134.61059674412));
#233366=CARTESIAN_POINT('Ctrl Pts',(206.128812449953,3.21833832869957,134.525752506211));
#233367=CARTESIAN_POINT('Ctrl Pts',(206.12132226278,3.31542344251232,134.43714886619));
#233368=CARTESIAN_POINT('Ctrl Pts',(206.113547928467,3.41619156940981,134.345183965593));
#233369=CARTESIAN_POINT('Ctrl Pts',(206.105773594154,3.51328995165438,134.248877485937));
#233370=CARTESIAN_POINT('Ctrl Pts',(206.097999259841,3.60632143845033,134.148553905203));
#233371=CARTESIAN_POINT('Ctrl Pts',(206.090234506665,3.69923827267255,134.048353963863));
#233372=CARTESIAN_POINT('Ctrl Pts',(206.082469753489,3.78809792067824,133.944147055788));
#233373=CARTESIAN_POINT('Ctrl Pts',(206.074705000313,3.87253733969881,133.836296899076));
#233374=CARTESIAN_POINT('Ctrl Pts',(206.066947959165,3.95689289267469,133.72855386018));
#233375=CARTESIAN_POINT('Ctrl Pts',(206.059190918017,4.03683671393217,133.617175079492));
#233376=CARTESIAN_POINT('Ctrl Pts',(206.051433876869,4.11204384499684,133.502559735371));
#233377=CARTESIAN_POINT('Ctrl Pts',(206.043682685331,4.18719426211104,133.388030823066));
#233378=CARTESIAN_POINT('Ctrl Pts',(206.035931493794,4.2576148851709,133.270270530956));
#233379=CARTESIAN_POINT('Ctrl Pts',(206.028180302257,4.32302238761605,133.14970931204));
#233380=CARTESIAN_POINT('Ctrl Pts',(206.020432405131,4.38840209056044,133.029199334061));
#233381=CARTESIAN_POINT('Ctrl Pts',(206.012684508006,4.44877272459587,132.90589113992));
#233382=CARTESIAN_POINT('Ctrl Pts',(206.00493661088,4.50389561038913,132.780242039417));
#233383=CARTESIAN_POINT('Ctrl Pts',(205.997190334417,4.55900696588485,132.654619221492));
#233384=CARTESIAN_POINT('Ctrl Pts',(205.989444057953,4.60887259954457,132.52665682896));
#233385=CARTESIAN_POINT('Ctrl Pts',(205.98169778149,4.65330109429353,132.396834161568));
#233386=CARTESIAN_POINT('Ctrl Pts',(205.973951447814,4.69772991718062,132.267010535338));
#233387=CARTESIAN_POINT('Ctrl Pts',(205.966205114138,4.73672139443581,132.135326976735));
#233388=CARTESIAN_POINT('Ctrl Pts',(205.958458780463,4.77013344123859,132.002279652926));
#233389=CARTESIAN_POINT('Ctrl Pts',(205.950710712019,4.80355297056946,131.869202533566));
#233390=CARTESIAN_POINT('Ctrl Pts',(205.942962643575,4.83139048788632,131.734761420386));
#233391=CARTESIAN_POINT('Ctrl Pts',(205.935214575131,4.85355474113685,131.599464030518));
#233392=CARTESIAN_POINT('Ctrl Pts',(205.927458271901,4.87574255095105,131.464022844171));
#233393=CARTESIAN_POINT('Ctrl Pts',(205.919701968672,4.89224498852538,131.327723949617));
#233394=CARTESIAN_POINT('Ctrl Pts',(205.911945665443,4.90302249002199,131.191082125681));
#233395=CARTESIAN_POINT('Ctrl Pts',(205.904185222415,4.91380574383149,131.054367371435));
#233396=CARTESIAN_POINT('Ctrl Pts',(205.896424779388,4.91885795864703,130.917309713606));
#233397=CARTESIAN_POINT('Ctrl Pts',(205.88866433636,4.91819175271269,130.780424326105));
#233398=CARTESIAN_POINT('Ctrl Pts',(205.880891435541,4.91752447732209,130.643319197341));
#233399=CARTESIAN_POINT('Ctrl Pts',(205.873118534722,4.91112045540052,130.506387282292));
#233400=CARTESIAN_POINT('Ctrl Pts',(205.865345633904,4.89904434121163,130.370139930193));
#233401=CARTESIAN_POINT('Ctrl Pts',(205.857855302258,4.8874072314151,130.238845594031));
#233402=CARTESIAN_POINT('Ctrl Pts',(205.850364970613,4.87050330540731,130.108187218426));
#233403=CARTESIAN_POINT('Ctrl Pts',(205.842874638967,4.84843500802732,129.978611844975));
#233404=CARTESIAN_POINT('Ctrl Pts',(205.835100308635,4.82552998301369,129.844123573455));
#233405=CARTESIAN_POINT('Ctrl Pts',(205.827325978302,4.79698868437903,129.710376028441));
#233406=CARTESIAN_POINT('Ctrl Pts',(205.81955164797,4.76286943415894,129.577878731987));
#233407=CARTESIAN_POINT('Ctrl Pts',(205.811786898866,4.72879223313221,129.445544727644));
#233408=CARTESIAN_POINT('Ctrl Pts',(205.804022149762,4.68915085502848,129.31445828105));
#233409=CARTESIAN_POINT('Ctrl Pts',(205.796257400658,4.64405507193892,129.185121428534));
#233410=CARTESIAN_POINT('Ctrl Pts',(205.788500363668,4.59900407893947,129.055913036128));
#233411=CARTESIAN_POINT('Ctrl Pts',(205.780743326677,4.54850958977095,128.928451146412));
#233412=CARTESIAN_POINT('Ctrl Pts',(205.772986289687,4.49273179575291,128.803224921535));
#233413=CARTESIAN_POINT('Ctrl Pts',(205.765235102389,4.43699606456529,128.67809313154));
#233414=CARTESIAN_POINT('Ctrl Pts',(205.757483915091,4.37598511729972,128.555194006304));
#233415=CARTESIAN_POINT('Ctrl Pts',(205.749732727793,4.30990796060895,128.434998586643));
#233416=CARTESIAN_POINT('Ctrl Pts',(205.741984835016,4.24385888898434,128.314854254173));
#233417=CARTESIAN_POINT('Ctrl Pts',(205.73423694224,4.17274807866374,128.197411683559));
#233418=CARTESIAN_POINT('Ctrl Pts',(205.726489049463,4.09683126462683,128.083118869452));
#233419=CARTESIAN_POINT('Ctrl Pts',(205.718742777414,4.0209303311019,127.968849963467));
#233420=CARTESIAN_POINT('Ctrl Pts',(205.710996505366,3.94022560970842,127.85772982891));
#233421=CARTESIAN_POINT('Ctrl Pts',(205.703250233317,3.85501688262898,127.750178583511));
#233422=CARTESIAN_POINT('Ctrl Pts',(205.695503904118,3.76980752690164,127.642626544626));
#233423=CARTESIAN_POINT('Ctrl Pts',(205.68775757492,3.68009434196701,127.538643753886));
#233424=CARTESIAN_POINT('Ctrl Pts',(205.680011245721,3.58621796636794,127.438617941692));
#233425=CARTESIAN_POINT('Ctrl Pts',(205.672263181812,3.49232056812825,127.338569729755));
#233426=CARTESIAN_POINT('Ctrl Pts',(205.664515117904,3.39425839154965,127.242480544672));
#233427=CARTESIAN_POINT('Ctrl Pts',(205.656767053995,3.29240926887433,127.150701592872));
#233428=CARTESIAN_POINT('Ctrl Pts',(205.649010755368,3.19045189995416,127.058825097503));
#233429=CARTESIAN_POINT('Ctrl Pts',(205.641254456741,3.0846998358618,126.971268248513));
#233430=CARTESIAN_POINT('Ctrl Pts',(205.633498158114,2.97556478881364,126.888342582614));
#233431=CARTESIAN_POINT('Ctrl Pts',(205.625737719733,2.86637149332416,126.805372656956));
#233432=CARTESIAN_POINT('Ctrl Pts',(205.617977281351,2.75379193784736,126.727039062836));
#233433=CARTESIAN_POINT('Ctrl Pts',(205.61021684297,2.63826637271815,126.653609648273));
#233434=CARTESIAN_POINT('Ctrl Pts',(205.602443946826,2.52255535542982,126.580062358127));
#233435=CARTESIAN_POINT('Ctrl Pts',(205.594671050682,2.40388921667307,126.511435175415));
#233436=CARTESIAN_POINT('Ctrl Pts',(205.586898154538,2.2827331157452,126.447950101467));
#233437=CARTESIAN_POINT('Ctrl Pts',(205.579407774743,2.16598059601619,126.386772477791));
#233438=CARTESIAN_POINT('Ctrl Pts',(205.571917394949,2.04691625263489,126.330369789491));
#233439=CARTESIAN_POINT('Ctrl Pts',(205.564427015154,1.92597157701165,126.278897486897));
#233440=CARTESIAN_POINT('Ctrl Pts',(205.556652678921,1.80044195106122,126.225473895836));
#233441=CARTESIAN_POINT('Ctrl Pts',(205.548878342688,1.67248897498338,126.177192652376));
#233442=CARTESIAN_POINT('Ctrl Pts',(205.541104006456,1.54257284960153,126.134280097257));
#233443=CARTESIAN_POINT('Ctrl Pts',(205.533339251373,1.412816833816,126.091420427889));
#233444=CARTESIAN_POINT('Ctrl Pts',(205.525574496289,1.28110285028441,126.053916403621));
#233445=CARTESIAN_POINT('Ctrl Pts',(205.517809741206,1.14791261180821,126.021947032549));
#233446=CARTESIAN_POINT('Ctrl Pts',(205.510052698165,1.01485465937561,125.990009413817));
#233447=CARTESIAN_POINT('Ctrl Pts',(205.502295655124,0.88032374757524,125.963595599504));
#233448=CARTESIAN_POINT('Ctrl Pts',(205.494538612083,0.744818010538801,
125.942835219743));
#233449=CARTESIAN_POINT('Ctrl Pts',(205.48678741867,0.609414459097139,125.922090495495));
#233450=CARTESIAN_POINT('Ctrl Pts',(205.479036225256,0.473037930525041,
125.906990778956));
#233451=CARTESIAN_POINT('Ctrl Pts',(205.471285031842,0.33619769877146,125.897614835498));
#233452=CARTESIAN_POINT('Ctrl Pts',(205.463537132872,0.199415627413407,
125.888242877042));
#233453=CARTESIAN_POINT('Ctrl Pts',(205.455789233902,0.0621706340948198,
125.884589879799));
#233454=CARTESIAN_POINT('Ctrl Pts',(205.448041334933,-0.0750221388880692,
125.88668283825));
#233455=CARTESIAN_POINT('Ctrl Pts',(205.440295056645,-0.212186214308715,
125.888775358903));
#233456=CARTESIAN_POINT('Ctrl Pts',(205.432548778357,-0.349297700448874,
125.896611438603));
#233457=CARTESIAN_POINT('Ctrl Pts',(205.424802500068,-0.485841100123671,
125.910165945515));
#233458=CARTESIAN_POINT('Ctrl Pts',(205.41705616459,-0.622385507893228,
125.9237205525));
#233459=CARTESIAN_POINT('Ctrl Pts',(205.409309829111,-0.758361431775545,
125.942993632321));
#233460=CARTESIAN_POINT('Ctrl Pts',(205.401563493633,-0.89325853914859,
125.967908173394));
#233461=CARTESIAN_POINT('Ctrl Pts',(205.393815423409,-1.02818585590989,
125.992828293927));
#233462=CARTESIAN_POINT('Ctrl Pts',(205.386067353186,-1.16203349102794,
126.02339231868));
#233463=CARTESIAN_POINT('Ctrl Pts',(205.378319282963,-1.29430173647038,
126.059472201863));
#233464=CARTESIAN_POINT('Ctrl Pts',(205.370562978002,-1.42671055811762,
126.095590431159));
#233465=CARTESIAN_POINT('Ctrl Pts',(205.36280667304,-1.55753625913267,126.137236126444));
#233466=CARTESIAN_POINT('Ctrl Pts',(205.355050368079,-1.68629419381508,
126.184231295306));
#233467=CARTESIAN_POINT('Ctrl Pts',(205.347289923343,-1.81512085051228,
126.231251546915));
#233468=CARTESIAN_POINT('Ctrl Pts',(205.339529478607,-1.94187718064387,
126.283626812052));
#233469=CARTESIAN_POINT('Ctrl Pts',(205.331769033871,-2.06609986951013,
126.341131473582));
#233470=CARTESIAN_POINT('Ctrl Pts',(205.323996131401,-2.19052197132574,
126.398728446543));
#233471=CARTESIAN_POINT('Ctrl Pts',(205.316223228931,-2.31240195646745,
126.461471091301));
#233472=CARTESIAN_POINT('Ctrl Pts',(205.308450326461,-2.43130161847012,
126.52908805286));
#233473=CARTESIAN_POINT('Ctrl Pts',(205.300960014754,-2.54587857780558,
126.594246739811));
#233474=CARTESIAN_POINT('Ctrl Pts',(205.293469703048,-2.65768789450607,
126.663931314284));
#233475=CARTESIAN_POINT('Ctrl Pts',(205.285979391341,-2.7663655623862,126.737862783097));
#233476=CARTESIAN_POINT('Ctrl Pts',(205.278237672039,-2.87869092774278,
126.814275715097));
#233477=CARTESIAN_POINT('Ctrl Pts',(205.270495952738,-2.98803353029666,
126.895472526408));
#233478=CARTESIAN_POINT('Ctrl Pts',(205.262754233436,-3.09395614481765,
126.981191979323));
#233479=CARTESIAN_POINT('Ctrl Pts',(205.255024754641,-3.19971128407027,
127.066775900384));
#233480=CARTESIAN_POINT('Ctrl Pts',(205.247295275847,-3.30205689954337,
127.156867976875));
#233481=CARTESIAN_POINT('Ctrl Pts',(205.239565797052,-3.40058421415425,
127.251163456565));
#233482=CARTESIAN_POINT('Ctrl Pts',(205.231843383955,-3.4990214626426,127.345372738552));
#233483=CARTESIAN_POINT('Ctrl Pts',(205.224120970858,-3.59364706915702,
127.443777510556));
#233484=CARTESIAN_POINT('Ctrl Pts',(205.216398557761,-3.68408468413249,
127.546032349475));
#233485=CARTESIAN_POINT('Ctrl Pts',(205.208681492833,-3.77445966639361,
127.648216371643));
#233486=CARTESIAN_POINT('Ctrl Pts',(205.200964427906,-3.86065216668493,
127.75424486186));
#233487=CARTESIAN_POINT('Ctrl Pts',(205.193247362978,-3.94232245691661,
127.863735393538));
#233488=CARTESIAN_POINT('Ctrl Pts',(205.185533932859,-4.02395427969229,
127.97317435417));
#233489=CARTESIAN_POINT('Ctrl Pts',(205.177820502739,-4.1010678957911,128.086071795385));
#233490=CARTESIAN_POINT('Ctrl Pts',(205.17010707262,-4.17336396541682,128.202012394391));
#233491=CARTESIAN_POINT('Ctrl Pts',(205.162394028974,-4.24565641272213,
128.317947184313));
#233492=CARTESIAN_POINT('Ctrl Pts',(205.154680985329,-4.31313157631286,
128.436924499339));
#233493=CARTESIAN_POINT('Ctrl Pts',(205.146967941683,-4.37553364940197,
128.558500349105));
#233494=CARTESIAN_POINT('Ctrl Pts',(205.139255293534,-4.43793252273594,
128.680069964896));
#233495=CARTESIAN_POINT('Ctrl Pts',(205.131542645386,-4.49525864776658,
128.804237496571));
#233496=CARTESIAN_POINT('Ctrl Pts',(205.123829997237,-4.54730272990832,
128.930535400245));
#233497=CARTESIAN_POINT('Ctrl Pts',(205.116113219495,-4.59937467808288,
129.056900927775));
#233498=CARTESIAN_POINT('Ctrl Pts',(205.108396441753,-4.64615878721881,
129.185398739042));
#233499=CARTESIAN_POINT('Ctrl Pts',(205.100679664011,-4.68749433319855,
129.315542314773));
#233500=CARTESIAN_POINT('Ctrl Pts',(205.0954453069,-4.71553259168844,129.403819828246));
#233501=CARTESIAN_POINT('Ctrl Pts',(205.090210949789,-4.74106497151865,
129.49285418659));
#233502=CARTESIAN_POINT('Ctrl Pts',(205.084976592678,-4.76405452823405,
129.582490119308));
#233503=CARTESIAN_POINT('Ctrl Pts',(210.579426101437,-2.14555810197798,
126.384433368448));
#233504=CARTESIAN_POINT('Ctrl Pts',(210.533016425084,-2.88204635455982,
126.741945114569));
#233505=CARTESIAN_POINT('Ctrl Pts',(210.440198811428,-4.16073755837059,
127.832228156677));
#233506=CARTESIAN_POINT('Ctrl Pts',(210.254565323169,-5.41774734084591,
130.983824311839));
#233507=CARTESIAN_POINT('Ctrl Pts',(210.022525636658,-3.70466367662459,
135.280954889074));
#233508=CARTESIAN_POINT('Ctrl Pts',(209.744078012845,1.77278938863763,136.341871604603));
#233509=CARTESIAN_POINT('Ctrl Pts',(209.465630389032,5.61248518735455,132.305536381355));
#233510=CARTESIAN_POINT('Ctrl Pts',(209.187182765219,4.2990952821384,126.894094626803));
#233511=CARTESIAN_POINT('Ctrl Pts',(208.908735141406,-0.967335548355457,
125.073681250508));
#233512=CARTESIAN_POINT('Ctrl Pts',(208.630287517594,-5.34357155608916,
128.520706403956));
#233513=CARTESIAN_POINT('Ctrl Pts',(208.351839893781,-4.80999390579215,
134.065650134797));
#233514=CARTESIAN_POINT('Ctrl Pts',(208.073392269968,0.144086686833323,
136.613971320579));
#233515=CARTESIAN_POINT('Ctrl Pts',(207.794944646155,4.96557142732685,133.823362329787));
#233516=CARTESIAN_POINT('Ctrl Pts',(207.516497022342,5.22403776314189,128.258534510045));
#233517=CARTESIAN_POINT('Ctrl Pts',(207.238049398529,0.681816090004523,
125.033145533949));
#233518=CARTESIAN_POINT('Ctrl Pts',(206.959601774716,-4.48693345015888,
127.111248278652));
#233519=CARTESIAN_POINT('Ctrl Pts',(206.681154150904,-5.53242507739068,
132.583126545744));
#233520=CARTESIAN_POINT('Ctrl Pts',(206.40270652709,-1.49388053201802,136.420413394932));
#233521=CARTESIAN_POINT('Ctrl Pts',(206.124258903278,3.91746311099657,135.0968180907));
#233522=CARTESIAN_POINT('Ctrl Pts',(205.845811279465,5.72885172159717,129.828666190814));
#233523=CARTESIAN_POINT('Ctrl Pts',(205.567363655652,2.27570431130586,125.457128678938));
#233524=CARTESIAN_POINT('Ctrl Pts',(205.288916031839,-3.26870357308214,
125.999436687584));
#233525=CARTESIAN_POINT('Ctrl Pts',(205.010468408026,-5.80933288384994,
130.9572347388));
#233526=CARTESIAN_POINT('Ctrl Pts',(204.732020784213,-3.01146890392974,
135.774549108008));
#233527=CARTESIAN_POINT('Ctrl Pts',(204.4535731604,2.5537877891123,136.024502973214));
#233528=CARTESIAN_POINT('Ctrl Pts',(204.175125536587,5.77223831170541,131.477401078575));
#233529=CARTESIAN_POINT('Ctrl Pts',(203.896677912775,3.6862837897924,126.311807855303));
#233530=CARTESIAN_POINT('Ctrl Pts',(203.618230288961,-1.78718543642468,
125.274651160291));
#233531=CARTESIAN_POINT('Ctrl Pts',(203.339782665149,-5.61831856260093,
129.319027308227));
#233532=CARTESIAN_POINT('Ctrl Pts',(203.061335041336,-4.28649139606962,
134.728352208566));
#233533=CARTESIAN_POINT('Ctrl Pts',(202.782887417523,0.984411954691954,
136.531720532469));
#233534=CARTESIAN_POINT('Ctrl Pts',(202.50443979371,5.3506888113544,133.071924892697));
#233535=CARTESIAN_POINT('Ctrl Pts',(202.225992169897,4.79994404549834,127.528348460205));
#233536=CARTESIAN_POINT('Ctrl Pts',(201.947544546084,-0.161714807569177,
124.995267158526));
#233537=CARTESIAN_POINT('Ctrl Pts',(201.669096922271,-4.97476565284641,
127.800458955558));
#233538=CARTESIAN_POINT('Ctrl Pts',(201.390649298458,-5.21624989388704,
133.366089631302));
#233539=CARTESIAN_POINT('Ctrl Pts',(201.112201674645,-0.664255310463968,
136.577616490799));
#233540=CARTESIAN_POINT('Ctrl Pts',(200.833754050833,4.49815745262305,134.483803242045));
#233541=CARTESIAN_POINT('Ctrl Pts',(200.55530642702,5.52698326394509,129.008761972148));
#233542=CARTESIAN_POINT('Ctrl Pts',(200.276858803207,1.47678146385132,125.183788137525));
#233543=CARTESIAN_POINT('Ctrl Pts',(199.998411179394,-3.93051035674001,
126.523845831826));
#233544=CARTESIAN_POINT('Ctrl Pts',(199.719963555581,-5.7258551755912,131.79748749945));
#233545=CARTESIAN_POINT('Ctrl Pts',(199.441515931768,-2.25941881165118,
136.158494079568));
#233546=CARTESIAN_POINT('Ctrl Pts',(199.163068307955,3.28331306145151,135.599313572066));
#233547=CARTESIAN_POINT('Ctrl Pts',(198.884620684142,5.80884062984016,130.633805545853));
#233548=CARTESIAN_POINT('Ctrl Pts',(198.606173060329,2.99632743704681,125.825029298466));
#233549=CARTESIAN_POINT('Ctrl Pts',(198.327725436517,-2.56966429165962,
125.592015279473));
#233550=CARTESIAN_POINT('Ctrl Pts',(198.049277812704,-5.77426007141042,
130.148891988961));
#233551=CARTESIAN_POINT('Ctrl Pts',(197.770830188891,-3.6725929338218,135.308112346714));
#233552=CARTESIAN_POINT('Ctrl Pts',(197.492382565078,1.80400769380988,136.328604885883));
#233553=CARTESIAN_POINT('Ctrl Pts',(197.213934941265,5.62281338150559,132.272586816804));
#233554=CARTESIAN_POINT('Ctrl Pts',(196.935487317452,4.27452826130232,126.867340597462));
#233555=CARTESIAN_POINT('Ctrl Pts',(196.657039693639,-1.00183950872307,
125.080023442474));
#233556=CARTESIAN_POINT('Ctrl Pts',(196.378592069827,-5.35756571281285,
128.553092501978));
#233557=CARTESIAN_POINT('Ctrl Pts',(196.100144446013,-4.78995075846325,
134.094966979145));
#233558=CARTESIAN_POINT('Ctrl Pts',(195.821696822201,0.179394940810534,
136.612934965078));
#233559=CARTESIAN_POINT('Ctrl Pts',(195.543249198387,4.98388545340951,133.79310689028));
#233560=CARTESIAN_POINT('Ctrl Pts',(195.264801574575,5.20842871066526,128.22676699923));
#233561=CARTESIAN_POINT('Ctrl Pts',(194.986353950762,0.64668042870769,125.029109720981));
#233562=CARTESIAN_POINT('Ctrl Pts',(194.70790632695,-4.50933557513701,127.138625880003));
#233563=CARTESIAN_POINT('Ctrl Pts',(194.429458703136,-5.52149247872048,
132.616773181746));
#233564=CARTESIAN_POINT('Ctrl Pts',(194.151011079324,-1.4596675342632,136.429401878284));
#233565=CARTESIAN_POINT('Ctrl Pts',(193.87256345551,3.9435205654586,135.072892454764));
#233566=CARTESIAN_POINT('Ctrl Pts',(193.594115831698,5.72280591721378,129.793810802232));
#233567=CARTESIAN_POINT('Ctrl Pts',(193.315668207884,2.24311220566103,125.443375061888));
#233568=CARTESIAN_POINT('Ctrl Pts',(193.037220584072,-3.29789204077089,
126.019423148508));
#233569=CARTESIAN_POINT('Ctrl Pts',(192.758772960259,-5.80829461271728,
130.992595012001));
#233570=CARTESIAN_POINT('Ctrl Pts',(192.480325336446,-2.98115818654302,
135.792788662769));
#233571=CARTESIAN_POINT('Ctrl Pts',(192.201877712633,2.58551697539033,136.008860638253));
#233572=CARTESIAN_POINT('Ctrl Pts',(191.92343008882,5.77622834646622,131.442251348686));
#233573=CARTESIAN_POINT('Ctrl Pts',(191.644982465007,3.658868051582,126.289451639914));
#233574=CARTESIAN_POINT('Ctrl Pts',(191.366534841194,-1.82081323706467,
125.285632716038));
#233575=CARTESIAN_POINT('Ctrl Pts',(191.088087217381,-5.6272561125207,129.35325512882));
#233576=CARTESIAN_POINT('Ctrl Pts',(190.809639593569,-4.26252552731426,
134.754372595315));
#233577=CARTESIAN_POINT('Ctrl Pts',(190.531191969755,1.01925778154541,136.525622023071));
#233578=CARTESIAN_POINT('Ctrl Pts',(190.252744345943,5.36439298267566,133.039311718326));
#233579=CARTESIAN_POINT('Ctrl Pts',(189.974296722129,4.77991309789331,127.499190535413));
#233580=CARTESIAN_POINT('Ctrl Pts',(189.695849098317,-0.197073412116412,
124.996359191464));
#233581=CARTESIAN_POINT('Ctrl Pts',(189.417401474504,-4.99295908396257,
127.830797421458));
#233582=CARTESIAN_POINT('Ctrl Pts',(189.138953850692,-5.20055927725872,
133.397794962038));
#233583=CARTESIAN_POINT('Ctrl Pts',(188.860506226878,-0.629099556198964,
136.581553036358));
#233584=CARTESIAN_POINT('Ctrl Pts',(188.582058603065,4.52047192378579,134.456353509349));
#233585=CARTESIAN_POINT('Ctrl Pts',(188.303610979253,5.51595054314194,128.975150924561));
#233586=CARTESIAN_POINT('Ctrl Pts',(188.02516335544,1.44254008251539,125.174902685784));
#233587=CARTESIAN_POINT('Ctrl Pts',(187.746715731627,-3.95649424194195,
126.547851272005));
#233588=CARTESIAN_POINT('Ctrl Pts',(187.468268107814,-5.71970364354381,
131.832324004755));
#233589=CARTESIAN_POINT('Ctrl Pts',(187.189820484001,-2.22678481978599,
136.172148603481));
#233590=CARTESIAN_POINT('Ctrl Pts',(186.911372860188,3.312440468869,135.579238274173));
#233591=CARTESIAN_POINT('Ctrl Pts',(186.632925236375,5.80769478834652,130.598448644184));
#233592=CARTESIAN_POINT('Ctrl Pts',(186.354477612562,2.96596131899707,125.806882058373));
#233593=CARTESIAN_POINT('Ctrl Pts',(186.076029988749,-2.60134570724499,
125.607754128061));
#233594=CARTESIAN_POINT('Ctrl Pts',(185.797582364937,-5.7781431113317,130.184053693262));
#233595=CARTESIAN_POINT('Ctrl Pts',(185.519134741124,-3.64510927408837,
135.33038501822));
#233596=CARTESIAN_POINT('Ctrl Pts',(185.240687117311,1.83760191255446,136.317521027561));
#233597=CARTESIAN_POINT('Ctrl Pts',(184.962239493498,5.63164671340385,132.238331952975));
#233598=CARTESIAN_POINT('Ctrl Pts',(184.683791869685,4.25048330587202,126.841393274542));
#233599=CARTESIAN_POINT('Ctrl Pts',(184.405344245872,-1.03666661210287,
125.086227982629));
#233600=CARTESIAN_POINT('Ctrl Pts',(184.126896622059,-5.37117055753467,
128.585747235914));
#233601=CARTESIAN_POINT('Ctrl Pts',(183.848448998247,-4.7698311568614,134.124063801647));
#233602=CARTESIAN_POINT('Ctrl Pts',(183.570001374433,0.214750057761129,
136.611735317726));
#233603=CARTESIAN_POINT('Ctrl Pts',(183.291553750621,5.00198646042476,133.762713190383));
#233604=CARTESIAN_POINT('Ctrl Pts',(183.013106126807,5.19264166658148,128.195109572179));
#233605=CARTESIAN_POINT('Ctrl Pts',(182.734658502995,0.611512855797894,
125.025280195685));
#233606=CARTESIAN_POINT('Ctrl Pts',(182.456210879182,-4.53156639540017,
127.166143403126));
#233607=CARTESIAN_POINT('Ctrl Pts',(182.177763255369,-5.5103575085511,132.650350493844));
#233608=CARTESIAN_POINT('Ctrl Pts',(181.899315631556,-1.42539926727337,
136.438183069882));
#233609=CARTESIAN_POINT('Ctrl Pts',(181.620868007743,3.96943126600311,135.048808039769));
#233610=CARTESIAN_POINT('Ctrl Pts',(181.34242038393,5.71654838332065,129.758993181434));
#233611=CARTESIAN_POINT('Ctrl Pts',(181.063972760118,2.21043680528058,125.429819927867));
#233612=CARTESIAN_POINT('Ctrl Pts',(180.785525136304,-3.32695821097111,
126.039587007222));
#233613=CARTESIAN_POINT('Ctrl Pts',(180.507077512492,-5.80704116228462,
131.027948262352));
#233614=CARTESIAN_POINT('Ctrl Pts',(180.228629888679,-2.95073697519064,
135.810843394787));
#233615=CARTESIAN_POINT('Ctrl Pts',(179.950182264866,2.61715034058839,135.993025435236));
#233616=CARTESIAN_POINT('Ctrl Pts',(179.671734641053,5.78000434826875,131.407077988614));
#233617=CARTESIAN_POINT('Ctrl Pts',(179.39328701724,3.63131672880039,126.26726272238));
#233618=CARTESIAN_POINT('Ctrl Pts',(179.114839393428,-1.8543735647511,125.296818772266));
#233619=CARTESIAN_POINT('Ctrl Pts',(178.836391769614,-5.63598514348121,
129.387536719606));
#233620=CARTESIAN_POINT('Ctrl Pts',(178.557944145802,-4.23840170853308,
134.780246613475));
#233621=CARTESIAN_POINT('Ctrl Pts',(178.279496521988,1.05406583912245,136.519311509933));
#233622=CARTESIAN_POINT('Ctrl Pts',(178.001048898175,5.3778983746034,133.006615727177));
#233623=CARTESIAN_POINT('Ctrl Pts',(177.722601274363,4.75970502876524,127.470155084831));
#233624=CARTESIAN_POINT('Ctrl Pts',(177.44415365055,-0.232424713990654,
124.997666442073));
#233625=CARTESIAN_POINT('Ctrl Pts',(177.165706026737,-5.01096749916768,
127.861246073811));
#233626=CARTESIAN_POINT('Ctrl Pts',(176.887258402924,-5.18467595198119,
133.429404192122));
#233627=CARTESIAN_POINT('Ctrl Pts',(176.608810779111,-0.593920490425269,
136.585275505922));
#233628=CARTESIAN_POINT('Ctrl Pts',(176.330363155298,4.54261888720253,134.428768450716));
#233629=CARTESIAN_POINT('Ctrl Pts',(176.051915531486,5.50471342676105,128.941607659011));
#233630=CARTESIAN_POINT('Ctrl Pts',(175.773467907672,1.40824524732727,125.166225835676));
#233631=CARTESIAN_POINT('Ctrl Pts',(175.49502028386,-3.98233151779528,126.572014438702));
#233632=CARTESIAN_POINT('Ctrl Pts',(175.216572660047,-5.7133401657742,131.867122418498));
#233633=CARTESIAN_POINT('Ctrl Pts',(174.938125036234,-2.19406831359054,
136.185604222037));
#233634=CARTESIAN_POINT('Ctrl Pts',(174.659677412421,3.34144513258691,135.558986041432));
#233635=CARTESIAN_POINT('Ctrl Pts',(174.381229788608,5.80633374058666,130.563099372659));
#233636=CARTESIAN_POINT('Ctrl Pts',(174.102782164795,2.93548529615992,125.788920001687));
#233637=CARTESIAN_POINT('Ctrl Pts',(173.824334540982,-2.63293072900865,
125.623685538813));
#233638=CARTESIAN_POINT('Ctrl Pts',(173.54588691717,-5.7818120400351,130.219238383264));
#233639=CARTESIAN_POINT('Ctrl Pts',(173.267439293356,-3.61749054349026,
135.352489976228));
#233640=CARTESIAN_POINT('Ctrl Pts',(172.988991669544,1.87112803828436,136.306232877052));
#233641=CARTESIAN_POINT('Ctrl Pts',(172.71054404573,5.64027136256211,132.204023952811));
#233642=CARTESIAN_POINT('Ctrl Pts',(172.432096421918,4.22628084721974,126.815592800833));
#233643=CARTESIAN_POINT('Ctrl Pts',(172.153648798105,-1.07145530142008,
125.092644410292));
#233644=CARTESIAN_POINT('Ctrl Pts',(171.875201174292,-5.38457637155629,
128.618484181386));
#233645=CARTESIAN_POINT('Ctrl Pts',(171.596753550479,-4.74953480741189,
134.153037611328));
#233646=CARTESIAN_POINT('Ctrl Pts',(171.318305926666,0.25009721706947,136.610320475968));
#233647=CARTESIAN_POINT('Ctrl Pts',(171.039858302853,5.01990211699227,133.732209867644));
#233648=CARTESIAN_POINT('Ctrl Pts',(170.76141067904,5.1766622072511,128.163548831885));
#233649=CARTESIAN_POINT('Ctrl Pts',(170.482963055228,0.576322623054293,
125.021664816339));
#233650=CARTESIAN_POINT('Ctrl Pts',(170.204515431414,-4.55362929680409,
127.193795741725));
#233651=CARTESIAN_POINT('Ctrl Pts',(169.926067807602,-5.4990183500578,132.683859402108));
#233652=CARTESIAN_POINT('Ctrl Pts',(169.647620183788,-1.39107818158956,
136.446755498118));
#233653=CARTESIAN_POINT('Ctrl Pts',(169.369172559976,3.99519487781229,135.024566345214));
#233654=CARTESIAN_POINT('Ctrl Pts',(169.090724936163,5.71007902062496,129.724214297113));
#233655=CARTESIAN_POINT('Ctrl Pts',(168.81227731235,2.17767949635139,125.416463949427));
#233656=CARTESIAN_POINT('Ctrl Pts',(168.533829688537,-3.35590109951139,
126.059927426375));
#233657=CARTESIAN_POINT('Ctrl Pts',(168.255382064725,-5.80557252980615,
131.063293227581));
#233658=CARTESIAN_POINT('Ctrl Pts',(167.976934440911,-2.92020642319446,
135.828712609743));
#233659=CARTESIAN_POINT('Ctrl Pts',(167.698486817099,2.64868672631821,135.976997964335));
#233660=CARTESIAN_POINT('Ctrl Pts',(167.420039193286,5.78356616988455,131.371882294628));
#233661=CARTESIAN_POINT('Ctrl Pts',(167.141591569473,3.60363084624196,126.245241928676));
#233662=CARTESIAN_POINT('Ctrl Pts',(166.86314394566,-1.88786517794308,125.308208912483));
#233663=CARTESIAN_POINT('Ctrl Pts',(166.584696321847,-5.64450533093961,
129.421870811324));
#233664=CARTESIAN_POINT('Ctrl Pts',(166.306248698034,-4.21412083421794,
134.805973303719));
#233665=CARTESIAN_POINT('Ctrl Pts',(166.027801074221,1.08883483790225,136.512789227187));
#233666=CARTESIAN_POINT('Ctrl Pts',(165.749353450409,5.3912044865292,132.973838130654));
#233667=CARTESIAN_POINT('Ctrl Pts',(165.470905826595,4.73932058701693,127.441243184462));
#233668=CARTESIAN_POINT('Ctrl Pts',(165.192458202783,-0.267767403281747,
124.999188861871));
#233669=CARTESIAN_POINT('Ctrl Pts',(164.914010578969,-5.02879023112935,
127.891803784357));
#233670=CARTESIAN_POINT('Ctrl Pts',(164.635562955157,-5.16860050662956,
133.46091615025));
#233671=CARTESIAN_POINT('Ctrl Pts',(164.357115331344,-0.55871941670932,
136.588783761558));
#233672=CARTESIAN_POINT('Ctrl Pts',(164.078667707531,4.56459752220588,134.401049088318));
#233673=CARTESIAN_POINT('Ctrl Pts',(163.800220083718,5.49327233119978,128.908133418456));
#233674=CARTESIAN_POINT('Ctrl Pts',(163.521772459905,1.37389822909362,125.157757908727));
#233675=CARTESIAN_POINT('Ctrl Pts',(163.243324836092,-4.00802122688977,
126.596334436543));
#233676=CARTESIAN_POINT('Ctrl Pts',(162.964877212279,-5.70676497808368,
131.901881451211));
#233677=CARTESIAN_POINT('Ctrl Pts',(162.686429588467,-2.16127050538683,
136.198860436632));
#233678=CARTESIAN_POINT('Ctrl Pts',(162.407981964654,3.37032597782655,135.538557624299));
#233679=CARTESIAN_POINT('Ctrl Pts',(162.129534340841,5.80475753699479,130.527759041158));
#233680=CARTESIAN_POINT('Ctrl Pts',(161.851086717028,2.90490049783562,125.771143793998));
#233681=CARTESIAN_POINT('Ctrl Pts',(161.572639093215,-2.66441818655578,
125.639808921385));
#233682=CARTESIAN_POINT('Ctrl Pts',(161.294191469402,-5.7852667215671,130.254444755185));
#233683=CARTESIAN_POINT('Ctrl Pts',(161.015743845589,-3.58973776544978,
135.37442640163));
#233684=CARTESIAN_POINT('Ctrl Pts',(160.737296221776,1.90458482867669,136.294740852644));
#233685=CARTESIAN_POINT('Ctrl Pts',(160.458848597964,5.64868700939082,132.169664087608));
#233686=CARTESIAN_POINT('Ctrl Pts',(160.18040097415,4.20192178217643,126.789940132385));
#233687=CARTESIAN_POINT('Ctrl Pts',(159.901953350338,-1.10620428756715,
125.099272487699));
#233688=CARTESIAN_POINT('Ctrl Pts',(159.623505726525,-5.39778265812024,
128.651302125312));
#233689=CARTESIAN_POINT('Ctrl Pts',(159.345058102712,-4.72906246220349,
134.18188733455));
#233690=CARTESIAN_POINT('Ctrl Pts',(159.066610478899,0.285435108933367,
136.608690492233));
#233691=CARTESIAN_POINT('Ctrl Pts',(158.788162855086,5.03763175924073,133.701598052375));
#233692=CARTESIAN_POINT('Ctrl Pts',(158.509715231273,5.16049092479898,128.132085947844));
#233693=CARTESIAN_POINT('Ctrl Pts',(158.23126760746,0.541111034464008,125.018263716911));
#233694=CARTESIAN_POINT('Ctrl Pts',(157.952819983648,-4.57552346179978,
127.221581871133));
#233695=CARTESIAN_POINT('Ctrl Pts',(157.674372359834,-5.48747542341729,
132.717298664853));
#233696=CARTESIAN_POINT('Ctrl Pts',(157.395924736022,-1.35670554899215,
136.455118845335));
#233697=CARTESIAN_POINT('Ctrl Pts',(157.117477112209,4.02081044620608,135.000168269382));
#233698=CARTESIAN_POINT('Ctrl Pts',(156.839029488396,5.70339806885126,129.68947543801));
#233699=CARTESIAN_POINT('Ctrl Pts',(156.560581864583,2.1448414927076,125.403307621479));
#233700=CARTESIAN_POINT('Ctrl Pts',(156.28213424077,-3.38471963390224,126.080443652244));
#233701=CARTESIAN_POINT('Ctrl Pts',(156.003686616957,-5.8038887697026,131.098628597966));
#233702=CARTESIAN_POINT('Ctrl Pts',(155.725238993144,-2.88956766187541,
135.846395645489));
#233703=CARTESIAN_POINT('Ctrl Pts',(155.446791369331,2.68012496398725,135.960778819456));
#233704=CARTESIAN_POINT('Ctrl Pts',(155.168343745519,5.78691367932904,131.336665570917));
#233705=CARTESIAN_POINT('Ctrl Pts',(154.889896121706,3.57581142981733,126.223390074792));
#233706=CARTESIAN_POINT('Ctrl Pts',(154.611448497893,-1.92128683559663,
125.319802714623));
#233707=CARTESIAN_POINT('Ctrl Pts',(154.33300087408,-5.65281635917722,129.456256131708));
#233708=CARTESIAN_POINT('Ctrl Pts',(154.054553250267,-4.18968380410554,
134.831551712731));
#233709=CARTESIAN_POINT('Ctrl Pts',(153.776105626454,1.12356348950664,136.50605541652));
#233710=CARTESIAN_POINT('Ctrl Pts',(153.497658002641,5.40431082539012,132.940980143345));
#233711=CARTESIAN_POINT('Ctrl Pts',(153.219210378828,4.71876052800142,127.412455905645));
#233712=CARTESIAN_POINT('Ctrl Pts',(152.940762755016,-0.303100170353132,
125.000926394444));
#233713=CARTESIAN_POINT('Ctrl Pts',(152.662315131202,-5.04642661941966,
127.922469420767));
#233714=CARTESIAN_POINT('Ctrl Pts',(152.38386750739,-5.15233353688545,133.492329668737));
#233715=CARTESIAN_POINT('Ctrl Pts',(152.105419883576,-0.523497639439988,
136.592077673268));
#233716=CARTESIAN_POINT('Ctrl Pts',(151.826972259764,4.58640701436939,134.373196449306));
#233717=CARTESIAN_POINT('Ctrl Pts',(151.548524635951,5.48162768041213,128.874729443297));
#233718=CARTESIAN_POINT('Ctrl Pts',(151.270077012138,1.33950030055583,125.149499218718));
#233719=CARTESIAN_POINT('Ctrl Pts',(150.991629388325,-4.03356241728369,
126.620810364342));
#233720=CARTESIAN_POINT('Ctrl Pts',(150.713181764512,-5.69997832411825,
131.936599814887));
#233721=CARTESIAN_POINT('Ctrl Pts',(150.434734140699,-2.1283926105098,136.211916756054));
#233722=CARTESIAN_POINT('Ctrl Pts',(150.156286516886,3.39908193439765,135.517953779753));
#233723=CARTESIAN_POINT('Ctrl Pts',(149.877838893074,5.8029662359777,130.49242895923));
#233724=CARTESIAN_POINT('Ctrl Pts',(149.599391269261,2.87420805735513,125.753554094008));
#233725=CARTESIAN_POINT('Ctrl Pts',(149.320943645448,-2.69580691310719,
125.65612367832));
#233726=CARTESIAN_POINT('Ctrl Pts',(149.042496021635,-5.7885070279132,130.289671504441));
#233727=CARTESIAN_POINT('Ctrl Pts',(148.764048397822,-3.56185196835627,
135.396193481562));
#233728=CARTESIAN_POINT('Ctrl Pts',(148.485600774009,1.93797104397778,136.283045380177));
#233729=CARTESIAN_POINT('Ctrl Pts',(148.207153150196,5.6568933420451,132.135253630582));
#233730=CARTESIAN_POINT('Ctrl Pts',(147.928705526383,4.17740701337624,126.764436219762));
#233731=CARTESIAN_POINT('Ctrl Pts',(147.65025790257,-1.14091228290746,125.106111969245));
#233732=CARTESIAN_POINT('Ctrl Pts',(147.371810278758,-5.41078892786276,
128.684199851613));
#233733=CARTESIAN_POINT('Ctrl Pts',(147.093362654945,-4.70841487984645,
134.210611902278));
#233734=CARTESIAN_POINT('Ctrl Pts',(146.814915031132,0.320762423894332,
136.60684542692));
#233735=CARTESIAN_POINT('Ctrl Pts',(146.536467407319,5.05517473019176,133.670878878906));
#233736=CARTESIAN_POINT('Ctrl Pts',(146.258019783506,5.14412841845787,128.100722085923));
#233737=CARTESIAN_POINT('Ctrl Pts',(145.979572159693,0.505879394805349,
125.015077023433));
#233738=CARTESIAN_POINT('Ctrl Pts',(145.70112453588,-4.59724807909095,127.249500761725));
#233739=CARTESIAN_POINT('Ctrl Pts',(145.422676912067,-5.47572915635697,
132.750667042976));
#233740=CARTESIAN_POINT('Ctrl Pts',(145.144229288255,-1.32228264317164,
136.463272801628));
#233741=CARTESIAN_POINT('Ctrl Pts',(144.865781664442,4.0462770219901,134.975614716357));
#233742=CARTESIAN_POINT('Ctrl Pts',(144.587334040629,5.69650577556471,129.654777891387));
#233743=CARTESIAN_POINT('Ctrl Pts',(144.308886416816,2.11192401117359,125.390351431538));
#233744=CARTESIAN_POINT('Ctrl Pts',(144.030438793003,-3.41341274626234,
126.101134924595));
#233745=CARTESIAN_POINT('Ctrl Pts',(143.75199116919,-5.80198994436631,131.133953064144));
#233746=CARTESIAN_POINT('Ctrl Pts',(143.473543545377,-2.85882182656403,
135.863891846773));
#233747=CARTESIAN_POINT('Ctrl Pts',(143.195095921564,2.71146388864014,135.944368601604));
#233748=CARTESIAN_POINT('Ctrl Pts',(142.916648297751,5.790046752559,131.301429122451));
#233749=CARTESIAN_POINT('Ctrl Pts',(142.638200673938,3.54785951038517,126.201707970457));
#233750=CARTESIAN_POINT('Ctrl Pts',(142.359753050125,-1.95463729925998,
125.331599749072));
#233751=CARTESIAN_POINT('Ctrl Pts',(142.081305426313,-5.66091792022584,
129.490691406602));
#233752=CARTESIAN_POINT('Ctrl Pts',(141.8028578025,-4.16509152371897,134.856980892698));
#233753=CARTESIAN_POINT('Ctrl Pts',(141.524410178687,1.15825050705268,136.499110327454));
#233754=CARTESIAN_POINT('Ctrl Pts',(141.245962554874,5.41721690552589,132.908042982814));
#233755=CARTESIAN_POINT('Ctrl Pts',(140.967514931061,4.69802561357932,127.383794315106));
#233756=CARTESIAN_POINT('Ctrl Pts',(140.689067307248,-0.338421705936203,
125.002878975406));
#233757=CARTESIAN_POINT('Ctrl Pts',(140.410619683435,-5.06387601051571,
127.953241846716));
#233758=CARTESIAN_POINT('Ctrl Pts',(140.132172059623,-5.13587564552739,
133.523643583541));
#233759=CARTESIAN_POINT('Ctrl Pts',(139.85372443581,-0.48825646377323,136.595157118993));
#233760=CARTESIAN_POINT('Ctrl Pts',(139.575276811997,4.60804655553434,134.34521156577));
#233761=CARTESIAN_POINT('Ctrl Pts',(139.296829188184,5.46977990589493,128.841396971331));
#233762=CARTESIAN_POINT('Ctrl Pts',(139.018381564371,1.30505273634171,125.141450071677));
#233763=CARTESIAN_POINT('Ctrl Pts',(138.739933940558,-4.05895414253892,
126.645441315135));
#233764=CARTESIAN_POINT('Ctrl Pts',(138.461486316745,-5.69298045535984,
131.971276223022));
#233765=CARTESIAN_POINT('Ctrl Pts',(138.183038692932,-2.09543584726193,
136.224772696493));
#233766=CARTESIAN_POINT('Ctrl Pts',(137.904591069119,3.42771193673771,135.49717527128));
#233767=CARTESIAN_POINT('Ctrl Pts',(137.626143445306,5.80095990391266,130.457110436044));
#233768=CARTESIAN_POINT('Ctrl Pts',(137.347695821494,2.84340911203807,125.736151553513));
#233769=CARTESIAN_POINT('Ctrl Pts',(137.069248197681,-2.727095745542,125.672629205068));
#233770=CARTESIAN_POINT('Ctrl Pts',(136.790800573868,-5.7915328390027,130.324917325691));
#233771=CARTESIAN_POINT('Ctrl Pts',(136.512352950055,-3.53383418552815,
135.417790409441));
#233772=CARTESIAN_POINT('Ctrl Pts',(136.233905326242,1.97128544704926,136.271146893031));
#233773=CARTESIAN_POINT('Ctrl Pts',(135.955457702429,5.66489005643625,132.100793856825));
#233774=CARTESIAN_POINT('Ctrl Pts',(135.677010078616,4.15273744922295,126.739082008025));
#233775=CARTESIAN_POINT('Ctrl Pts',(135.398562454803,-1.17557800132362,
125.113162601491));
#233776=CARTESIAN_POINT('Ctrl Pts',(135.12011483099,-5.42359469883174,128.717176141249));
#233777=CARTESIAN_POINT('Ctrl Pts',(134.841667207177,-4.68759282544451,
134.239210250113));
#233778=CARTESIAN_POINT('Ctrl Pts',(134.563219583365,0.356077852885664,
136.604785348398));
#233779=CARTESIAN_POINT('Ctrl Pts',(134.284771959552,5.0725303797842,133.640053485549));
#233780=CARTESIAN_POINT('Ctrl Pts',(134.006324335739,5.12757529454644,128.069458408322));
#233781=CARTESIAN_POINT('Ctrl Pts',(133.727876711926,0.470629009599695,
125.012104853988));
#233782=CARTESIAN_POINT('Ctrl Pts',(133.449429088113,-4.61880234366392,
127.277551378957));
#233783=CARTESIAN_POINT('Ctrl Pts',(133.1709814643,-5.46377998413907,132.783963299997));
#233784=CARTESIAN_POINT('Ctrl Pts',(132.892533840487,-1.28781073968153,
136.47121706485));
#233785=CARTESIAN_POINT('Ctrl Pts',(132.614086216674,4.07159366149105,134.950906595976));
#233786=CARTESIAN_POINT('Ctrl Pts',(132.335638592862,5.68940239616175,129.620122942976));
#233787=CARTESIAN_POINT('Ctrl Pts',(132.057190969048,2.07892827151876,125.377595859696));
#233788=CARTESIAN_POINT('Ctrl Pts',(131.778743345236,-3.44197937335791,
126.122000476702));
#233789=CARTESIAN_POINT('Ctrl Pts',(131.500295721423,-5.79987612415893,
131.169265317152));
#233790=CARTESIAN_POINT('Ctrl Pts',(131.22184809761,-2.82797005655853,135.881200565267));
#233791=CARTESIAN_POINT('Ctrl Pts',(130.943400473797,2.74270233900145,135.927767918864));
#233792=CARTESIAN_POINT('Ctrl Pts',(130.664952849984,5.79296527347731,131.26617425493));
#233793=CARTESIAN_POINT('Ctrl Pts',(130.386505226171,3.51977612371406,126.180196419108));
#233794=CARTESIAN_POINT('Ctrl Pts',(130.108057602358,-1.98791533311939,
125.343599578688));
#233795=CARTESIAN_POINT('Ctrl Pts',(129.829609978546,-5.66880971387908,
129.52517535999));
#233796=CARTESIAN_POINT('Ctrl Pts',(129.551162354732,-4.14034490433441,
134.882259901329));
#233797=CARTESIAN_POINT('Ctrl Pts',(129.27271473092,1.19289460520041,136.491954217345));
#233798=CARTESIAN_POINT('Ctrl Pts',(128.994267107107,5.42992224869717,132.875027869557));
#233799=CARTESIAN_POINT('Ctrl Pts',(128.715819483294,4.67711661209022,127.355259474909));
#233800=CARTESIAN_POINT('Ctrl Pts',(128.437371859481,-0.373730701178542,
125.005046532403));
#233801=CARTESIAN_POINT('Ctrl Pts',(128.158924235668,-5.0811377578241,127.984119921918));
#233802=CARTESIAN_POINT('Ctrl Pts',(127.880476611855,-5.11922744240848,
133.554856734316));
#233803=CARTESIAN_POINT('Ctrl Pts',(127.602028988042,-0.452997195583419,
136.598021984625));
#233804=CARTESIAN_POINT('Ctrl Pts',(127.323581364229,4.62951534383955,134.3170954747));
#233805=CARTESIAN_POINT('Ctrl Pts',(127.045133740417,5.45772944667181,128.808137237705));
#233806=CARTESIAN_POINT('Ctrl Pts',(126.766686116604,1.2705568129186,125.133610765869));
#233807=CARTESIAN_POINT('Ctrl Pts',(126.488238492791,-4.08419546175569,
126.67022637621));
#233808=CARTESIAN_POINT('Ctrl Pts',(126.209790868978,-5.68577163111709,
132.005909390672));
#233809=CARTESIAN_POINT('Ctrl Pts',(125.931343245165,-2.06240143686808,
136.237427781569));
#233810=CARTESIAN_POINT('Ctrl Pts',(125.652895621352,3.45621492395137,135.476222868834));
#233811=CARTESIAN_POINT('Ctrl Pts',(125.374447997539,5.79873861514512,130.421804780342));
#233812=CARTESIAN_POINT('Ctrl Pts',(125.096000373726,2.8125048031507,125.718936817367));
#233813=CARTESIAN_POINT('Ctrl Pts',(124.817552749914,-2.75828352444112,
125.68932489001));
#233814=CARTESIAN_POINT('Ctrl Pts',(124.5391051261,-5.79434404271298,130.36018091289));
#233815=CARTESIAN_POINT('Ctrl Pts',(124.260657502288,-3.50568545517477,
135.439216384981));
#233816=CARTESIAN_POINT('Ctrl Pts',(123.982209878475,2.00452680341345,136.25904583211));
#233817=CARTESIAN_POINT('Ctrl Pts',(123.703762254662,5.67267685624313,132.066286043259));
#233818=CARTESIAN_POINT('Ctrl Pts',(123.425314630849,4.12791400385628,126.71387843668));
#233819=CARTESIAN_POINT('Ctrl Pts',(123.146867007036,-1.21020015826455,
125.120424123171));
#233820=CARTESIAN_POINT('Ctrl Pts',(122.868419383223,-5.43619949650465,
128.750229772276));
#233821=CARTESIAN_POINT('Ctrl Pts',(122.58997175941,-4.66659707056658,134.267681318331));
#233822=CARTESIAN_POINT('Ctrl Pts',(122.311524135597,0.391380087281262,
136.602510333005));
#233823=CARTESIAN_POINT('Ctrl Pts',(122.033076511785,5.08969806489794,133.609123014551));
#233824=CARTESIAN_POINT('Ctrl Pts',(121.754628887972,5.11083216644683,128.038296073528));
#233825=CARTESIAN_POINT('Ctrl Pts',(121.476181264159,0.435361185062875,
125.00934731871));
#233826=CARTESIAN_POINT('Ctrl Pts',(121.197733640346,-4.64018545681751,
127.305732683402));
#233827=CARTESIAN_POINT('Ctrl Pts',(120.919286016533,-5.45162834954452,
132.817186202114));
#233828=CARTESIAN_POINT('Ctrl Pts',(120.64083839272,-1.25329111589093,136.478951340622));
#233829=CARTESIAN_POINT('Ctrl Pts',(120.362390768907,4.09675942659154,134.92604482381));
#233830=CARTESIAN_POINT('Ctrl Pts',(120.083943145094,5.68208819386074,129.585511876926));
#233831=CARTESIAN_POINT('Ctrl Pts',(119.805495521281,2.04585549641223,125.36504137862));
#233832=CARTESIAN_POINT('Ctrl Pts',(119.527047897469,-3.47041845664194,
126.143039535386));
#233833=CARTESIAN_POINT('Ctrl Pts',(119.248600273655,-5.79754738740892,
131.204564048482));
#233834=CARTESIAN_POINT('Ctrl Pts',(118.970152649843,-2.7970134950826,135.898321159589));
#233835=CARTESIAN_POINT('Ctrl Pts',(118.69170502603,2.77383915751901,135.910977386384));
#233836=CARTESIAN_POINT('Ctrl Pts',(118.413257402217,5.795669133937,131.230902274733));
#233837=CARTESIAN_POINT('Ctrl Pts',(118.134809778404,3.49156231044436,126.158856217863));
#233838=CARTESIAN_POINT('Ctrl Pts',(117.856362154591,-2.02111970404504,
125.355801758813));
#233839=CARTESIAN_POINT('Ctrl Pts',(117.577914530778,-5.67649144770371,
129.559706714059));
#233840=CARTESIAN_POINT('Ctrl Pts',(117.299466906965,-4.11544486294674,
134.907387801903));
#233841=CARTESIAN_POINT('Ctrl Pts',(117.021019283153,1.22749450019975,136.484587351363));
#233842=CARTESIAN_POINT('Ctrl Pts',(116.74257165934,5.44242638410263,132.841936026965));
#233843=CARTESIAN_POINT('Ctrl Pts',(116.464124035527,4.65603429832517,127.326852442422));
#233844=CARTESIAN_POINT('Ctrl Pts',(116.185676411714,-0.409025847692317,
125.007428985116));
#233845=CARTESIAN_POINT('Ctrl Pts',(115.907228787901,-5.09821122170419,
128.015102502178));
#233846=CARTESIAN_POINT('Ctrl Pts',(115.628781164088,-5.10238954443416,
133.585967964446));
#233847=CARTESIAN_POINT('Ctrl Pts',(115.350333540275,-0.417721141415912,
136.600672164005));
#233848=CARTESIAN_POINT('Ctrl Pts',(115.071885916462,4.65081258375125,134.288849217947));
#233849=CARTESIAN_POINT('Ctrl Pts',(114.793438292649,5.44547674927697,128.77495147487));
#233850=CARTESIAN_POINT('Ctrl Pts',(114.514990668836,1.23601380854556,125.125981591782));
#233851=CARTESIAN_POINT('Ctrl Pts',(114.236543045024,-4.10928543960769,
126.695164629152));
#233852=CARTESIAN_POINT('Ctrl Pts',(113.958095421211,-5.67835211851559,
132.040498034489));
#233853=CARTESIAN_POINT('Ctrl Pts',(113.679647797398,-2.02929060343055,
136.249881542344));
#233854=CARTESIAN_POINT('Ctrl Pts',(113.401200173585,3.48458983985001,135.455097348814));
#233855=CARTESIAN_POINT('Ctrl Pts',(113.122752549772,5.79630245198571,130.386513300387));
#233856=CARTESIAN_POINT('Ctrl Pts',(112.844304925959,2.78149627586357,125.701910523471));
#233857=CARTESIAN_POINT('Ctrl Pts',(112.565857302146,-2.78936909412988,
125.706210114483));
#233858=CARTESIAN_POINT('Ctrl Pts',(112.287409678333,-5.7969405348739,130.395460959329));
#233859=CARTESIAN_POINT('Ctrl Pts',(112.008962054521,-3.47740682035766,
135.460470614237));
#233860=CARTESIAN_POINT('Ctrl Pts',(111.730514430707,2.03769388129978,136.246742645822));
#233861=CARTESIAN_POINT('Ctrl Pts',(111.452066806895,5.68025345292297,132.031731468582));
#233862=CARTESIAN_POINT('Ctrl Pts',(111.173619183082,4.10293759711819,126.688826439658));
#233863=CARTESIAN_POINT('Ctrl Pts',(110.895171559269,-1.24477747079359,
125.127896265209));
#233864=CARTESIAN_POINT('Ctrl Pts',(110.616723935456,-5.44860285380605,
128.783359519875));
#233865=CARTESIAN_POINT('Ctrl Pts',(110.338276311643,-4.64542839321807,
134.296024051927));
#233866=CARTESIAN_POINT('Ctrl Pts',(110.05982868783,0.426667818943798,136.600020465042));
#233867=CARTESIAN_POINT('Ctrl Pts',(109.781381064017,5.10667714937814,133.57808861205));
#233868=CARTESIAN_POINT('Ctrl Pts',(109.502933440204,5.0938996545818,128.007236236273));
#233869=CARTESIAN_POINT('Ctrl Pts',(109.224485816392,0.400077228057368,
125.006804519781));
#233870=CARTESIAN_POINT('Ctrl Pts',(108.946038192578,-4.66139662619255,
127.334043630792));
#233871=CARTESIAN_POINT('Ctrl Pts',(108.667590568766,-5.43927470285667,
132.850334518237));
#233872=CARTESIAN_POINT('Ctrl Pts',(108.389142944953,-1.21872505093712,
136.486475342347));
#233873=CARTESIAN_POINT('Ctrl Pts',(108.11069532114,4.1217733847649,134.901030321119));
#233874=CARTESIAN_POINT('Ctrl Pts',(107.832247697327,5.67456343969215,129.550945975765));
#233875=CARTESIAN_POINT('Ctrl Pts',(107.553800073514,2.01270691137792,125.352688453517));
#233876=CARTESIAN_POINT('Ctrl Pts',(107.275352449701,-3.49872894229381,
126.164251321038));
#233877=CARTESIAN_POINT('Ctrl Pts',(106.996904825888,-5.7950038204084,131.239847950126));
#233878=CARTESIAN_POINT('Ctrl Pts',(106.718457202076,-2.76595328924301,
135.91525299533));
#233879=CARTESIAN_POINT('Ctrl Pts',(106.440009578262,2.80487319040651,135.893997626342));
#233880=CARTESIAN_POINT('Ctrl Pts',(106.16156195445,5.7981582337456,131.195614488879));
#233881=CARTESIAN_POINT('Ctrl Pts',(105.883114330637,3.46321911604922,126.137688157493));
#233882=CARTESIAN_POINT('Ctrl Pts',(105.604666706824,-2.05424918163679,
125.36820583729));
#233883=CARTESIAN_POINT('Ctrl Pts',(105.326219083011,-5.68396283705021,
129.594284189235));
#233884=CARTESIAN_POINT('Ctrl Pts',(105.047771459198,-4.09039232223623,
134.932363663296));
#233885=CARTESIAN_POINT('Ctrl Pts',(104.769323835385,1.26204890993897,136.47701000249));
#233886=CARTESIAN_POINT('Ctrl Pts',(104.490876211572,5.45472884839698,132.808768681268));
#233887=CARTESIAN_POINT('Ctrl Pts',(104.21242858776,4.63477945349693,127.29857427028));
#233888=CARTESIAN_POINT('Ctrl Pts',(103.933980963947,-0.444305837602887,
125.010026245263));
#233889=CARTESIAN_POINT('Ctrl Pts',(103.655533340134,-5.1150957694926,128.046188439421));
#233890=CARTESIAN_POINT('Ctrl Pts',(103.377085716321,-5.08536257553889,
133.616976121092));
#233891=CARTESIAN_POINT('Ctrl Pts',(103.098638092508,-0.38242960843803,
136.603107558928));
#233892=CARTESIAN_POINT('Ctrl Pts',(102.820190468695,4.6719374860923,134.260473842188));
#233893=CARTESIAN_POINT('Ctrl Pts',(102.541742844882,5.4330222677386,128.741840912539));
#233894=CARTESIAN_POINT('Ctrl Pts',(102.263295221069,1.2014250032263,125.118562832119));
#233895=CARTESIAN_POINT('Ctrl Pts',(101.984847597256,-4.13422314637653,
126.720255149861));
#233896=CARTESIAN_POINT('Ctrl Pts',(101.706399973443,-5.67072219248816,
132.07504087278));
#233897=CARTESIAN_POINT('Ctrl Pts',(101.427952349631,-1.99610457388343,
136.262133517338));
#233898=CARTESIAN_POINT('Ctrl Pts',(101.149504725818,3.51283563299066,135.433799494034));
#233899=CARTESIAN_POINT('Ctrl Pts',(100.871057102005,5.7936515047074,130.351237303918));
#233900=CARTESIAN_POINT('Ctrl Pts',(100.592609478192,2.75038467920892,125.685073302739));
#233901=CARTESIAN_POINT('Ctrl Pts',(100.314161854379,-2.82035130272114,
125.723284252797));
#233902=CARTESIAN_POINT('Ctrl Pts',(100.035714230566,-5.79932221927147,
130.430756157697));
#233903=CARTESIAN_POINT('Ctrl Pts',(99.7572666067534,-3.44899932895201,
135.481552309624));
#233904=CARTESIAN_POINT('Ctrl Pts',(99.4788189829407,2.07078545168999,136.234237790066));
#233905=CARTESIAN_POINT('Ctrl Pts',(99.2003713591278,5.6876195657222,131.997131413226));
#233906=CARTESIAN_POINT('Ctrl Pts',(98.9219237353147,4.07780915451857,126.663926945268));
#233907=CARTESIAN_POINT('Ctrl Pts',(98.6434761115021,-1.27930865763567,
125.13557875072));
#233908=CARTESIAN_POINT('Ctrl Pts',(98.3650284876889,-5.460804311125,128.816564156414));
#233909=CARTESIAN_POINT('Ctrl Pts',(98.0865808638763,-4.62408757781209,
134.324237400649));
#233910=CARTESIAN_POINT('Ctrl Pts',(97.8081332400632,0.461939740273397,
136.597315836771));
#233911=CARTESIAN_POINT('Ctrl Pts',(97.5296856162504,5.12346700405862,133.546951428038));
#233912=CARTESIAN_POINT('Ctrl Pts',(97.2512379924375,5.07677838639178,127.97628004749));
#233913=CARTESIAN_POINT('Ctrl Pts',(96.9727903686245,0.364778446043045,
125.004476551425));
#233914=CARTESIAN_POINT('Ctrl Pts',(96.6943427448119,-4.68243506580139,
127.362483172053));
#233915=CARTESIAN_POINT('Ctrl Pts',(96.4158951209985,-5.42671950184442,
132.883407020047));
#233916=CARTESIAN_POINT('Ctrl Pts',(96.1374474971861,-1.18411382567837,
136.493788791223));
#233917=CARTESIAN_POINT('Ctrl Pts',(95.8589998733729,4.14663460910971,134.875864014826));
#233918=CARTESIAN_POINT('Ctrl Pts',(95.5805522495601,5.66682841248846,129.516426520346));
#233919=CARTESIAN_POINT('Ctrl Pts',(95.3021046257473,1.97948374474885,125.340537542131));
#233920=CARTESIAN_POINT('Ctrl Pts',(95.0236570019342,-3.52690978125809,
126.185635047646));
#233921=CARTESIAN_POINT('Ctrl Pts',(94.7452093781216,-5.79224551741027,
131.275115714627));
#233922=CARTESIAN_POINT('Ctrl Pts',(94.4667617543085,-2.73479058998699,
135.931995445075));
#233923=CARTESIAN_POINT('Ctrl Pts',(94.1883141304955,2.8358032876865,135.876829267928));
#233924=CARTESIAN_POINT('Ctrl Pts',(93.909866506683,5.80043248066857,131.160312204968));
#233925=CARTESIAN_POINT('Ctrl Pts',(93.6314188828698,3.43474759079615,126.116693022386));
#233926=CARTESIAN_POINT('Ctrl Pts',(93.352971259057,-2.08730253826965,125.380811354481));
#233927=CARTESIAN_POINT('Ctrl Pts',(93.0745236352441,-5.69122360506351,
129.628906504239));
#233928=CARTESIAN_POINT('Ctrl Pts',(92.7960760114314,-4.06518821053398,
134.957186560018));
#233929=CARTESIAN_POINT('Ctrl Pts',(92.5176283876181,1.29655655399172,136.469222451509));
#233930=CARTESIAN_POINT('Ctrl Pts',(92.2391807638055,5.46682918570788,132.775527061492));
#233931=CARTESIAN_POINT('Ctrl Pts',(91.9607331399925,4.61335286521161,127.270426006341));
#233932=CARTESIAN_POINT('Ctrl Pts',(91.6822855161797,-0.479569363597252,
125.012838216602));
#233933=CARTESIAN_POINT('Ctrl Pts',(91.4038378923669,-5.13179077552621,
128.077376581749));
#233934=CARTESIAN_POINT('Ctrl Pts',(91.1253902685539,-5.06814716666323,
133.647880055237));
#233935=CARTESIAN_POINT('Ctrl Pts',(90.846942644741,-0.347123904390365,
136.605328079151));
#233936=CARTESIAN_POINT('Ctrl Pts',(90.5684950209282,4.69288926807169,134.231970398883));
#233937=CARTESIAN_POINT('Ctrl Pts',(90.2900473971151,5.42036646356212,128.708806777632));
#233938=CARTESIAN_POINT('Ctrl Pts',(90.0115997733025,1.16679167866171,125.111354761782));
#233939=CARTESIAN_POINT('Ctrl Pts',(89.7331521494893,-4.15900765798632,
126.7454970086));
#233940=CARTESIAN_POINT('Ctrl Pts',(89.4547045256766,-5.66288213576447,
132.109536625546));
#233941=CARTESIAN_POINT('Ctrl Pts',(89.1762569018636,-1.96284457794726,
136.274183252551));
#233942=CARTESIAN_POINT('Ctrl Pts',(88.8978092780507,3.5409512567151,135.412330093694));
#233943=CARTESIAN_POINT('Ctrl Pts',(88.619361654238,5.79078587154194,130.3159780981));
#233944=CARTESIAN_POINT('Ctrl Pts',(88.3409140304249,2.71917116603865,125.668425779081));
#233945=CARTESIAN_POINT('Ctrl Pts',(88.0624664066122,-2.85122900215762,
125.740546672265));
#233946=CARTESIAN_POINT('Ctrl Pts',(87.7840187827991,-5.80148900765152,
130.466065200115));
#233947=CARTESIAN_POINT('Ctrl Pts',(87.5055711589863,-3.42046403360785,
135.502460689953));
#233948=CARTESIAN_POINT('Ctrl Pts',(87.2271235351733,2.10380028836375,136.221531728214));
#233949=CARTESIAN_POINT('Ctrl Pts',(86.9486759113605,5.69477492168681,131.962487159311));
#233950=CARTESIAN_POINT('Ctrl Pts',(86.6702282875477,4.05252960720113,126.63918087617));
#233951=CARTESIAN_POINT('Ctrl Pts',(86.3917806637346,-1.31379243922498,
125.14347129503));
#233952=CARTESIAN_POINT('Ctrl Pts',(86.113333039922,-5.47280341633199,128.849842451481));
#233953=CARTESIAN_POINT('Ctrl Pts',(85.8348854161089,-4.6025754151404,134.352320319043));
#233954=CARTESIAN_POINT('Ctrl Pts',(85.5564377922961,0.497194544256039,
136.594396548415));
#233955=CARTESIAN_POINT('Ctrl Pts',(85.2779901684829,5.1400670067851,133.515712616316));
#233956=CARTESIAN_POINT('Ctrl Pts',(84.9995425446705,5.05946899631168,127.945428654274));
#233957=CARTESIAN_POINT('Ctrl Pts',(84.7210949208572,0.329466147029263,
125.002363499906));
#233958=CARTESIAN_POINT('Ctrl Pts',(84.4426472970446,-4.70329999605691,
127.391050253351));
#233959=CARTESIAN_POINT('Ctrl Pts',(84.1641996732315,-5.41396321174535,
132.916402482027));
#233960=CARTESIAN_POINT('Ctrl Pts',(83.8857520494189,-1.14945872264635,
136.500891416245));
#233961=CARTESIAN_POINT('Ctrl Pts',(83.6073044256056,4.17134217838416,134.850546837477));
#233962=CARTESIAN_POINT('Ctrl Pts',(83.328856801793,5.65888339887398,129.481954789796));
#233963=CARTESIAN_POINT('Ctrl Pts',(83.05040917798,1.94618722762166,125.328589094719));
#233964=CARTESIAN_POINT('Ctrl Pts',(82.7719615541671,-3.5549599292834,126.207189922827));
#233965=CARTESIAN_POINT('Ctrl Pts',(82.4935139303543,-5.78927258062435,
131.310366035126));
#233966=CARTESIAN_POINT('Ctrl Pts',(82.2150663065413,-2.70352655206008,
135.948547888425));
#233967=CARTESIAN_POINT('Ctrl Pts',(81.9366186827285,2.86662830323276,135.859472947324));
#233968=CARTESIAN_POINT('Ctrl Pts',(81.6581710589156,5.80249179043285,131.124996731141));
#233969=CARTESIAN_POINT('Ctrl Pts',(81.3797234351026,3.40614878970799,126.095871590527));
#233970=CARTESIAN_POINT('Ctrl Pts',(81.1012758112897,-2.12027854913937,
125.393617843285));
#233971=CARTESIAN_POINT('Ctrl Pts',(80.822828187477,-5.6982734826932,129.663572376127));
#233972=CARTESIAN_POINT('Ctrl Pts',(80.5443805636639,-4.03983346178761,
134.981855572247));
#233973=CARTESIAN_POINT('Ctrl Pts',(80.2659329398512,1.33101615366455,136.461224986989));
#233974=CARTESIAN_POINT('Ctrl Pts',(79.9874853160382,5.47872694765296,132.742212399419));
#233975=CARTESIAN_POINT('Ctrl Pts',(79.7090376922254,4.59175532743923,127.242408693648));
#233976=CARTESIAN_POINT('Ctrl Pts',(79.4305900684125,-0.514815118972584,
125.015864794932));
#233977=CARTESIAN_POINT('Ctrl Pts',(79.1521424445996,-5.1482956211654,128.108665773475));
#233978=CARTESIAN_POINT('Ctrl Pts',(78.8736948207867,-5.05074395573051,
133.678678621723));
#233979=CARTESIAN_POINT('Ctrl Pts',(78.5952471969738,-0.31180533753877,
136.607333642391));
#233980=CARTESIAN_POINT('Ctrl Pts',(78.3167995731609,4.71366715331346,134.203339944237));
#233981=CARTESIAN_POINT('Ctrl Pts',(78.0383519493481,5.407509805713,128.675850294243));
#233982=CARTESIAN_POINT('Ctrl Pts',(77.7599043255351,1.1321151182024,125.104357647873));
#233983=CARTESIAN_POINT('Ctrl Pts',(77.4814567017223,-4.18363805603787,
126.770889270024));
#233984=CARTESIAN_POINT('Ctrl Pts',(77.2030090779094,-5.65483223886072,
132.143984014535));
#233985=CARTESIAN_POINT('Ctrl Pts',(76.9245614540965,-1.92951184808342,
136.286030301474));
#233986=CARTESIAN_POINT('Ctrl Pts',(76.6461138302835,3.56893566918854,135.390689943351));
#233987=CARTESIAN_POINT('Ctrl Pts',(76.3676662064707,5.78770565867644,130.280736989476));
#233988=CARTESIAN_POINT('Ctrl Pts',(76.0892185826578,2.68785689298084,125.651968569378));
#233989=CARTESIAN_POINT('Ctrl Pts',(75.8107709588449,-2.8820010482549,125.75799673322));
#233990=CARTESIAN_POINT('Ctrl Pts',(75.532323335032,-5.8034408197229,130.501386778194));
#233991=CARTESIAN_POINT('Ctrl Pts',(75.2538757112192,-3.39180199171105,
135.523194980456));
#233992=CARTESIAN_POINT('Ctrl Pts',(74.9754280874062,2.13673716794415,136.208624931095));
#233993=CARTESIAN_POINT('Ctrl Pts',(74.6969804635933,5.70171925567246,131.92779999059));
#233994=CARTESIAN_POINT('Ctrl Pts',(74.4185328397805,4.02709989190878,126.61458914934));
#233995=CARTESIAN_POINT('Ctrl Pts',(74.1400852159675,-1.34822753775231,
125.151573605674));
#233996=CARTESIAN_POINT('Ctrl Pts',(73.8616375921548,-5.48459972479585,
128.883193171938));
#233997=CARTESIAN_POINT('Ctrl Pts',(73.5831899683417,-4.58089270234404,
134.380271766487));
#233998=CARTESIAN_POINT('Ctrl Pts',(73.3047423445289,0.532430924512096,
136.591262708148));
#233999=CARTESIAN_POINT('Ctrl Pts',(73.026294720716,5.15647654243839,133.484373334449));
#234000=CARTESIAN_POINT('Ctrl Pts',(72.7478470969032,5.04197212574731,127.914683199832));
#234001=CARTESIAN_POINT('Ctrl Pts',(72.46939947309,0.294141639526237,125.000465443524));
#234002=CARTESIAN_POINT('Ctrl Pts',(72.1909518492774,-4.72399064380143,
127.419743816117));
#234003=CARTESIAN_POINT('Ctrl Pts',(71.9125042254643,-5.40100630524849,
132.949319681519));
#234004=CARTESIAN_POINT('Ctrl Pts',(71.6340566016516,-1.11476102599866,
136.507782954223));
#234005=CARTESIAN_POINT('Ctrl Pts',(71.3556089778387,4.19589517704018,134.82507972721));
#234006=CARTESIAN_POINT('Ctrl Pts',(71.0771613540258,5.65072869325411,129.447532061481));
#234007=CARTESIAN_POINT('Ctrl Pts',(70.7987137302128,1.91281859381102,125.316843554035));
#234008=CARTESIAN_POINT('Ctrl Pts',(70.5202661064001,-3.58287834696108,
126.22891514786));
#234009=CARTESIAN_POINT('Ctrl Pts',(70.241818482587,-5.78608512021397,131.345597605407));
#234010=CARTESIAN_POINT('Ctrl Pts',(69.9633708587742,-2.67216233396265,
135.964909712024));
#234011=CARTESIAN_POINT('Ctrl Pts',(69.6849232349613,2.89734709481291,135.841929307673));
#234012=CARTESIAN_POINT('Ctrl Pts',(69.4064756111484,5.80433608672999,131.089669376025));
#234013=CARTESIAN_POINT('Ctrl Pts',(69.1280279873355,3.37742377252397,126.07522463346));
#234014=CARTESIAN_POINT('Ctrl Pts',(68.8495803635227,-2.15317599230747,
125.406624829152));
#234015=CARTESIAN_POINT('Ctrl Pts',(68.5711327397097,-5.70511220870344,
129.698280520343));
#234016=CARTESIAN_POINT('Ctrl Pts',(68.2926851158969,-4.01432901552682,
135.006369785865));
#234017=CARTESIAN_POINT('Ctrl Pts',(68.014237492084,1.36542643204398,136.45301790528));
#234018=CARTESIAN_POINT('Ctrl Pts',(67.735789868271,5.49042169335597,132.708825929535));
#234019=CARTESIAN_POINT('Ctrl Pts',(67.4573422444582,4.56998764048497,127.214523370394));
#234020=CARTESIAN_POINT('Ctrl Pts',(67.1788946206453,-0.550041797684044,
125.019105868103));
#234021=CARTESIAN_POINT('Ctrl Pts',(66.9004469968323,-5.164609694817,128.140054855163));
#234022=CARTESIAN_POINT('Ctrl Pts',(66.6219993730196,-5.03315358762317,
133.709370679297));
#234023=CARTESIAN_POINT('Ctrl Pts',(66.3435517492066,-0.2764752166261,136.609124174332));
#234024=CARTESIAN_POINT('Ctrl Pts',(66.0651041253938,4.73427037188528,134.174583539162));
#234025=CARTESIAN_POINT('Ctrl Pts',(65.7866565015808,5.39445277059944,128.642972683589));
#234026=CARTESIAN_POINT('Ctrl Pts',(65.508208877768,1.0973966068015,125.097571749668));
#234027=CARTESIAN_POINT('Ctrl Pts',(65.2297612539551,-4.20811342784249,
126.796430993211));
#234028=CARTESIAN_POINT('Ctrl Pts',(64.9513136301422,-5.64657280006891,
132.178381763287));
#234029=CARTESIAN_POINT('Ctrl Pts',(64.6728660063292,-1.89610761944867,
136.297674225111));
#234030=CARTESIAN_POINT('Ctrl Pts',(64.3944183825164,3.59678783343796,135.368879844889));
#234031=CARTESIAN_POINT('Ctrl Pts',(64.1159707587035,5.78441098024938,130.245515283918));
#234032=CARTESIAN_POINT('Ctrl Pts',(63.8375231348906,2.65644302039782,125.635702283457));
#234033=CARTESIAN_POINT('Ctrl Pts',(63.5590755110777,-2.91266630074331,
125.775633789045));
#234034=CARTESIAN_POINT('Ctrl Pts',(63.2806278872649,-5.80517758316048,
130.53671958308));
#234035=CARTESIAN_POINT('Ctrl Pts',(63.0021802634519,-3.36301426534433,
135.543754412816));
#234036=CARTESIAN_POINT('Ctrl Pts',(62.723732639639,2.16959486994269,136.195517876976));
#234037=CARTESIAN_POINT('Ctrl Pts',(62.4452850158262,5.70845231035428,131.893071192411));
#234038=CARTESIAN_POINT('Ctrl Pts',(62.1668373920132,4.00152095094907,126.590152676031));
#234039=CARTESIAN_POINT('Ctrl Pts',(61.8883897682004,-1.38261267721222,
125.159885382419));
#234040=CARTESIAN_POINT('Ctrl Pts',(61.6099421443874,-5.49619279939966,
128.916615081961));
#234041=CARTESIAN_POINT('Ctrl Pts',(61.3314945205747,-4.55904024288434,
134.408090707227));
#234042=CARTESIAN_POINT('Ctrl Pts',(61.0530468967616,0.567647575344072,
136.587914432096));
#234043=CARTESIAN_POINT('Ctrl Pts',(60.7745992729488,5.17269500295686,133.452934743723));
#234044=CARTESIAN_POINT('Ctrl Pts',(60.496151649136,5.02428842305186,127.884044823451));
#234045=CARTESIAN_POINT('Ctrl Pts',(60.2177040253229,0.258806232497024,
124.998782452612));
#234046=CARTESIAN_POINT('Ctrl Pts',(59.9392564015102,-4.74450624233532,
127.448562797104));
#234047=CARTESIAN_POINT('Ctrl Pts',(59.6608087776971,-5.38784926247686,
132.982157398764));
#234048=CARTESIAN_POINT('Ctrl Pts',(59.3823611538844,-1.08002202147149,
136.514463149789));
#234049=CARTESIAN_POINT('Ctrl Pts',(59.1039135300714,4.22029269525717,134.799463627718));
#234050=CARTESIAN_POINT('Ctrl Pts',(58.8254659062585,5.64236459780459,129.413159610949));
#234051=CARTESIAN_POINT('Ctrl Pts',(58.5470182824457,1.8793790798041,125.305301355313));
#234052=CARTESIAN_POINT('Ctrl Pts',(58.2685706586328,-3.61066399976409,
126.250809917708));
#234053=CARTESIAN_POINT('Ctrl Pts',(57.9901230348199,-5.78268325429153,
131.380809119953));
#234054=CARTESIAN_POINT('Ctrl Pts',(57.711675411007,-2.64069909790739,135.981080309579));
#234055=CARTESIAN_POINT('Ctrl Pts',(57.4332277871941,2.92795852413098,135.824198999061));
#234056=CARTESIAN_POINT('Ctrl Pts',(57.1547801633813,5.80596530121877,131.054331448687));
#234057=CARTESIAN_POINT('Ctrl Pts',(56.8763325395683,3.34857360366007,126.054752916266));
#234058=CARTESIAN_POINT('Ctrl Pts',(56.5978849157555,-2.18599364874745,
125.419831830104));
#234059=CARTESIAN_POINT('Ctrl Pts',(56.3194372919424,-5.71173952968275,
129.733029650764));
#234060=CARTESIAN_POINT('Ctrl Pts',(56.0409896681298,-3.98867581682796,
135.030728292487));
#234061=CARTESIAN_POINT('Ctrl Pts',(55.7625420443167,1.39978611404518,136.444601510497));
#234062=CARTESIAN_POINT('Ctrl Pts',(55.4840944205039,5.50191298946419,132.675368888989));
#234063=CARTESIAN_POINT('Ctrl Pts',(55.2056467966909,4.54805061095778,127.186771069878));
#234064=CARTESIAN_POINT('Ctrl Pts',(54.9271991728781,-0.585248094394635,
125.022561316018));
#234065=CARTESIAN_POINT('Ctrl Pts',(54.6487515490652,-5.18073239195715,
128.171542663682));
#234066=CARTESIAN_POINT('Ctrl Pts',(54.3703039252523,-5.01537671415865,
133.739955090657));
#234067=CARTESIAN_POINT('Ctrl Pts',(54.0918563014394,-0.241134850822232,
136.610699608625));
#234068=CARTESIAN_POINT('Ctrl Pts',(53.8134086776265,4.75469816032759,134.145702249237));
#234069=CARTESIAN_POINT('Ctrl Pts',(53.5349610538137,5.38119584205463,128.610175163959));
#234070=CARTESIAN_POINT('Ctrl Pts',(53.2565134300007,1.06263743096531,125.090997318624));
#234071=CARTESIAN_POINT('Ctrl Pts',(52.9780658061879,-4.23243286645675,
126.822121231705));
#234072=CARTESIAN_POINT('Ctrl Pts',(52.6996181823749,-5.63810412544538,
132.21272859718));
#234073=CARTESIAN_POINT('Ctrl Pts',(52.4211705585621,-1.86263312984859,
136.309114591992));
#234074=CARTESIAN_POINT('Ctrl Pts',(52.1427229347491,3.62450671739182,135.346900606486));
#234075=CARTESIAN_POINT('Ctrl Pts',(51.8642753109363,5.7809019583462,130.210314286579));
#234076=CARTESIAN_POINT('Ctrl Pts',(51.5858276871234,2.62493071234137,125.619627524071));
#234077=CARTESIAN_POINT('Ctrl Pts',(51.3073800633105,-2.94322362331098,
125.793457186192));
#234078=CARTESIAN_POINT('Ctrl Pts',(51.0289324394976,-5.80669923360788,
130.572062305503));
#234079=CARTESIAN_POINT('Ctrl Pts',(50.7504848156848,-3.33410192124705,
135.564138225197));
#234080=CARTESIAN_POINT('Ctrl Pts',(50.4720371918718,2.20237217680579,136.182211051539));
#234081=CARTESIAN_POINT('Ctrl Pts',(50.193589568059,5.71497383623647,131.858302051661));
#234082=CARTESIAN_POINT('Ctrl Pts',(49.915141944246,3.97579373215887,126.565872361749));
#234083=CARTESIAN_POINT('Ctrl Pts',(49.6366943204332,-1.41694658345112,
125.168406317271));
#234084=CARTESIAN_POINT('Ctrl Pts',(49.3582466966203,-5.50758221055828,
128.950106943089));
#234085=CARTESIAN_POINT('Ctrl Pts',(49.0797990728074,-4.53701884651156,
134.435776110423));
#234086=CARTESIAN_POINT('Ctrl Pts',(48.8013514489945,0.602843191786665,
136.584351844331));
#234087=CARTESIAN_POINT('Ctrl Pts',(48.5229038251815,5.18872178735999,133.421398009111));
#234088=CARTESIAN_POINT('Ctrl Pts',(48.2444562013688,5.006418543501,127.853514660444));
#234089=CARTESIAN_POINT('Ctrl Pts',(47.9660085775558,0.223461235307256,
124.997314589534));
#234090=CARTESIAN_POINT('Ctrl Pts',(47.6875609537429,-4.7648460314457,127.477506128414));
#234091=CARTESIAN_POINT('Ctrl Pts',(47.40911332993,-5.37449257096935,133.014914416948));
#234092=CARTESIAN_POINT('Ctrl Pts',(47.1306657061172,-1.04524299633083,
136.520931755405));
#234093=CARTESIAN_POINT('Ctrl Pts',(46.8522180823042,4.24453382897653,134.773699488214));
#234094=CARTESIAN_POINT('Ctrl Pts',(46.5737704584914,5.6337914224598,129.378838711881));
#234095=CARTESIAN_POINT('Ctrl Pts',(46.2953228346785,1.84586992471411,125.293962926255));
#234096=CARTESIAN_POINT('Ctrl Pts',(46.0168752108656,-3.63831585808481,
126.272873421051));
#234097=CARTESIAN_POINT('Ctrl Pts',(45.7384275870526,-5.77906710891461,
131.415999273987));
#234098=CARTESIAN_POINT('Ctrl Pts',(45.4599799632399,-2.60913800977569,
135.997059081882));
#234099=CARTESIAN_POINT('Ctrl Pts',(45.1815323394269,2.95846145686929,135.806282678493));
#234100=CARTESIAN_POINT('Ctrl Pts',(44.903084715614,5.80737937352832,131.018984258588));
#234101=CARTESIAN_POINT('Ctrl Pts',(44.6246370918012,3.31959935216964,126.034457197533));
#234102=CARTESIAN_POINT('Ctrl Pts',(44.3461894679882,-2.21873030238901,
125.43323835675));
#234103=CARTESIAN_POINT('Ctrl Pts',(44.0677418441753,-5.7181552000533,129.767818479747));
#234104=CARTESIAN_POINT('Ctrl Pts',(43.7892942203624,-3.96287481627985,
135.054930189501));
#234105=CARTESIAN_POINT('Ctrl Pts',(43.5108465965496,1.43409392645716,136.435976114513));
#234106=CARTESIAN_POINT('Ctrl Pts',(43.2323989727367,5.51320041016325,132.641842517543));
#234107=CARTESIAN_POINT('Ctrl Pts',(42.9539513489238,4.52594505174265,127.159152820475));
#234108=CARTESIAN_POINT('Ctrl Pts',(42.6755037251109,-0.620432704521861,
125.026231010632));
#234109=CARTESIAN_POINT('Ctrl Pts',(42.397056101298,-5.19666311515333,128.203128032237));
#234110=CARTESIAN_POINT('Ctrl Pts',(42.1186084774851,-4.99741399406557,
133.770430722483));
#234111=CARTESIAN_POINT('Ctrl Pts',(41.8401608536722,-0.205785549677785,
136.612059886891));
#234112=CARTESIAN_POINT('Ctrl Pts',(41.5617132298594,4.77494976168102,134.11669714467));
#234113=CARTESIAN_POINT('Ctrl Pts',(41.2832656060464,5.36773951131901,128.577458950676));
#234114=CARTESIAN_POINT('Ctrl Pts',(41.0048179822336,1.02783887870806,125.084634598359));
#234115=CARTESIAN_POINT('Ctrl Pts',(40.7263703584206,-4.25659547071474,
126.847959033542));
#234116=CARTESIAN_POINT('Ctrl Pts',(40.4479227346078,-5.62942652880005,
132.24702324348));
#234117=CARTESIAN_POINT('Ctrl Pts',(40.1694751107948,-1.82908961969292,
136.320350978189));
#234118=CARTESIAN_POINT('Ctrl Pts',(39.891027486982,3.65209129391637,135.324753042595));
#234119=CARTESIAN_POINT('Ctrl Pts',(39.6125798631691,5.77717872299504,130.175135301845));
#234120=CARTESIAN_POINT('Ctrl Pts',(39.3341322393562,2.59332113651206,125.603744886877));
#234121=CARTESIAN_POINT('Ctrl Pts',(39.0556846155433,-2.97367188364494,
125.811466264208));
#234122=CARTESIAN_POINT('Ctrl Pts',(38.7772369917304,-5.80800571467979,
130.607413635826));
#234123=CARTESIAN_POINT('Ctrl Pts',(38.4987893679175,-3.30506603077697,
135.584345662267));
#234124=CARTESIAN_POINT('Ctrl Pts',(38.2203417441046,2.23506787395795,136.16870494788));
#234125=CARTESIAN_POINT('Ctrl Pts',(37.9418941202917,5.72128359166147,131.823493856722));
#234126=CARTESIAN_POINT('Ctrl Pts',(37.6634464964789,3.94991918886983,126.541749106207));
#234127=CARTESIAN_POINT('Ctrl Pts',(37.3849988726659,-1.45122798421329,
125.177136094481));
#234128=CARTESIAN_POINT('Ctrl Pts',(37.1065512488531,-5.51876753623267,
128.983667514269));
#234129=CARTESIAN_POINT('Ctrl Pts',(36.8281036250402,-4.51482932923697,
134.463326950183));
#234130=CARTESIAN_POINT('Ctrl Pts',(36.5496560012273,0.6380164696531,136.580575076865));
#234131=CARTESIAN_POINT('Ctrl Pts',(36.2712083774144,5.20455630176915,133.389764299214));
#234132=CARTESIAN_POINT('Ctrl Pts',(35.9927607536015,4.9883631492699,127.82309384212));
#234133=CARTESIAN_POINT('Ctrl Pts',(35.7143131297886,0.188107957679239,
124.996061908681));
#234134=CARTESIAN_POINT('Ctrl Pts',(35.4358655059757,-4.78500925743413,
127.50657273754));
#234135=CARTESIAN_POINT('Ctrl Pts',(35.1574178821628,-5.36093672566315,
133.047589522248));
#234136=CARTESIAN_POINT('Ctrl Pts',(34.87897025835,-1.01042523932657,136.527188531377));
#234137=CARTESIAN_POINT('Ctrl Pts',(34.6005226345371,4.26861767993396,134.747788263399));
#234138=CARTESIAN_POINT('Ctrl Pts',(34.3220750107242,5.62500948490202,129.34457063605));
#234139=CARTESIAN_POINT('Ctrl Pts',(34.0436273869112,1.81229237023524,125.282828687009));
#234140=CARTESIAN_POINT('Ctrl Pts',(33.7651797630984,-3.66583289727342,
126.295104840318));
#234141=CARTESIAN_POINT('Ctrl Pts',(33.4867321392855,-5.77523681808073,
131.451166763527));
#234142=CARTESIAN_POINT('Ctrl Pts',(33.2082845154725,-2.57748023907555,
136.012845436834));
#234143=CARTESIAN_POINT('Ctrl Pts',(32.9298368916598,2.98885476273036,135.788181009863));
#234144=CARTESIAN_POINT('Ctrl Pts',(32.6513892678468,5.80857825125962,130.983629115531));
#234145=CARTESIAN_POINT('Ctrl Pts',(32.3729416440339,3.29050209170421,126.014338229324));
#234146=CARTESIAN_POINT('Ctrl Pts',(32.094494020221,-2.25138474016344,125.446843912307));
#234147=CARTESIAN_POINT('Ctrl Pts',(31.8160463964081,-5.72435898208005,
129.802645718181));
#234148=CARTESIAN_POINT('Ctrl Pts',(31.5375987725953,-3.93692696994811,
135.078974580096));
#234149=CARTESIAN_POINT('Ctrl Pts',(31.2591511487823,1.46834859799131,136.427142036947));
#234150=CARTESIAN_POINT('Ctrl Pts',(30.9807035249695,5.52428353719365,132.608248057529));
#234151=CARTESIAN_POINT('Ctrl Pts',(30.7022559011566,4.50367178196922,127.131669645585));
#234152=CARTESIAN_POINT('Ctrl Pts',(30.4238082773436,-0.655594324287056,
125.030114815962));
#234153=CARTESIAN_POINT('Ctrl Pts',(30.1453606535308,-5.21240127408669,
128.234809790423));
#234154=CARTESIAN_POINT('Ctrl Pts',(29.8669130297179,-4.97926609295916,
133.80079644549));
#234155=CARTESIAN_POINT('Ctrl Pts',(29.588465405905,-0.170428623074124,
136.613204958723));
#234156=CARTESIAN_POINT('Ctrl Pts',(29.3100177820921,4.79502442551506,134.087569300254));
#234157=CARTESIAN_POINT('Ctrl Pts',(29.0315701582792,5.35408427702179,128.544825256054));
#234158=CARTESIAN_POINT('Ctrl Pts',(28.7531225344664,0.99300223950345,125.078483824645));
#234159=CARTESIAN_POINT('Ctrl Pts',(28.4746749106534,-4.28060034526213,
126.873943441297));
#234160=CARTESIAN_POINT('Ctrl Pts',(28.1962272868406,-5.6205403316845,132.281264431386));
#234161=CARTESIAN_POINT('Ctrl Pts',(27.9177796630277,-1.79547833194873,
136.331382967337));
#234162=CARTESIAN_POINT('Ctrl Pts',(27.6393320392148,3.67954054085496,135.3024379739));
#234163=CARTESIAN_POINT('Ctrl Pts',(27.3608844154018,5.77324141216173,130.139979633288));
#234164=CARTESIAN_POINT('Ctrl Pts',(27.082436791589,2.56161546421434,125.58805496041));
#234165=CARTESIAN_POINT('Ctrl Pts',(26.8039891677761,-3.00400995347367,
125.82966035576));
#234166=CARTESIAN_POINT('Ctrl Pts',(26.5255415439632,-5.80909697796402,
130.642772264091));
#234167=CARTESIAN_POINT('Ctrl Pts',(26.2470939201503,-3.27590766986969,
135.604375975235));
#234168=CARTESIAN_POINT('Ctrl Pts',(25.9686462963375,2.2676807498481,136.155000066467));
#234169=CARTESIAN_POINT('Ctrl Pts',(25.6901986725246,5.727381342819,131.788647897428));
#234170=CARTESIAN_POINT('Ctrl Pts',(25.4117510487116,3.92389827987267,126.517783803302));
#234171=CARTESIAN_POINT('Ctrl Pts',(25.1333034248988,-1.48545560918882,
125.186074390566));
#234172=CARTESIAN_POINT('Ctrl Pts',(24.8548558010858,-5.5297483619465,129.017295551901));
#234173=CARTESIAN_POINT('Ctrl Pts',(24.576408177273,-4.49247251330123,134.490742205601));
#234174=CARTESIAN_POINT('Ctrl Pts',(24.2979605534601,0.673166105584617,
136.576584269648));
#234175=CARTESIAN_POINT('Ctrl Pts',(24.0195129296472,5.22019795943058,133.358034786234));
#234176=CARTESIAN_POINT('Ctrl Pts',(23.7410653058343,4.97012290940784,127.792783495733));
#234177=CARTESIAN_POINT('Ctrl Pts',(23.4626176820214,0.152747709641667,
124.995024456474));
#234178=CARTESIAN_POINT('Ctrl Pts',(23.1841700582085,-4.80499517314482,
127.53576154741));
#234179=CARTESIAN_POINT('Ctrl Pts',(22.9057224343956,-5.34718222887511,
133.080181503877));
#234180=CARTESIAN_POINT('Ctrl Pts',(22.6272748105827,-0.975570040643468,
136.533233245855));
#234181=CARTESIAN_POINT('Ctrl Pts',(22.3488271867698,4.29254335569345,134.721730913422));
#234182=CARTESIAN_POINT('Ctrl Pts',(22.070379562957,5.61601911054919,129.310356653276));
#234183=CARTESIAN_POINT('Ctrl Pts',(21.791931939144,1.77864766059611,125.27189905016));
#234184=CARTESIAN_POINT('Ctrl Pts',(21.5134843153312,-3.69321409767591,
126.317503351717));
#234185=CARTESIAN_POINT('Ctrl Pts',(21.2350366915183,-5.77119252372273,
131.486310285425));
#234186=CARTESIAN_POINT('Ctrl Pts',(20.9565890677054,-2.54572695889727,
136.028438789465));
#234187=CARTESIAN_POINT('Ctrl Pts',(20.6781414438925,3.01913731547902,135.769894663934));
#234188=CARTESIAN_POINT('Ctrl Pts',(20.3996938200796,5.80956188998761,130.948267329615));
#234189=CARTESIAN_POINT('Ctrl Pts',(20.1212461962667,3.26128290047392,125.994396757156));
#234190=CARTESIAN_POINT('Ctrl Pts',(19.8427985724538,-2.28395575204823,
125.460647992615));
#234191=CARTESIAN_POINT('Ctrl Pts',(19.5643509486409,-5.7303506458796,129.837510075529));
#234192=CARTESIAN_POINT('Ctrl Pts',(19.285903324828,-3.91083323933969,135.102860573299));
#234193=CARTESIAN_POINT('Ctrl Pts',(19.0074557010152,1.50254885932817,136.418099605148));
#234194=CARTESIAN_POINT('Ctrl Pts',(18.7290080772022,5.53516195986603,132.574586753804));
#234195=CARTESIAN_POINT('Ctrl Pts',(18.4505604533894,4.48123162698169,127.104322563612));
#234196=CARTESIAN_POINT('Ctrl Pts',(18.1721128295765,-0.690731650763477,
125.034212588094));
#234197=CARTESIAN_POINT('Ctrl Pts',(17.8936652057636,-5.22794628557398,
128.26658676426));
#234198=CARTESIAN_POINT('Ctrl Pts',(17.6152175819507,-4.96093368331654,
133.831051134467));
#234199=CARTESIAN_POINT('Ctrl Pts',(17.3367699581378,-0.135065381175154,
136.614134781694));
#234200=CARTESIAN_POINT('Ctrl Pts',(17.0583223343249,4.81492140795562,134.058319795333));
#234201=CARTESIAN_POINT('Ctrl Pts',(16.779874710512,5.34023064516271,128.512275289347));
#234202=CARTESIAN_POINT('Ctrl Pts',(16.5014270866992,0.958128804235671,
125.0725452254));
#234203=CARTESIAN_POINT('Ctrl Pts',(16.2229794628862,-4.30444660058956,
126.900073492105));
#234204=CARTESIAN_POINT('Ctrl Pts',(15.9445318390734,-5.61144586338,132.315450892077));
#234205=CARTESIAN_POINT('Ctrl Pts',(15.6660842152604,-1.76180051209467,
136.342210150638));
#234206=CARTESIAN_POINT('Ctrl Pts',(15.3876365914476,3.70685344106567,135.279956227294));
#234207=CARTESIAN_POINT('Ctrl Pts',(15.1091889676347,5.76909017174479,130.104848583611));
#234208=CARTESIAN_POINT('Ctrl Pts',(14.8307413438218,2.52981487031356,125.572558326068));
#234209=CARTESIAN_POINT('Ctrl Pts',(14.5522937200089,-3.03423670860886,
125.848038786661));
#234210=CARTESIAN_POINT('Ctrl Pts',(14.273846096196,-5.80997298302346,130.678136880072));
#234211=CARTESIAN_POINT('Ctrl Pts',(13.9953984723831,-3.24662791899898,
135.624228421867));
#234212=CARTESIAN_POINT('Ctrl Pts',(13.7169508485702,2.30020959599411,136.141096915141));
#234213=CARTESIAN_POINT('Ctrl Pts',(13.4385032247574,5.73326686375462,131.753765465006));
#234214=CARTESIAN_POINT('Ctrl Pts',(13.1600556009444,3.89773196938174,126.493977341077));
#234215=CARTESIAN_POINT('Ctrl Pts',(12.8816079771316,-1.51962819006047,
125.195220874312));
#234216=CARTESIAN_POINT('Ctrl Pts',(12.6031603533186,-5.54052428080121,
129.050989809886));
#234217=CARTESIAN_POINT('Ctrl Pts',(12.3247127295058,-4.46994922714442,
134.518020860792));
#234218=CARTESIAN_POINT('Ctrl Pts',(12.0462651056929,0.708290797098533,
136.572379570561));
#234219=CARTESIAN_POINT('Ctrl Pts',(11.76781748188,5.23564618073708,133.326210645918));
#234220=CARTESIAN_POINT('Ctrl Pts',(11.4893698580671,4.95169849981347,127.762584744442));
#234221=CARTESIAN_POINT('Ctrl Pts',(11.2109222342542,0.117381801481337,
124.994202271355));
#234222=CARTESIAN_POINT('Ctrl Pts',(10.9324746104413,-4.82480303799234,
127.565071476419));
#234223=CARTESIAN_POINT('Ctrl Pts',(10.6540269866284,-5.33322959028317,
133.112689154126));
#234224=CARTESIAN_POINT('Ctrl Pts',(10.3755793628155,-0.940678691853753,
136.539065674851));
#234225=CARTESIAN_POINT('Ctrl Pts',(10.0971317390026,4.31630996968034,134.695528403849));
#234226=CARTESIAN_POINT('Ctrl Pts',(9.81868411518972,5.60682063254294,129.276198031366));
#234227=CARTESIAN_POINT('Ctrl Pts',(9.54023649137686,1.74493704251384,125.261174420708));
#234228=CARTESIAN_POINT('Ctrl Pts',(9.26178886756394,-3.72045844467185,
126.340068125262));
#234229=CARTESIAN_POINT('Ctrl Pts',(8.98334124375105,-5.76693437570339,
131.52142853743));
#234230=CARTESIAN_POINT('Ctrl Pts',(8.70489361993813,-2.51387934587036,
136.043838561958));
#234231=CARTESIAN_POINT('Ctrl Pts',(8.42644599612531,3.0493079929842,135.751424318317));
#234232=CARTESIAN_POINT('Ctrl Pts',(8.14799837231237,5.81033025326331,130.912900211183));
#234233=CARTESIAN_POINT('Ctrl Pts',(7.86955074849947,3.23194286120641,125.974633519968));
#234234=CARTESIAN_POINT('Ctrl Pts',(7.59110312468663,-2.3164421311127,125.47465008616));
#234235=CARTESIAN_POINT('Ctrl Pts',(7.31265550087371,-5.73612996942864,
129.872410259879));
#234236=CARTESIAN_POINT('Ctrl Pts',(7.0342078770608,-3.88459459136738,135.126587284006));
#234237=CARTESIAN_POINT('Ctrl Pts',(6.75576025324794,1.53669344316449,136.408849154185));
#234238=CARTESIAN_POINT('Ctrl Pts',(6.47731262943506,5.54583527507644,132.540859853697));
#234239=CARTESIAN_POINT('Ctrl Pts',(6.19886500562214,4.45862541830825,127.077112587908));
#234240=CARTESIAN_POINT('Ctrl Pts',(5.92041738180924,-0.725843381924555,
125.038524175185));
#234241=CARTESIAN_POINT('Ctrl Pts',(5.64196975799638,-5.24329757358911,
128.29845777624));
#234242=CARTESIAN_POINT('Ctrl Pts',(5.36352213418349,-4.94241744445191,
133.861193668313));
#234243=CARTESIAN_POINT('Ctrl Pts',(5.08507451037056,-0.0996971343788212,
136.614849321347));
#234244=CARTESIAN_POINT('Ctrl Pts',(4.80662688655771,4.83463997171276,134.028949713759));
#234245=CARTESIAN_POINT('Ctrl Pts',(4.5281792627448,5.32617912909322,128.479810256704));
#234246=CARTESIAN_POINT('Ctrl Pts',(4.24973163893191,0.923219865152705,
125.066819020683));
#234247=CARTESIAN_POINT('Ctrl Pts',(3.97128401511898,-4.32813335306523,
126.926348217707));
#234248=CARTESIAN_POINT('Ctrl Pts',(3.69283639130614,-5.60214346088543,
132.349581358763));
#234249=CARTESIAN_POINT('Ctrl Pts',(3.41438876749324,-1.72805740807474,
136.352832126888));
#234250=CARTESIAN_POINT('Ctrl Pts',(3.13594114368033,3.73402898245891,135.257308635848));
#234251=CARTESIAN_POINT('Ctrl Pts',(2.85749351986744,5.76472515556999,130.06974345461));
#234252=CARTESIAN_POINT('Ctrl Pts',(2.5790458960546,2.49792053319242,125.557255558086));
#234253=CARTESIAN_POINT('Ctrl Pts',(2.30059827224166,-3.06435102898697,
125.866600875889));
#234254=CARTESIAN_POINT('Ctrl Pts',(2.02215064842876,-5.81063369739741,
130.713506173321));
#234255=CARTESIAN_POINT('Ctrl Pts',(1.74370302461591,-3.21722786313679,
135.643902266527));
#234256=CARTESIAN_POINT('Ctrl Pts',(1.46525540080302,2.33265320702766,136.12699600909));
#234257=CARTESIAN_POINT('Ctrl Pts',(1.18680777699008,5.73893993637821,131.718847852038));
#234258=CARTESIAN_POINT('Ctrl Pts',(0.908360153177235,3.87142122699929,
126.47033060169));
#234259=CARTESIAN_POINT('Ctrl Pts',(0.629912529364331,-1.55374446055069,
125.204575206795));
#234260=CARTESIAN_POINT('Ctrl Pts',(0.351464905551429,-5.55109489349118,
129.084749039672));
#234261=CARTESIAN_POINT('Ctrl Pts',(0.0730172817385382,-4.44726030537518,
134.545161904937));
#234262=CARTESIAN_POINT('Ctrl Pts',(-0.205430342074321,0.743389242636492,
136.56796113541));
#234263=CARTESIAN_POINT('Ctrl Pts',(-0.48387796588724,5.25090039324876,
133.294293057522));
#234264=CARTESIAN_POINT('Ctrl Pts',(-0.762325589700153,4.93309060321035,
127.732498707276));
#234265=CARTESIAN_POINT('Ctrl Pts',(-1.040773213513,0.0820115436953976,
124.993595383789));
#234266=CARTESIAN_POINT('Ctrl Pts',(-1.3192208373259,-4.84443211798899,
127.594501438479));
#234267=CARTESIAN_POINT('Ctrl Pts',(-1.5976684611388,-5.31907932690746,
133.145111268411));
#234268=CARTESIAN_POINT('Ctrl Pts',(-1.8761160849517,-0.905752485869179,
136.544685602242));
#234269=CARTESIAN_POINT('Ctrl Pts',(-2.15456370876455,4.33991664121397,
134.669181705622));
#234270=CARTESIAN_POINT('Ctrl Pts',(-2.43301133257747,5.59741439173625,
129.242096036083));
#234271=CARTESIAN_POINT('Ctrl Pts',(-2.71145895639038,1.71116176514775,
125.250655196059));
#234272=CARTESIAN_POINT('Ctrl Pts',(-2.98990658020324,-3.74756492871192,
126.362798324807));
#234273=CARTESIAN_POINT('Ctrl Pts',(-3.26835420401613,-5.76246253181,131.556520218218));
#234274=CARTESIAN_POINT('Ctrl Pts',(-3.54680182782904,-2.48193858011979,
136.059044183669));
#234275=CARTESIAN_POINT('Ctrl Pts',(-3.82524945164193,3.0793656772603,135.732770657435));
#234276=CARTESIAN_POINT('Ctrl Pts',(-4.1036970754548,5.81088331261472,130.877529070775));
#234277=CARTESIAN_POINT('Ctrl Pts',(-4.38214469926771,3.20248306110764,
125.955049250094));
#234278=CARTESIAN_POINT('Ctrl Pts',(-4.66059232308062,-2.34884267356213,
125.488849674089));
#234279=CARTESIAN_POINT('Ctrl Pts',(-4.93903994689347,-5.7416967385722,
129.907344977992));
#234280=CARTESIAN_POINT('Ctrl Pts',(-5.21748757070636,-3.85821199831392,
135.150153833014));
#234281=CARTESIAN_POINT('Ctrl Pts',(-5.49593519451928,1.57078108426016,
136.399391026839));
#234282=CARTESIAN_POINT('Ctrl Pts',(-5.77438281833216,5.55630308732125,
132.507068606974));
#234283=CARTESIAN_POINT('Ctrl Pts',(-6.05283044214503,4.43585399363028,
127.050040726751));
#234284=CARTESIAN_POINT('Ctrl Pts',(-6.33127806595794,-0.76092821669219,
125.043049417465));
#234285=CARTESIAN_POINT('Ctrl Pts',(-6.60972568977086,-5.25845456928442,
128.330421645371));
#234286=CARTESIAN_POINT('Ctrl Pts',(-6.88817331358369,-4.92371806249131,
133.891222930087));
#234287=CARTESIAN_POINT('Ctrl Pts',(-7.16662093739661,-0.0643251932685087,
136.615348551203));
#234288=CARTESIAN_POINT('Ctrl Pts',(-7.44506856120951,4.8541793861078,133.999460143849));
#234289=CARTESIAN_POINT('Ctrl Pts',(-7.72351618502242,5.3119302494974,128.44743136113));
#234290=CARTESIAN_POINT('Ctrl Pts',(-8.00196380883526,0.888276715818123,
125.06130542268));
#234291=CARTESIAN_POINT('Ctrl Pts',(-8.28041143264819,-4.35165972496785,
126.952766644486));
#234292=CARTESIAN_POINT('Ctrl Pts',(-8.55885905646108,-5.59263346890473,
132.383654566726));
#234293=CARTESIAN_POINT('Ctrl Pts',(-8.83730668027396,-1.69425027025207,
136.363248502487));
#234294=CARTESIAN_POINT('Ctrl Pts',(-9.11575430408684,3.76106615803527,
135.234496038775));
#234295=CARTESIAN_POINT('Ctrl Pts',(-9.39420192789976,5.7601465253845,130.034665547118));
#234296=CARTESIAN_POINT('Ctrl Pts',(-9.67264955171265,2.4659336347071,125.542147223509));
#234297=CARTESIAN_POINT('Ctrl Pts',(-9.95109717552551,-3.09435179871079,
125.885345935621));
#234298=CARTESIAN_POINT('Ctrl Pts',(-10.2295447993384,-5.81107909660284,
130.748878833214));
#234299=CARTESIAN_POINT('Ctrl Pts',(-10.5079924231513,-3.18770859171301,
135.663396780189));
#234300=CARTESIAN_POINT('Ctrl Pts',(-10.7864400469642,2.36501038073878,
136.112697870828));
#234301=CARTESIAN_POINT('Ctrl Pts',(-11.0648876707771,5.74440035047196,
131.683896352409));
#234302=CARTESIAN_POINT('Ctrl Pts',(-11.34333529459,3.84496702767957,126.446844461378));
#234303=CARTESIAN_POINT('Ctrl Pts',(-11.6217829184029,-1.58780315646856,
125.214137041385));
#234304=CARTESIAN_POINT('Ctrl Pts',(-11.9002305422157,-5.56145980831845,
129.118571990297));
#234305=CARTESIAN_POINT('Ctrl Pts',(-12.1786781660286,-4.42440658873985,
134.572164332316));
#234306=CARTESIAN_POINT('Ctrl Pts',(-12.4571257898416,0.778460141612691,
136.563329127923));
#234307=CARTESIAN_POINT('Ctrl Pts',(-12.7355734136544,5.26596003171537,
133.262283203764));
#234308=CARTESIAN_POINT('Ctrl Pts',(-13.0140210374673,4.91429990912079,
127.702526499083));
#234309=CARTESIAN_POINT('Ctrl Pts',(-13.2924686612802,0.0466382469415425,
124.993203816266));
#234310=CARTESIAN_POINT('Ctrl Pts',(-13.5709162850931,-4.86388168577195,
127.624050343051));
#234311=CARTESIAN_POINT('Ctrl Pts',(-13.849363908906,-5.30473196309121,
133.177446645321));
#234312=CARTESIAN_POINT('Ctrl Pts',(-14.1278115327188,-0.87079271689315,
136.550092819781));
#234313=CARTESIAN_POINT('Ctrl Pts',(-14.4062591565318,4.36336249554048,
134.642691795028));
#234314=CARTESIAN_POINT('Ctrl Pts',(-14.6847067803446,5.58780073668082,
129.20805193109));
#234315=CARTESIAN_POINT('Ctrl Pts',(-14.9631544041576,1.67732308005318,
125.240341766008));
#234316=CARTESIAN_POINT('Ctrl Pts',(-15.2416020279704,-3.77453254535539,
126.385693108075));
#234317=CARTESIAN_POINT('Ctrl Pts',(-15.5200496517834,-5.75777715774833,
131.591584027456));
#234318=CARTESIAN_POINT('Ctrl Pts',(-15.7984972755962,-2.44990584522241,
136.074055091149));
#234319=CARTESIAN_POINT('Ctrl Pts',(-16.0769448994091,3.1093092545088,135.713934372506));
#234320=CARTESIAN_POINT('Ctrl Pts',(-16.355392523222,5.81122104754806,130.842155219084));
#234321=CARTESIAN_POINT('Ctrl Pts',(-16.6338401470349,3.17290459182133,
125.935644673236));
#234322=CARTESIAN_POINT('Ctrl Pts',(-16.9122877708478,-2.38115617878252,
125.50324623023));
#234323=CARTESIAN_POINT('Ctrl Pts',(-17.1907353946607,-5.74705074703162,
129.94231293535));
#234324=CARTESIAN_POINT('Ctrl Pts',(-17.4691830184736,-3.83168643779603,
135.173559347056));
#234325=CARTESIAN_POINT('Ctrl Pts',(-17.7476306422864,1.6048105194851,136.389725573584));
#234326=CARTESIAN_POINT('Ctrl Pts',(-18.0260782660994,5.56656500871184,
132.473214265779));
#234327=CARTESIAN_POINT('Ctrl Pts',(-18.3045258899123,4.4129181967513,127.023107983299));
#234328=CARTESIAN_POINT('Ctrl Pts',(-18.5829735137251,-0.795984854984928,
125.047788147249));
#234329=CARTESIAN_POINT('Ctrl Pts',(-18.861421137538,-5.27341671101187,
128.362477187221));
#234330=CARTESIAN_POINT('Ctrl Pts',(-19.1398687613509,-4.90483623034722,
133.921137807042));
#234331=CARTESIAN_POINT('Ctrl Pts',(-19.4183163851638,-0.0289508685644962,
136.615632452765));
#234332=CARTESIAN_POINT('Ctrl Pts',(-19.6967640089767,4.87353892710056,
133.969852178351));
#234333=CARTESIAN_POINT('Ctrl Pts',(-19.9752116327896,5.29748453437273,
128.415139802436));
#234334=CARTESIAN_POINT('Ctrl Pts',(-20.2536592566025,0.853300651063172,
125.056004635698));
#234335=CARTESIAN_POINT('Ctrl Pts',(-20.5321068804154,-4.37502484451904,
126.979327793496));
#234336=CARTESIAN_POINT('Ctrl Pts',(-20.8105545042282,-5.58291623983416,
132.417669253371));
#234337=CARTESIAN_POINT('Ctrl Pts',(-21.0890021280412,-1.66038035136256,
136.37345889145));
#234338=CARTESIAN_POINT('Ctrl Pts',(-21.367449751854,3.78796396592178,135.211519281404));
#234339=CARTESIAN_POINT('Ctrl Pts',(-21.6458973756669,5.75535445085128,
129.999616160961));
#234340=CARTESIAN_POINT('Ctrl Pts',(-21.9243449994798,2.43385536014432,
125.527233882186));
#234341=CARTESIAN_POINT('Ctrl Pts',(-22.2027926232928,-3.12423790609075,
125.904273271251));
#234342=CARTESIAN_POINT('Ctrl Pts',(-22.4812402471056,-5.81130916413533,
130.784253549004));
#234343=CARTESIAN_POINT('Ctrl Pts',(-22.7596878709185,-3.15807119857507,
135.682711240481));
#234344=CARTESIAN_POINT('Ctrl Pts',(-23.0381354947314,2.39727991812053,
136.098203030175));
#234345=CARTESIAN_POINT('Ctrl Pts',(-23.3165831185443,5.74964790369824,
131.648912261261));
#234346=CARTESIAN_POINT('Ctrl Pts',(-23.5950307423572,3.81837035169266,
126.423519790431));
#234347=CARTESIAN_POINT('Ctrl Pts',(-23.8734783661701,-1.62180301575654,
125.223906023766));
#234348=CARTESIAN_POINT('Ctrl Pts',(-24.151925989983,-5.57161864120731,
129.15245740844));
#234349=CARTESIAN_POINT('Ctrl Pts',(-24.4303736137958,-4.4013889240913,
134.599027142342));
#234350=CARTESIAN_POINT('Ctrl Pts',(-24.7088212376087,0.813502194462058,
136.558483719739));
#234351=CARTESIAN_POINT('Ctrl Pts',(-24.9872688614217,5.28082453809644,
133.230182270781));
#234352=CARTESIAN_POINT('Ctrl Pts',(-25.2657164852345,4.89532711384086,
127.672669230493));
#234353=CARTESIAN_POINT('Ctrl Pts',(-25.5441641090475,0.0112632219902977,
124.993027583295));
#234354=CARTESIAN_POINT('Ctrl Pts',(-25.8226117328602,-4.88315102063038,
127.65371709519));
#234355=CARTESIAN_POINT('Ctrl Pts',(-26.1010593566733,-5.29018803048126,
133.209694086655));
#234356=CARTESIAN_POINT('Ctrl Pts',(-26.3795069804861,-0.835800680372761,
136.555287127099));
#234357=CARTESIAN_POINT('Ctrl Pts',(-26.6579546042989,4.38664666386508,
134.616059653661));
#234358=CARTESIAN_POINT('Ctrl Pts',(-26.9364022281119,5.57798002361419,
129.174066977901));
#234359=CARTESIAN_POINT('Ctrl Pts',(-27.2148498519247,1.64342224113504,
125.23023451272));
#234360=CARTESIAN_POINT('Ctrl Pts',(-27.4932974757377,-3.80136029530733,
126.408751626694));
#234361=CARTESIAN_POINT('Ctrl Pts',(-27.7717450995505,-5.75287842713667,
131.626618665841));
#234362=CARTESIAN_POINT('Ctrl Pts',(-28.0501927233634,-2.41778232816299,
136.088870728161));
#234363=CARTESIAN_POINT('Ctrl Pts',(-28.3286403471763,3.13913761515943,
135.694916161515));
#234364=CARTESIAN_POINT('Ctrl Pts',(-28.6070879709892,5.8113434455484,130.8067799669));
#234365=CARTESIAN_POINT('Ctrl Pts',(-28.8855355948021,3.14320854938853,
125.916420508438));
#234366=CARTESIAN_POINT('Ctrl Pts',(-29.163983218615,-2.41338144938502,
125.517839221114));
#234367=CARTESIAN_POINT('Ctrl Pts',(-29.4424308424279,-5.75219179641212,
129.977312836202));
#234368=CARTESIAN_POINT('Ctrl Pts',(-29.7208784662408,-3.80501889272807,
135.196802958832));
#234369=CARTESIAN_POINT('Ctrl Pts',(-29.9993260900537,1.6387804878663,136.379853152576));
#234370=CARTESIAN_POINT('Ctrl Pts',(-30.2777737138665,5.576620658989,132.439298084597));
#234371=CARTESIAN_POINT('Ctrl Pts',(-30.5562213376795,4.38981887756547,
126.996315355552));
#234372=CARTESIAN_POINT('Ctrl Pts',(-30.8346689614924,-0.831011997766135,
125.052740188944));
#234373=CARTESIAN_POINT('Ctrl Pts',(-31.1131165853052,-5.2881834443438,
128.394623213959));
#234374=CARTESIAN_POINT('Ctrl Pts',(-31.3915642091181,-4.88577264769286,
133.950937190672));
#234375=CARTESIAN_POINT('Ctrl Pts',(-31.670011832931,0.00642452892459172,
136.615701015511));
#234376=CARTESIAN_POINT('Ctrl Pts',(-31.9484594567439,4.89271787731614,
133.940126914399));
#234377=CARTESIAN_POINT('Ctrl Pts',(-32.2269070805568,5.28284251901049,
128.382936777197));
#234378=CARTESIAN_POINT('Ctrl Pts',(-32.5053547043697,0.818292966938792,
125.050916856162));
#234379=CARTESIAN_POINT('Ctrl Pts',(-32.7838023281826,-4.3982278459157,
127.006030680504));
#234380=CARTESIAN_POINT('Ctrl Pts',(-33.0622499519955,-5.57299213374921,
132.451624158271));
#234381=CARTESIAN_POINT('Ctrl Pts',(-33.3406975758084,-1.62644890646854,
136.383462915428));
#234382=CARTESIAN_POINT('Ctrl Pts',(-33.6191451996212,3.81472140941051,
135.188379215148));
#234383=CARTESIAN_POINT('Ctrl Pts',(-33.8975928234342,5.75034910954236,
129.964596594906));
#234384=CARTESIAN_POINT('Ctrl Pts',(-34.176040447247,2.40168689817613,125.512516086734));
#234385=CARTESIAN_POINT('Ctrl Pts',(-34.4544880710599,-3.15400824368619,
125.923382181419));
#234386=CARTESIAN_POINT('Ctrl Pts',(-34.7329356948729,-5.81132389146964,
130.81962900987));
#234387=CARTESIAN_POINT('Ctrl Pts',(-35.0113833186857,-3.1283167819475,
135.701844931696));
#234388=CARTESIAN_POINT('Ctrl Pts',(-35.2898309424986,2.42946062341331,
136.083512024245));
#234389=CARTESIAN_POINT('Ctrl Pts',(-35.5682785663115,5.75468240160701,
131.613896874941));
#234390=CARTESIAN_POINT('Ctrl Pts',(-35.8467261901244,3.79163218458816,
126.400357453152));
#234391=CARTESIAN_POINT('Ctrl Pts',(-36.1251738139373,-1.65574277853735,
125.233881791944));
#234392=CARTESIAN_POINT('Ctrl Pts',(-36.4036214377501,-5.58157101571846,
129.186404038463));
#234393=CARTESIAN_POINT('Ctrl Pts',(-36.6820690615631,-4.37820816435757,
134.625749339604));
#234394=CARTESIAN_POINT('Ctrl Pts',(-36.960516685376,0.848514102688449,
136.553425090409));
#234395=CARTESIAN_POINT('Ctrl Pts',(-37.2389643091888,5.29549336158222,
133.197991448084));
#234396=CARTESIAN_POINT('Ctrl Pts',(-37.5174119330018,4.87617292041449,
127.64292800788));
#234397=CARTESIAN_POINT('Ctrl Pts',(-37.7958595568146,-0.0241122203237842,
124.993066691407));
#234398=CARTESIAN_POINT('Ctrl Pts',(-38.0743071806275,-4.90223940853195,
127.683500595584));
#234399=CARTESIAN_POINT('Ctrl Pts',(-38.3527548044404,-5.27544806800837,
133.241852397473));
#234400=CARTESIAN_POINT('Ctrl Pts',(-38.6312024282533,-0.800777672950798,
136.560268331721));
#234401=CARTESIAN_POINT('Ctrl Pts',(-38.9096500520661,4.40976828338437,
134.589286268384));
#234402=CARTESIAN_POINT('Ctrl Pts',(-39.1880976758791,5.56795261644649,
129.140142435842));
#234403=CARTESIAN_POINT('Ctrl Pts',(-39.4665452996919,1.6094605046014,125.220333810727));
#234404=CARTESIAN_POINT('Ctrl Pts',(-39.7449929235049,-3.82804718445556,
126.43197302622));
#234405=CARTESIAN_POINT('Ctrl Pts',(-40.0234405473177,-5.74776652149929,
131.661622835152));
#234406=CARTESIAN_POINT('Ctrl Pts',(-40.3018881711306,-2.38556921929025,
136.103490545709));
#234407=CARTESIAN_POINT('Ctrl Pts',(-40.5803357949436,3.16884965391132,
135.675716729192));
#234408=CARTESIAN_POINT('Ctrl Pts',(-40.8587834187564,5.81125050208024,
130.771404625066));
#234409=CARTESIAN_POINT('Ctrl Pts',(-41.1372310425694,3.11339603420704,
125.897377468058));
#234410=CARTESIAN_POINT('Ctrl Pts',(-41.4156786663821,-2.4455172912504,
125.532628105994));
#234411=CARTESIAN_POINT('Ctrl Pts',(-41.6941262901951,-5.75711969621025,
130.012343383614));
#234412=CARTESIAN_POINT('Ctrl Pts',(-41.9725739140079,-3.77821035128576,
135.219883807042));
#234413=CARTESIAN_POINT('Ctrl Pts',(-42.2510215378209,1.67268973063362,
136.369774129642));
#234414=CARTESIAN_POINT('Ctrl Pts',(-42.5294691616338,5.58646966553678,
132.405321320208));
#234415=CARTESIAN_POINT('Ctrl Pts',(-42.8079167854466,4.366556892027,126.969663836325));
#234416=CARTESIAN_POINT('Ctrl Pts',(-43.0863644092596,-0.866008347092154,
125.057905359049));
#234417=CARTESIAN_POINT('Ctrl Pts',(-43.3648120330724,-5.3027542220935,
128.426858534403));
#234418=CARTESIAN_POINT('Ctrl Pts',(-43.6432596568854,-4.86652802093628,
133.98061997675));
#234419=CARTESIAN_POINT('Ctrl Pts',(-43.9217072806982,0.0417996883503892,
136.615554236903));
#234420=CARTESIAN_POINT('Ctrl Pts',(-44.2001549045111,4.9117155260715,133.910285453475));
#234421=CARTESIAN_POINT('Ctrl Pts',(-44.478602528324,5.26800474597596,128.350823478709));
#234422=CARTESIAN_POINT('Ctrl Pts',(-44.7570501521369,0.783254960667603,
125.046042272601));
#234423=CARTESIAN_POINT('Ctrl Pts',(-45.0354977759497,-4.42126786936209,
127.032874316024));
#234424=CARTESIAN_POINT('Ctrl Pts',(-45.3139453997627,-5.56286151839129,
132.485518023215));
#234425=CARTESIAN_POINT('Ctrl Pts',(-45.5923930235756,-1.59245719291215,
136.393260203719));
#234426=CARTESIAN_POINT('Ctrl Pts',(-45.8708406473885,3.84133749699455,
135.165076697471));
#234427=CARTESIAN_POINT('Ctrl Pts',(-46.1492882712014,5.74513068693249,
129.929608146614));
#234428=CARTESIAN_POINT('Ctrl Pts',(-46.4277358950142,2.3694294408167,125.497994382526));
#234429=CARTESIAN_POINT('Ctrl Pts',(-46.7061835188271,-3.18366170834627,
125.942671958037));
#234430=CARTESIAN_POINT('Ctrl Pts',(-46.98463114264,-5.81112327806003,130.85500390496));
#234431=CARTESIAN_POINT('Ctrl Pts',(-47.263078766453,-3.09844644439114,
135.720797144829));
#234432=CARTESIAN_POINT('Ctrl Pts',(-47.5415263902657,2.46155130414924,
136.068625397419));
#234433=CARTESIAN_POINT('Ctrl Pts',(-47.8199740140787,5.75950365764311,
131.578851490957));
#234434=CARTESIAN_POINT('Ctrl Pts',(-48.0984216378915,3.76475351715869,
126.377358307829));
#234435=CARTESIAN_POINT('Ctrl Pts',(-48.3768692617045,-1.6896211871606,
125.244063976264));
#234436=CARTESIAN_POINT('Ctrl Pts',(-48.6553168855173,-5.59131656306301,
129.220410622463));
#234437=CARTESIAN_POINT('Ctrl Pts',(-48.9337645093303,-4.35486516851022,
134.652329933902));
#234438=CARTESIAN_POINT('Ctrl Pts',(-49.2122121331431,0.883494568912716,
136.548153427379));
#234439=CARTESIAN_POINT('Ctrl Pts',(-49.4906597569561,5.3099659586141,133.165711928516));
#234440=CARTESIAN_POINT('Ctrl Pts',(-49.7691073807689,4.85683803860733,
127.613303933314));
#234441=CARTESIAN_POINT('Ctrl Pts',(-50.0475550045819,-0.0594867691506708,
124.993321139153));
#234442=CARTESIAN_POINT('Ctrl Pts',(-50.3260026283946,-4.92114614214944,
127.713399740592));
#234443=CARTESIAN_POINT('Ctrl Pts',(-50.6044502522077,-5.26051262186729,
133.273920386136));
#234444=CARTESIAN_POINT('Ctrl Pts',(-50.8828978760204,-0.765724992417492,
136.565036249065));
#234445=CARTESIAN_POINT('Ctrl Pts',(-51.1613454998334,4.4327264973184,134.562372631296));
#234446=CARTESIAN_POINT('Ctrl Pts',(-51.4397931236463,5.55771888674681,
129.106279562002));
#234447=CARTESIAN_POINT('Ctrl Pts',(-51.7182407474591,1.57543912891688,
125.210640026899));
#234448=CARTESIAN_POINT('Ctrl Pts',(-51.9966883712721,-3.85459222390762,
126.455356446176));
#234449=CARTESIAN_POINT('Ctrl Pts',(-52.2751359950849,-5.7424416302597,
131.696595238295));
#234450=CARTESIAN_POINT('Ctrl Pts',(-52.5535836188979,-2.35326771227282,
136.117914002047));
#234451=CARTESIAN_POINT('Ctrl Pts',(-52.8320312427106,3.19844426977395,
135.656336786975));
#234452=CARTESIAN_POINT('Ctrl Pts',(-53.1104788665238,5.81094222058764,
130.736030504428));
#234453=CARTESIAN_POINT('Ctrl Pts',(-53.3889264903363,3.08346815099054,
125.878516257743));
#234454=CARTESIAN_POINT('Ctrl Pts',(-53.6673741141495,-2.47756251357323,
125.547612336859));
#234455=CARTESIAN_POINT('Ctrl Pts',(-53.9458217379622,-5.76183426382087,
130.047403279515));
#234456=CARTESIAN_POINT('Ctrl Pts',(-54.2242693617753,-3.75126180686946,
135.242801036416));
#234457=CARTESIAN_POINT('Ctrl Pts',(-54.502716985588,1.70653699126786,136.359488878264));
#234458=CARTESIAN_POINT('Ctrl Pts',(-54.7811646094011,5.59611166339667,
132.371285231631));
#234459=CARTESIAN_POINT('Ctrl Pts',(-55.0596122332138,4.3431331021171,126.943154413196));
#234460=CARTESIAN_POINT('Ctrl Pts',(-55.3380598570268,-0.900972606160421,
125.063283466166));
#234461=CARTESIAN_POINT('Ctrl Pts',(-55.6165074808396,-5.31712850433539,
128.459181954061));
#234462=CARTESIAN_POINT('Ctrl Pts',(-55.8949551046525,-4.84710306319425,
134.01018506537));
#234463=CARTESIAN_POINT('Ctrl Pts',(-56.1734027284654,0.0771732988733811,
136.615192122377));
#234464=CARTESIAN_POINT('Ctrl Pts',(-56.4518503522783,4.93053116940174,
133.880328901363));
#234465=CARTESIAN_POINT('Ctrl Pts',(-56.7302979760911,5.25297176508825,
128.318801096944));
#234466=CARTESIAN_POINT('Ctrl Pts',(-57.0087455999042,0.748187930595796,
125.041381065643));
#234467=CARTESIAN_POINT('Ctrl Pts',(-57.2871932237169,-4.44414406110167,
127.059857705357));
#234468=CARTESIAN_POINT('Ctrl Pts',(-57.5656408475299,-5.55252476915405,
132.519349592253));
#234469=CARTESIAN_POINT('Ctrl Pts',(-57.8440884713427,-1.55840647026886,
136.402850393281));
#234470=CARTESIAN_POINT('Ctrl Pts',(-58.1225360951557,3.867811242405,135.141612591857));
#234471=CARTESIAN_POINT('Ctrl Pts',(-58.4009837189685,5.73969937639226,
129.894652112598));
#234472=CARTESIAN_POINT('Ctrl Pts',(-58.6794313427815,2.33708418337799,
125.483669307672));
#234473=CARTESIAN_POINT('Ctrl Pts',(-58.9578789665944,-3.21319720125095,
125.962141886319));
#234474=CARTESIAN_POINT('Ctrl Pts',(-59.2363265904072,-5.81070733134035,
130.890376923444));
#234475=CARTESIAN_POINT('Ctrl Pts',(-59.5147742142201,-3.06846129276222,
135.739567177598));
#234476=CARTESIAN_POINT('Ctrl Pts',(-59.793221838033,2.49355077119662,136.053543701326));
#234477=CARTESIAN_POINT('Ctrl Pts',(-60.071669461846,5.76411149315304,131.543777407928));
#234478=CARTESIAN_POINT('Ctrl Pts',(-60.3501170856587,3.73773534540316,
126.354523206705));
#234479=CARTESIAN_POINT('Ctrl Pts',(-60.6285647094717,-1.72343698624942,
125.254452199421));
#234480=CARTESIAN_POINT('Ctrl Pts',(-60.9070123332846,-5.6008549221161,
129.254475900312));
#234481=CARTESIAN_POINT('Ctrl Pts',(-61.1854599570975,-4.33136080153256,
134.678767940282));
#234482=CARTESIAN_POINT('Ctrl Pts',(-61.4639075809103,0.918442296920838,
136.542668925995));
#234483=CARTESIAN_POINT('Ctrl Pts',(-61.7423552047232,5.32424179290464,
133.133344908207));
#234484=CARTESIAN_POINT('Ctrl Pts',(-62.0208028285362,4.83732318488056,
127.583798104527));
#234485=CARTESIAN_POINT('Ctrl Pts',(-62.299250452349,-0.0948591136734494,
124.993790917104));
#234486=CARTESIAN_POINT('Ctrl Pts',(-62.5776980761619,-4.93987052088691,
127.743413422294));
#234487=CARTESIAN_POINT('Ctrl Pts',(-62.8561456999749,-5.24538224549645,
133.305896864355));
#234488=CARTESIAN_POINT('Ctrl Pts',(-63.1345933237877,-0.730643937663188,
136.569590702456));
#234489=CARTESIAN_POINT('Ctrl Pts',(-63.4130409476006,4.45552045494177,
134.53531973969));
#234490=CARTESIAN_POINT('Ctrl Pts',(-63.6914885714135,5.5472792137301,129.072479611178));
#234491=CARTESIAN_POINT('Ctrl Pts',(-63.9699361952264,1.54135937475606,
125.201153520444));
#234492=CARTESIAN_POINT('Ctrl Pts',(-64.2483838190392,-3.88099443002729,
126.478901020081));
#234493=CARTESIAN_POINT('Ctrl Pts',(-64.5268314428522,-5.73690395073373,
131.731534579357));
#234494=CARTESIAN_POINT('Ctrl Pts',(-64.805279066665,-2.32087900405488,
136.132140562712));
#234495=CARTESIAN_POINT('Ctrl Pts',(-65.083726690478,3.22792036610792,135.636777052998));
#234496=CARTESIAN_POINT('Ctrl Pts',(-65.3621743142908,5.81041861249411,
130.700658915789));
#234497=CARTESIAN_POINT('Ctrl Pts',(-65.6406219381037,3.05342600872776,
125.859837576403));
#234498=CARTESIAN_POINT('Ctrl Pts',(-65.9190695619166,-2.50951592890599,
125.562791358466));
#234499=CARTESIAN_POINT('Ctrl Pts',(-66.1975171857295,-5.76633532454392,
130.082491224748));
#234500=CARTESIAN_POINT('Ctrl Pts',(-66.4759648095424,-3.72417425806736,
135.26555379775));
#234501=CARTESIAN_POINT('Ctrl Pts',(-66.7544124333553,1.74032101554631,
136.348997779564));
#234502=CARTESIAN_POINT('Ctrl Pts',(-67.0328600571681,5.60554629528092,
132.337191080086));
#234503=CARTESIAN_POINT('Ctrl Pts',(-67.3113076809811,4.31954837581292,
126.916788068483));
#234504=CARTESIAN_POINT('Ctrl Pts',(-67.5897553047939,-0.935903479357421,
125.068874311009));
#234505=CARTESIAN_POINT('Ctrl Pts',(-67.8682029286069,-5.33130575842519,
128.491592275178));
#234506=CARTESIAN_POINT('Ctrl Pts',(-68.1466505524197,-4.82749849426569,
134.039631360986));
#234507=CARTESIAN_POINT('Ctrl Pts',(-68.4250981762326,0.112544049711387,
136.614614685353));
#234508=CARTESIAN_POINT('Ctrl Pts',(-68.7035458000455,4.94916411008632,
133.850258368115));
#234509=CARTESIAN_POINT('Ctrl Pts',(-68.9819934238584,5.23774413340002,
128.286870818499));
#234510=CARTESIAN_POINT('Ctrl Pts',(-69.2604410476712,0.713093176145084,
125.036933408012));
#234511=CARTESIAN_POINT('Ctrl Pts',(-69.5388886714842,-4.46685557344872,
127.086979848621));
#234512=CARTESIAN_POINT('Ctrl Pts',(-69.8173362952971,-5.54198226906957,
132.553117611744));
#234513=CARTESIAN_POINT('Ctrl Pts',(-70.09578391911,-1.52429800030071,136.412233128746));
#234514=CARTESIAN_POINT('Ctrl Pts',(-70.3742315429229,3.89414166464747,
135.117987767775));
#234515=CARTESIAN_POINT('Ctrl Pts',(-70.6526791667357,5.73405537918087,
129.859729788164));
#234516=CARTESIAN_POINT('Ctrl Pts',(-70.9311267905487,2.3046523244254,125.469541392991));
#234517=CARTESIAN_POINT('Ctrl Pts',(-71.2095744143614,-3.24261362795168,
125.981791244794));
#234518=CARTESIAN_POINT('Ctrl Pts',(-71.4880220381746,-5.81007606672361,
130.925746754563));
#234519=CARTESIAN_POINT('Ctrl Pts',(-71.7664696619872,-3.03836243817177,
135.758154334473));
#234520=CARTESIAN_POINT('Ctrl Pts',(-72.0449172858002,2.52545783880292,
136.038267494822));
#234521=CARTESIAN_POINT('Ctrl Pts',(-72.3233649096131,5.76850573739207,
131.508675925537));
#234522=CARTESIAN_POINT('Ctrl Pts',(-72.601812533426,3.71057867048956,126.331852995942));
#234523=CARTESIAN_POINT('Ctrl Pts',(-72.8802601572389,-1.75718892274731,
125.265046076474));
#234524=CARTESIAN_POINT('Ctrl Pts',(-73.1587077810518,-5.61018573943046,
129.28859860971));
#234525=CARTESIAN_POINT('Ctrl Pts',(-73.4371554048648,-4.30769593438731,
134.705062379074));
#234526=CARTESIAN_POINT('Ctrl Pts',(-73.7156030286775,0.953355991712339,
136.536971789486));
#234527=CARTESIAN_POINT('Ctrl Pts',(-73.9940506524905,5.33832033545752,
133.100891586529));
#234528=CARTESIAN_POINT('Ctrl Pts',(-74.2724982763033,4.81762908236426,
127.554411614868));
#234529=CARTESIAN_POINT('Ctrl Pts',(-74.5509459001162,-0.130227943157576,
124.994476007852));
#234530=CARTESIAN_POINT('Ctrl Pts',(-74.8293935239292,-4.95841185090586,
127.77354052852));
#234531=CARTESIAN_POINT('Ctrl Pts',(-75.107841147742,-5.23005749955717,
133.337780647228));
#234532=CARTESIAN_POINT('Ctrl Pts',(-75.3862887715549,-0.695535808628632,
136.573931523126));
#234533=CARTESIAN_POINT('Ctrl Pts',(-75.6647363953679,4.4781493116164,134.508128596022));
#234534=CARTESIAN_POINT('Ctrl Pts',(-75.9431840191806,5.53663398424198,
129.038743835842));
#234535=CARTESIAN_POINT('Ctrl Pts',(-76.2216316429937,1.50722250495638,
125.191874642891));
#234536=CARTESIAN_POINT('Ctrl Pts',(-76.5000792668064,-3.90725282447187,
126.502605875483));
#234537=CARTESIAN_POINT('Ctrl Pts',(-76.7785268906195,-5.73115368812196,
131.766439563647));
#234538=CARTESIAN_POINT('Ctrl Pts',(-77.0569745144322,-2.28840429481114,
136.146169700531));
#234539=CARTESIAN_POINT('Ctrl Pts',(-77.3354221382452,3.25727685066645,
135.617038252052));
#234540=CARTESIAN_POINT('Ctrl Pts',(-77.613869762058,5.80967969720196,130.665291169852));
#234541=CARTESIAN_POINT('Ctrl Pts',(-77.8923173858709,3.0232707206408,125.841342116181));
#234542=CARTESIAN_POINT('Ctrl Pts',(-78.1707650096839,-2.54137635320382,
125.57816460835));
#234543=CARTESIAN_POINT('Ctrl Pts',(-78.4492126334967,-5.77062271159095,
130.117605919119));
#234544=CARTESIAN_POINT('Ctrl Pts',(-78.7276602573096,-3.69694870861804,
135.288141247929));
#234545=CARTESIAN_POINT('Ctrl Pts',(-79.0061078811224,1.77404055158998,
136.338301222296));
#234546=CARTESIAN_POINT('Ctrl Pts',(-79.2845555049354,5.61477321158579,
132.303040128944));
#234547=CARTESIAN_POINT('Ctrl Pts',(-79.5630031287483,4.29580358705489,
126.8905657792));
#234548=CARTESIAN_POINT('Ctrl Pts',(-79.8414507525611,-0.970799672307275,
125.074677686406));
#234549=CARTESIAN_POINT('Ctrl Pts',(-80.1198983763742,-5.34528545901998,
128.524088296775));
#234550=CARTESIAN_POINT('Ctrl Pts',(-80.3983460001869,-4.80771504060458,
134.068957772455));
#234551=CARTESIAN_POINT('Ctrl Pts',(-80.6767936239998,0.147910630189091,
136.613821947228));
#234552=CARTESIAN_POINT('Ctrl Pts',(-80.9552412478128,4.96761365767528,
133.820074968005));
#234553=CARTESIAN_POINT('Ctrl Pts',(-81.2336888716256,5.22232241517632,
128.255033826564));
#234554=CARTESIAN_POINT('Ctrl Pts',(-81.5121364954386,0.6779719977639,125.032699464516));
#234555=CARTESIAN_POINT('Ctrl Pts',(-81.7905841192513,-4.48940156482041,
127.114239740797));
#234556=CARTESIAN_POINT('Ctrl Pts',(-82.0690317430644,-5.53123440879372,
132.586820830401));
#234557=CARTESIAN_POINT('Ctrl Pts',(-82.3474793668772,-1.490133046909,136.421408062431));
#234558=CARTESIAN_POINT('Ctrl Pts',(-82.62592699069,3.92032778803891,135.094203100652));
#234559=CARTESIAN_POINT('Ctrl Pts',(-82.9043746145031,5.72819890443852,
129.824842467372));
#234560=CARTESIAN_POINT('Ctrl Pts',(-83.1828222383158,2.27213506573304,
125.455611161998));
#234561=CARTESIAN_POINT('Ctrl Pts',(-83.4612698621288,-3.27190989841242,
126.001619305352));
#234562=CARTESIAN_POINT('Ctrl Pts',(-83.7397174859417,-5.80922950760163,
130.961112087674));
#234563=CARTESIAN_POINT('Ctrl Pts',(-84.0181651097544,-3.00815099594316,
135.776557926701));
#234564=CARTESIAN_POINT('Ctrl Pts',(-84.2966127335676,2.55727132464077,
136.022797343974));
#234565=CARTESIAN_POINT('Ctrl Pts',(-84.5750603573801,5.77268622752965,
131.473548344486));
#234566=CARTESIAN_POINT('Ctrl Pts',(-84.8535079811934,3.68328449871872,
126.309348515594));
#234567=CARTESIAN_POINT('Ctrl Pts',(-85.131955605006,-1.79087574596318,
125.275845214866));
#234568=CARTESIAN_POINT('Ctrl Pts',(-85.4104032288191,-5.61930866924928,
129.322777486226));
#234569=CARTESIAN_POINT('Ctrl Pts',(-85.6888508526319,-4.28387144398495,
134.731212275928));
#234570=CARTESIAN_POINT('Ctrl Pts',(-85.9672984764448,0.98823435954663,
136.531062228962));
#234571=CARTESIAN_POINT('Ctrl Pts',(-86.2457461002577,5.35220106458756,
133.068353166051));
#234572=CARTESIAN_POINT('Ctrl Pts',(-86.5241937240705,4.79775646083024,
127.525145553266));
#234573=CARTESIAN_POINT('Ctrl Pts',(-86.8026413478836,-0.165591946996939,
124.995376386011));
#234574=CARTESIAN_POINT('Ctrl Pts',(-87.0810889716963,-4.97676944515001,
127.803779942897));
#234575=CARTESIAN_POINT('Ctrl Pts',(-87.3595365955093,-5.21453895191432,
133.36957055329));
#234576=CARTESIAN_POINT('Ctrl Pts',(-87.6379842193221,-0.660401906259044,
136.578058550223));
#234577=CARTESIAN_POINT('Ctrl Pts',(-87.916431843135,4.50061222882128,134.480800207869));
#234578=CARTESIAN_POINT('Ctrl Pts',(-88.1948794669479,5.52578359274576,
129.005073486085));
#234579=CARTESIAN_POINT('Ctrl Pts',(-88.4733270907608,1.47302978447255,
125.182803738068));
#234580=CARTESIAN_POINT('Ctrl Pts',(-88.7517747145737,-3.93336643422502,
126.526470133988));
#234581=CARTESIAN_POINT('Ctrl Pts',(-89.0302223383866,-5.7251910555031,
131.801308897747));
#234582=CARTESIAN_POINT('Ctrl Pts',(-89.3086699621995,-2.25584478790559,
136.16000089565));
#234583=CARTESIAN_POINT('Ctrl Pts',(-89.5871175860123,3.28651263563227,
135.597121115567));
#234584=CARTESIAN_POINT('Ctrl Pts',(-89.8655652098253,5.80872550209253,
130.629928577187));
#234585=CARTESIAN_POINT('Ctrl Pts',(-90.1440128336381,2.99300340414587,
125.823030562435));
#234586=CARTESIAN_POINT('Ctrl Pts',(-90.4224604574511,-2.57314260586573,
125.593731516848));
#234587=CARTESIAN_POINT('Ctrl Pts',(-90.7009080812639,-5.77469626609129,
130.152746061436));
#234588=CARTESIAN_POINT('Ctrl Pts',(-90.9793557050769,-3.66958616737523,
135.310562549967));
#234589=CARTESIAN_POINT('Ctrl Pts',(-91.2578033288896,1.80769434990835,
136.327399602824));
#234590=CARTESIAN_POINT('Ctrl Pts',(-91.5362509527026,5.62379207040447,
132.268833643682));
#234591=CARTESIAN_POINT('Ctrl Pts',(-91.8146985765155,4.27189961571542,
126.864488517025));
#234592=CARTESIAN_POINT('Ctrl Pts',(-92.0931462003284,-1.00565989191805,
125.080693377311));
#234593=CARTESIAN_POINT('Ctrl Pts',(-92.3715938241412,-5.3590670880956,
128.556668814702));
#234594=CARTESIAN_POINT('Ctrl Pts',(-92.6500414479542,-4.78775343529548,
134.098163213075));
#234595=CARTESIAN_POINT('Ctrl Pts',(-92.928489071767,0.183271729783054,
136.612813937377));
#234596=CARTESIAN_POINT('Ctrl Pts',(-93.2069366955801,4.98587912851244,
133.789779819492));
#234597=CARTESIAN_POINT('Ctrl Pts',(-93.4853843193926,5.2067071818758,128.223291300872));
#234598=CARTESIAN_POINT('Ctrl Pts',(-93.7638319432059,0.642825696881324,
125.028679392048));
#234599=CARTESIAN_POINT('Ctrl Pts',(-94.0422795670186,-4.51178119976554,
127.14163637176));
#234600=CARTESIAN_POINT('Ctrl Pts',(-94.3207271908314,-5.52028158659305,
132.62045799934));
#234601=CARTESIAN_POINT('Ctrl Pts',(-94.5991748146444,-1.45591287608963,
136.430374854359));
#234602=CARTESIAN_POINT('Ctrl Pts',(-94.8776224384574,3.94636864224209,
135.07025947184));
#234603=CARTESIAN_POINT('Ctrl Pts',(-95.1560700622702,5.7221301691794,129.789991442987));
#234604=CARTESIAN_POINT('Ctrl Pts',(-95.4345176860831,2.23953361224044,
125.441879130882));
#234605=CARTESIAN_POINT('Ctrl Pts',(-95.7129653098959,-3.30108492704829,
126.021625333256));
#234606=CARTESIAN_POINT('Ctrl Pts',(-95.9914129337089,-5.80816768534362,
130.996471612301));
#234607=CARTESIAN_POINT('Ctrl Pts',(-96.2698605575217,-2.97782808557417,
135.794777272329));
#234608=CARTESIAN_POINT('Ctrl Pts',(-96.5483081813347,2.58899004984866,
136.007133822036));
#234609=CARTESIAN_POINT('Ctrl Pts',(-96.8267558051475,5.77665280865574,
131.438395966436));
#234610=CARTESIAN_POINT('Ctrl Pts',(-97.1052034289604,3.65585384148698,
126.287010599573));
#234611=CARTESIAN_POINT('Ctrl Pts',(-97.3836510527732,-1.82449620761995,
125.286849214428));
#234612=CARTESIAN_POINT('Ctrl Pts',(-97.6620986765863,-5.62822337351841,
129.35701126335));
#234613=CARTESIAN_POINT('Ctrl Pts',(-97.9405463003989,-4.25988821315111,
134.757216661848));
#234614=CARTESIAN_POINT('Ctrl Pts',(-98.2189939242121,1.02307610799351,
136.524940463405));
#234615=CARTESIAN_POINT('Ctrl Pts',(-98.4974415480248,5.36588346593846,
133.035730852497));
#234616=CARTESIAN_POINT('Ctrl Pts',(-98.7758891718378,4.77770605666655,
127.496001004183));
#234617=CARTESIAN_POINT('Ctrl Pts',(-99.0543367956506,-0.200949814765295,
124.996492018215));
#234618=CARTESIAN_POINT('Ctrl Pts',(-99.3327844194636,-4.99494262337204,
127.834130544897));
#234619=CARTESIAN_POINT('Ctrl Pts',(-99.6112320432764,-5.19882717761281,
133.401265404553));
#234620=CARTESIAN_POINT('Ctrl Pts',(-99.8896796670892,-0.625243532454567,
136.581971630822));
#234621=CARTESIAN_POINT('Ctrl Pts',(-100.168127290903,4.5229083741848,134.453335587896));
#234622=CARTESIAN_POINT('Ctrl Pts',(-100.446574914715,5.51472844130613,
128.971469809575));
#234623=CARTESIAN_POINT('Ctrl Pts',(-100.725022538528,1.43878248032906,
125.173941142103));
#234624=CARTESIAN_POINT('Ctrl Pts',(-101.003470162341,-3.95933429163924,
126.550492911299));
#234625=CARTESIAN_POINT('Ctrl Pts',(-101.281917786154,-5.71901627382367,
131.836141289563));
#234626=CARTESIAN_POINT('Ctrl Pts',(-101.560365409967,-2.22320168984167,
136.17363363555));
#234627=CARTESIAN_POINT('Ctrl Pts',(-101.83881303378,3.31562663766449,135.577026381578));
#234628=CARTESIAN_POINT('Ctrl Pts',(-102.117260657593,5.80755606252295,
130.594572448163));
#234629=CARTESIAN_POINT('Ctrl Pts',(-102.395708281405,2.96262518080941,
125.804903593708));
#234630=CARTESIAN_POINT('Ctrl Pts',(-102.674155905219,-2.60481350978186,
125.609491507123));
#234631=CARTESIAN_POINT('Ctrl Pts',(-102.952603529031,-5.77855583709781,
130.187910349571));
#234632=CARTESIAN_POINT('Ctrl Pts',(-103.231051152844,-3.64208764826766,
135.332816873036));
#234633=CARTESIAN_POINT('Ctrl Pts',(-103.509498776657,1.84128116344741,
136.316293325111));
#234634=CARTESIAN_POINT('Ctrl Pts',(-103.78794640047,5.63260253753978,132.234572891835));
#234635=CARTESIAN_POINT('Ctrl Pts',(-104.066394024283,4.24783734756473,
126.838557248259));
#234636=CARTESIAN_POINT('Ctrl Pts',(-104.344841648096,-1.04048284643121,
125.086921160811));
#234637=CARTESIAN_POINT('Ctrl Pts',(-104.623289271909,-5.3726501349701,
128.589332621676));
#234638=CARTESIAN_POINT('Ctrl Pts',(-104.901736895722,-4.76761441802147,
134.12724660063));
#234639=CARTESIAN_POINT('Ctrl Pts',(-105.180184519534,0.218626038175886,
136.611590693152));
#234640=CARTESIAN_POINT('Ctrl Pts',(-105.458632143348,5.00395984576562,
133.759374045173));
#234641=CARTESIAN_POINT('Ctrl Pts',(-105.73707976716,5.1908990121252,128.191644417652));
#234642=CARTESIAN_POINT('Ctrl Pts',(-106.015527390973,0.607655575856702,
125.024873339572));
#234643=CARTESIAN_POINT('Ctrl Pts',(-106.293975014786,-4.53399364899913,
127.169168726316));
#234644=CARTESIAN_POINT('Ctrl Pts',(-106.572422638599,-5.50912420832816,
132.654027872123));
#234645=CARTESIAN_POINT('Ctrl Pts',(-106.850870262412,-1.42163875588365,
136.43913317226));
#234646=CARTESIAN_POINT('Ctrl Pts',(-107.129317886225,3.97226326230387,
135.046157768576));
#234647=CARTESIAN_POINT('Ctrl Pts',(-107.407765510038,5.71584939828273,
129.755178006424));
#234648=CARTESIAN_POINT('Ctrl Pts',(-107.686213133851,2.20684917200607,
125.428345808491));
#234649=CARTESIAN_POINT('Ctrl Pts',(-107.964660757664,-3.3301376327682,
126.041808587174));
#234650=CARTESIAN_POINT('Ctrl Pts',(-108.243108381476,-5.80689063929651,
131.031824018185));
#234651=CARTESIAN_POINT('Ctrl Pts',(-108.521556005289,-2.94739483068967,
135.812811696231));
#234652=CARTESIAN_POINT('Ctrl Pts',(-108.800003629102,2.62061283907833,
135.991277509423));
#234653=CARTESIAN_POINT('Ctrl Pts',(-109.078451252915,5.7804053337882,131.403220093974));
#234654=CARTESIAN_POINT('Ctrl Pts',(-109.356898876728,3.62828771524594,
126.264840075618));
#234655=CARTESIAN_POINT('Ctrl Pts',(-109.635346500541,-1.85804906189805,
125.298057667405));
#234656=CARTESIAN_POINT('Ctrl Pts',(-109.913794124354,-5.636929521901,129.391298672536));
#234657=CARTESIAN_POINT('Ctrl Pts',(-110.192241748167,-4.2357471305931,
134.783074573235));
#234658=CARTESIAN_POINT('Ctrl Pts',(-110.470689371979,1.05787994597834,
136.518606719657));
#234659=CARTESIAN_POINT('Ctrl Pts',(-110.749136995792,5.37936703250445,
133.003025854698));
#234660=CARTESIAN_POINT('Ctrl Pts',(-111.027584619605,4.75747861284798,
127.466979047582));
#234661=CARTESIAN_POINT('Ctrl Pts',(-111.306032243418,-0.23630023626489,
124.997822863128));
#234662=CARTESIAN_POINT('Ctrl Pts',(-111.584479867231,-5.01293071215839,
127.864591209862));
#234663=CARTESIAN_POINT('Ctrl Pts',(-111.862927491044,-5.18292275885852,
133.432864026556));
#234664=CARTESIAN_POINT('Ctrl Pts',(-112.141375114857,-0.590061990020461,
136.585670619917));
#234665=CARTESIAN_POINT('Ctrl Pts',(-112.41982273867,4.54503692151536,134.425735753813));
#234666=CARTESIAN_POINT('Ctrl Pts',(-112.698270362483,5.50346893957634,
128.937934051507));
#234667=CARTESIAN_POINT('Ctrl Pts',(-112.976717986295,1.40448186157095,
125.165287183403));
#234668=CARTESIAN_POINT('Ctrl Pts',(-113.255165610108,-3.98515543446448,
126.574673317241));
#234669=CARTESIAN_POINT('Ctrl Pts',(-113.533613233921,-5.71262957189362,
131.870935448366));
#234670=CARTESIAN_POINT('Ctrl Pts',(-113.812060857734,-2.19047621022174,
136.187067415062));
#234671=CARTESIAN_POINT('Ctrl Pts',(-114.090508481547,3.34461777793161,
135.556754794705));
#234672=CARTESIAN_POINT('Ctrl Pts',(-114.36895610536,5.80617142182825,130.559224092919));
#234673=CARTESIAN_POINT('Ctrl Pts',(-114.647403729173,2.9321371763071,125.786961881698));
#234674=CARTESIAN_POINT('Ctrl Pts',(-114.925851352986,-2.63638789137572,
125.625443995184));
#234675=CARTESIAN_POINT('Ctrl Pts',(-115.204298976799,-5.78220128159277,
130.223097480497));
#234676=CARTESIAN_POINT('Ctrl Pts',(-115.482746600612,-3.61445417026275,
135.354903392492));
#234677=CARTESIAN_POINT('Ctrl Pts',(-115.761194224424,1.87479974763623,
136.304982800703));
#234678=CARTESIAN_POINT('Ctrl Pts',(-116.039641848237,5.64120428651674,
132.200259142944));
#234679=CARTESIAN_POINT('Ctrl Pts',(-116.31808947205,4.22361767423897,126.812772933795));
#234680=CARTESIAN_POINT('Ctrl Pts',(-116.596537095863,-1.07526724547036,
125.093360806132));
#234681=CARTESIAN_POINT('Ctrl Pts',(-116.874984719676,-5.38603409631742,
128.622078507325));
#234682=CARTESIAN_POINT('Ctrl Pts',(-117.153432343489,-4.7472987350426,
134.156206857421));
#234683=CARTESIAN_POINT('Ctrl Pts',(-117.431879967302,0.253972245300257,
136.610152259881));
#234684=CARTESIAN_POINT('Ctrl Pts',(-117.710327591115,5.02185513944583,
133.728858771743));
#234685=CARTESIAN_POINT('Ctrl Pts',(-117.988775214928,5.17489849170343,
128.160094349593));
#234686=CARTESIAN_POINT('Ctrl Pts',(-118.26722283874,0.572462937930709,
125.021281448121));
#234687=CARTESIAN_POINT('Ctrl Pts',(-118.545670462553,-4.55603808943068,
127.196835784245));
#234688=CARTESIAN_POINT('Ctrl Pts',(-118.824118086366,-5.49776268743969,
132.687529204804));
#234689=CARTESIAN_POINT('Ctrl Pts',(-119.102565710179,-1.38731195633035,
136.447682691592));
#234690=CARTESIAN_POINT('Ctrl Pts',(-119.381013333992,3.99801068868978,
135.021898883958));
#234691=CARTESIAN_POINT('Ctrl Pts',(-119.659460957805,5.70935682448427,
129.720403447709));
#234692=CARTESIAN_POINT('Ctrl Pts',(-119.937908581618,2.17408295616475,
125.415011696306));
#234693=CARTESIAN_POINT('Ctrl Pts',(-120.216356205431,-3.3590669390133,
126.062168319208));
#234694=CARTESIAN_POINT('Ctrl Pts',(-120.494803829244,-5.80539841678086,
131.067167995328));
#234695=CARTESIAN_POINT('Ctrl Pts',(-120.773251453056,-2.91685235900652,
135.830660530138));
#234696=CARTESIAN_POINT('Ctrl Pts',(-121.051699076869,2.65213852053535,
135.975228993696));
#234697=CARTESIAN_POINT('Ctrl Pts',(-121.330146700682,5.78394366387473,
131.368022030553));
#234698=CARTESIAN_POINT('Ctrl Pts',(-121.608594324495,3.60058714147007,
126.242837765265));
#234699=CARTESIAN_POINT('Ctrl Pts',(-121.887041948308,-1.89153306548558,
125.309470158462));
#234700=CARTESIAN_POINT('Ctrl Pts',(-122.165489572121,-5.64542679178685,
129.425638443252));
#234701=CARTESIAN_POINT('Ctrl Pts',(-122.443937195934,-4.21144909086733,
134.808785051914));
#234702=CARTESIAN_POINT('Ctrl Pts',(-122.722384819747,1.09264458383337,
136.512061232418));
#234703=CARTESIAN_POINT('Ctrl Pts',(-123.00083244356,5.39265126464657,132.97023938455));
#234704=CARTESIAN_POINT('Ctrl Pts',(-123.279280067372,4.73707487890982,
127.438080758883));
#234705=CARTESIAN_POINT('Ctrl Pts',(-123.557727691185,-0.27164190157181,
124.999368871432));
#234706=CARTESIAN_POINT('Ctrl Pts',(-123.836175314998,-5.03073304495359,
127.895160809065));
#234707=CARTESIAN_POINT('Ctrl Pts',(-124.114622938811,-5.16682628499523,
133.464365248398));
#234708=CARTESIAN_POINT('Ctrl Pts',(-124.393070562624,-0.554858582622917,
136.589155380447));
#234709=CARTESIAN_POINT('Ctrl Pts',(-124.671518186437,4.56699705083122,
134.398001728342));
#234710=CARTESIAN_POINT('Ctrl Pts',(-124.94996581025,5.49200550478084,128.904467454562));
#234711=CARTESIAN_POINT('Ctrl Pts',(-125.228413434063,1.37012919922165,
125.156842182641));
#234712=CARTESIAN_POINT('Ctrl Pts',(-125.506861057876,-4.0108289058903,
126.599010455801));
#234713=CARTESIAN_POINT('Ctrl Pts',(-125.785308681688,-5.70603118637341,
131.905690084846));
#234714=CARTESIAN_POINT('Ctrl Pts',(-126.063756305501,-2.1576695617001,
136.200301736396));
#234715=CARTESIAN_POINT('Ctrl Pts',(-126.342203929314,3.37348498215772,
135.536307106118));
#234716=CARTESIAN_POINT('Ctrl Pts',(-126.620651553127,5.8045716313158,130.523884821299));
#234717=CARTESIAN_POINT('Ctrl Pts',(-126.89909917694,2.90154052038371,125.769206091244));
#234718=CARTESIAN_POINT('Ctrl Pts',(-127.177546800753,-2.66786458064647,
125.641588389905));
#234719=CARTESIAN_POINT('Ctrl Pts',(-127.455994424566,-5.7856324644928,
130.258306150342));
#234720=CARTESIAN_POINT('Ctrl Pts',(-127.734442048379,-3.5866867573295,
135.376821289913));
#234721=CARTESIAN_POINT('Ctrl Pts',(-128.012889672192,1.90824886043053,
136.293468448719));
#234722=CARTESIAN_POINT('Ctrl Pts',(-128.291337296005,5.64959699859458,
132.16589366852));
#234723=CARTESIAN_POINT('Ctrl Pts',(-128.569784919818,4.19924149320669,
126.787136529081));
#234724=CARTESIAN_POINT('Ctrl Pts',(-128.84823254363,-1.11001180008614,
125.100012074652));
#234725=CARTESIAN_POINT('Ctrl Pts',(-129.126680167443,-5.39921847619124,
128.654905258242));
#234726=CARTESIAN_POINT('Ctrl Pts',(-129.405127791256,-4.72680713916258,
134.185042910317));
#234727=CARTESIAN_POINT('Ctrl Pts',(-129.683575415069,0.289309041389885,
136.608498690867));
#234728=CARTESIAN_POINT('Ctrl Pts',(-129.962023038882,5.03956434643776,
133.69823512996));
#234729=CARTESIAN_POINT('Ctrl Pts',(-130.240470662695,5.15870621351431,
128.128642265792));
#234730=CARTESIAN_POINT('Ctrl Pts',(-130.518918286508,0.537249087180579,
125.017903850796));
#234731=CARTESIAN_POINT('Ctrl Pts',(-130.79736591032,-4.57791370419536,
127.224636520332));
#234732=CARTESIAN_POINT('Ctrl Pts',(-131.075813534134,-5.4861974449331,
132.720960755981));
#234733=CARTESIAN_POINT('Ctrl Pts',(-131.354261157946,-1.35293374942274,
136.456023095549));
#234734=CARTESIAN_POINT('Ctrl Pts',(-131.632708781759,4.02360996731925,
134.99748371691));
#234735=CARTESIAN_POINT('Ctrl Pts',(-131.911156405572,5.7026526883694,129.685669055425));
#234736=CARTESIAN_POINT('Ctrl Pts',(-132.189604029385,2.1412361788793,125.401877288427));
#234737=CARTESIAN_POINT('Ctrl Pts',(-132.468051653198,-3.38787177379785,
126.082703774923));
#234738=CARTESIAN_POINT('Ctrl Pts',(-132.746499277011,-5.80369107309236,
131.102502234048));
#234739=CARTESIAN_POINT('Ctrl Pts',(-133.024946900823,-2.88620180228584,
135.848323112653));
#234740=CARTESIAN_POINT('Ctrl Pts',(-133.303394524637,2.68356592602436,
135.95898886954));
#234741=CARTESIAN_POINT('Ctrl Pts',(-133.581842148449,5.78726766780228,
131.332803080451));
#234742=CARTESIAN_POINT('Ctrl Pts',(-133.860289772262,3.57275314661281,
126.221004483821));
#234743=CARTESIAN_POINT('Ctrl Pts',(-134.138737396075,-1.92494697761906,
125.321086264707));
#234744=CARTESIAN_POINT('Ctrl Pts',(-134.417185019888,-5.65371486830715,
129.460029303025));
#234745=CARTESIAN_POINT('Ctrl Pts',(-134.695632643701,-4.1869949943469,
134.834347145171));
#234746=CARTESIAN_POINT('Ctrl Pts',(-134.974080267514,1.1273687333409,136.505304244234));
#234747=CARTESIAN_POINT('Ctrl Pts',(-135.252527891327,5.40573567011315,
132.937372656969));
#234748=CARTESIAN_POINT('Ctrl Pts',(-135.53097551514,4.71649561092,127.409307208922));
#234749=CARTESIAN_POINT('Ctrl Pts',(-135.809423138953,-0.306973501088704,
125.001129985841));
#234750=CARTESIAN_POINT('Ctrl Pts',(-136.087870762765,-5.04834896208586,
127.925838209736));
#234751=CARTESIAN_POINT('Ctrl Pts',(-136.366318386578,-5.15053835248403,
133.49576790279));
#234752=CARTESIAN_POINT('Ctrl Pts',(-136.644766010391,-0.519634614735935,
136.592425783278));
#234753=CARTESIAN_POINT('Ctrl Pts',(-136.923213634204,4.58878794839197,
134.37013453918));
#234754=CARTESIAN_POINT('Ctrl Pts',(-137.201661258017,5.48033856170195,
128.871071258858));
#234755=CARTESIAN_POINT('Ctrl Pts',(-137.48010888183,1.33572576623031,125.148606452753));
#234756=CARTESIAN_POINT('Ctrl Pts',(-137.758556505643,-4.03635375457527,
126.623503425159));
#234757=CARTESIAN_POINT('Ctrl Pts',(-138.037004129456,-5.69922136176977,
131.940403911158));
#234758=CARTESIAN_POINT('Ctrl Pts',(-138.315451753269,-2.12478295993955,
136.213336109146));
#234759=CARTESIAN_POINT('Ctrl Pts',(-138.593899377082,3.40222718065648,
135.515684073514));
#234760=CARTESIAN_POINT('Ctrl Pts',(-138.872347000894,5.80275675026745,
130.488555942812));
#234761=CARTESIAN_POINT('Ctrl Pts',(-139.150794624707,2.870836346809,125.751636880291));
#234762=CARTESIAN_POINT('Ctrl Pts',(-139.42924224852,-2.69924241121433,
125.65792409305));
#234763=CARTESIAN_POINT('Ctrl Pts',(-139.707689872333,-5.78884925865424,
130.293535054436));
#234764=CARTESIAN_POINT('Ctrl Pts',(-139.986137496146,-3.55878643839929,
135.398569753122));
#234765=CARTESIAN_POINT('Ctrl Pts',(-140.264585119959,1.94162726236197,
136.281750695826));
#234766=CARTESIAN_POINT('Ctrl Pts',(-140.543032743772,5.65778036277742,
132.131477741989));
#234767=CARTESIAN_POINT('Ctrl Pts',(-140.821480367585,4.17470970773734,
126.761648984083));
#234768=CARTESIAN_POINT('Ctrl Pts',(-141.099927991397,-1.14471522280625,
125.106874719905));
#234769=CARTESIAN_POINT('Ctrl Pts',(-141.37837561521,-5.41220278603824,
128.687811658017));
#234770=CARTESIAN_POINT('Ctrl Pts',(-141.656823239023,-4.70614038970644,
134.213753690789));
#234771=CARTESIAN_POINT('Ctrl Pts',(-141.935270862836,0.324635117026387,
136.60663004738));
#234772=CARTESIAN_POINT('Ctrl Pts',(-142.213718486649,5.05708681051884,
133.667504254592));
#234773=CARTESIAN_POINT('Ctrl Pts',(-142.492166110462,5.14232277757003,
128.097289331719));
#234774=CARTESIAN_POINT('Ctrl Pts',(-142.770613734275,0.502015328467386,
125.014740672754));
#234775=CARTESIAN_POINT('Ctrl Pts',(-143.049061358088,-4.59961968268416,
127.252569904414));
#234776=CARTESIAN_POINT('Ctrl Pts',(-143.327508981901,-5.4744289093626,
132.754321286837));
#234777=CARTESIAN_POINT('Ctrl Pts',(-143.605956605714,-1.31850540905707,
136.464154075075));
#234778=CARTESIAN_POINT('Ctrl Pts',(-143.884404229526,4.04906014960179,
134.972913172143));
#234779=CARTESIAN_POINT('Ctrl Pts',(-144.162851853339,5.69573723836169,
129.650976116669));
#234780=CARTESIAN_POINT('Ctrl Pts',(-144.441299477152,2.10831005730047,
125.388943071553));
#234781=CARTESIAN_POINT('Ctrl Pts',(-144.719747100965,-3.41655106974776,
126.103414193369));
#234782=CARTESIAN_POINT('Ctrl Pts',(-144.998194724778,-5.80176867149642,
131.13782542502));
#234783=CARTESIAN_POINT('Ctrl Pts',(-145.276642348591,-2.85544429629671,
135.865798789283));
#234784=CARTESIAN_POINT('Ctrl Pts',(-145.555089972404,2.71489389099137,
135.942557738738));
#234785=CARTESIAN_POINT('Ctrl Pts',(-145.833537596217,5.79037722239768,
131.29756454872));
#234786=CARTESIAN_POINT('Ctrl Pts',(-146.111985220029,3.54478676207412,
126.199341040322));
#234787=CARTESIAN_POINT('Ctrl Pts',(-146.390432843843,-1.95828956013508,
125.332905555698));
#234788=CARTESIAN_POINT('Ctrl Pts',(-146.668880467655,-5.66179344434354,
129.49446997749));
#234789=CARTESIAN_POINT('Ctrl Pts',(-146.947328091469,-4.16238574718705,
134.859759905796));
#234790=CARTESIAN_POINT('Ctrl Pts',(-147.225775715281,1.16205110778606,
136.498336005488));
#234791=CARTESIAN_POINT('Ctrl Pts',(-147.504223339094,5.41861976405632,
132.904426889841));
#234792=CARTESIAN_POINT('Ctrl Pts',(-147.782670962907,4.6957415714508,127.380659463914));
#234793=CARTESIAN_POINT('Ctrl Pts',(-148.06111858672,-0.342293725589094,
125.003106141093));
#234794=CARTESIAN_POINT('Ctrl Pts',(-148.339566210533,-5.06577781079073,
127.956622275114));
#234795=CARTESIAN_POINT('Ctrl Pts',(-148.618013834346,-5.1340595648799,
133.527070826096));
#234796=CARTESIAN_POINT('Ctrl Pts',(-148.896461458158,-0.48439139159784,
136.595481707227));
#234797=CARTESIAN_POINT('Ctrl Pts',(-149.174909081971,4.61040880672808,
134.342135218952));
#234798=CARTESIAN_POINT('Ctrl Pts',(-149.453356705784,5.4684685426618,128.837746701901));
#234799=CARTESIAN_POINT('Ctrl Pts',(-149.731804329597,1.30127283742975,
125.140580298914));
#234800=CARTESIAN_POINT('Ctrl Pts',(-150.01025195341,-4.06172903468827,
126.648151317718));
#234801=CARTESIAN_POINT('Ctrl Pts',(-150.288699577223,-5.69220035042211,
131.975075640969));
#234802=CARTESIAN_POINT('Ctrl Pts',(-150.567147201036,-2.09181762356486,
136.226170050321));
#234803=CARTESIAN_POINT('Ctrl Pts',(-150.845594824849,3.43084330837664,
135.494886461086));
#234804=CARTESIAN_POINT('Ctrl Pts',(-151.124042448661,5.80072684593324,
130.453238766583));
#234805=CARTESIAN_POINT('Ctrl Pts',(-151.402490072475,2.84002579333802,
125.734254899877));
#234806=CARTESIAN_POINT('Ctrl Pts',(-151.680937696287,-2.73052022036177,
125.674450499292));
#234807=CARTESIAN_POINT('Ctrl Pts',(-151.9593853201,-5.79185154487752,130.32878288736));
#234808=CARTESIAN_POINT('Ctrl Pts',(-152.237832943913,-3.53075424732904,
135.420147976222));
#234809=CARTESIAN_POINT('Ctrl Pts',(-152.516280567726,1.97493371658077,
136.269829976228));
#234810=CARTESIAN_POINT('Ctrl Pts',(-152.794728191539,5.66575407582884,
132.097012638644));
#234811=CARTESIAN_POINT('Ctrl Pts',(-153.073175815352,4.15002322686382,
126.736311243251));
#234812=CARTESIAN_POINT('Ctrl Pts',(-153.351623439165,-1.17937622768304,
125.113948487592));
#234813=CARTESIAN_POINT('Ctrl Pts',(-153.630071062978,-5.42498654472129,
128.720796487292));
#234814=CARTESIAN_POINT('Ctrl Pts',(-153.90851868679,-4.6852992524868,134.242338134946));
#234815=CARTESIAN_POINT('Ctrl Pts',(-154.186966310604,0.359949163189457,
136.604546398667));
#234816=CARTESIAN_POINT('Ctrl Pts',(-154.465413934416,5.0744218823891,133.636667284384));
#234817=CARTESIAN_POINT('Ctrl Pts',(-154.743861558229,5.12574879096345,
128.066036709167));
#234818=CARTESIAN_POINT('Ctrl Pts',(-155.022309182042,0.466762967392146,
125.011792031209));
#234819=CARTESIAN_POINT('Ctrl Pts',(-155.300756805855,-4.62115522057418,
127.280634901405));
#234820=CARTESIAN_POINT('Ctrl Pts',(-155.579204429668,-5.46245751681569,
132.787609561181));
#234821=CARTESIAN_POINT('Ctrl Pts',(-155.857652053481,-1.28402821098903,
136.472075328871));
#234822=CARTESIAN_POINT('Ctrl Pts',(-156.136099677293,4.07436029247137,
134.948188160129));
#234823=CARTESIAN_POINT('Ctrl Pts',(-156.414547301107,5.68861073071636,
129.616325916999));
#234824=CARTESIAN_POINT('Ctrl Pts',(-156.692994924919,2.07530581151645,
125.376209524969));
#234825=CARTESIAN_POINT('Ctrl Pts',(-156.971442548732,-3.44510376414151,
126.124298807112));
#234826=CARTESIAN_POINT('Ctrl Pts',(-157.249890172545,-5.79963128322921,
131.173136259331));
#234827=CARTESIAN_POINT('Ctrl Pts',(-157.528337796358,-2.82458098076833,
135.883086912459));
#234828=CARTESIAN_POINT('Ctrl Pts',(-157.806785420171,2.74612125456611,
135.925936210153));
#234829=CARTESIAN_POINT('Ctrl Pts',(-158.085233043984,5.79327221243612,
131.262307741136));
#234830=CARTESIAN_POINT('Ctrl Pts',(-158.363680667797,3.51668902415852,
126.177848237519));
#234831=CARTESIAN_POINT('Ctrl Pts',(-158.64212829161,-1.9915595775106,125.344927593469));
#234832=CARTESIAN_POINT('Ctrl Pts',(-158.920575915422,-5.66966222054205,
129.528959190434));
#234833=CARTESIAN_POINT('Ctrl Pts',(-159.199023539236,-4.13762226129274,
134.885022392109));
#234834=CARTESIAN_POINT('Ctrl Pts',(-159.477471163048,1.19669042199943,
136.491156774389));
#234835=CARTESIAN_POINT('Ctrl Pts',(-159.755918786861,5.43130306905165,
132.871403303985));
#234836=CARTESIAN_POINT('Ctrl Pts',(-160.034366410674,4.67481352955083,
127.352138585409));
#234837=CARTESIAN_POINT('Ctrl Pts',(-160.312814034487,-0.377601266270116,
125.005297263965));
#234838=CARTESIAN_POINT('Ctrl Pts',(-160.5912616583,-5.08301894523598,127.987511864483));
#234839=CARTESIAN_POINT('Ctrl Pts',(-160.869709282113,-5.1173905328107,
133.558272858373));
#234840=CARTESIAN_POINT('Ctrl Pts',(-161.148156905926,-0.449130219157962,
136.598323039052));
#234841=CARTESIAN_POINT('Ctrl Pts',(-161.426604529739,4.63185882466967,
134.314004805186));
#234842=CARTESIAN_POINT('Ctrl Pts',(-161.705052153551,5.45639588750942,
128.804495018547));
#234843=CARTESIAN_POINT('Ctrl Pts',(-161.983499777364,1.26677168948586,
125.13276401854));
#234844=CARTESIAN_POINT('Ctrl Pts',(-162.261947401177,-4.08695380593746,
126.67295322014));
#234845=CARTESIAN_POINT('Ctrl Pts',(-162.54039502499,-5.68496841249774,
132.009703989503));
#234846=CARTESIAN_POINT('Ctrl Pts',(-162.818842648803,-2.05877477411906,
136.238803084352));
#234847=CARTESIAN_POINT('Ctrl Pts',(-163.097290272616,3.45933230493559,
135.473915039499));
#234848=CARTESIAN_POINT('Ctrl Pts',(-163.375737896429,5.79848199353304,
130.417934601304));
#234849=CARTESIAN_POINT('Ctrl Pts',(-163.654185520242,2.80911000166655,
125.717060794092));
#234850=CARTESIAN_POINT('Ctrl Pts',(-163.932633144055,-2.76169684907854,
125.691166996241));
#234851=CARTESIAN_POINT('Ctrl Pts',(-164.211080767867,-5.79463921191188,
130.36404834299));
#234852=CARTESIAN_POINT('Ctrl Pts',(-164.489528391681,-3.50259122286156,
135.441555159625));
#234853=CARTESIAN_POINT('Ctrl Pts',(-164.767976015493,2.00816698890481,
136.257706731653));
#234854=CARTESIAN_POINT('Ctrl Pts',(-165.046423639306,5.67351784227885,
132.062499635604));
#234855=CARTESIAN_POINT('Ctrl Pts',(-165.324871263119,4.12518296535417,
126.711124245485));
#234856=CARTESIAN_POINT('Ctrl Pts',(-165.603318886932,-1.21399353033979,
125.121233115594));
#234857=CARTESIAN_POINT('Ctrl Pts',(-165.881766510745,-5.43756927853226,
128.753858523801));
#234858=CARTESIAN_POINT('Ctrl Pts',(-166.160214134558,-4.66428449978105,
134.270795183582));
#234859=CARTESIAN_POINT('Ctrl Pts',(-166.438661758371,0.395249871304121,
136.602247821935));
#234860=CARTESIAN_POINT('Ctrl Pts',(-166.717109382183,5.09156891968999,
133.60572536201));
#234861=CARTESIAN_POINT('Ctrl Pts',(-166.995557005996,5.10898486785074,
128.034885556215));
#234862=CARTESIAN_POINT('Ctrl Pts',(-167.274004629809,0.431493310242956,
125.009058035423));
#234863=CARTESIAN_POINT('Ctrl Pts',(-167.552452253622,-4.64251951985801,
127.30883047135));
#234864=CARTESIAN_POINT('Ctrl Pts',(-167.830899877435,-5.45028371089662,
132.820824345507));
#234865=CARTESIAN_POINT('Ctrl Pts',(-168.109347501248,-1.24950343278299,
136.479786563416));
#234866=CARTESIAN_POINT('Ctrl Pts',(-168.387795125061,4.09950945842204,
134.923309597059));
#234867=CARTESIAN_POINT('Ctrl Pts',(-168.666242748874,5.68127342950807,
129.581719740392));
#234868=CARTESIAN_POINT('Ctrl Pts',(-168.944690372687,2.04222466451309,
125.36367712052));
#234869=CARTESIAN_POINT('Ctrl Pts',(-169.223137996499,-3.47352879894819,
126.145356842267));
#234870=CARTESIAN_POINT('Ctrl Pts',(-169.501585620313,-5.79727898749155,
131.208433428525));
#234871=CARTESIAN_POINT('Ctrl Pts',(-169.780033244125,-2.79361299935373,
135.900186841566));
#234872=CARTESIAN_POINT('Ctrl Pts',(-170.058480867939,2.77724685960862,
135.909124899701));
#234873=CARTESIAN_POINT('Ctrl Pts',(-170.336928491751,5.79595253064181,
131.227033964152));
#234874=CARTESIAN_POINT('Ctrl Pts',(-170.615376115564,3.48846097403773,
126.156526871832));
#234875=CARTESIAN_POINT('Ctrl Pts',(-170.893823739377,-2.02475579691427,
125.357151932539));
#234876=CARTESIAN_POINT('Ctrl Pts',(-171.17227136319,-5.67732090532164,
129.563495663847));
#234877=CARTESIAN_POINT('Ctrl Pts',(-171.450718987003,-4.11270545428381,
134.910133667999));
#234878=CARTESIAN_POINT('Ctrl Pts',(-171.729166610815,1.23128539240979,
136.483766816968));
#234879=CARTESIAN_POINT('Ctrl Pts',(-172.007614234629,5.44378511511418,
132.838303123102));
#234880=CARTESIAN_POINT('Ctrl Pts',(-172.286061858441,4.65371226071637,
127.323745630264));
#234881=CARTESIAN_POINT('Ctrl Pts',(-172.564509482254,-0.412894814796852,
125.00770327326));
#234882=CARTESIAN_POINT('Ctrl Pts',(-172.842957106067,-5.10007172654484,
128.018505833219));
#234883=CARTESIAN_POINT('Ctrl Pts',(-173.12140472988,-5.10053187395325,
133.589372843419));
#234884=CARTESIAN_POINT('Ctrl Pts',(-173.399852353693,-0.413852404033268,
136.600949673471));
#234885=CARTESIAN_POINT('Ctrl Pts',(-173.678299977506,4.65313720737985,
134.285744340263));
#234886=CARTESIAN_POINT('Ctrl Pts',(-173.956747601319,5.44412104360021,
128.771317440947));
#234887=CARTESIAN_POINT('Ctrl Pts',(-174.235195225131,1.23222360085094,
125.125157901261));
#234888=CARTESIAN_POINT('Ctrl Pts',(-174.513642848945,-4.11202713361109,
126.697908213384));
#234889=CARTESIAN_POINT('Ctrl Pts',(-174.792090472757,-5.67752581597763,
132.044287673595));
#234890=CARTESIAN_POINT('Ctrl Pts',(-175.070538096571,-2.02565563601667,
136.251234743121));
#234891=CARTESIAN_POINT('Ctrl Pts',(-175.348985720383,3.48769311466452,
135.452770585855));
#234892=CARTESIAN_POINT('Ctrl Pts',(-175.627433344196,5.79602227624969,
130.382644755183));
#234893=CARTESIAN_POINT('Ctrl Pts',(-175.905880968009,2.77809011739122,
125.700055200075));
#234894=CARTESIAN_POINT('Ctrl Pts',(-176.184328591822,-2.79277114210269,
125.708072964459));
#234895=CARTESIAN_POINT('Ctrl Pts',(-176.462776215635,-5.79721215645926,
130.399330114555));
#234896=CARTESIAN_POINT('Ctrl Pts',(-176.741223839448,-3.47429840858841,
135.462790510077));
#234897=CARTESIAN_POINT('Ctrl Pts',(-177.019671463261,2.04132584786218,
136.245381411334));
#234898=CARTESIAN_POINT('Ctrl Pts',(-177.298119087073,5.68107137443935,
132.02794001176));
#234899=CARTESIAN_POINT('Ctrl Pts',(-177.576566710886,4.10018984367198,
126.686088924097));
#234900=CARTESIAN_POINT('Ctrl Pts',(-177.855014334699,-1.24856584802001,
125.128728333976));
#234901=CARTESIAN_POINT('Ctrl Pts',(-178.133461958512,-5.4499505212146,
128.786996542421));
#234902=CARTESIAN_POINT('Ctrl Pts',(-178.411909582325,-4.64309691029714,
134.29912378221));
#234903=CARTESIAN_POINT('Ctrl Pts',(-178.690357206138,0.430535933288815,
136.599734402363));
#234904=CARTESIAN_POINT('Ctrl Pts',(-178.968804829951,5.10852728703229,
133.574679634036));
#234905=CARTESIAN_POINT('Ctrl Pts',(-179.247252453763,5.09203162942501,
128.00383702718));
#234906=CARTESIAN_POINT('Ctrl Pts',(-179.525700077576,0.396207663951002,
125.006538786706));
#234907=CARTESIAN_POINT('Ctrl Pts',(-179.80414770139,-4.66371178887382,
127.337155569449));
#234908=CARTESIAN_POINT('Ctrl Pts',(-180.082595325202,-5.43790794271038,
132.853964409027));
#234909=CARTESIAN_POINT('Ctrl Pts',(-180.361042949015,-1.2149323537682,
136.487287492965));
#234910=CARTESIAN_POINT('Ctrl Pts',(-180.639490572828,4.12450671554208,
134.898278404822));
#234911=CARTESIAN_POINT('Ctrl Pts',(-180.917938196641,5.67372560662389,
129.547158869193));
#234912=CARTESIAN_POINT('Ctrl Pts',(-181.196385820454,2.00906784212309,
125.351346322599));
#234913=CARTESIAN_POINT('Ctrl Pts',(-181.474833444267,-3.50182512086801,
126.166587518521));
#234914=CARTESIAN_POINT('Ctrl Pts',(-181.75328106808,-5.79471187144949,
131.243715624654));
#234915=CARTESIAN_POINT('Ctrl Pts',(-182.031728691892,-2.76254149958135,
135.917097942958));
#234916=CARTESIAN_POINT('Ctrl Pts',(-182.310176315705,2.80826955274668,
135.892124430331));
#234917=CARTESIAN_POINT('Ctrl Pts',(-182.588623939518,5.79841807769547,
131.191744524852));
#234918=CARTESIAN_POINT('Ctrl Pts',(-182.867071563331,3.46010365771282,
126.135377733334));
#234919=CARTESIAN_POINT('Ctrl Pts',(-183.145519187144,-2.05787698824661,
125.369578119929));
#234920=CARTESIAN_POINT('Ctrl Pts',(-183.423966810957,-5.68476921488759,
129.598078117967));
#234921=CARTESIAN_POINT('Ctrl Pts',(-183.70241443477,-4.08763624946197,
134.93509280296));
#234922=CARTESIAN_POINT('Ctrl Pts',(-183.980862058583,1.26583473708647,
136.476166407061));
#234923=CARTESIAN_POINT('Ctrl Pts',(-184.259309682396,5.45606543971754,
132.805127573733));
#234924=CARTESIAN_POINT('Ctrl Pts',(-184.537757306209,4.63243854686269,
127.295481650585));
#234925=CARTESIAN_POINT('Ctrl Pts',(-184.816204930021,-0.448173063354899,
125.010324079826));
#234926=CARTESIAN_POINT('Ctrl Pts',(-185.094652553834,-5.11693552282041,
128.049603032828));
#234927=CARTESIAN_POINT('Ctrl Pts',(-185.373100177647,-5.08348421301165,
133.620369628814));
#234928=CARTESIAN_POINT('Ctrl Pts',(-185.65154780146,-0.378559253454916,
136.60336151315));
#234929=CARTESIAN_POINT('Ctrl Pts',(-185.929995425273,4.67424316637891,
134.257354871388));
#234930=CARTESIAN_POINT('Ctrl Pts',(-186.208443049086,5.4316444657843,128.73821519851));
#234931=CARTESIAN_POINT('Ctrl Pts',(-186.486890672899,1.19762985171755,
125.117762228929));
#234932=CARTESIAN_POINT('Ctrl Pts',(-186.765338296712,-4.13694808860639,
126.72301537273));
#234933=CARTESIAN_POINT('Ctrl Pts',(-187.043785920525,-5.66987283665109,
132.078825411735));
#234934=CARTESIAN_POINT('Ctrl Pts',(-187.322233544337,-1.99246143649967,
136.263464565965));
#234935=CARTESIAN_POINT('Ctrl Pts',(-187.600681168151,3.51592468664221,
135.43145388367));
#234936=CARTESIAN_POINT('Ctrl Pts',(-187.879128791963,5.79334778522967,
130.347370535898));
#234937=CARTESIAN_POINT('Ctrl Pts',(-188.157576415776,2.74696728996466,
125.683238747971));
#234938=CARTESIAN_POINT('Ctrl Pts',(-188.436024039589,-2.82374194796541,
125.72516777749));
#234939=CARTESIAN_POINT('Ctrl Pts',(-188.714471663402,-5.79957028317828,
130.434626894674));
#234940=CARTESIAN_POINT('Ctrl Pts',(-188.992919287215,-3.44587685290989,
135.483853240698));
#234941=CARTESIAN_POINT('Ctrl Pts',(-189.271366911028,2.07440906473995,
136.232854471987));
#234942=CARTESIAN_POINT('Ctrl Pts',(-189.54981453484,5.68841439241029,131.993335047731));
#234943=CARTESIAN_POINT('Ctrl Pts',(-189.828262158654,4.07504478794802,
126.661206206783));
#234944=CARTESIAN_POINT('Ctrl Pts',(-190.106709782466,-1.28309189963338,
125.136433864998));
#234945=CARTESIAN_POINT('Ctrl Pts',(-190.385157406279,-5.46212981397553,
128.820209315208));
#234946=CARTESIAN_POINT('Ctrl Pts',(-190.663605030092,-4.62173726915045,
134.327322881104));
#234947=CARTESIAN_POINT('Ctrl Pts',(-190.942052653905,0.465806041606811,
136.597006233083));
#234948=CARTESIAN_POINT('Ctrl Pts',(-191.220500277718,5.12529635601715,
133.543531250871));
#234949=CARTESIAN_POINT('Ctrl Pts',(-191.49894790153,5.07488970389458,127.972892272577));
#234950=CARTESIAN_POINT('Ctrl Pts',(-191.777395525344,0.360907336037817,
125.004234378408));
#234951=CARTESIAN_POINT('Ctrl Pts',(-192.055843149156,-4.68473124233415,
127.365609146106));
#234952=CARTESIAN_POINT('Ctrl Pts',(-192.33429077297,-5.42533067084548,
132.887028523726));
#234953=CARTESIAN_POINT('Ctrl Pts',(-192.612738396782,-1.1803162549878,
136.494577839569));
#234954=CARTESIAN_POINT('Ctrl Pts',(-192.891186020595,4.14935113754904,
134.873095510955));
#234955=CARTESIAN_POINT('Ctrl Pts',(-193.169633644408,5.66596754175055,
129.512644584067));
#234956=CARTESIAN_POINT('Ctrl Pts',(-193.448081268221,1.97583657298603,
125.339217588127));
#234957=CARTESIAN_POINT('Ctrl Pts',(-193.726528892034,-3.52999168137001,
126.187990049162));
#234958=CARTESIAN_POINT('Ctrl Pts',(-194.004976515847,-5.79193003022761,
131.27898154032));
#234959=CARTESIAN_POINT('Ctrl Pts',(-194.28342413966,-2.73136763281852,
135.933819589987));
#234960=CARTESIAN_POINT('Ctrl Pts',(-194.561871763472,2.83918818442447,
135.874935432001));
#234961=CARTESIAN_POINT('Ctrl Pts',(-194.840319387286,5.80066876223446,
131.156440730899));
#234962=CARTESIAN_POINT('Ctrl Pts',(-195.118767011098,3.43161812597426,
126.114401605713));
#234963=CARTESIAN_POINT('Ctrl Pts',(-195.397214634911,-2.09092192419104,
125.382205695184));
#234964=CARTESIAN_POINT('Ctrl Pts',(-195.675662258724,-5.69200687323938,
129.63270527133));
#234965=CARTESIAN_POINT('Ctrl Pts',(-195.954109882537,-4.06241557577554,
134.95989887212));
#234966=CARTESIAN_POINT('Ctrl Pts',(-196.23255750635,1.30033717579212,136.468355826305));
#234967=CARTESIAN_POINT('Ctrl Pts',(-196.511005130163,5.46814358780935,
132.771877885207));
#234968=CARTESIAN_POINT('Ctrl Pts',(-196.789452753976,4.61099317629508,
127.267347693709));
#234969=CARTESIAN_POINT('Ctrl Pts',(-197.067900377789,-0.483434704694746,
125.013159586548));
#234970=CARTESIAN_POINT('Ctrl Pts',(-197.346348001602,-5.13360970916836,
128.080802310993));
#234971=CARTESIAN_POINT('Ctrl Pts',(-197.624795625414,-5.06624818169292,
133.651262065958));
#234972=CARTESIAN_POINT('Ctrl Pts',(-197.903243249227,-0.343252075224855,
136.605558468718));
#234973=CARTESIAN_POINT('Ctrl Pts',(-198.18169087304,4.69517591957924,134.228837450539));
#234974=CARTESIAN_POINT('Ctrl Pts',(-198.460138496853,5.41896661638458,
128.705189517851));
#234975=CARTESIAN_POINT('Ctrl Pts',(-198.738586120666,1.1629917239694,125.110577275591));
#234976=CARTESIAN_POINT('Ctrl Pts',(-199.017033744479,-4.16171574746965,
126.748273767825));
#234977=CARTESIAN_POINT('Ctrl Pts',(-199.295481368292,-5.6620097581009,
132.113315924113));
#234978=CARTESIAN_POINT('Ctrl Pts',(-199.573928992105,-1.95919340559182,
136.275492099704));
#234979=CARTESIAN_POINT('Ctrl Pts',(-199.852376615917,3.54402597473752,
135.409965722843));
#234980=CARTESIAN_POINT('Ctrl Pts',(-200.13082423973,5.79045861957696,130.312113250549));
#234981=CARTESIAN_POINT('Ctrl Pts',(-200.409271863544,2.71574267265526,
125.666612060922));
#234982=CARTESIAN_POINT('Ctrl Pts',(-200.687719487356,-2.85460811903155,
125.742450801881));
#234983=CARTESIAN_POINT('Ctrl Pts',(-200.966167111169,-5.80171350468764,
130.469937375411));
#234984=CARTESIAN_POINT('Ctrl Pts',(-201.244614734982,-3.41732760899753,
135.504742570997));
#234985=CARTESIAN_POINT('Ctrl Pts',(-201.523062358795,2.10741541362659,
136.220126377805));
#234986=CARTESIAN_POINT('Ctrl Pts',(-201.801509982608,5.69554662409457,
131.958686025817));
#234987=CARTESIAN_POINT('Ctrl Pts',(-202.079957606421,4.04974872994014,
126.636477015578));
#234988=CARTESIAN_POINT('Ctrl Pts',(-202.358405230234,-1.31757040580477,
125.144349423131));
#234989=CARTESIAN_POINT('Ctrl Pts',(-202.636852854047,-5.47410670550813,
128.853495611451));
#234990=CARTESIAN_POINT('Ctrl Pts',(-202.915300477859,-4.6002063678289,
134.355391435336));
#234991=CARTESIAN_POINT('Ctrl Pts',(-203.193748101672,0.501058889310003,
136.594063415189));
#234992=CARTESIAN_POINT('Ctrl Pts',(-203.472195725485,5.14187550526088,
133.512281366733));
#234993=CARTESIAN_POINT('Ctrl Pts',(-203.750643349298,5.05755972645996,
127.942052439074));
#234994=CARTESIAN_POINT('Ctrl Pts',(-204.029090973111,0.325593634571106,
125.002144895921));
#234995=CARTESIAN_POINT('Ctrl Pts',(-204.307538596924,-4.70557710135553,
127.394190146963));
#234996=CARTESIAN_POINT('Ctrl Pts',(-204.585986220737,-5.41255236135747,
132.920015464399));
#234997=CARTESIAN_POINT('Ctrl Pts',(-204.864433844549,-1.14565641915494,
136.50165733308));
#234998=CARTESIAN_POINT('Ctrl Pts',(-205.142881468362,4.17404180382362,
134.847761848621));
#234999=CARTESIAN_POINT('Ctrl Pts',(-205.421329092175,5.6579995223666,129.478178163952));
#235000=CARTESIAN_POINT('Ctrl Pts',(-205.699776715988,1.94253208849746,
125.327291366541));
#235001=CARTESIAN_POINT('Ctrl Pts',(-205.978224339801,-3.55802743673226,
126.209563641112));
#235002=CARTESIAN_POINT('Ctrl Pts',(-206.256671963614,-5.78893356690891,
131.314229868733));
#235003=CARTESIAN_POINT('Ctrl Pts',(-206.535119587427,-2.70009255422283,
135.950351163029));
#235004=CARTESIAN_POINT('Ctrl Pts',(-206.81356721124,2.87000160893922,135.857558541658));
#235005=CARTESIAN_POINT('Ctrl Pts',(-207.092014835053,5.80270450085972,
131.121123890489));
#235006=CARTESIAN_POINT('Ctrl Pts',(-207.370462458865,3.40300543436423,
126.09359926625));
#235007=CARTESIAN_POINT('Ctrl Pts',(-207.648910082679,-2.12388938025395,
125.395034190384));
#235008=CARTESIAN_POINT('Ctrl Pts',(-207.927357706491,-5.69903361218359,
129.667375840811));
#235009=CARTESIAN_POINT('Ctrl Pts',(-208.205805330304,-4.03704436778601,
134.984550956282));
#235010=CARTESIAN_POINT('Ctrl Pts',(-208.484252954117,1.33479143002538,
136.460335364123));
#235011=CARTESIAN_POINT('Ctrl Pts',(-208.76270057793,5.48001911182977,132.738555289606));
#235012=CARTESIAN_POINT('Ctrl Pts',(-209.041148201743,4.58937694367963,
127.239344802146));
#235013=CARTESIAN_POINT('Ctrl Pts',(-209.319595825556,-0.518678432184342,
125.016209688352));
#235014=CARTESIAN_POINT('Ctrl Pts',(-209.598043449369,-5.15009366772074,
128.112102511612));
#235015=CARTESIAN_POINT('Ctrl Pts',(-209.876491073182,-5.04882441868487,
133.682049010123));
#235016=CARTESIAN_POINT('Ctrl Pts',(-210.154938696994,-0.307932177662294,
136.607540458767));
#235017=CARTESIAN_POINT('Ctrl Pts',(-210.433386320807,4.71593469130848,
134.200193134443));
#235018=CARTESIAN_POINT('Ctrl Pts',(-210.71183394462,5.40608796518471,128.672241622749));
#235019=CARTESIAN_POINT('Ctrl Pts',(-210.990281568433,1.12831050113542,
125.103603307488));
#235020=CARTESIAN_POINT('Ctrl Pts',(-211.268729192246,-4.18632919242468,
126.773682462711));
#235021=CARTESIAN_POINT('Ctrl Pts',(-211.547176816059,-5.65393687169752,
132.14775793267));
#235022=CARTESIAN_POINT('Ctrl Pts',(-211.825624439872,-1.92585277605142,
136.287316898656));
#235023=CARTESIAN_POINT('Ctrl Pts',(-212.104072063685,3.57199593764717,
135.388306899624));
#235024=CARTESIAN_POINT('Ctrl Pts',(-212.382519687498,5.78735488635066,
130.276874205606));
#235025=CARTESIAN_POINT('Ctrl Pts',(-212.660967311311,2.68441742250212,
125.650175755035));
#235026=CARTESIAN_POINT('Ctrl Pts',(-212.939414935123,-2.88536851154432,
125.759921397201));
#235027=CARTESIAN_POINT('Ctrl Pts',(-213.217862558936,-5.80364174156953,
130.505260248325));
#235028=CARTESIAN_POINT('Ctrl Pts',(-213.496310182749,-3.38865173475374,
135.525457726916));
#235029=CARTESIAN_POINT('Ctrl Pts',(-213.774757806562,2.14034367146046,
136.20719760043));
#235030=CARTESIAN_POINT('Ctrl Pts',(-214.053205430375,5.7024678052036,131.923994229952));
#235031=CARTESIAN_POINT('Ctrl Pts',(-214.331653054188,4.02430260700449,
126.611902266833));
#235032=CARTESIAN_POINT('Ctrl Pts',(-214.610100678001,-1.35200008892003,
125.152474715061));
#235033=CARTESIAN_POINT('Ctrl Pts',(-214.888548301814,-5.48588075200302,
128.886854197714));
#235034=CARTESIAN_POINT('Ctrl Pts',(-215.166995925626,-4.5785050041694,
134.383328404815));
#235035=CARTESIAN_POINT('Ctrl Pts',(-215.445443549439,0.536293170092427,
136.59090605773));
#235036=CARTESIAN_POINT('Ctrl Pts',(-215.723891173253,5.15826412041666,
133.480931139593));
#235037=CARTESIAN_POINT('Ctrl Pts',(-216.002338797065,5.04004233928969,
127.911318669453));
#235038=CARTESIAN_POINT('Ctrl Pts',(-216.280786420879,0.290267868112,125.000270416672));
#235039=CARTESIAN_POINT('Ctrl Pts',(-216.559234044691,-4.72624859348692,
127.422897512942));
#235040=CARTESIAN_POINT('Ctrl Pts',(-216.837681668504,-5.39957348775117,
132.952924008705));
#235041=CARTESIAN_POINT('Ctrl Pts',(-217.116129292317,-1.11095413060172,
136.508525711168));
#235042=CARTESIAN_POINT('Ctrl Pts',(-217.39457691613,4.19857779944424,134.822278356567));
#235043=CARTESIAN_POINT('Ctrl Pts',(-217.673024539943,5.64982184372931,
129.443760886018));
#235044=CARTESIAN_POINT('Ctrl Pts',(-217.951472163756,1.90915562276867,
125.315568099769));
#235045=CARTESIAN_POINT('Ctrl Pts',(-218.229919787568,-3.58593134807924,
126.231307494954));
#235046=CARTESIAN_POINT('Ctrl Pts',(-218.508367411381,-5.78572259252759,
131.349459303753));
#235047=CARTESIAN_POINT('Ctrl Pts',(-218.786815035194,-2.66871742270537,
135.966692049498));
#235048=CARTESIAN_POINT('Ctrl Pts',(-219.065262659007,2.90070868448967,
135.839994403207));
#235049=CARTESIAN_POINT('Ctrl Pts',(-219.34371028282,5.80452521813531,131.085795312298));
#235050=CARTESIAN_POINT('Ctrl Pts',(-219.622157906633,3.37426664313623,
126.07297148578));
#235051=CARTESIAN_POINT('Ctrl Pts',(-219.900605530446,-2.15677813481551,
125.408063130162));
#235052=CARTESIAN_POINT('Ctrl Pts',(-220.179053154259,-5.70584917134113,
129.702088541682));
#235053=CARTESIAN_POINT('Ctrl Pts',(-220.457500778071,-4.01152356563293,
135.009048141953));
#235054=CARTESIAN_POINT('Ctrl Pts',(-220.735948401884,1.36919622307095,
136.452105317718));
#235055=CARTESIAN_POINT('Ctrl Pts',(-221.014396025697,5.49169157172664,
132.705161021709));
#235056=CARTESIAN_POINT('Ctrl Pts',(-221.29284364951,4.56759065001379,127.211474013555));
#235057=CARTESIAN_POINT('Ctrl Pts',(-221.571291273323,-0.553902939853376,
125.019474272218));
#235058=CARTESIAN_POINT('Ctrl Pts',(-221.849738897136,-5.16638678765824,
128.143502474846));
#235059=CARTESIAN_POINT('Ctrl Pts',(-222.128186520948,-5.03121356963114,
133.712729320486));
#235060=CARTESIAN_POINT('Ctrl Pts',(-222.406634144762,-0.272600869560251,
136.609307409853));
#235061=CARTESIAN_POINT('Ctrl Pts',(-222.685081768574,4.73651871234416,
134.171422984523));
#235062=CARTESIAN_POINT('Ctrl Pts',(-222.963529392388,5.39300898940659,
128.639372734101));
#235063=CARTESIAN_POINT('Ctrl Pts',(-223.2419770162,1.09358746834067,125.096840583045));
#235064=CARTESIAN_POINT('Ctrl Pts',(-223.520424640014,-4.21078751141269,
126.799240515859));
#235065=CARTESIAN_POINT('Ctrl Pts',(-223.798872263826,-5.64565447658353,
132.182150161146));
#235066=CARTESIAN_POINT('Ctrl Pts',(-224.077319887639,-1.89244078332859,
136.298938524645));
#235067=CARTESIAN_POINT('Ctrl Pts',(-224.355767511452,3.59983353893359,
135.366478216591));
#235068=CARTESIAN_POINT('Ctrl Pts',(-224.634215135265,5.78403670056078,
130.241654706868));
#235069=CARTESIAN_POINT('Ctrl Pts',(-224.912662759078,2.65299270027449,
125.633930439363));
#235070=CARTESIAN_POINT('Ctrl Pts',(-225.191110382891,-2.91602198566553,
125.77757891607));
#235071=CARTESIAN_POINT('Ctrl Pts',(-225.469558006704,-5.8053549223724,
130.540594204513));
#235072=CARTESIAN_POINT('Ctrl Pts',(-225.748005630516,-3.35985029277391,
135.545997940844));
#235073=CARTESIAN_POINT('Ctrl Pts',(-226.026453254329,2.17319261807209,
136.194068618944));
#235074=CARTESIAN_POINT('Ctrl Pts',(-226.304900878142,5.7091776792716,131.88926094565));
#235075=CARTESIAN_POINT('Ctrl Pts',(-226.583348501955,3.99870736205508,
126.587482871174));
#235076=CARTESIAN_POINT('Ctrl Pts',(-226.861796125768,-1.38637967317499,
125.160809439701));
#235077=CARTESIAN_POINT('Ctrl Pts',(-227.140243749581,-5.49745151716988,
128.920283837883));
#235078=CARTESIAN_POINT('Ctrl Pts',(-227.418691373394,-4.55663398232247,
134.411132754326));
#235079=CARTESIAN_POINT('Ctrl Pts',(-227.697138997207,0.571507578333558,
136.5875342777));
#235080=CARTESIAN_POINT('Ctrl Pts',(-227.97558662102,5.17446159419872,133.44948173115));
#235081=CARTESIAN_POINT('Ctrl Pts',(-228.254034244832,5.02233819149715,
127.880692102567));
#235082=CARTESIAN_POINT('Ctrl Pts',(-228.532481868645,0.254931345670833,
124.998611010119));
#235083=CARTESIAN_POINT('Ctrl Pts',(-228.810929492458,-4.74674495273865,
127.451730180279));
#235084=CARTESIAN_POINT('Ctrl Pts',(-229.089377116271,-5.38639453096373,
132.985752937203));
#235085=CARTESIAN_POINT('Ctrl Pts',(-229.367824740084,-1.07621067523457,
136.515182719319));
#235086=CARTESIAN_POINT('Ctrl Pts',(-229.646272363897,4.22295821522052,
134.796645979094));
#235087=CARTESIAN_POINT('Ctrl Pts',(-229.92471998771,5.64143480886619,129.409394025606));
#235088=CARTESIAN_POINT('Ctrl Pts',(-230.203167611523,1.87570841257552,
125.304048222223));
#235089=CARTESIAN_POINT('Ctrl Pts',(-230.481615235336,-3.61370238142155,
126.25322080496));
#235090=CARTESIAN_POINT('Ctrl Pts',(-230.760062859148,-5.78229722606833,
131.384668539942));
#235091=CARTESIAN_POINT('Ctrl Pts',(-231.038510482961,-2.63724340088164,
135.982841643878));
#235092=CARTESIAN_POINT('Ctrl Pts',(-231.316958106774,2.93130827321233,
135.822243667495));
#235093=CARTESIAN_POINT('Ctrl Pts',(-231.595405730587,5.80613084659478,
131.050456305442));
#235094=CARTESIAN_POINT('Ctrl Pts',(-231.8738533544,3.34540281721704,126.052519028673));
#235095=CARTESIAN_POINT('Ctrl Pts',(-232.152300978213,-2.18958696916944,
125.42129203173));
#235096=CARTESIAN_POINT('Ctrl Pts',(-232.430748602025,-5.71245329815966,
129.736842087648));
#235097=CARTESIAN_POINT('Ctrl Pts',(-232.709196225839,-3.98585411499877,
135.033389521383));
#235098=CARTESIAN_POINT('Ctrl Pts',(-232.987643849651,1.40355028004735,
136.443665992055));
#235099=CARTESIAN_POINT('Ctrl Pts',(-233.266091473464,5.50316053497282,
132.671696318956));
#235100=CARTESIAN_POINT('Ctrl Pts',(-233.544539097277,4.5456351025967,127.183736360699));
#235101=CARTESIAN_POINT('Ctrl Pts',(-233.82298672109,-0.589106922445798,
125.022953217175));
#235102=CARTESIAN_POINT('Ctrl Pts',(-234.101434344904,-5.18248846523346,
128.175001037157));
#235103=CARTESIAN_POINT('Ctrl Pts',(-234.379881968716,-5.01341628710851,
133.743301860178));
#235104=CARTESIAN_POINT('Ctrl Pts',(-234.658329592529,-0.237259460132118,
136.610859256499));
#235105=CARTESIAN_POINT('Ctrl Pts',(-234.936777216342,4.75692721993639,
134.14252806687));
#235106=CARTESIAN_POINT('Ctrl Pts',(-235.215224840155,5.37973017369771,
128.606584069875));
#235107=CARTESIAN_POINT('Ctrl Pts',(-235.493672463967,1.05882391226032,
125.090289352854));
#235108=CARTESIAN_POINT('Ctrl Pts',(-235.772120087781,-4.23508979812022,
126.824946980203));
#235109=CARTESIAN_POINT('Ctrl Pts',(-236.050567711593,-5.63716287966734,
132.216491335124));
#235110=CARTESIAN_POINT('Ctrl Pts',(-236.329015335406,-1.85895866551617,
136.310356547029));
#235111=CARTESIAN_POINT('Ctrl Pts',(-236.607462959219,3.62753774706455,
135.344480482612));
#235112=CARTESIAN_POINT('Ctrl Pts',(-236.885910583032,5.78050418516386,
130.206456059403));
#235113=CARTESIAN_POINT('Ctrl Pts',(-237.164358206845,2.62146967042642,
125.617876715884));
#235114=CARTESIAN_POINT('Ctrl Pts',(-237.442805830658,-2.94656740551997,
125.795422704185));
#235115=CARTESIAN_POINT('Ctrl Pts',(-237.72125345447,-5.80685298361372,
130.575937934662));
#235116=CARTESIAN_POINT('Ctrl Pts',(-237.999701078284,-3.33092435030571,
135.566362451659));
#235117=CARTESIAN_POINT('Ctrl Pts',(-238.278148702096,2.20596103623244,
136.180739919846));
#235118=CARTESIAN_POINT('Ctrl Pts',(-238.55659632591,5.7156759976606,131.854487459968));
#235119=CARTESIAN_POINT('Ctrl Pts',(-238.835043949722,3.97296394353457,
126.56321973347));
#235120=CARTESIAN_POINT('Ctrl Pts',(-239.113491573535,-1.42070788462113,
125.169353288205));
#235121=CARTESIAN_POINT('Ctrl Pts',(-239.391939197348,-5.50881857224844,
128.95378329321));
#235122=CARTESIAN_POINT('Ctrl Pts',(-239.670386821161,-4.53459411272838,
134.438803453569));
#235123=CARTESIAN_POINT('Ctrl Pts',(-239.948834444974,0.606700809151854,
136.583948200045));
#235124=CARTESIAN_POINT('Ctrl Pts',(-240.227282068787,5.1904673264033,133.417934306771));
#235125=CARTESIAN_POINT('Ctrl Pts',(-240.5057296926,5.00444793911587,127.850173873291));
#235126=CARTESIAN_POINT('Ctrl Pts',(-240.784177316413,0.21958537665436,
124.997166737753));
#235127=CARTESIAN_POINT('Ctrl Pts',(-241.062624940225,-4.76706541961049,
127.48068708057));
#235128=CARTESIAN_POINT('Ctrl Pts',(-241.341072564039,-5.37301597934592,
133.018501033406));
#235129=CARTESIAN_POINT('Ctrl Pts',(-241.619520187851,-1.04142734048567,
136.521628110858));
#235130=CARTESIAN_POINT('Ctrl Pts',(-241.897967811664,4.24718214772698,
134.770865666018));
#235131=CARTESIAN_POINT('Ctrl Pts',(-242.176415435477,5.63283872856131,
129.375078856195));
#235132=CARTESIAN_POINT('Ctrl Pts',(-242.45486305929,1.84219169731802,125.292732160775));
#235133=CARTESIAN_POINT('Ctrl Pts',(-242.733310683103,-3.64133950769301,
126.275302759127));
#235134=CARTESIAN_POINT('Ctrl Pts',(-243.011758306915,-5.77865759445851,
131.419856272607));
#235135=CARTESIAN_POINT('Ctrl Pts',(-243.290205930729,-2.60567165503458,
135.998799347738));
#235136=CARTESIAN_POINT('Ctrl Pts',(-243.568653554541,2.96179924122969,
135.80430699228));
#235137=CARTESIAN_POINT('Ctrl Pts',(-243.847101178355,5.80752132674009,
131.015108179419));
#235138=CARTESIAN_POINT('Ctrl Pts',(-244.125548802166,3.31641502616601,
126.032242652805));
#235139=CARTESIAN_POINT('Ctrl Pts',(-244.403996425981,-2.22231466757369,
125.434720404883));
#235140=CARTESIAN_POINT('Ctrl Pts',(-244.682444049792,-5.71884574792013,
129.771635190908));
#235141=CARTESIAN_POINT('Ctrl Pts',(-244.960891673606,-3.96003696707471,
135.05757419259));
#235142=CARTESIAN_POINT('Ctrl Pts',(-245.239339297418,1.43785232795156,
136.435017699859));
#235143=CARTESIAN_POINT('Ctrl Pts',(-245.517786921232,5.51442557658153,
132.638162421391));
#235144=CARTESIAN_POINT('Ctrl Pts',(-245.796234545044,4.52351111499922,
127.156132871406));
#235145=CARTESIAN_POINT('Ctrl Pts',(-246.074682168857,-0.624289075464052,
125.026646394309));
#235146=CARTESIAN_POINT('Ctrl Pts',(-246.353129792671,-5.19839810379266,
128.206597031353));
#235147=CARTESIAN_POINT('Ctrl Pts',(-246.631577416483,-4.99543323060155,
133.773765496319));
#235148=CARTESIAN_POINT('Ctrl Pts',(-246.910025040296,-0.201909258968066,
136.612195941205));
#235149=CARTESIAN_POINT('Ctrl Pts',(-247.188472664109,4.77715945784187,
134.113509452194));
#235150=CARTESIAN_POINT('Ctrl Pts',(-247.466920287922,5.36625201010822,
128.573876845067));
#235151=CARTESIAN_POINT('Ctrl Pts',(-247.745367911734,1.02402112107033,
125.083949859676));
#235152=CARTESIAN_POINT('Ctrl Pts',(-248.023815535548,-4.25923515201858,
126.850800903184));
#235153=CARTESIAN_POINT('Ctrl Pts',(-248.30226315936,-5.62846239560694,
132.250780182078));
#235154=CARTESIAN_POINT('Ctrl Pts',(-248.580710783174,-1.82540766330725,
136.32157054271));
#235155=CARTESIAN_POINT('Ctrl Pts',(-248.859158406986,3.65510753545023,
135.322314512822));
#235156=CARTESIAN_POINT('Ctrl Pts',(-249.137606030799,5.7767574710584,130.171279567513));
#235157=CARTESIAN_POINT('Ctrl Pts',(-249.416053654612,2.58984950105633,
125.602015179472));
#235158=CARTESIAN_POINT('Ctrl Pts',(-249.694501278425,-2.97700363923603,
125.813452100338));
#235159=CARTESIAN_POINT('Ctrl Pts',(-249.972948902238,-5.80813586978118,
130.611290129096));
#235160=CARTESIAN_POINT('Ctrl Pts',(-250.251396526051,-3.30187497921299,
135.586550504748));
#235161=CARTESIAN_POINT('Ctrl Pts',(-250.529844149864,2.23864771169993,
136.167211997028));
#235162=CARTESIAN_POINT('Ctrl Pts',(-250.808291773676,5.72196251956533,
131.819675061465));
#235163=CARTESIAN_POINT('Ctrl Pts',(-251.08673939749,3.94707330538994,126.539113752772));
#235164=CARTESIAN_POINT('Ctrl Pts',(-251.365187021302,-1.45498345124562,
125.178105944033));
#235165=CARTESIAN_POINT('Ctrl Pts',(-251.643634645115,-5.5199814959705,
128.987351322257));
#235166=CARTESIAN_POINT('Ctrl Pts',(-251.922082268928,-4.51238621219265,
134.466339477392));
#235167=CARTESIAN_POINT('Ctrl Pts',(-252.200529892741,0.641871558658502,
136.580147957277));
#235168=CARTESIAN_POINT('Ctrl Pts',(-252.478977516554,5.20628072353487,
133.386290036154));
#235169=CARTESIAN_POINT('Ctrl Pts',(-252.757425140367,4.98637224582674,
127.819765111179));
#235170=CARTESIAN_POINT('Ctrl Pts',(-253.035872764179,0.184231269403876,
124.995937655572));
#235171=CARTESIAN_POINT('Ctrl Pts',(-253.314320387993,-4.78720923844335,
127.509767136124));
#235172=CARTESIAN_POINT('Ctrl Pts',(-253.592768011806,-5.35943833369967,
133.051167092665));
#235173=CARTESIAN_POINT('Ctrl Pts',(-253.871215635618,-1.00660540571931,
136.527861630253));
#235174=CARTESIAN_POINT('Ctrl Pts',(-254.149663259431,4.27124868131666,
134.744938404161));
#235175=CARTESIAN_POINT('Ctrl Pts',(-254.428110883244,5.62403395537261,
129.340816589823));
#235176=CARTESIAN_POINT('Ctrl Pts',(-254.706558507057,1.80860665472018,
125.281620447135));
#235177=CARTESIAN_POINT('Ctrl Pts',(-254.98500613087,-3.66884158147516,
126.297552326988));
#235178=CARTESIAN_POINT('Ctrl Pts',(-255.263453754682,-5.77480406163408,
131.45502159855));
#235179=CARTESIAN_POINT('Ctrl Pts',(-255.541901378496,-2.57400292253984,
136.014563813166));
#235180=CARTESIAN_POINT('Ctrl Pts',(-255.820349002309,2.99217964199006,
135.78618647082));
#235181=CARTESIAN_POINT('Ctrl Pts',(-256.098796626121,5.80869814913581,
130.979749546569));
#235182=CARTESIAN_POINT('Ctrl Pts',(-256.377244249934,3.28730143236016,
126.01214820295));
#235183=CARTESIAN_POINT('Ctrl Pts',(-256.655691873747,-2.25495451926359,
125.448338134603));
#235184=CARTESIAN_POINT('Ctrl Pts',(-256.93413949756,-5.72503666514098,
129.806484721847));
#235185=CARTESIAN_POINT('Ctrl Pts',(-257.212587121373,-3.93405347634203,
135.081566970265));
#235186=CARTESIAN_POINT('Ctrl Pts',(-257.491034745186,1.47206408278265,
136.426225506557));
#235187=CARTESIAN_POINT('Ctrl Pts',(-257.769482368999,5.52555616721843,
132.604438319186));
#235188=CARTESIAN_POINT('Ctrl Pts',(-258.047929992812,4.50108754276566,
127.128895412351));
#235189=CARTESIAN_POINT('Ctrl Pts',(-258.326377616624,-0.659198908970111,
125.030117734768));
#235190=CARTESIAN_POINT('Ctrl Pts',(-258.604825240438,-5.21458571703409,
128.239112839452));
#235191=CARTESIAN_POINT('Ctrl Pts',(-258.883272864251,-4.97637574492231,
133.802560593787));
#235192=CARTESIAN_POINT('Ctrl Pts',(-259.161720488063,-0.168236736403017,
136.616288572087));
#235193=CARTESIAN_POINT('Ctrl Pts',(-259.440168111876,4.80044487344316,
134.078525892203));
#235194=CARTESIAN_POINT('Ctrl Pts',(-259.672207798387,5.25516631655033,
129.4749169549));
#235195=CARTESIAN_POINT('Ctrl Pts',(-259.857849473896,3.17366342871357,
126.795179433485));
#235196=CARTESIAN_POINT('Ctrl Pts',(-259.9506752748,1.64266665146648,126.102093112095));
#235197=CARTESIAN_POINT('Ctrl Pts',(-259.997093138402,0.835778587061721,
125.962806053044));
#235198=CARTESIAN_POINT('Ctrl Pts',(210.385579563201,-2.29217962691353,
126.082387726892));
#235199=CARTESIAN_POINT('Ctrl Pts',(210.339169886847,-3.0789974560272,126.464330840008));
#235200=CARTESIAN_POINT('Ctrl Pts',(210.246352273192,-4.44507089109247,
127.629120819077));
#235201=CARTESIAN_POINT('Ctrl Pts',(210.060718784933,-5.78798125627161,
130.996088365878));
#235202=CARTESIAN_POINT('Ctrl Pts',(209.828679098422,-3.95783017776954,
135.586872998689));
#235203=CARTESIAN_POINT('Ctrl Pts',(209.550231474609,1.89393692750204,136.720289837399));
#235204=CARTESIAN_POINT('Ctrl Pts',(209.271783850796,5.99602695027556,132.40812259401));
#235205=CARTESIAN_POINT('Ctrl Pts',(208.993336226983,4.59288360023261,126.626877830413));
#235206=CARTESIAN_POINT('Ctrl Pts',(208.71488860317,-1.03344059257722,124.682062423228));
#235207=CARTESIAN_POINT('Ctrl Pts',(208.436440979357,-5.70873650289865,
128.364647771496));
#235208=CARTESIAN_POINT('Ctrl Pts',(208.157993355544,-5.13869562717284,
134.288517668348));
#235209=CARTESIAN_POINT('Ctrl Pts',(207.879545731732,0.153933173725622,
137.010984097728));
#235210=CARTESIAN_POINT('Ctrl Pts',(207.601098107919,5.30490488755997,134.029672582798));
#235211=CARTESIAN_POINT('Ctrl Pts',(207.322650484106,5.58103410012833,128.084559773234));
#235212=CARTESIAN_POINT('Ctrl Pts',(207.044202860293,0.728409521696789,
124.638756607567));
#235213=CARTESIAN_POINT('Ctrl Pts',(206.76575523648,-4.79355811073501,126.858871164077));
#235214=CARTESIAN_POINT('Ctrl Pts',(206.487307612667,-5.91049575314416,
132.704682504842));
#235215=CARTESIAN_POINT('Ctrl Pts',(206.208859988854,-1.59596820864792,
136.804198957117));
#235216=CARTESIAN_POINT('Ctrl Pts',(205.930412365042,4.1851717387407,135.390152799229));
#235217=CARTESIAN_POINT('Ctrl Pts',(205.651964741228,6.12034565262566,129.76198992389));
#235218=CARTESIAN_POINT('Ctrl Pts',(205.373517117416,2.43121966936229,125.091713591677));
#235219=CARTESIAN_POINT('Ctrl Pts',(205.095069493603,-3.49207776276838,
125.671081434371));
#235220=CARTESIAN_POINT('Ctrl Pts',(204.81662186979,-6.20632667560231,130.96768173473));
#235221=CARTESIAN_POINT('Ctrl Pts',(204.538174245977,-3.21726438559061,
136.114198085604));
#235222=CARTESIAN_POINT('Ctrl Pts',(204.259726622164,2.72830660529182,136.381233108793));
#235223=CARTESIAN_POINT('Ctrl Pts',(203.981278998351,6.16669716267351,131.523394807979));
#235224=CARTESIAN_POINT('Ctrl Pts',(203.702831374538,3.9381942601484,126.004799186432));
#235225=CARTESIAN_POINT('Ctrl Pts',(203.424383750725,-1.909316761502,124.896766062528));
#235226=CARTESIAN_POINT('Ctrl Pts',(203.145936126912,-6.00225896230248,
129.217523725228));
#235227=CARTESIAN_POINT('Ctrl Pts',(202.867488503099,-4.57941839934143,
134.996506974633));
#235228=CARTESIAN_POINT('Ctrl Pts',(202.589040879287,1.05168395343957,136.923112517541));
#235229=CARTESIAN_POINT('Ctrl Pts',(202.310593255474,5.71634013176502,133.226883983125));
#235230=CARTESIAN_POINT('Ctrl Pts',(202.032145631661,5.12795898713612,127.30447482202));
#235231=CARTESIAN_POINT('Ctrl Pts',(201.753698007848,-0.172765951628197,
124.598289728405));
#235232=CARTESIAN_POINT('Ctrl Pts',(201.475250384035,-5.31472742110118,
127.595180598346));
#235233=CARTESIAN_POINT('Ctrl Pts',(201.196802760222,-5.57271402936141,
133.541151128878));
#235234=CARTESIAN_POINT('Ctrl Pts',(200.918355136409,-0.709648686901125,
136.972144879116));
#235235=CARTESIAN_POINT('Ctrl Pts',(200.639907512596,4.80554913058071,134.735246206027));
#235236=CARTESIAN_POINT('Ctrl Pts',(200.361459888783,5.90468206117194,128.886055711564));
#235237=CARTESIAN_POINT('Ctrl Pts',(200.083012264971,1.57770063730838,124.799693711321));
#235238=CARTESIAN_POINT('Ctrl Pts',(199.804564641158,-4.19911059728431,
126.231327253625));
#235239=CARTESIAN_POINT('Ctrl Pts',(199.526117017345,-6.11714433092778,
131.865355052293));
#235240=CARTESIAN_POINT('Ctrl Pts',(199.247669393532,-2.4138212635637,136.524380797905));
#235241=CARTESIAN_POINT('Ctrl Pts',(198.969221769719,3.50768562329156,135.926987436306));
#235242=CARTESIAN_POINT('Ctrl Pts',(198.690774145906,6.20580078231077,130.622150282517));
#235243=CARTESIAN_POINT('Ctrl Pts',(198.412326522093,3.20108819260905,125.484755525167));
#235244=CARTESIAN_POINT('Ctrl Pts',(198.13387889828,-2.74526806424844,125.235817970576));
#235245=CARTESIAN_POINT('Ctrl Pts',(197.855431274468,-6.16885708386238,
130.104099070135));
#235246=CARTESIAN_POINT('Ctrl Pts',(197.576983650655,-3.92356780882929,
135.615886322105));
#235247=CARTESIAN_POINT('Ctrl Pts',(197.298536026841,1.92728860557448,136.706116507701));
#235248=CARTESIAN_POINT('Ctrl Pts',(197.020088403029,6.00706094473797,132.372921347066));
#235249=CARTESIAN_POINT('Ctrl Pts',(196.741640779216,4.56663773692898,126.598295504472));
#235250=CARTESIAN_POINT('Ctrl Pts',(196.463193155403,-1.07030245846182,
124.688838023107));
#235251=CARTESIAN_POINT('Ctrl Pts',(196.184745531591,-5.72368698170812,
128.399247046161));
#235252=CARTESIAN_POINT('Ctrl Pts',(195.906297907777,-5.11728278641862,
134.319837945007));
#235253=CARTESIAN_POINT('Ctrl Pts',(195.627850283965,0.191654296427489,
137.009876920548));
#235254=CARTESIAN_POINT('Ctrl Pts',(195.349402660151,5.32447044368961,133.997349569974));
#235255=CARTESIAN_POINT('Ctrl Pts',(195.070955036339,5.56435836804288,128.050621358318));
#235256=CARTESIAN_POINT('Ctrl Pts',(194.792507412526,0.690872786183208,
124.634444998269));
#235257=CARTESIAN_POINT('Ctrl Pts',(194.514059788713,-4.81749113516689,
126.888119675218));
#235258=CARTESIAN_POINT('Ctrl Pts',(194.2356121649,-5.89881605082435,132.740628459178));
#235259=CARTESIAN_POINT('Ctrl Pts',(193.957164541087,-1.55941718895885,
136.81380168864));
#235260=CARTESIAN_POINT('Ctrl Pts',(193.678716917274,4.21300988779493,135.364592151301));
#235261=CARTESIAN_POINT('Ctrl Pts',(193.400269293461,6.11388669464029,129.724752614155));
#235262=CARTESIAN_POINT('Ctrl Pts',(193.121821669648,2.39640030908087,125.077020090361));
#235263=CARTESIAN_POINT('Ctrl Pts',(192.843374045836,-3.52326088986039,
125.692433714928));
#235264=CARTESIAN_POINT('Ctrl Pts',(192.564926422022,-6.20521745188322,
131.005458431507));
#235265=CARTESIAN_POINT('Ctrl Pts',(192.28647879821,-3.1848823173506,136.133684081248));
#235266=CARTESIAN_POINT('Ctrl Pts',(192.008031174397,2.76220407667619,136.36452181979));
#235267=CARTESIAN_POINT('Ctrl Pts',(191.729583550584,6.17095986540858,131.485843042463));
#235268=CARTESIAN_POINT('Ctrl Pts',(191.451135926771,3.90890500597959,125.980915208923));
#235269=CARTESIAN_POINT('Ctrl Pts',(191.172688302958,-1.94524259331895,
124.908498067517));
#235270=CARTESIAN_POINT('Ctrl Pts',(190.894240679145,-6.01180727974115,
129.254090580708));
#235271=CARTESIAN_POINT('Ctrl Pts',(190.615793055332,-4.5538147691942,135.024305522869));
#235272=CARTESIAN_POINT('Ctrl Pts',(190.337345431519,1.08891104802307,136.916597252826));
#235273=CARTESIAN_POINT('Ctrl Pts',(190.058897807707,5.73098080836918,133.192042114338));
#235274=CARTESIAN_POINT('Ctrl Pts',(189.780450183893,5.10655917980125,127.273324325042));
#235275=CARTESIAN_POINT('Ctrl Pts',(189.502002560081,-0.210540865719208,
124.599456387862));
#235276=CARTESIAN_POINT('Ctrl Pts',(189.223554936268,-5.33416414113684,
127.627592311355));
#235277=CARTESIAN_POINT('Ctrl Pts',(188.945107312455,-5.55595115925501,
133.575023114497));
#235278=CARTESIAN_POINT('Ctrl Pts',(188.666659688642,-0.672090485321342,
136.976350437346));
#235279=CARTESIAN_POINT('Ctrl Pts',(188.388212064829,4.82938851117716,134.705920634282));
#235280=CARTESIAN_POINT('Ctrl Pts',(188.109764441016,5.89289539464864,128.850147777659));
#235281=CARTESIAN_POINT('Ctrl Pts',(187.831316817203,1.54111929438253,124.790201052305));
#235282=CARTESIAN_POINT('Ctrl Pts',(187.552869193391,-4.22687014955807,
126.256973159398));
#235283=CARTESIAN_POINT('Ctrl Pts',(187.274421569578,-6.11057242014135,
131.902572188318));
#235284=CARTESIAN_POINT('Ctrl Pts',(186.995973945765,-2.37895715467313,
136.538968434335));
#235285=CARTESIAN_POINT('Ctrl Pts',(186.717526321952,3.53880351742172,135.905540247907));
#235286=CARTESIAN_POINT('Ctrl Pts',(186.439078698139,6.20457663716883,130.584377187674));
#235287=CARTESIAN_POINT('Ctrl Pts',(186.160631074326,3.16864693777749,125.465368152723));
#235288=CARTESIAN_POINT('Ctrl Pts',(185.882183450513,-2.77911450042273,
125.25263236868));
#235289=CARTESIAN_POINT('Ctrl Pts',(185.6037358267,-6.17300548002561,130.14166362836));
#235290=CARTESIAN_POINT('Ctrl Pts',(185.325288202887,-3.89420599156785,
135.639681046572));
#235291=CARTESIAN_POINT('Ctrl Pts',(185.046840579075,1.96317856060187,136.694275209062));
#235292=CARTESIAN_POINT('Ctrl Pts',(184.768392955261,6.0164979221829,132.336325600291));
#235293=CARTESIAN_POINT('Ctrl Pts',(184.489945331449,4.54094961554151,126.570575013045));
#235294=CARTESIAN_POINT('Ctrl Pts',(184.211497707636,-1.10750955006109,
124.695466564429));
#235295=CARTESIAN_POINT('Ctrl Pts',(183.933050083823,-5.73822154400692,
128.434133314579));
#235296=CARTESIAN_POINT('Ctrl Pts',(183.65460246001,-5.09578826671723,134.350923164133));
#235297=CARTESIAN_POINT('Ctrl Pts',(183.376154836197,0.229425484589131,
137.008595292604));
#235298=CARTESIAN_POINT('Ctrl Pts',(183.097707212384,5.34380842361613,133.964878848429));
#235299=CARTESIAN_POINT('Ctrl Pts',(182.819259588571,5.54749248089459,128.016800549989));
#235300=CARTESIAN_POINT('Ctrl Pts',(182.540811964758,0.653301958305029,
124.630353773773));
#235301=CARTESIAN_POINT('Ctrl Pts',(182.262364340946,-4.84124114839195,
126.917517669999));
#235302=CARTESIAN_POINT('Ctrl Pts',(181.983916717133,-5.88692014749505,
132.776500352206));
#235303=CARTESIAN_POINT('Ctrl Pts',(181.70546909332,-1.52280712308763,136.82318296266));
#235304=CARTESIAN_POINT('Ctrl Pts',(181.427021469507,4.24069125417353,135.33886187379));
#235305=CARTESIAN_POINT('Ctrl Pts',(181.148573845694,6.10720153813428,129.687555653153));
#235306=CARTESIAN_POINT('Ctrl Pts',(180.870126221881,2.36149196193127,125.062538635854));
#235307=CARTESIAN_POINT('Ctrl Pts',(180.591678598068,-3.55431336199069,
125.713975516152));
#235308=CARTESIAN_POINT('Ctrl Pts',(180.313230974255,-6.20387834410407,
131.04322762551));
#235309=CARTESIAN_POINT('Ctrl Pts',(180.034783350442,-3.15238220429199,
136.15297262387));
#235310=CARTESIAN_POINT('Ctrl Pts',(179.75633572663,2.79599917883219,136.347604482659));
#235311=CARTESIAN_POINT('Ctrl Pts',(179.477888102817,6.17499390876314,131.448266031944));
#235312=CARTESIAN_POINT('Ctrl Pts',(179.199440479004,3.8794709017638,125.957209961944));
#235313=CARTESIAN_POINT('Ctrl Pts',(178.920992855191,-1.98109634126673,
124.920448547985));
#235314=CARTESIAN_POINT('Ctrl Pts',(178.642545231378,-6.02113282860982,
129.290714880887));
#235315=CARTESIAN_POINT('Ctrl Pts',(178.364097607565,-4.52804239515191,
135.051947700091));
#235316=CARTESIAN_POINT('Ctrl Pts',(178.085649983752,1.12609779228193,136.909855496619));
#235317=CARTESIAN_POINT('Ctrl Pts',(177.807202359939,5.74540912154417,133.157111769304));
#235318=CARTESIAN_POINT('Ctrl Pts',(177.528754736127,5.08497014694685,127.242304671825));
#235319=CARTESIAN_POINT('Ctrl Pts',(177.250307112313,-0.248307978092709,
124.600852972375));
#235320=CARTESIAN_POINT('Ctrl Pts',(176.971859488501,-5.35340320178418,
127.660121740658));
#235321=CARTESIAN_POINT('Ctrl Pts',(176.693411864688,-5.53898241132168,
133.608792432211));
#235322=CARTESIAN_POINT('Ctrl Pts',(176.414964240875,-0.634507379188621,
136.980327290216));
#235323=CARTESIAN_POINT('Ctrl Pts',(176.136516617062,4.85304893701009,134.676450488799));
#235324=CARTESIAN_POINT('Ctrl Pts',(175.858068993249,5.88089036471739,128.814312257825));
#235325=CARTESIAN_POINT('Ctrl Pts',(175.579621369436,1.50448084471559,124.780931250186));
#235326=CARTESIAN_POINT('Ctrl Pts',(175.301173745623,-4.25447307360455,
126.282787570284));
#235327=CARTESIAN_POINT('Ctrl Pts',(175.02272612181,-6.10377407984646,131.939748629711));
#235328=CARTESIAN_POINT('Ctrl Pts',(174.744278497998,-2.34400489265046,
136.553343572764));
#235329=CARTESIAN_POINT('Ctrl Pts',(174.465830874185,3.56979027988629,135.883904033421));
#235330=CARTESIAN_POINT('Ctrl Pts',(174.187383250372,6.20312257915782,130.546612244398));
#235331=CARTESIAN_POINT('Ctrl Pts',(173.908935626559,3.13608826756835,125.446178618609));
#235332=CARTESIAN_POINT('Ctrl Pts',(173.630488002746,-2.81285795548731,
125.269652488117));
#235333=CARTESIAN_POINT('Ctrl Pts',(173.352040378933,-6.17692513320066,
130.179252743065));
#235334=CARTESIAN_POINT('Ctrl Pts',(173.07359275512,-3.86469987307124,135.663296596462));
#235335=CARTESIAN_POINT('Ctrl Pts',(172.795145131307,1.99899576932572,136.682215657471));
#235336=CARTESIAN_POINT('Ctrl Pts',(172.516697507494,6.02571195608475,132.29967308599));
#235337=CARTESIAN_POINT('Ctrl Pts',(172.238249883681,4.51509322759614,126.543011406101));
#235338=CARTESIAN_POINT('Ctrl Pts',(171.959802259869,-1.14467560248665,
124.702321473066));
#235339=CARTESIAN_POINT('Ctrl Pts',(171.681354636056,-5.75254347439624,
128.469107412642));
#235340=CARTESIAN_POINT('Ctrl Pts',(171.402907012243,-5.07410492070761,
134.38187696408));
#235341=CARTESIAN_POINT('Ctrl Pts',(171.12445938843,0.267188171305193,137.007083764462));
#235342=CARTESIAN_POINT('Ctrl Pts',(170.846011764617,5.36294838675633,133.932291012718));
#235343=CARTESIAN_POINT('Ctrl Pts',(170.567564140804,5.53042102937231,127.983083035723));
#235344=CARTESIAN_POINT('Ctrl Pts',(170.289116516991,0.615706922082464,
124.62649132937));
#235345=CARTESIAN_POINT('Ctrl Pts',(170.010668893178,-4.86481176764585,
126.947059693175));
#235346=CARTESIAN_POINT('Ctrl Pts',(169.732221269365,-5.87480610217478,
132.812299166869));
#235347=CARTESIAN_POINT('Ctrl Pts',(169.453773645553,-1.48614062903852,
136.832341207004));
#235348=CARTESIAN_POINT('Ctrl Pts',(169.17532602174,4.26821548017818,135.312963568669));
#235349=CARTESIAN_POINT('Ctrl Pts',(168.896878397927,6.10029007702938,129.650400075769));
#235350=CARTESIAN_POINT('Ctrl Pts',(168.618430774114,2.32649610882855,125.048269946673));
#235351=CARTESIAN_POINT('Ctrl Pts',(168.339983150301,-3.58523412773234,
125.735705943466));
#235352=CARTESIAN_POINT('Ctrl Pts',(168.061535526488,-6.2023093493314,131.08098796821));
#235353=CARTESIAN_POINT('Ctrl Pts',(167.783087902675,-3.11976527855146,
136.172062971709));
#235354=CARTESIAN_POINT('Ctrl Pts',(167.504640278862,2.82969067421049,136.330481738588));
#235355=CARTESIAN_POINT('Ctrl Pts',(167.22619265505,6.17879913544756,131.410665161273));
#235356=CARTESIAN_POINT('Ctrl Pts',(166.947745031236,3.84989304232704,125.933684327914));
#235357=CARTESIAN_POINT('Ctrl Pts',(166.669297407424,-2.01687667896098,
124.93261705898));
#235358=CARTESIAN_POINT('Ctrl Pts',(166.39084978361,-6.03023526218728,129.327395269766));
#235359=CARTESIAN_POINT('Ctrl Pts',(166.112402159798,-4.50210223283349,
135.079432481411));
#235360=CARTESIAN_POINT('Ctrl Pts',(165.833954535985,1.16324280857304,136.902887499053));
#235361=CARTESIAN_POINT('Ctrl Pts',(165.555506912173,5.75962453647134,133.122094242209));
#235362=CARTESIAN_POINT('Ctrl Pts',(165.277059288359,5.06319268865361,127.2114170119));
#235363=CARTESIAN_POINT('Ctrl Pts',(164.998611664547,-0.286065889322858,
124.602479430144));
#235364=CARTESIAN_POINT('Ctrl Pts',(164.720164040733,-5.37244389010723,
127.692767680889));
#235365=CARTESIAN_POINT('Ctrl Pts',(164.441716416921,-5.52180841435808,
133.642457830674));
#235366=CARTESIAN_POINT('Ctrl Pts',(164.163268793108,-0.596900761151562,
136.984075290369));
#235367=CARTESIAN_POINT('Ctrl Pts',(163.884821169295,4.87652953132996,134.646836861603));
#235368=CARTESIAN_POINT('Ctrl Pts',(163.606373545482,5.86866741623098,128.778550479967));
#235369=CARTESIAN_POINT('Ctrl Pts',(163.327925921669,1.46778664595768,124.771884648456));
#235370=CARTESIAN_POINT('Ctrl Pts',(163.049478297856,-4.28191834658676,
126.308769529723));
#235371=CARTESIAN_POINT('Ctrl Pts',(162.771030674043,-6.09674956195837,
131.976882998882));
#235372=CARTESIAN_POINT('Ctrl Pts',(162.49258305023,-2.30896577266445,136.567505680515));
#235373=CARTESIAN_POINT('Ctrl Pts',(162.214135426418,3.60064476245918,135.862079594585));
#235374=CARTESIAN_POINT('Ctrl Pts',(161.935687802605,6.20143866215845,130.508856852083));
#235375=CARTESIAN_POINT('Ctrl Pts',(161.657240178792,3.10341338845521,125.427187633898));
#235376=CARTESIAN_POINT('Ctrl Pts',(161.378792554979,-2.84649717906582,
125.2868776982));
#235377=CARTESIAN_POINT('Ctrl Pts',(161.100344931166,-6.18061589814333,
130.216865021372));
#235378=CARTESIAN_POINT('Ctrl Pts',(160.821897307353,-3.83505054669964,
135.686732096692));
#235379=CARTESIAN_POINT('Ctrl Pts',(160.54344968354,2.0347389045262,136.6699382998));
#235380=CARTESIAN_POINT('Ctrl Pts',(160.265002059727,6.03470270501411,132.262965162335));
#235381=CARTESIAN_POINT('Ctrl Pts',(159.986554435914,4.48906953121078,126.51560570502));
#235382=CARTESIAN_POINT('Ctrl Pts',(159.708106812101,-1.18179923853688,
124.709402495009));
#235383=CARTESIAN_POINT('Ctrl Pts',(159.429659188289,-5.76665224217155,
128.50416804437));
#235384=CARTESIAN_POINT('Ctrl Pts',(159.151211564475,-5.05223355187421,
134.412698197843));
#235385=CARTESIAN_POINT('Ctrl Pts',(158.872763940663,0.304940957265202,
137.005342392132));
#235386=CARTESIAN_POINT('Ctrl Pts',(158.59431631685,5.38188962387183,133.899587270395));
#235387=CARTESIAN_POINT('Ctrl Pts',(158.315868693037,5.51314464606502,127.949470064936));
#235388=CARTESIAN_POINT('Ctrl Pts',(158.037421069224,0.57808907061355,124.622857808186));
#235389=CARTESIAN_POINT('Ctrl Pts',(157.758973445411,-4.88820211951067,
126.976744650055));
#235390=CARTESIAN_POINT('Ctrl Pts',(157.480525821598,-5.86247436375394,
132.848023576631));
#235391=CARTESIAN_POINT('Ctrl Pts',(157.202078197785,-1.44941906550188,
136.841276082311));
#235392=CARTESIAN_POINT('Ctrl Pts',(156.923630573973,4.29558154588865,135.286898195607));
#235393=CARTESIAN_POINT('Ctrl Pts',(156.645182950159,6.09315256743229,129.613287258817));
#235394=CARTESIAN_POINT('Ctrl Pts',(156.366735326347,2.29141404655692,125.034214551549));
#235395=CARTESIAN_POINT('Ctrl Pts',(156.088287702534,-3.61602204130483,
125.757624191644));
#235396=CARTESIAN_POINT('Ctrl Pts',(155.809840078721,-6.2005105257049,131.11873806038));
#235397=CARTESIAN_POINT('Ctrl Pts',(155.531392454908,-3.08703274876129,
136.190954417361));
#235398=CARTESIAN_POINT('Ctrl Pts',(155.252944831095,2.86327731436015,136.313154222067));
#235399=CARTESIAN_POINT('Ctrl Pts',(154.974497207282,6.18237540445775,131.373041823765));
#235400=CARTESIAN_POINT('Ctrl Pts',(154.696049583469,3.82017252368788,125.910339178587));
#235401=CARTESIAN_POINT('Ctrl Pts',(154.417601959656,-2.05258228054818,
124.945003149591));
#235402=CARTESIAN_POINT('Ctrl Pts',(154.139154335844,-6.03911424317947,
129.364130388138));
#235403=CARTESIAN_POINT('Ctrl Pts',(153.860706712031,-4.47599524346119,
135.106758848372));
#235404=CARTESIAN_POINT('Ctrl Pts',(153.582259088218,1.20034472047403,136.895693518332));
#235405=CARTESIAN_POINT('Ctrl Pts',(153.303811464405,5.77362652639317,133.086990830643));
#235406=CARTESIAN_POINT('Ctrl Pts',(153.025363840592,5.04122761189337,127.180662489822));
#235407=CARTESIAN_POINT('Ctrl Pts',(152.746916216779,-0.323813200276178,
124.604335700902));
#235408=CARTESIAN_POINT('Ctrl Pts',(152.468468592966,-5.39128550054617,
127.725528922339));
#235409=CARTESIAN_POINT('Ctrl Pts',(152.190020969154,-5.5044298047531,133.6760180624));
#235410=CARTESIAN_POINT('Ctrl Pts',(151.91157334534,-0.55927202473736,136.987594298923));
#235411=CARTESIAN_POINT('Ctrl Pts',(151.633125721528,4.89982942405471,134.617080850036));
#235412=CARTESIAN_POINT('Ctrl Pts',(151.354678097715,5.85622700211526,128.742863769248));
#235413=CARTESIAN_POINT('Ctrl Pts',(151.076230473902,1.43103805782584,124.763061582343));
#235414=CARTESIAN_POINT('Ctrl Pts',(150.797782850089,-4.3092049515099,126.334918074943));
#235415=CARTESIAN_POINT('Ctrl Pts',(150.519335226276,-6.0894991267732,132.013973919806));
#235416=CARTESIAN_POINT('Ctrl Pts',(150.240887602463,-2.27384109310269,
136.581454232806));
#235417=CARTESIAN_POINT('Ctrl Pts',(149.96243997865,3.63136582181627,135.840067740113));
#235418=CARTESIAN_POINT('Ctrl Pts',(149.683992354837,6.19952494856889,130.471112409769));
#235419=CARTESIAN_POINT('Ctrl Pts',(149.405544731024,3.0706235112177,125.40839590231));
#235420=CARTESIAN_POINT('Ctrl Pts',(149.127097107212,-2.88003092464457,
125.30430736064));
#235421=CARTESIAN_POINT('Ctrl Pts',(148.848649483398,-6.18407763809098,
130.254499069545));
#235422=CARTESIAN_POINT('Ctrl Pts',(148.570201859586,-3.80525911111971,
135.709986678852));
#235423=CARTESIAN_POINT('Ctrl Pts',(148.291754235773,2.07040664172831,136.657443590992));
#235424=CARTESIAN_POINT('Ctrl Pts',(148.01330661196,6.04346983581547,132.226203189553));
#235425=CARTESIAN_POINT('Ctrl Pts',(147.734858988147,4.46287949070312,126.488358925329));
#235426=CARTESIAN_POINT('Ctrl Pts',(147.456411364334,-1.21887908258166,
124.716709367866));
#235427=CARTESIAN_POINT('Ctrl Pts',(147.177963740522,-5.78054732452736,
128.53931391058));
#235428=CARTESIAN_POINT('Ctrl Pts',(146.899516116708,-5.03017497066859,
134.44338572333));
#235429=CARTESIAN_POINT('Ctrl Pts',(146.621068492896,0.342682443525903,
137.003371240143));
#235430=CARTESIAN_POINT('Ctrl Pts',(146.342620869082,5.40063143308812,133.866768833311));
#235431=CARTESIAN_POINT('Ctrl Pts',(146.06417324527,5.49566397115542,127.915962883168));
#235432=CARTESIAN_POINT('Ctrl Pts',(145.785725621457,0.540449797841529,
124.619453344862));
#235433=CARTESIAN_POINT('Ctrl Pts',(145.507277997644,-4.91141133724831,
127.006571440652));
#235434=CARTESIAN_POINT('Ctrl Pts',(145.228830373831,-5.84992538918966,
132.883672257711));
#235435=CARTESIAN_POINT('Ctrl Pts',(144.950382750018,-1.41264379320865,
136.849987257496));
#235436=CARTESIAN_POINT('Ctrl Pts',(144.671935126205,4.32278843724517,135.260666720466));
#235437=CARTESIAN_POINT('Ctrl Pts',(144.393487502392,6.08578927382608,129.576218577526));
#235438=CARTESIAN_POINT('Ctrl Pts',(144.11503987858,2.25624707509518,125.020372971309));
#235439=CARTESIAN_POINT('Ctrl Pts',(143.836592254767,-3.64667596185081,
125.779729448496));
#235440=CARTESIAN_POINT('Ctrl Pts',(143.558144630954,-6.19848193988065,
131.156476503179));
#235441=CARTESIAN_POINT('Ctrl Pts',(143.279697007141,-3.05418582783736,
136.209646260801));
#235442=CARTESIAN_POINT('Ctrl Pts',(143.001249383328,2.89675785471595,136.295622575173));
#235443=CARTESIAN_POINT('Ctrl Pts',(142.722801759515,6.18572258327378,131.335397413564));
#235444=CARTESIAN_POINT('Ctrl Pts',(142.444354135702,3.79031044715096,125.887175379022));
#235445=CARTESIAN_POINT('Ctrl Pts',(142.165906511889,-2.0882118229442,124.957606360848));
#235446=CARTESIAN_POINT('Ctrl Pts',(141.887458888076,-6.04776944257254,
129.400918874772));
#235447=CARTESIAN_POINT('Ctrl Pts',(141.609011264264,-4.44972239443904,
135.133925788383));
#235448=CARTESIAN_POINT('Ctrl Pts',(141.33056364045,1.2374021531599,136.888273821029));
#235449=CARTESIAN_POINT('Ctrl Pts',(141.052116016638,5.78741457246075,133.051802835376));
#235450=CARTESIAN_POINT('Ctrl Pts',(140.773668392825,5.01907573059014,127.15004224521));
#235451=CARTESIAN_POINT('Ctrl Pts',(140.495220769012,-0.361548512212229,
124.606421715863));
#235452=CARTESIAN_POINT('Ctrl Pts',(140.216773145199,-5.4099273349182,127.758404251031));
#235453=CARTESIAN_POINT('Ctrl Pts',(139.938325521386,-5.48684722647749,
133.709471883804));
#235454=CARTESIAN_POINT('Ctrl Pts',(139.659877897573,-0.521622564292735,
136.990884185479));
#235455=CARTESIAN_POINT('Ctrl Pts',(139.38143027376,4.92294775179823,134.58718355672));
#235456=CARTESIAN_POINT('Ctrl Pts',(139.102982649947,5.84356958335437,128.707253448052));
#235457=CARTESIAN_POINT('Ctrl Pts',(138.824535026135,1.39423644205237,124.754462378786));
#235458=CARTESIAN_POINT('Ctrl Pts',(138.546087402322,-4.33633187725888,
126.361232236999));
#235459=CARTESIAN_POINT('Ctrl Pts',(138.267639778509,-6.08202304295846,
132.051020018064));
#235460=CARTESIAN_POINT('Ctrl Pts',(137.989192154696,-2.23863215552307,
136.595188712768));
#235461=CARTESIAN_POINT('Ctrl Pts',(137.710744530883,3.66195231957746,135.817869285661));
#235462=CARTESIAN_POINT('Ctrl Pts',(137.43229690707,6.19738150930245,130.433380316089));
#235463=CARTESIAN_POINT('Ctrl Pts',(137.153849283257,3.03771985089675,125.389804120178));
#235464=CARTESIAN_POINT('Ctrl Pts',(136.875401659444,-2.91345794961824,
125.321940829576));
#235465=CARTESIAN_POINT('Ctrl Pts',(136.596954035631,-6.1873102247676,130.29215349304));
#235466=CARTESIAN_POINT('Ctrl Pts',(136.318506411819,-3.77532667026395,
135.733059481234));
#235467=CARTESIAN_POINT('Ctrl Pts',(136.040058788006,2.10599765925102,136.644731994041));
#235468=CARTESIAN_POINT('Ctrl Pts',(135.761611164193,6.05201302361958,132.189388529871));
#235469=CARTESIAN_POINT('Ctrl Pts',(135.48316354038,4.4365240765547,126.461272076668));
#235470=CARTESIAN_POINT('Ctrl Pts',(135.204715916567,-1.25591376061384,
124.724241820878));
#235471=CARTESIAN_POINT('Ctrl Pts',(134.926268292754,-5.79422820657625,
128.574543708929));
#235472=CARTESIAN_POINT('Ctrl Pts',(134.647820668941,-5.00792999447956,
134.473938403405));
#235473=CARTESIAN_POINT('Ctrl Pts',(134.369373045128,0.380411231562576,
137.001170381535));
#235474=CARTESIAN_POINT('Ctrl Pts',(134.090925421316,5.41917311992063,133.833836917565));
#235475=CARTESIAN_POINT('Ctrl Pts',(133.812477797503,5.4779796523963,127.88256273204));
#235476=CARTESIAN_POINT('Ctrl Pts',(133.53403017369,0.502790498503515,124.616278065551));
#235477=CARTESIAN_POINT('Ctrl Pts',(133.255582549877,-4.93443856083268,
127.036538959725));
#235478=CARTESIAN_POINT('Ctrl Pts',(132.977134926064,-5.83715964348875,
132.919243889133));
#235479=CARTESIAN_POINT('Ctrl Pts',(132.698687302251,-1.37581617488021,
136.858474409763));
#235480=CARTESIAN_POINT('Ctrl Pts',(132.420239678438,4.34983514608645,135.234270115264));
#235481=CARTESIAN_POINT('Ctrl Pts',(132.141792054625,6.07820046906025,129.539195405491));
#235482=CARTESIAN_POINT('Ctrl Pts',(131.863344430812,2.22099649756843,125.006745718858));
#235483=CARTESIAN_POINT('Ctrl Pts',(131.584896806999,-3.67719475347803,
125.802020894903));
#235484=CARTESIAN_POINT('Ctrl Pts',(131.306449183186,-6.1962236670286,131.194201898194));
#235485=CARTESIAN_POINT('Ctrl Pts',(131.028001559374,-3.02122573293442,
136.228137809392));
#235486=CARTESIAN_POINT('Ctrl Pts',(130.749553935561,2.93013105464412,136.277887447547));
#235487=CARTESIAN_POINT('Ctrl Pts',(130.471106311748,6.18884054786473,131.2977333256));
#235488=CARTESIAN_POINT('Ctrl Pts',(130.192658687935,3.76030791926647,125.864193787566));
#235489=CARTESIAN_POINT('Ctrl Pts',(129.914211064122,-2.12376398588317,
124.970426225734));
#235490=CARTESIAN_POINT('Ctrl Pts',(129.635763440309,-6.05620053964477,
129.437759366456));
#235491=CARTESIAN_POINT('Ctrl Pts',(129.357315816496,-4.42328465931731,
135.160932294765));
#235492=CARTESIAN_POINT('Ctrl Pts',(129.078868192683,1.27441373345414,136.880628682086));
#235493=CARTESIAN_POINT('Ctrl Pts',(128.800420568871,5.80098816375315,133.01653156031));
#235494=CARTESIAN_POINT('Ctrl Pts',(128.521972945058,4.99673786558976,127.11955741271));
#235495=CARTESIAN_POINT('Ctrl Pts',(128.243525321245,-0.399270426835251,
124.608737397728));
#235496=CARTESIAN_POINT('Ctrl Pts',(127.965077697432,-5.42836870244348,
127.791392448756));
#235497=CARTESIAN_POINT('Ctrl Pts',(127.686630073619,-5.46906133106002,
133.742818055242));
#235498=CARTESIAN_POINT('Ctrl Pts',(127.408182449806,-0.483953774931917,
136.993944828129));
#235499=CARTESIAN_POINT('Ctrl Pts',(127.129734825993,4.9458836579024,134.557146089508));
#235500=CARTESIAN_POINT('Ctrl Pts',(126.85128720218,5.8306956289736,128.671720835934));
#235501=CARTESIAN_POINT('Ctrl Pts',(126.572839578367,1.35738316233494,124.746087356435));
#235502=CARTESIAN_POINT('Ctrl Pts',(126.294391954555,-4.36329811863544,
126.387711040812));
#235503=CARTESIAN_POINT('Ctrl Pts',(126.015944330741,-6.07432158754323,
132.088019920899));
#235504=CARTESIAN_POINT('Ctrl Pts',(125.737496706929,-2.20334026460562,
136.608708611466));
#235505=CARTESIAN_POINT('Ctrl Pts',(125.459049083116,3.69240312234872,135.795485053802));
#235506=CARTESIAN_POINT('Ctrl Pts',(125.180601459303,6.19500842378515,130.39566196922));
#235507=CARTESIAN_POINT('Ctrl Pts',(124.90215383549,3.00470362674961,125.371412976429));
#235508=CARTESIAN_POINT('Ctrl Pts',(124.623706211677,-2.9467770153362,125.339777451594));
#235509=CARTESIAN_POINT('Ctrl Pts',(124.345258587864,-6.19031353838844,
130.329826896558));
#235510=CARTESIAN_POINT('Ctrl Pts',(124.066810964051,-3.74525433329013,
135.755949648866));
#235511=CARTESIAN_POINT('Ctrl Pts',(123.788363340238,2.14151063825588,136.631803979981));
#235512=CARTESIAN_POINT('Ctrl Pts',(123.509915716426,6.0603319518555,132.152522547471));
#235513=CARTESIAN_POINT('Ctrl Pts',(123.231468092613,4.4100042653751,126.43434616275));
#235514=CARTESIAN_POINT('Ctrl Pts',(122.9530204688,-1.29290190029971,124.731999574929));
#235515=CARTESIAN_POINT('Ctrl Pts',(122.674572844987,-5.80769438136815,
128.609856133963));
#235516=CARTESIAN_POINT('Ctrl Pts',(122.396125221174,-4.98549944760296,
134.504355105923));
#235517=CARTESIAN_POINT('Ctrl Pts',(122.117677597361,0.418125923321227,
136.998739897863));
#235518=CARTESIAN_POINT('Ctrl Pts',(121.839229973548,5.43751399730024,133.80079274346));
#235519=CARTESIAN_POINT('Ctrl Pts',(121.560782349735,5.46009234508668,127.849270849208));
#235520=CARTESIAN_POINT('Ctrl Pts',(121.282334725922,0.465112568078527,
124.613332087916));
#235521=CARTESIAN_POINT('Ctrl Pts',(121.00388710211,-4.95728293698158,127.066646096814));
#235522=CARTESIAN_POINT('Ctrl Pts',(120.725439478297,-5.82417759969065,
132.954737152777));
#235523=CARTESIAN_POINT('Ctrl Pts',(120.446991854484,-1.33893757517749,
136.866737224615));
#235524=CARTESIAN_POINT('Ctrl Pts',(120.168544230671,4.37672067018674,135.207709358136));
#235525=CARTESIAN_POINT('Ctrl Pts',(119.890096606858,6.07038643434081,129.502219114618));
#235526=CARTESIAN_POINT('Ctrl Pts',(119.611648983045,2.18566362019961,124.993333299159));
#235527=CARTESIAN_POINT('Ctrl Pts',(119.333201359232,-3.7075772853013,125.82449770485));
#235528=CARTESIAN_POINT('Ctrl Pts',(119.054753735419,-6.19373579082994,
131.231912847497));
#235529=CARTESIAN_POINT('Ctrl Pts',(118.776306111606,-2.98815368540088,
136.246428377926));
#235530=CARTESIAN_POINT('Ctrl Pts',(118.497858487794,2.96339567748857,136.259949496373));
#235531=CARTESIAN_POINT('Ctrl Pts',(118.219410863981,6.1917291826932,131.26005095553));
#235532=CARTESIAN_POINT('Ctrl Pts',(117.940963240168,3.73016605178927,125.841395255808));
#235533=CARTESIAN_POINT('Ctrl Pts',(117.662515616355,-2.15923745196658,
124.983462269205));
#235534=CARTESIAN_POINT('Ctrl Pts',(117.384067992542,-6.06440722197891,
129.474650498052));
#235535=CARTESIAN_POINT('Ctrl Pts',(117.105620368729,-4.39668301775581,
135.187777366781));
#235536=CARTESIAN_POINT('Ctrl Pts',(116.827172744916,1.31137808987868,136.872758384795));
#235537=CARTESIAN_POINT('Ctrl Pts',(116.548725121103,5.81434679729579,132.981178312436));
#235538=CARTESIAN_POINT('Ctrl Pts',(116.27027749729,4.97421484463032,127.089209121948));
#235539=CARTESIAN_POINT('Ctrl Pts',(115.991829873478,-0.436977546345769,
124.611282660692));
#235540=CARTESIAN_POINT('Ctrl Pts',(115.713382249665,-5.44660891977013,
127.824492293124));
#235541=CARTESIAN_POINT('Ctrl Pts',(115.434934625852,-5.45107277756375,
133.776055341058));
#235542=CARTESIAN_POINT('Ctrl Pts',(115.156487002039,-0.446267052485976,
136.99677611346));
#235543=CARTESIAN_POINT('Ctrl Pts',(114.878039378226,4.9686362924688,134.526969561451));
#235544=CARTESIAN_POINT('Ctrl Pts',(114.599591754413,5.81760561602206,128.636267249567));
#235545=CARTESIAN_POINT('Ctrl Pts',(114.3211441306,1.32047958428524,124.737936825626));
#235546=CARTESIAN_POINT('Ctrl Pts',(114.042696506787,-4.39010267639563,
126.414353505198));
#235547=CARTESIAN_POINT('Ctrl Pts',(113.764248882975,-6.06639504590774,
132.124972257267));
#235548=CARTESIAN_POINT('Ctrl Pts',(113.485801259161,-2.16796672810439,
136.622013427915));
#235549=CARTESIAN_POINT('Ctrl Pts',(113.207353635349,3.72271710176439,135.772915873991));
#235550=CARTESIAN_POINT('Ctrl Pts',(112.928906011536,6.19240577995249,130.357958766832));
#235551=CARTESIAN_POINT('Ctrl Pts',(112.650458387723,2.97157606220462,125.353223152553));
#235552=CARTESIAN_POINT('Ctrl Pts',(112.37201076391,-2.9799868871482,125.357816565752));
#235553=CARTESIAN_POINT('Ctrl Pts',(112.093563140097,-6.19308746766462,
130.367517884098));
#235554=CARTESIAN_POINT('Ctrl Pts',(111.815115516284,-3.71504321453968,
135.778656333547));
#235555=CARTESIAN_POINT('Ctrl Pts',(111.536667892471,2.1769442627965,136.618660027865));
#235556=CARTESIAN_POINT('Ctrl Pts',(111.258220268658,6.06842631226225,132.115606608435));
#235557=CARTESIAN_POINT('Ctrl Pts',(110.979772644846,4.38332103986566,126.407582181323));
#235558=CARTESIAN_POINT('Ctrl Pts',(110.701325021032,-1.32984213103019,
124.739982342551));
#235559=CARTESIAN_POINT('Ctrl Pts',(110.42287739722,-5.82094534990898,128.645249877167));
#235560=CARTESIAN_POINT('Ctrl Pts',(110.144429773407,-4.96288416121089,
134.534634703787));
#235561=CARTESIAN_POINT('Ctrl Pts',(109.865982149594,0.455825121270016,
136.996079879188));
#235562=CARTESIAN_POINT('Ctrl Pts',(109.587534525781,5.45565338559904,133.767637535461));
#235563=CARTESIAN_POINT('Ctrl Pts',(109.309086901968,5.44200271204727,127.816088468313));
#235564=CARTESIAN_POINT('Ctrl Pts',(109.030639278155,0.427417402736423,
124.610615521118));
#235565=CARTESIAN_POINT('Ctrl Pts',(108.752191654342,-4.97994361918818,
127.096891736289));
#235566=CARTESIAN_POINT('Ctrl Pts',(108.473744030529,-5.81097973884976,
132.990150733429));
#235567=CARTESIAN_POINT('Ctrl Pts',(108.195296406717,-1.30200936065053,
136.874775395874));
#235568=CARTESIAN_POINT('Ctrl Pts',(107.916848782904,4.40344401329306,135.180985433302));
#235569=CARTESIAN_POINT('Ctrl Pts',(107.638401159091,6.06234745921968,129.465291075077));
#235570=CARTESIAN_POINT('Ctrl Pts',(107.359953535278,2.15024975226158,124.980136209215));
#235571=CARTESIAN_POINT('Ctrl Pts',(107.081505911465,-3.73782243148481,
125.847159045447));
#235572=CARTESIAN_POINT('Ctrl Pts',(106.803058287652,-6.19101840347381,
131.269607953695));
#235573=CARTESIAN_POINT('Ctrl Pts',(106.524610663839,-2.95497091073364,
136.264517288637));
#235574=CARTESIAN_POINT('Ctrl Pts',(106.246163040026,2.99655049061638,136.241809386346));
#235575=CARTESIAN_POINT('Ctrl Pts',(105.967715416213,6.1943883807198,131.222351699685));
#235576=CARTESIAN_POINT('Ctrl Pts',(105.689267792401,3.69988596163724,125.818780628557));
#235577=CARTESIAN_POINT('Ctrl Pts',(105.410820168588,-2.19463090671215,
124.996714008204));
#235578=CARTESIAN_POINT('Ctrl Pts',(105.132372544775,-6.07238918547325,
129.511590902545));
#235579=CARTESIAN_POINT('Ctrl Pts',(104.853924920962,-4.36991845548819,
135.214460009678));
#235580=CARTESIAN_POINT('Ctrl Pts',(104.575477297149,1.34829385270585,136.864663220793));
#235581=CARTESIAN_POINT('Ctrl Pts',(104.297029673336,5.82748997807964,132.945744401783));
#235582=CARTESIAN_POINT('Ctrl Pts',(104.018582049523,4.95150750231056,127.058998497491));
#235583=CARTESIAN_POINT('Ctrl Pts',(103.74013442571,-0.474668473492613,
124.614057410436));
#235584=CARTESIAN_POINT('Ctrl Pts',(103.461686801897,-5.46464731100027,
127.857702557609));
#235585=CARTESIAN_POINT('Ctrl Pts',(103.183239178085,-5.43288223256107,
133.809182509633));
#235586=CARTESIAN_POINT('Ctrl Pts',(102.904791554272,-0.408563793450433,
136.999377936557));
#235587=CARTESIAN_POINT('Ctrl Pts',(102.626343930459,4.99120481239017,134.496655090749));
#235588=CARTESIAN_POINT('Ctrl Pts',(102.347896306646,5.80430002955499,128.600894002697));
#235589=CARTESIAN_POINT('Ctrl Pts',(102.069448682833,1.28352707537895,124.730011088381));
#235590=CARTESIAN_POINT('Ctrl Pts',(101.79100105902,-4.41674455728669,126.441158642913));
#235591=CARTESIAN_POINT('Ctrl Pts',(101.512553435207,-6.05824371177293,
132.161875657885));
#235592=CARTESIAN_POINT('Ctrl Pts',(101.234105811394,-2.13251285679878,
136.635102669099));
#235593=CARTESIAN_POINT('Ctrl Pts',(100.955658187581,3.75289313452884,135.750162582539));
#235594=CARTESIAN_POINT('Ctrl Pts',(100.677210563769,6.18957367424645,130.320272106026));
#235595=CARTESIAN_POINT('Ctrl Pts',(100.398762939956,2.93833838481571,125.33523532258));
#235596=CARTESIAN_POINT('Ctrl Pts',(100.120315316143,-3.01308633445025,
125.376057503601));
#235597=CARTESIAN_POINT('Ctrl Pts',(99.8418676923298,-6.19563190980719,
130.405225059005));
#235598=CARTESIAN_POINT('Ctrl Pts',(99.5634200685172,-3.68469443349671,
135.801178693871));
#235599=CARTESIAN_POINT('Ctrl Pts',(99.2849724447041,2.2122972198669,136.605300624745));
#235600=CARTESIAN_POINT('Ctrl Pts',(99.0065248208913,6.07629580490035,132.078642080696));
#235601=CARTESIAN_POINT('Ctrl Pts',(98.7280771970783,4.35647538878314,126.380981124141));
#235602=CARTESIAN_POINT('Ctrl Pts',(98.4496295732656,-1.36673308397146,
124.748189827941));
#235603=CARTESIAN_POINT('Ctrl Pts',(98.1711819494526,-5.8339806211792,128.680723627015));
#235604=CARTESIAN_POINT('Ctrl Pts',(97.8927343256397,-4.94008497332115,
134.564776074971));
#235605=CARTESIAN_POINT('Ctrl Pts',(97.6142867018267,0.493507428451318,
136.993190424079));
#235606=CARTESIAN_POINT('Ctrl Pts',(97.3358390780141,5.47359061265531,133.734372522146));
#235607=CARTESIAN_POINT('Ctrl Pts',(97.0573914542009,5.42371142359607,127.783016818942));
#235608=CARTESIAN_POINT('Ctrl Pts',(96.7789438303882,0.389706399285272,
124.608128465823));
#235609=CARTESIAN_POINT('Ctrl Pts',(96.5004962065753,-5.0024197677526,127.127274757387));
#235610=CARTESIAN_POINT('Ctrl Pts',(96.2220485827623,-5.79756655001767,
133.025483318824));
#235611=CARTESIAN_POINT('Ctrl Pts',(95.9436009589496,-1.26503289968789,
136.882588625681));
#235612=CARTESIAN_POINT('Ctrl Pts',(95.6651533351365,4.4300041851621,135.154099331026));
#235613=CARTESIAN_POINT('Ctrl Pts',(95.3867057113237,6.05408384158403,129.428412655251));
#235614=CARTESIAN_POINT('Ctrl Pts',(95.1082580875108,2.11475620602821,124.967154938047));
#235615=CARTESIAN_POINT('Ctrl Pts',(94.8298104636979,-3.76792907128354,
125.870004076972));
#235616=CARTESIAN_POINT('Ctrl Pts',(94.5513628398851,-6.18807160565406,
131.307285819983));
#235617=CARTESIAN_POINT('Ctrl Pts',(94.2729152160721,-2.92167863853249,
136.282403871234));
#235618=CARTESIAN_POINT('Ctrl Pts',(93.9944675922592,3.02959426546386,136.223467789656));
#235619=CARTESIAN_POINT('Ctrl Pts',(93.7160199684464,6.19681804340696,131.184636955029));
#235620=CARTESIAN_POINT('Ctrl Pts',(93.4375723446334,3.66946877085029,125.796350743805));
#235621=CARTESIAN_POINT('Ctrl Pts',(93.1591247208205,-2.22994303860241,
125.010180951684));
#235622=CARTESIAN_POINT('Ctrl Pts',(92.8806770970077,-6.08014613435319,
129.548579211095));
#235623=CARTESIAN_POINT('Ctrl Pts',(92.6022294731947,-4.3429919642852,135.24097923472));
#235624=CARTESIAN_POINT('Ctrl Pts',(92.323781849382,1.38515965400848,136.856343490049));
#235625=CARTESIAN_POINT('Ctrl Pts',(92.045334225569,5.84041721907928,132.910231141365));
#235626=CARTESIAN_POINT('Ctrl Pts',(91.7668866017561,4.9286166800594,127.028926658805));
#235627=CARTESIAN_POINT('Ctrl Pts',(91.4884389779432,-0.512341811624615,
124.617061544141));
#235628=CARTESIAN_POINT('Ctrl Pts',(91.2099913541303,-5.48248320771468,
127.891022011592));
#235629=CARTESIAN_POINT('Ctrl Pts',(90.9315437303175,-5.41449037010934,
133.842198333429));
#235630=CARTESIAN_POINT('Ctrl Pts',(90.6530961065044,-0.370845394933272,
137.00175020101));
#235631=CARTESIAN_POINT('Ctrl Pts',(90.3746484826917,5.01358838138169,134.466203800718));
#235632=CARTESIAN_POINT('Ctrl Pts',(90.0962008588786,5.79077936261581,128.565602406094));
#235633=CARTESIAN_POINT('Ctrl Pts',(89.817753235066,1.24652700490487,124.722310438393));
#235634=CARTESIAN_POINT('Ctrl Pts',(89.5393056112528,-4.44322277408392,
126.468125460682));
#235635=CARTESIAN_POINT('Ctrl Pts',(89.2608579874402,-6.04986788718945,
132.198728755283));
#235636=CARTESIAN_POINT('Ctrl Pts',(88.9824103636271,-2.09697996444503,
136.647975849991));
#235637=CARTESIAN_POINT('Ctrl Pts',(88.7039627398144,3.78293010245805,135.727226022576));
#235638=CARTESIAN_POINT('Ctrl Pts',(88.4255151160013,6.18651221161165,130.282603383299));
#235639=CARTESIAN_POINT('Ctrl Pts',(88.1470674921886,2.9049918262175,125.317450153056));
#235640=CARTESIAN_POINT('Ctrl Pts',(87.8686198683756,-3.04607413073006,
125.394499589218));
#235641=CARTESIAN_POINT('Ctrl Pts',(87.5901722445627,-6.19794677053091,
130.442947024027));
#235642=CARTESIAN_POINT('Ctrl Pts',(87.3117246207499,-3.65420911474647,
135.823515895262));
#235643=CARTESIAN_POINT('Ctrl Pts',(87.033276996937,2.24756819945024,136.59172626566));
#235644=CARTESIAN_POINT('Ctrl Pts',(86.754829373124,6.08394013816284,132.041630333989));
#235645=CARTESIAN_POINT('Ctrl Pts',(86.4763817493112,4.32946830690299,126.35454397691));
#235646=CARTESIAN_POINT('Ctrl Pts',(86.1979341254982,-1.40357339211569,
124.756621726966));
#235647=CARTESIAN_POINT('Ctrl Pts',(85.9194865016854,-5.84679971215209,
128.716276069012));
#235648=CARTESIAN_POINT('Ctrl Pts',(85.6410388778725,-4.91710272876601,
134.594778102578));
#235649=CARTESIAN_POINT('Ctrl Pts',(85.3625912540596,0.531171448533366,
136.990071639606));
#235650=CARTESIAN_POINT('Ctrl Pts',(85.0841436302467,5.49132501379855,133.700998936161));
#235651=CARTESIAN_POINT('Ctrl Pts',(84.8056960064338,5.4052191575235,127.750057126576));
#235652=CARTESIAN_POINT('Ctrl Pts',(84.527248382621,0.351980955120191,124.60587101419));
#235653=CARTESIAN_POINT('Ctrl Pts',(84.2488007588079,-5.02471054981291,
127.157794034254));
#235654=CARTESIAN_POINT('Ctrl Pts',(83.9703531349953,-5.78393853022499,
133.0607335997));
#235655=CARTESIAN_POINT('Ctrl Pts',(83.6919055111822,-1.22800956246596,
136.890176624513));
#235656=CARTESIAN_POINT('Ctrl Pts',(83.4134578873695,4.45640020159694,135.127052047582));
#235657=CARTESIAN_POINT('Ctrl Pts',(83.1350102635564,6.04559588764522,129.391585221682));
#235658=CARTESIAN_POINT('Ctrl Pts',(82.8565626397436,2.07918429672594,124.954389966684));
#235659=CARTESIAN_POINT('Ctrl Pts',(82.5781150159307,-3.79789608908488,
125.893031952893));
#235660=CARTESIAN_POINT('Ctrl Pts',(82.2996673921181,-6.18489550656524,
131.344945050191));
#235661=CARTESIAN_POINT('Ctrl Pts',(82.0212197683047,-2.88827810245507,
136.300087462925));
#235662=CARTESIAN_POINT('Ctrl Pts',(81.7427721444922,3.06252577758164,136.204925385956));
#235663=CARTESIAN_POINT('Ctrl Pts',(81.464324520679,6.19901808072266,131.146908119091));
#235664=CARTESIAN_POINT('Ctrl Pts',(81.1858768968663,3.6389156065486,125.774106432701));
#235665=CARTESIAN_POINT('Ctrl Pts',(80.9074292730533,-2.26517253913331,
125.023862600622));
#235666=CARTESIAN_POINT('Ctrl Pts',(80.6289816492404,-6.08767778118217,
129.585614053086));
#235667=CARTESIAN_POINT('Ctrl Pts',(80.3505340254275,-4.31590454191782,
135.267334059228));
#235668=CARTESIAN_POINT('Ctrl Pts',(80.0720864016147,1.42197412771073,136.847799500855));
#235669=CARTESIAN_POINT('Ctrl Pts',(79.7936387778018,5.85312804127117,132.874639847142));
#235670=CARTESIAN_POINT('Ctrl Pts',(79.5151911539889,4.90554322610457,126.998994720211));
#235671=CARTESIAN_POINT('Ctrl Pts',(79.236743530176,-0.54999616474248,124.62029495049));
#235672=CARTESIAN_POINT('Ctrl Pts',(78.9582959063631,-5.50011594899764,
127.924449420408));
#235673=CARTESIAN_POINT('Ctrl Pts',(78.6798482825503,-5.39589787172579,
133.87510158903));
#235674=CARTESIAN_POINT('Ctrl Pts',(78.4014006587372,-0.333113254603616,
137.003892818912));
#235675=CARTESIAN_POINT('Ctrl Pts',(78.1229530349246,5.035786170012,134.435616819741));
#235676=CARTESIAN_POINT('Ctrl Pts',(77.8445054111114,5.77704411621779,128.530393767498));
#235677=CARTESIAN_POINT('Ctrl Pts',(77.5660577872988,1.20948074391421,124.71483516101));
#235678=CARTESIAN_POINT('Ctrl Pts',(77.2876101634857,-4.46953634562727,
126.49525295924));
#235679=CARTESIAN_POINT('Ctrl Pts',(77.009162539673,-6.04126788252658,132.235530183857));
#235680=CARTESIAN_POINT('Ctrl Pts',(76.73071491586,-2.06136936772754,136.660632493573));
#235681=CARTESIAN_POINT('Ctrl Pts',(76.4522672920471,3.81282689252116,135.704107044024));
#235682=CARTESIAN_POINT('Ctrl Pts',(76.1738196682342,6.18322150549176,130.244953994479));
#235683=CARTESIAN_POINT('Ctrl Pts',(75.8953720444213,2.87153762207887,125.299868303017));
#235684=CARTESIAN_POINT('Ctrl Pts',(75.6169244206085,-3.07894905361277,
125.413142139227));
#235685=CARTESIAN_POINT('Ctrl Pts',(75.3384767967955,-6.20003196405775,
130.480682381363));
#235686=CARTESIAN_POINT('Ctrl Pts',(75.0600291729826,-3.62358838793365,
135.84566711001));
#235687=CARTESIAN_POINT('Ctrl Pts',(74.7815815491698,2.28275589456742,136.577937453613));
#235688=CARTESIAN_POINT('Ctrl Pts',(74.5031339253568,6.09135902878616,132.004572739798));
#235689=CARTESIAN_POINT('Ctrl Pts',(74.224686301544,4.30230079498258,126.328271719272));
#235690=CARTESIAN_POINT('Ctrl Pts',(73.946238677731,-1.44036169033171,124.76527772718));
#235691=CARTESIAN_POINT('Ctrl Pts',(73.6677910539182,-5.85940214781156,
128.75190588575));
#235692=CARTESIAN_POINT('Ctrl Pts',(73.3893434301052,-4.89393827916089,
134.624639674871));
#235693=CARTESIAN_POINT('Ctrl Pts',(73.1108958062924,0.56881578586215,136.986723641335));
#235694=CARTESIAN_POINT('Ctrl Pts',(72.8324481824796,5.50885593187395,133.66751801418));
#235695=CARTESIAN_POINT('Ctrl Pts',(72.5540005586665,5.38652659906729,127.717210612549));
#235696=CARTESIAN_POINT('Ctrl Pts',(72.2755529348538,0.314242468171368,
124.603843249867));
#235697=CARTESIAN_POINT('Ctrl Pts',(71.9971053110409,-5.04681513937595,
127.188448435987));
#235698=CARTESIAN_POINT('Ctrl Pts',(71.7186576872279,-5.77009618446306,
133.095900269846));
#235699=CARTESIAN_POINT('Ctrl Pts',(71.4402100634152,-1.19094072089807,
136.897539111196));
#235700=CARTESIAN_POINT('Ctrl Pts',(71.1617624396021,4.48263108448347,135.099844585217));
#235701=CARTESIAN_POINT('Ctrl Pts',(70.8833148157894,6.03688391192757,129.354810139024));
#235702=CARTESIAN_POINT('Ctrl Pts',(70.6048671919763,2.04353534248492,124.941841768133));
#235703=CARTESIAN_POINT('Ctrl Pts',(70.3264195681636,-3.82772237444985,
125.916241819903));
#235704=CARTESIAN_POINT('Ctrl Pts',(70.0479719443506,-6.18149022389895,
131.382584248845));
#235705=CARTESIAN_POINT('Ctrl Pts',(69.7695243205378,-2.85477054017052,
136.317567408437));
#235706=CARTESIAN_POINT('Ctrl Pts',(69.4910766967249,3.09534380668036,136.186182862342));
#235707=CARTESIAN_POINT('Ctrl Pts',(69.2126290729119,6.20098841114368,131.109166589932));
#235708=CARTESIAN_POINT('Ctrl Pts',(68.934181449099,3.60822760089105,125.752048519516));
#235709=CARTESIAN_POINT('Ctrl Pts',(68.6557338252862,-2.30031810286251,
125.037758448041));
#235710=CARTESIAN_POINT('Ctrl Pts',(68.3772862014732,-6.09498384687224,
129.622694056181));
#235711=CARTESIAN_POINT('Ctrl Pts',(68.0988385776604,-4.28865719212064,
135.293523506613));
#235712=CARTESIAN_POINT('Ctrl Pts',(67.8203909538475,1.45873590963839,136.83903156981));
#235713=CARTESIAN_POINT('Ctrl Pts',(67.5419433300346,5.86562197365073,132.83897183796));
#235714=CARTESIAN_POINT('Ctrl Pts',(67.2634957062218,4.88228799544191,126.969203790852));
#235715=CARTESIAN_POINT('Ctrl Pts',(66.9850480824087,-0.587630137549865,
124.623757509667));
#235716=CARTESIAN_POINT('Ctrl Pts',(66.706600458596,-5.51754488146136,127.957983545393));
#235717=CARTESIAN_POINT('Ctrl Pts',(66.428152834783,-5.37710542636232,133.907891057196));
#235718=CARTESIAN_POINT('Ctrl Pts',(66.1497052109702,-0.295368770640213,
137.00580571087));
#235719=CARTESIAN_POINT('Ctrl Pts',(65.8712575871573,5.05779735573374,134.404895281231));
#235720=CARTESIAN_POINT('Ctrl Pts',(65.5928099633443,5.76309479932555,128.495269391582));
#235721=CARTESIAN_POINT('Ctrl Pts',(65.3143623395316,1.17238966517029,124.707585533234));
#235722=CARTESIAN_POINT('Ctrl Pts',(65.0359147157185,-4.49568429685739,
126.522540133366));
#235723=CARTESIAN_POINT('Ctrl Pts',(64.7574670919057,-6.03244401646077,
132.272278579917));
#235724=CARTESIAN_POINT('Ctrl Pts',(64.4790194680927,-2.02568238621027,
136.673072130848));
#235725=CARTESIAN_POINT('Ctrl Pts',(64.20057184428,3.84258239688126,135.680806503568));
#235726=CARTESIAN_POINT('Ctrl Pts',(63.922124220467,6.17970167782515,130.207325334677));
#235727=CARTESIAN_POINT('Ctrl Pts',(63.6436765966542,2.8379770120581,125.282490423967));
#235728=CARTESIAN_POINT('Ctrl Pts',(63.3652289728412,-3.11170988490585,
125.431984462817));
#235729=CARTESIAN_POINT('Ctrl Pts',(63.0867813490283,-6.20188741312008,
130.518429732716));
#235730=CARTESIAN_POINT('Ctrl Pts',(62.8083337252156,-3.59283338772076,
135.86763151729));
#235731=CARTESIAN_POINT('Ctrl Pts',(62.5298861014024,2.31785900132509,136.563934699553));
#235732=CARTESIAN_POINT('Ctrl Pts',(62.2514384775899,6.09855220186056,131.967470671305));
#235733=CARTESIAN_POINT('Ctrl Pts',(61.9729908537767,4.27497385972414,126.302165324755));
#235734=CARTESIAN_POINT('Ctrl Pts',(61.6945432299639,-1.47709661541541,
124.774157507831));
#235735=CARTESIAN_POINT('Ctrl Pts',(61.416095606151,-5.87178746116934,128.787611756953));
#235736=CARTESIAN_POINT('Ctrl Pts',(61.1376479823382,-4.8705924828735,134.65435968532));
#235737=CARTESIAN_POINT('Ctrl Pts',(60.8592003585251,0.606439045512412,
136.983146553331));
#235738=CARTESIAN_POINT('Ctrl Pts',(60.5807527347125,5.52618271726667,133.633930996847));
#235739=CARTESIAN_POINT('Ctrl Pts',(60.3023051108993,5.36763444088732,127.684478494003));
#235740=CARTESIAN_POINT('Ctrl Pts',(60.0238574870866,0.276492336852797,
124.602045247997));
#235741=CARTESIAN_POINT('Ctrl Pts',(59.7454098632736,-5.06873271734795,
127.219236826675));
#235742=CARTESIAN_POINT('Ctrl Pts',(59.4669622394608,-5.75604002566515,
133.130982026147));
#235743=CARTESIAN_POINT('Ctrl Pts',(59.1885146156479,-1.15382774858414,
136.904675812908));
#235744=CARTESIAN_POINT('Ctrl Pts',(58.9100669918351,4.50869586182645,135.072477952114));
#235745=CARTESIAN_POINT('Ctrl Pts',(58.6316193680221,6.02794823725661,129.318088769994));
#235746=CARTESIAN_POINT('Ctrl Pts',(58.3531717442092,2.00781066429043,124.929510807376));
#235747=CARTESIAN_POINT('Ctrl Pts',(58.0747241203963,-3.85740682215468,
125.939632817953));
#235748=CARTESIAN_POINT('Ctrl Pts',(57.7962764965834,-6.17785588383907,
131.42020202121));
#235749=CARTESIAN_POINT('Ctrl Pts',(57.5178288727705,-2.82115719331391,
136.334843060042));
#235750=CARTESIAN_POINT('Ctrl Pts',(57.2393812489577,3.12804713667602,136.167240913326));
#235751=CARTESIAN_POINT('Ctrl Pts',(56.9609336251447,6.20272896165862,131.071413766074));
#235752=CARTESIAN_POINT('Ctrl Pts',(56.6824860013319,3.57740589103289,125.730177821614));
#235753=CARTESIAN_POINT('Ctrl Pts',(56.404038377519,-2.33537842745856,125.051867979023));
#235754=CARTESIAN_POINT('Ctrl Pts',(56.125590753706,-6.10206406069443,129.659817846364));
#235755=CARTESIAN_POINT('Ctrl Pts',(55.8471431298932,-4.26125092455389,
135.319546606417));
#235756=CARTESIAN_POINT('Ctrl Pts',(55.5686955060803,1.49544363757083,136.830040021814));
#235757=CARTESIAN_POINT('Ctrl Pts',(55.2902478822675,5.87789855325116,132.80322843551));
#235758=CARTESIAN_POINT('Ctrl Pts',(55.0118002584545,4.85885184980179,126.939554974638));
#235759=CARTESIAN_POINT('Ctrl Pts',(54.7333526346416,-0.625242335506623,
124.627449093364));
#235760=CARTESIAN_POINT('Ctrl Pts',(54.4549050108287,-5.53476935927053,
127.991623143927));
#235761=CARTESIAN_POINT('Ctrl Pts',(54.1764573870159,-5.35811373037978,
133.9405655229));
#235762=CARTESIAN_POINT('Ctrl Pts',(53.8980097632029,-0.257613341678002,
137.007488805997));
#235763=CARTESIAN_POINT('Ctrl Pts',(53.61956213939,5.07962112291461,134.374040323585));
#235764=CARTESIAN_POINT('Ctrl Pts',(53.3411145155772,5.74893192883615,128.460230579889));
#235765=CARTESIAN_POINT('Ctrl Pts',(53.0626668917642,1.13525514309568,124.7005618237));
#235766=CARTESIAN_POINT('Ctrl Pts',(52.7842192679514,-4.52166565885288,
126.549985971924));
#235767=CARTESIAN_POINT('Ctrl Pts',(52.5057716441385,-6.0233966159634,132.308972581737));
#235768=CARTESIAN_POINT('Ctrl Pts',(52.2273240203255,-1.98992034228702,
136.685294300858));
#235769=CARTESIAN_POINT('Ctrl Pts',(51.9488763965128,3.87219551293788,135.657325264614));
#235770=CARTESIAN_POINT('Ctrl Pts',(51.6704287726998,6.17595285904027,130.169718798237));
#235771=CARTESIAN_POINT('Ctrl Pts',(51.391981148887,2.80431123975502,125.265317159845));
#235772=CARTESIAN_POINT('Ctrl Pts',(51.113533525074,-3.14435541064497,125.451025861782));
#235773=CARTESIAN_POINT('Ctrl Pts',(50.8350859012611,-6.20351304896362,
130.556187679343));
#235774=CARTESIAN_POINT('Ctrl Pts',(50.5566382774483,-3.5619452537452,135.889408303207));
#235775=CARTESIAN_POINT('Ctrl Pts',(50.2781906536353,2.35287621896542,136.549718522358));
#235776=CARTESIAN_POINT('Ctrl Pts',(49.9997430298226,6.10551939084041,131.930325503341));
#235777=CARTESIAN_POINT('Ctrl Pts',(49.7212954060095,4.2474885137371,126.27622576074));
#235778=CARTESIAN_POINT('Ctrl Pts',(49.4428477821967,-1.51377680614101,
124.783260739875));
#235779=CARTESIAN_POINT('Ctrl Pts',(49.1644001583838,-5.88395519328364,
128.823392359526));
#235780=CARTESIAN_POINT('Ctrl Pts',(48.8859525345709,-4.84706620499019,
134.683937032636));
#235781=CARTESIAN_POINT('Ctrl Pts',(48.607504910758,0.644039833341117,136.97934050814));
#235782=CARTESIAN_POINT('Ctrl Pts',(48.3290572869451,5.54330472792681,133.600239128744));
#235783=CARTESIAN_POINT('Ctrl Pts',(48.0506096631323,5.34854338303893,127.651861983834));
#235784=CARTESIAN_POINT('Ctrl Pts',(47.7721620393193,0.23873196000854,124.600477075203));
#235785=CARTESIAN_POINT('Ctrl Pts',(47.4937144155065,-5.09046247156518,
127.250158065443));
#235786=CARTESIAN_POINT('Ctrl Pts',(47.2152667916935,-5.74177057468722,
133.165977568637));
#235787=CARTESIAN_POINT('Ctrl Pts',(46.9368191678807,-1.11667202075834,
136.911586465198));
#235788=CARTESIAN_POINT('Ctrl Pts',(46.6583715440677,4.53459356778643,135.044953162355));
#235789=CARTESIAN_POINT('Ctrl Pts',(46.379923920255,6.01878919474683,129.281422475313));
#235790=CARTESIAN_POINT('Ctrl Pts',(46.101476296442,1.97201158593325,124.917397541337));
#235791=CARTESIAN_POINT('Ctrl Pts',(45.8230286726291,-3.88694833223118,
125.963204080281));
#235792=CARTESIAN_POINT('Ctrl Pts',(45.5445810488162,-6.17399262105761,
131.457796973343));
#235793=CARTESIAN_POINT('Ctrl Pts',(45.2661334250033,-2.78743930743976,
136.351913777587));
#235794=CARTESIAN_POINT('Ctrl Pts',(44.9876858011905,3.16063455573481,136.148100240809));
#235795=CARTESIAN_POINT('Ctrl Pts',(44.7092381773775,6.20423966777097,131.033651046464));
#235796=CARTESIAN_POINT('Ctrl Pts',(44.4307905535647,3.54645161908363,125.708495149421));
#235797=CARTESIAN_POINT('Ctrl Pts',(44.1523429297517,-2.37035221374829,
125.066190670735));
#235798=CARTESIAN_POINT('Ctrl Pts',(43.8738953059389,-6.10891816028884,
129.696984048001));
#235799=CARTESIAN_POINT('Ctrl Pts',(43.5954476821259,-4.23368675476706,
135.345402394343));
#235800=CARTESIAN_POINT('Ctrl Pts',(43.3170000583131,1.53209595128933,136.820825190051));
#235801=CARTESIAN_POINT('Ctrl Pts',(43.0385524345002,5.88995732515911,132.767410964279));
#235802=CARTESIAN_POINT('Ctrl Pts',(42.7601048106873,4.83523565761953,126.910049370218));
#235803=CARTESIAN_POINT('Ctrl Pts',(42.4816571868744,-0.662831364878718,
124.631369564788));
#235804=CARTESIAN_POINT('Ctrl Pts',(42.2032095630615,-5.55178874416567,
128.025366969483));
#235805=CARTESIAN_POINT('Ctrl Pts',(41.9247619392486,-5.33892348752252,
133.973123775378));
#235806=CARTESIAN_POINT('Ctrl Pts',(41.6463143154357,-0.219848366758665,
137.008942041929));
#235807=CARTESIAN_POINT('Ctrl Pts',(41.3678666916229,5.10125666286673,134.343053090145));
#235808=CARTESIAN_POINT('Ctrl Pts',(41.0894190678099,5.73455602955998,128.425278630796));
#235809=CARTESIAN_POINT('Ctrl Pts',(40.8109714439971,1.09807855372398,124.693764292674));
#235810=CARTESIAN_POINT('Ctrl Pts',(40.5325238201841,-4.5474794688646,126.5775894579));
#235811=CARTESIAN_POINT('Ctrl Pts',(40.2540761963713,-6.01412601628932,
132.345610829607));
#235812=CARTESIAN_POINT('Ctrl Pts',(39.9756285725584,-1.95408456113369,
136.697298550707));
#235813=CARTESIAN_POINT('Ctrl Pts',(39.6971809487455,3.90166514336576,135.633664197272));
#235814=CARTESIAN_POINT('Ctrl Pts',(39.4187333249326,6.171975188051,130.132135778682));
#235815=CARTESIAN_POINT('Ctrl Pts',(39.1402857011198,2.77054155266769,125.248349147017));
#235816=CARTESIAN_POINT('Ctrl Pts',(38.8618380773068,-3.17688442113803,
125.470265630536));
#235817=CARTESIAN_POINT('Ctrl Pts',(38.583390453494,-6.20490881134979,130.593954822108));
#235818=CARTESIAN_POINT('Ctrl Pts',(38.304942829681,-3.53092513057837,135.910996660811));
#235819=CARTESIAN_POINT('Ctrl Pts',(38.0264952058682,2.38780624991219,136.535289448812));
#235820=CARTESIAN_POINT('Ctrl Pts',(37.7480475820552,6.11226033755391,131.893138612335));
#235821=CARTESIAN_POINT('Ctrl Pts',(37.4695999582424,4.21984577550119,126.250453988427));
#235822=CARTESIAN_POINT('Ctrl Pts',(37.1911523344295,-1.55040090331038,
124.792587085991));
#235823=CARTESIAN_POINT('Ctrl Pts',(36.9127047106166,-5.89590489327443,
128.859246367608));
#235824=CARTESIAN_POINT('Ctrl Pts',(36.6342570868037,-4.82336031728617,
134.713370620821));
#235825=CARTESIAN_POINT('Ctrl Pts',(36.3558094629908,0.681616756036961,
136.975305646799));
#235826=CARTESIAN_POINT('Ctrl Pts',(36.0773618391779,5.56022132939171,133.566443658335));
#235827=CARTESIAN_POINT('Ctrl Pts',(35.798914215365,5.32925413294858,127.619362290662));
#235828=CARTESIAN_POINT('Ctrl Pts',(35.5204665915522,0.200962736863706,
124.599138789596));
#235829=CARTESIAN_POINT('Ctrl Pts',(35.2420189677392,-5.11200359682353,
127.281211006494));
#235830=CARTESIAN_POINT('Ctrl Pts',(34.9635713439263,-5.72728836028912,
133.200885600541));
#235831=CARTESIAN_POINT('Ctrl Pts',(34.6851237201134,-1.07947491424015,
136.918270811987));
#235832=CARTESIAN_POINT('Ctrl Pts',(34.4066760963006,4.56032324271418,135.017271235878));
#235833=CARTESIAN_POINT('Ctrl Pts',(34.1282284724876,6.00940712379002,129.244812613665));
#235834=CARTESIAN_POINT('Ctrl Pts',(33.8497808486748,1.93613943396156,124.905502418881));
#235835=CARTESIAN_POINT('Ctrl Pts',(33.5713332248619,-3.91634581000783,
125.986954733445));
#235836=CARTESIAN_POINT('Ctrl Pts',(33.292885601049,-6.16990057870911,131.495367712155));
#235837=CARTESIAN_POINT('Ctrl Pts',(33.0144379772361,-2.753618131977,136.368778928511));
#235838=CARTESIAN_POINT('Ctrl Pts',(32.7359903534233,3.19310485631782,136.128761554055));
#235839=CARTESIAN_POINT('Ctrl Pts',(32.4575427296103,6.20552047350092,130.995879830412));
#235840=CARTESIAN_POINT('Ctrl Pts',(32.1790951057975,3.51536593206519,125.687001306397));
#235841=CARTESIAN_POINT('Ctrl Pts',(31.9006474819845,-2.40523816576522,
125.080725992446));
#235842=CARTESIAN_POINT('Ctrl Pts',(31.6221998581717,-6.11554589167424,
129.734191283883));
#235843=CARTESIAN_POINT('Ctrl Pts',(31.3437522343588,-4.20596570416061,
135.371089912296));
#235844=CARTESIAN_POINT('Ctrl Pts',(31.0653046105458,1.56869149262894,136.811387415981));
#235845=CARTESIAN_POINT('Ctrl Pts',(30.786856986733,5.90179784253235,132.731520751495));
#235846=CARTESIAN_POINT('Ctrl Pts',(30.5084093629201,4.81144029400183,126.880688070935));
#235847=CARTESIAN_POINT('Ctrl Pts',(30.2299617391072,-0.700395832790832,
124.635518778667));
#235848=CARTESIAN_POINT('Ctrl Pts',(29.9515141152943,-5.56860240548724,
128.05921377167));
#235849=CARTESIAN_POINT('Ctrl Pts',(29.6730664914815,-5.31953540889204,
134.005564608172));
#235850=CARTESIAN_POINT('Ctrl Pts',(29.3946188676685,-0.182075245277261,
137.010165364815));
#235851=CARTESIAN_POINT('Ctrl Pts',(29.1161712438556,5.12270317387725,134.311934729152));
#235852=CARTESIAN_POINT('Ctrl Pts',(28.8377236200427,5.71996763420123,128.390414839463));
#235853=CARTESIAN_POINT('Ctrl Pts',(28.5592759962298,1.06086127464794,124.687193192043));
#235854=CARTESIAN_POINT('Ctrl Pts',(28.280828372417,-4.57312477035222,126.605349568435));
#235855=CARTESIAN_POINT('Ctrl Pts',(28.0023807486041,-6.00463256096402,
132.382191965885));
#235856=CARTESIAN_POINT('Ctrl Pts',(27.7239331247912,-1.91817637065835,
136.709084435575));
#235857=CARTESIAN_POINT('Ctrl Pts',(27.4454855009783,3.93099019615694,135.60982417831));
#235858=CARTESIAN_POINT('Ctrl Pts',(27.1670378771654,6.16776881225138,130.094577668667));
#235859=CARTESIAN_POINT('Ctrl Pts',(26.8885902533525,2.73666920214424,125.231587014236));
#235860=CARTESIAN_POINT('Ctrl Pts',(26.6101426295396,-3.20929571101057,
125.48970305614));
#235861=CARTESIAN_POINT('Ctrl Pts',(26.3316950057267,-6.2060746485581,130.631729761538));
#235862=CARTESIAN_POINT('Ctrl Pts',(26.0532473819138,-3.49977416768234,
135.932395790139));
#235863=CARTESIAN_POINT('Ctrl Pts',(25.774799758101,2.42264779982026,136.52064801359));
#235864=CARTESIAN_POINT('Ctrl Pts',(25.4963521342881,6.11877479221284,131.85591137626));
#235865=CARTESIAN_POINT('Ctrl Pts',(25.2179045104751,4.19204666932822,126.224850962798));
#235866=CARTESIAN_POINT('Ctrl Pts',(24.9394568866623,-1.58696754980412,
124.802136200585));
#235867=CARTESIAN_POINT('Ctrl Pts',(24.6610092628494,-5.90763611834117,
128.895172452612));
#235868=CARTESIAN_POINT('Ctrl Pts',(24.3825616390365,-4.79947569819179,
134.742659359205));
#235869=CARTESIAN_POINT('Ctrl Pts',(24.1041140152236,0.719168421173241,
136.97104211882));
#235870=CARTESIAN_POINT('Ctrl Pts',(23.8256663914108,5.57693189481048,133.532545837923));
#235871=CARTESIAN_POINT('Ctrl Pts',(23.5472187675978,5.3097674053865,127.586980618775));
#235872=CARTESIAN_POINT('Ctrl Pts',(23.2687711437849,0.163186066970757,
124.598030440764));
#235873=CARTESIAN_POINT('Ctrl Pts',(22.990323519972,-5.13335529490864,127.312394499151));
#235874=CARTESIAN_POINT('Ctrl Pts',(22.7118758961592,-5.71259391911463,
133.235704828331));
#235875=CARTESIAN_POINT('Ctrl Pts',(22.4334282723462,-1.04223780738205,
136.924728605587));
#235876=CARTESIAN_POINT('Ctrl Pts',(22.1549806485334,4.58588393318709,134.98943319845));
#235877=CARTESIAN_POINT('Ctrl Pts',(21.8765330247205,5.9998023720423,129.208260541641));
#235878=CARTESIAN_POINT('Ctrl Pts',(21.5980854009075,1.90019553763114,124.893825880784));
#235879=CARTESIAN_POINT('Ctrl Pts',(21.3196377770947,-3.94559816615024,
126.010883897355));
#235880=CARTESIAN_POINT('Ctrl Pts',(21.0411901532818,-6.16557990842568,
131.532912845442));
#235881=CARTESIAN_POINT('Ctrl Pts',(20.7627425294689,-2.71969492018171,
136.385437887866));
#235882=CARTESIAN_POINT('Ctrl Pts',(20.484294905656,3.22545683522612,136.109225569666));
#235883=CARTESIAN_POINT('Ctrl Pts',(20.2058472818431,6.20657133138755,130.958101517545));
#235884=CARTESIAN_POINT('Ctrl Pts',(19.9273996580302,3.48414998186958,125.665697089004));
#235885=CARTESIAN_POINT('Ctrl Pts',(19.6489520342174,-2.44003499079723,
125.095473405541));
#235886=CARTESIAN_POINT('Ctrl Pts',(19.3705044104044,-6.12194700925765,
129.771438175283));
#235887=CARTESIAN_POINT('Ctrl Pts',(19.0920567865916,-4.17808879994825,
135.396608208416));
#235888=CARTESIAN_POINT('Ctrl Pts',(18.8136091627787,1.60522890552839,136.801727049323));
#235889=CARTESIAN_POINT('Ctrl Pts',(18.5351615389658,5.91341966661616,132.695559127084));
#235890=CARTESIAN_POINT('Ctrl Pts',(18.2567139151529,4.78746664069464,126.85147216478));
#235891=CARTESIAN_POINT('Ctrl Pts',(17.97826629134,-0.737934347277788,124.63989658125));
#235892=CARTESIAN_POINT('Ctrl Pts',(17.6998186675271,-5.58520972019883,
128.093162296283));
#235893=CARTESIAN_POINT('Ctrl Pts',(17.4213710437142,-5.29995021292075,
134.037886819174));
#235894=CARTESIAN_POINT('Ctrl Pts',(17.1429234199013,-0.144295376930669,
137.011158729324));
#235895=CARTESIAN_POINT('Ctrl Pts',(16.8644757960885,5.14395986123776,134.280686393713));
#235896=CARTESIAN_POINT('Ctrl Pts',(16.5860281722755,5.70516728333829,128.355640497777));
#235897=CARTESIAN_POINT('Ctrl Pts',(16.3075805484627,1.02360468496723,124.6808487653));
#235898=CARTESIAN_POINT('Ctrl Pts',(16.0291329246498,-4.5986006130197,126.633265274869));
#235899=CARTESIAN_POINT('Ctrl Pts',(15.7506853008369,-5.99491660177097,
132.418714635041));
#235900=CARTESIAN_POINT('Ctrl Pts',(15.472237677024,-1.88219710145218,136.720651518731));
#235901=CARTESIAN_POINT('Ctrl Pts',(15.1937900532111,3.96016958466077,135.585806091128));
#235902=CARTESIAN_POINT('Ctrl Pts',(14.9153424293982,6.16333388751023,130.057045859918));
#235903=CARTESIAN_POINT('Ctrl Pts',(14.6368948055853,2.70269544333712,125.215031382631));
#235904=CARTESIAN_POINT('Ctrl Pts',(14.3584471817724,-3.24158807925031,
125.509337418335));
#235905=CARTESIAN_POINT('Ctrl Pts',(14.0799995579596,-6.20701051738803,
130.669511097867));
#235906=CARTESIAN_POINT('Ctrl Pts',(13.8015519341466,-3.46849351936748,
135.953604898237));
#235907=CARTESIAN_POINT('Ctrl Pts',(13.5231043103337,2.45739957762318,136.505794759238));
#235908=CARTESIAN_POINT('Ctrl Pts',(13.2446566865208,6.12506251342167,131.818645174584));
#235909=CARTESIAN_POINT('Ctrl Pts',(12.966209062708,4.16409222532429,126.199417632585));
#235910=CARTESIAN_POINT('Ctrl Pts',(12.687761438895,-1.62347539063169,124.811907729812));
#235911=CARTESIAN_POINT('Ctrl Pts',(12.4093138150822,-5.91914843377905,
128.931169283287));
#235912=CARTESIAN_POINT('Ctrl Pts',(12.1308661912693,-4.77541323276041,
134.771802162479));
#235913=CARTESIAN_POINT('Ctrl Pts',(11.8524185674564,0.756693437259193,
136.96655008219));
#235914=CARTESIAN_POINT('Ctrl Pts',(11.5739709436435,5.59343580496719,133.498546923603));
#235915=CARTESIAN_POINT('Ctrl Pts',(11.2955233198306,5.2900839224404,127.554718168085));
#235916=CARTESIAN_POINT('Ctrl Pts',(11.0170756960177,0.125403350157864,
124.597152069781));
#235917=CARTESIAN_POINT('Ctrl Pts',(10.7386280722048,-5.15451677462551,
127.343707387895));
#235918=CARTESIAN_POINT('Ctrl Pts',(10.460180448392,-5.69768779567166,133.270433961767));
#235919=CARTESIAN_POINT('Ctrl Pts',(10.1817328245791,-1.0049620800187,136.930959606699));
#235920=CARTESIAN_POINT('Ctrl Pts',(9.90328520076621,4.61127469204443,134.961440081617));
#235921=CARTESIAN_POINT('Ctrl Pts',(9.62483757695328,5.98997529541125,129.171767613693));
#235922=CARTESIAN_POINT('Ctrl Pts',(9.34638995314043,1.86418122885626,124.882368359726));
#235923=CARTESIAN_POINT('Ctrl Pts',(9.0679423293275,-3.97470431670162,126.034990685308));
#235924=CARTESIAN_POINT('Ctrl Pts',(8.78949470551463,-6.16103077031137,
131.57043098196));
#235925=CARTESIAN_POINT('Ctrl Pts',(8.5110470817017,-2.68567092909101,136.401890038352));
#235926=CARTESIAN_POINT('Ctrl Pts',(8.2325994578889,3.25768929364524,136.089493011555));
#235927=CARTESIAN_POINT('Ctrl Pts',(7.95415183407592,6.20739220249103,130.920317507753));
#235928=CARTESIAN_POINT('Ctrl Pts',(7.67570421026306,3.45280492521512,125.644583286679));
#235929=CARTESIAN_POINT('Ctrl Pts',(7.39725658645018,-2.47474139943534,
125.110432363552));
#235930=CARTESIAN_POINT('Ctrl Pts',(7.11880896263729,-6.1281212758433,129.808723342005));
#235931=CARTESIAN_POINT('Ctrl Pts',(6.84036133882437,-4.15005707511893,
135.421956337113));
#235932=CARTESIAN_POINT('Ctrl Pts',(6.56191371501151,1.64170683608044,136.791844448048));
#235933=CARTESIAN_POINT('Ctrl Pts',(6.28346609119863,5.92482236675955,132.659527423617));
#235934=CARTESIAN_POINT('Ctrl Pts',(6.00501846738572,4.76331558605049,126.822402734361));
#235935=CARTESIAN_POINT('Ctrl Pts',(5.72657084357281,-0.775445517336138,
124.644502810313));
#235936=CARTESIAN_POINT('Ctrl Pts',(5.44812321975995,-5.60161007291028,
128.127211285347));
#235937=CARTESIAN_POINT('Ctrl Pts',(5.16967559594705,-5.28016862534525,
134.070089210674));
#235938=CARTESIAN_POINT('Ctrl Pts',(4.89122797213414,-0.106510161665837,
137.011922098645));
#235939=CARTESIAN_POINT('Ctrl Pts',(4.6127803483213,5.16502593727395,134.249309241742));
#235940=CARTESIAN_POINT('Ctrl Pts',(4.33433272450837,5.69015552540359,128.320956894316));
#235941=CARTESIAN_POINT('Ctrl Pts',(4.05588510069549,0.986310165238503,
124.674731247541));
#235942=CARTESIAN_POINT('Ctrl Pts',(3.77743747688256,-4.62390605285035,
126.661335542776));
#235943=CARTESIAN_POINT('Ctrl Pts',(3.49898985306972,-5.98497849873861,
132.455177483715));
#235944=CARTESIAN_POINT('Ctrl Pts',(3.22054222925682,-1.84614808674025,
136.731999371551));
#235945=CARTESIAN_POINT('Ctrl Pts',(2.94209460544391,3.9892022276243,135.561610825727));
#235946=CARTESIAN_POINT('Ctrl Pts',(2.66364698163102,6.15867057816533,130.019541743194));
#235947=CARTESIAN_POINT('Ctrl Pts',(2.38519935781816,2.66862153515642,125.198682865676));
#235948=CARTESIAN_POINT('Ctrl Pts',(2.10675173400524,-3.27376032925169,
125.529167989562));
#235949=CARTESIAN_POINT('Ctrl Pts',(1.82830411019233,-6.20771638316062,
130.707297431096));
#235950=CARTESIAN_POINT('Ctrl Pts',(1.54985648637947,-3.43708434474973,
135.974623199195));
#235951=CARTESIAN_POINT('Ctrl Pts',(1.27140886256659,2.49206029558105,136.490730236146));
#235952=CARTESIAN_POINT('Ctrl Pts',(0.992961238753657,6.13112326818657,
131.78134138822));
#235953=CARTESIAN_POINT('Ctrl Pts',(0.714513614940807,4.13598347935162,
126.174154940227));
#235954=CARTESIAN_POINT('Ctrl Pts',(0.436065991127901,-1.65992307298164,
124.821901311585));
#235955=CARTESIAN_POINT('Ctrl Pts',(0.157618367314999,-5.93044141299494,
128.967235525755));
#235956=CARTESIAN_POINT('Ctrl Pts',(-0.120829256497892,-4.75117381263555,
134.800797950748));
#235957=CARTESIAN_POINT('Ctrl Pts',(-0.399276880310752,0.794190413791566,
136.961829703365));
#235958=CARTESIAN_POINT('Ctrl Pts',(-0.67772450412367,5.60973244830296,
133.464448175219));
#235959=CARTESIAN_POINT('Ctrl Pts',(-0.956172127936585,5.27020441348929,
127.522576134092));
#235960=CARTESIAN_POINT('Ctrl Pts',(-1.23461975174943,0.0876159864779326,
124.596503709192));
#235961=CARTESIAN_POINT('Ctrl Pts',(-1.51306737556233,-5.17548725182775,
127.375148512417));
#235962=CARTESIAN_POINT('Ctrl Pts',(-1.79151499937523,-5.6825705423121,
133.305071713949));
#235963=CARTESIAN_POINT('Ctrl Pts',(-2.06996262318813,-0.967649113415911,
136.936963584433));
#235964=CARTESIAN_POINT('Ctrl Pts',(-2.34841024700098,4.63649457842225,
134.933292922676));
#235965=CARTESIAN_POINT('Ctrl Pts',(-2.62685787081389,5.97992625804282,
129.13533518208));
#235966=CARTESIAN_POINT('Ctrl Pts',(-2.90530549462681,1.82809784216042,
124.871130280269));
#235967=CARTESIAN_POINT('Ctrl Pts',(-3.18375311843967,-4.00366318312286,
126.059274204017));
#235968=CARTESIAN_POINT('Ctrl Pts',(-3.46220074225256,-6.15625333293613,
131.607920731459));
#235969=CARTESIAN_POINT('Ctrl Pts',(-3.74064836606547,-2.65154741947636,
136.418134770325));
#235970=CARTESIAN_POINT('Ctrl Pts',(-4.01909598987837,3.28980103718956,
136.06956461092));
#235971=CARTESIAN_POINT('Ctrl Pts',(-4.29754361369122,6.20798305639367,
130.882529201136));
#235972=CARTESIAN_POINT('Ctrl Pts',(-4.57599123750414,3.42133192360438,
125.623660681799));
#235973=CARTESIAN_POINT('Ctrl Pts',(-4.85443886131705,-2.5093561056208,
125.125602312169));
#235974=CARTESIAN_POINT('Ctrl Pts',(-5.13288648512991,-6.13406846264146,
129.846045402432));
#235975=CARTESIAN_POINT('Ctrl Pts',(-5.41133410894279,-4.12187156839848,
135.447133359102));
#235976=CARTESIAN_POINT('Ctrl Pts',(-5.68978173275571,1.67812393258193,
136.781739978358));
#235977=CARTESIAN_POINT('Ctrl Pts',(-5.9682293565686,5.93600552043131,132.623426976261));
#235978=CARTESIAN_POINT('Ctrl Pts',(-6.24667698038146,4.73898802499559,
126.793480856855));
#235979=CARTESIAN_POINT('Ctrl Pts',(-6.52512460419438,-0.812927952975666,
124.649337295173));
#235980=CARTESIAN_POINT('Ctrl Pts',(-6.80357222800728,-5.61780285590049,
128.161359477164));
#235981=CARTESIAN_POINT('Ctrl Pts',(-7.08201985182013,-5.26019137917956,
134.1021705894));
#235982=CARTESIAN_POINT('Ctrl Pts',(-7.36046747563304,-0.0687209996277829,
137.012455444495));
#235983=CARTESIAN_POINT('Ctrl Pts',(-7.63891509944595,5.18590062137458,
134.217804435933));
#235984=CARTESIAN_POINT('Ctrl Pts',(-7.91736272325884,5.67493291666336,
128.286365314294));
#235985=CARTESIAN_POINT('Ctrl Pts',(-8.1958103470717,0.948979097423875,
124.668840865451));
#235986=CARTESIAN_POINT('Ctrl Pts',(-8.47425797088461,-4.64904015214177,
126.689559331999));
#235987=CARTESIAN_POINT('Ctrl Pts',(-8.75270559469752,-5.97481862012702,
132.491579160764));
#235988=CARTESIAN_POINT('Ctrl Pts',(-9.03115321851038,-1.81003066233205,
136.743127573537));
#235989=CARTESIAN_POINT('Ctrl Pts',(-9.30960084232328,4.0180870492325,135.537239278668));
#235990=CARTESIAN_POINT('Ctrl Pts',(-9.58804846613619,6.15377905701727,
129.982066708221));
#235991=CARTESIAN_POINT('Ctrl Pts',(-9.86649608994908,2.63444874022312,
125.182542069172));
#235992=CARTESIAN_POINT('Ctrl Pts',(-10.144943713762,-3.30581126886015,
125.549194034992));
#235993=CARTESIAN_POINT('Ctrl Pts',(-10.4233913375749,-6.20819221971975,
130.745087361036));
#235994=CARTESIAN_POINT('Ctrl Pts',(-10.7018389613878,-3.40554780770759,
135.995449914173));
#235995=CARTESIAN_POINT('Ctrl Pts',(-10.9802865852006,2.52662866932821,
136.475455002538));
#235996=CARTESIAN_POINT('Ctrl Pts',(-11.2587342090136,6.13695683192405,
131.744001399476));
#235997=CARTESIAN_POINT('Ctrl Pts',(-11.5371818328265,4.10772147299012,
126.149063821843));
#235998=CARTESIAN_POINT('Ctrl Pts',(-11.8156294566394,-1.69630924627168,
124.832116575588));
#235999=CARTESIAN_POINT('Ctrl Pts',(-12.0940770804522,-5.94151463752335,
129.003369843568));
#236000=CARTESIAN_POINT('Ctrl Pts',(-12.3725247042651,-4.72675833601782,
134.829645649562));
#236001=CARTESIAN_POINT('Ctrl Pts',(-12.6509723280781,0.83165796130609,
136.956881157257));
#236002=CARTESIAN_POINT('Ctrl Pts',(-12.9294199518909,5.62582122093989,
133.430250856313));
#236003=CARTESIAN_POINT('Ctrl Pts',(-13.2078675757038,5.25012961517551,
127.490555707831));
#236004=CARTESIAN_POINT('Ctrl Pts',(-13.4863151995167,0.0498253761554086,
124.596085383024));
#236005=CARTESIAN_POINT('Ctrl Pts',(-13.7647628233296,-5.19626594944658,
127.406716707655));
#236006=CARTESIAN_POINT('Ctrl Pts',(-14.0432104471424,-5.66724271921134,
133.339616801361));
#236007=CARTESIAN_POINT('Ctrl Pts',(-14.3216580709554,-0.930300290219375,
136.942740316309));
#236008=CARTESIAN_POINT('Ctrl Pts',(-14.6001056947683,4.6615426577884,134.904992764631));
#236009=CARTESIAN_POINT('Ctrl Pts',(-14.8785533185811,5.96965563230779,
129.098964596818));
#236010=CARTESIAN_POINT('Ctrl Pts',(-15.157000942394,1.79194671462675,124.860112058844));
#236011=CARTESIAN_POINT('Ctrl Pts',(-15.4354485662069,-4.03247369233249,
126.08373355365));
#236012=CARTESIAN_POINT('Ctrl Pts',(-15.7138961900198,-6.15124777332969,
131.645380704742));
#236013=CARTESIAN_POINT('Ctrl Pts',(-15.9923438138327,-2.61732565579698,
136.434171481834));
#236014=CARTESIAN_POINT('Ctrl Pts',(-16.2707914376456,3.32179087594663,
136.049441106215));
#236015=CARTESIAN_POINT('Ctrl Pts',(-16.5492390614585,6.2083438712012,130.844737997954));
#236016=CARTESIAN_POINT('Ctrl Pts',(-16.8276866852714,3.38973214328102,
125.602930049661));
#236017=CARTESIAN_POINT('Ctrl Pts',(-17.1061343090842,-2.54387782669295,
125.140982689263));
#236018=CARTESIAN_POINT('Ctrl Pts',(-17.3845819328972,-6.13978834927694,
129.883402973582));
#236019=CARTESIAN_POINT('Ctrl Pts',(-17.66302955671,-4.09353332421128,135.47213834144));
#236020=CARTESIAN_POINT('Ctrl Pts',(-17.9414771805229,1.71447884558397,
136.771414014676));
#236021=CARTESIAN_POINT('Ctrl Pts',(-18.2199248043358,5.94696871323555,
132.587259122732));
#236022=CARTESIAN_POINT('Ctrl Pts',(-18.4983724281487,4.71448485899666,
126.764707603974));
#236023=CARTESIAN_POINT('Ctrl Pts',(-18.7768200519616,-0.850380265270943,
124.654399856686));
#236024=CARTESIAN_POINT('Ctrl Pts',(-19.0552676757745,-5.63378746913994,
128.19560560636));
#236025=CARTESIAN_POINT('Ctrl Pts',(-19.3337152995874,-5.24001921468789,
134.134129766565));
#236026=CARTESIAN_POINT('Ctrl Pts',(-19.6121629234003,-0.0309292911078312,
137.012758747106));
#236027=CARTESIAN_POINT('Ctrl Pts',(-19.8906105472132,5.2065831400206,134.18617314371));
#236028=CARTESIAN_POINT('Ctrl Pts',(-20.1690581710261,5.65950002119693,
128.251867039513));
#236029=CARTESIAN_POINT('Ctrl Pts',(-20.447505794839,0.911612864839816,
124.663177837304));
#236030=CARTESIAN_POINT('Ctrl Pts',(-20.7259534186518,-4.67400197954067,
126.717935596697));
#236031=CARTESIAN_POINT('Ctrl Pts',(-21.0044010424647,-5.96443734241423,
132.527918317308));
#236032=CARTESIAN_POINT('Ctrl Pts',(-21.2828486662776,-1.77384616657202,
136.754035712331));
#236033=CARTESIAN_POINT('Ctrl Pts',(-21.5612962900905,4.0468229791472,135.512692353051));
#236034=CARTESIAN_POINT('Ctrl Pts',(-21.8397439139034,6.14865950532324,
129.944622143653));
#236035=CARTESIAN_POINT('Ctrl Pts',(-22.1181915377163,2.60017832482316,
125.166609591221));
#236036=CARTESIAN_POINT('Ctrl Pts',(-22.3966391615293,-3.33773971041633,
125.569414812551));
#236037=CARTESIAN_POINT('Ctrl Pts',(-22.6750867853421,-6.20843800943312,
130.782879487369));
#236038=CARTESIAN_POINT('Ctrl Pts',(-22.953534409155,-3.37388507683905,
136.016084271426));
#236039=CARTESIAN_POINT('Ctrl Pts',(-23.2319820329679,2.56110341792085,
136.45996962444));
#236040=CARTESIAN_POINT('Ctrl Pts',(-23.5104296567807,6.14256298846929,
131.706626591997));
#236041=CARTESIAN_POINT('Ctrl Pts',(-23.7888772805937,4.07930725349882,
126.124145207193));
#236042=CARTESIAN_POINT('Ctrl Pts',(-24.0673249044065,-1.73263256219878,
124.842553143289));
#236043=CARTESIAN_POINT('Ctrl Pts',(-24.3457725282195,-5.95236769704188,
129.039570897758));
#236044=CARTESIAN_POINT('Ctrl Pts',(-24.6242201520323,-4.70216770763169,
134.858344189959));
#236045=CARTESIAN_POINT('Ctrl Pts',(-24.9026677758452,0.86909469142902,
136.951704627238));
#236046=CARTESIAN_POINT('Ctrl Pts',(-25.1811153996581,5.64170152670257,
133.395956234079));
#236047=CARTESIAN_POINT('Ctrl Pts',(-25.459563023471,5.22986027137813,127.458658075828));
#236048=CARTESIAN_POINT('Ctrl Pts',(-25.7380106472839,0.0120329195352371,
124.595897106778));
#236049=CARTESIAN_POINT('Ctrl Pts',(-26.0164582710968,-5.21685209751974,
127.438410803838));
#236050=CARTESIAN_POINT('Ctrl Pts',(-26.2949058949097,-5.6517048943475,
133.374067943923));
#236051=CARTESIAN_POINT('Ctrl Pts',(-26.5733535187226,-0.892916994403456,
136.948289588268));
#236052=CARTESIAN_POINT('Ctrl Pts',(-26.8518011425354,4.68641800197708,
134.876540656153));
#236053=CARTESIAN_POINT('Ctrl Pts',(-27.1302487663484,5.95916379878798,
129.062657205632));
#236054=CARTESIAN_POINT('Ctrl Pts',(-27.4086963901612,1.75572918584856,
124.849314103734));
#236055=CARTESIAN_POINT('Ctrl Pts',(-27.6871440139742,-4.06113477674652,
126.108367827853));
#236056=CARTESIAN_POINT('Ctrl Pts',(-27.965591637787,-6.1460142769749,131.682809513716));
#236057=CARTESIAN_POINT('Ctrl Pts',(-28.2440392616,-2.5830069061529,136.449999578631));
#236058=CARTESIAN_POINT('Ctrl Pts',(-28.5224868854127,3.3536576245212,136.029123243122));
#236059=CARTESIAN_POINT('Ctrl Pts',(-28.8009345092257,6.20847463354345,
130.806945298572));
#236060=CARTESIAN_POINT('Ctrl Pts',(-29.0793821330386,3.35800675518651,
125.582392158445));
#236061=CARTESIAN_POINT('Ctrl Pts',(-29.3578297568515,-2.57830528343674,
125.156572924908));
#236062=CARTESIAN_POINT('Ctrl Pts',(-29.6362773806644,-6.14528072379723,
129.920794671155));
#236063=CARTESIAN_POINT('Ctrl Pts',(-29.9147250044772,-4.06504339264135,
135.496970357558));
#236064=CARTESIAN_POINT('Ctrl Pts',(-30.1931726282902,1.75077022794215,
136.760866939637));
#236065=CARTESIAN_POINT('Ctrl Pts',(-30.471620252103,5.95771153892721,132.551025203244));
#236066=CARTESIAN_POINT('Ctrl Pts',(-30.750067875916,4.68980699602731,126.736084041921));
#236067=CARTESIAN_POINT('Ctrl Pts',(-31.0285154997288,-0.887801066412759,
124.659690307256));
#236068=CARTESIAN_POINT('Ctrl Pts',(-31.3069631235417,-5.6495633203129,
128.229948403933));
#236069=CARTESIAN_POINT('Ctrl Pts',(-31.5854107473546,-5.21965287935721,
134.16596555791));
#236070=CARTESIAN_POINT('Ctrl Pts',(-31.8638583711675,0.00686356350839004,
137.012831995241));
#236071=CARTESIAN_POINT('Ctrl Pts',(-32.1423059949804,5.22707272681363,
134.154416537178));
#236072=CARTESIAN_POINT('Ctrl Pts',(-32.4207536187933,5.64385741087595,
128.217463348321));
#236073=CARTESIAN_POINT('Ctrl Pts',(-32.6992012426062,0.874212852105795,
124.657742372942));
#236074=CARTESIAN_POINT('Ctrl Pts',(-32.9776488664191,-4.69879061007736,
126.746463285377));
#236075=CARTESIAN_POINT('Ctrl Pts',(-33.2560964902319,-5.9538350502823,
132.564193606789));
#236076=CARTESIAN_POINT('Ctrl Pts',(-33.5345441140448,-1.73759594028995,
136.764723383724));
#236077=CARTESIAN_POINT('Ctrl Pts',(-33.8129917378578,4.07540895254819,
135.487970958469));
#236078=CARTESIAN_POINT('Ctrl Pts',(-34.0914393616706,6.14331211279008,
129.907209437008));
#236079=CARTESIAN_POINT('Ctrl Pts',(-34.3698869854835,2.56581155885918,
125.150886022208));
#236080=CARTESIAN_POINT('Ctrl Pts',(-34.6483346092964,-3.3695444708001,
125.589829572953));
#236081=CARTESIAN_POINT('Ctrl Pts',(-34.9267822331094,-6.2084537431929,
130.820672409693));
#236082=CARTESIAN_POINT('Ctrl Pts',(-35.2052298569221,-3.34209732541825,
136.036525506343));
#236083=CARTESIAN_POINT('Ctrl Pts',(-35.4836774807351,2.59548326388451,
136.444274675672));
#236084=CARTESIAN_POINT('Ctrl Pts',(-35.7621251045479,6.14794153008404,
131.66921835072));
#236085=CARTESIAN_POINT('Ctrl Pts',(-36.0405727283609,4.05074187377708,
126.099400019648));
#236086=CARTESIAN_POINT('Ctrl Pts',(-36.3190203521737,-1.76889167478912,
124.85321062796));
#236087=CARTESIAN_POINT('Ctrl Pts',(-36.5974679759867,-5.96300018938643,
129.075837346879));
#236088=CARTESIAN_POINT('Ctrl Pts',(-36.8759155997995,-4.67740283869194,
134.886892508504));
#236089=CARTESIAN_POINT('Ctrl Pts',(-37.1543632236125,0.906499216928551,
136.946300305126));
#236090=CARTESIAN_POINT('Ctrl Pts',(-37.4328108474252,5.65737277714046,
133.361565579315));
#236091=CARTESIAN_POINT('Ctrl Pts',(-37.7112584712383,5.2093971331851,127.426884420063));
#236092=CARTESIAN_POINT('Ctrl Pts',(-37.9897060950511,-0.0257599829691867,
124.595938887431));
#236093=CARTESIAN_POINT('Ctrl Pts',(-38.268153718864,-5.23724493321992,
127.470229626529));
#236094=CARTESIAN_POINT('Ctrl Pts',(-38.5466013426768,-5.63595764348039,
133.408423865036));
#236095=CARTESIAN_POINT('Ctrl Pts',(-38.8250489664898,-0.855500611219946,
136.953611194679));
#236096=CARTESIAN_POINT('Ctrl Pts',(-39.1034965903026,4.71111968922328,
134.847937651547));
#236097=CARTESIAN_POINT('Ctrl Pts',(-39.3819442141156,5.94845114626212,
129.026414353905));
#236098=CARTESIAN_POINT('Ctrl Pts',(-39.6603918379284,1.71944659787975,
124.838736815064));
#236099=CARTESIAN_POINT('Ctrl Pts',(-39.9388394617414,-4.08964537431793,
126.133176113797));
#236100=CARTESIAN_POINT('Ctrl Pts',(-40.2172870855541,-6.14055303780089,
131.720205771443));
#236101=CARTESIAN_POINT('Ctrl Pts',(-40.495734709367,-2.54859244223803,
136.465618474199));
#236102=CARTESIAN_POINT('Ctrl Pts',(-40.7741823331801,3.3854001020792,136.008611774531));
#236103=CARTESIAN_POINT('Ctrl Pts',(-41.0526299569928,6.20837533857501,
130.769152503414));
#236104=CARTESIAN_POINT('Ctrl Pts',(-41.3310775808058,3.3261569349168,125.562047769191));
#236105=CARTESIAN_POINT('Ctrl Pts',(-41.6095252046187,-2.61263720013008,
125.172372441404));
#236106=CARTESIAN_POINT('Ctrl Pts',(-41.8879728284316,-6.15054538268038,
129.958219109591));
#236107=CARTESIAN_POINT('Ctrl Pts',(-42.1664204522444,-4.03640282939359,
135.521628487296));
#236108=CARTESIAN_POINT('Ctrl Pts',(-42.4448680760573,1.78699673486542,
136.750099144066));
#236109=CARTESIAN_POINT('Ctrl Pts',(-42.7233156998703,5.96823359942677,
132.514726560457));
#236110=CARTESIAN_POINT('Ctrl Pts',(-43.0017633236831,4.66495535053527,
126.707611231352));
#236111=CARTESIAN_POINT('Ctrl Pts',(-43.2802109474961,-0.925188969759574,
124.665208450844));
#236112=CARTESIAN_POINT('Ctrl Pts',(-43.5586585713089,-5.6651298248394,
128.264386597296));
#236113=CARTESIAN_POINT('Ctrl Pts',(-43.8371061951219,-5.19909312786956,
134.197676783747));
#236114=CARTESIAN_POINT('Ctrl Pts',(-44.1155538189346,0.0446561637927345,
137.012675186187));
#236115=CARTESIAN_POINT('Ctrl Pts',(-44.3940014427476,5.24736862250453,
134.122535793092));
#236116=CARTESIAN_POINT('Ctrl Pts',(-44.6724490665605,5.62800566534308,
128.183155515557));
#236117=CARTESIAN_POINT('Ctrl Pts',(-44.9508966903734,0.836780445093053,
124.65253467378));
#236118=CARTESIAN_POINT('Ctrl Pts',(-45.2293443141862,-4.72340512520001,
126.775141340936));
#236119=CARTESIAN_POINT('Ctrl Pts',(-45.5077919379991,-5.94301213660306,
132.600403685011));
#236120=CARTESIAN_POINT('Ctrl Pts',(-45.7862395618121,-1.7012813267513,
136.775190191685));
#236121=CARTESIAN_POINT('Ctrl Pts',(-46.0646871856249,4.10384391017172,
135.463076010984));
#236122=CARTESIAN_POINT('Ctrl Pts',(-46.3431348094379,6.13773707756737,
129.869829974632));
#236123=CARTESIAN_POINT('Ctrl Pts',(-46.6215824332507,2.5313497158043,125.135371944775));
#236124=CARTESIAN_POINT('Ctrl Pts',(-46.9000300570636,-3.40122437147435,
125.610437559721));
#236125=CARTESIAN_POINT('Ctrl Pts',(-47.1784776808764,-6.20823942041608,
130.858464727578));
#236126=CARTESIAN_POINT('Ctrl Pts',(-47.4569253046894,-3.31018573135201,
136.056772861467));
#236127=CARTESIAN_POINT('Ctrl Pts',(-47.7353729285023,2.62976693326135,
136.428370737814));
#236128=CARTESIAN_POINT('Ctrl Pts',(-48.0138205523151,6.15309225746451,
131.631778061822));
#236129=CARTESIAN_POINT('Ctrl Pts',(-48.2922681761281,4.02202639232555,
126.074829176147));
#236130=CARTESIAN_POINT('Ctrl Pts',(-48.570715799941,-1.80508524044794,
124.864088634681));
#236131=CARTESIAN_POINT('Ctrl Pts',(-48.8491634237538,-5.97341172056607,
129.112167847066));
#236132=CARTESIAN_POINT('Ctrl Pts',(-49.1276110475668,-4.65246464686987,
134.915289547327));
#236133=CARTESIAN_POINT('Ctrl Pts',(-49.4060586713796,0.943870151766231,
136.940668391181));
#236134=CARTESIAN_POINT('Ctrl Pts',(-49.6845062951925,5.6728343915496,133.327080166382));
#236135=CARTESIAN_POINT('Ctrl Pts',(-49.9629539190054,5.18874095886556,
127.395235917922));
#236136=CARTESIAN_POINT('Ctrl Pts',(-50.2414015428183,-0.0635519309279763,
124.596210723434));
#236137=CARTESIAN_POINT('Ctrl Pts',(-50.5198491666312,-5.25744370088312,
127.50217199667));
#236138=CARTESIAN_POINT('Ctrl Pts',(-50.798296790444,-5.6200015501302,133.442683291627));
#236139=CARTESIAN_POINT('Ctrl Pts',(-51.076744414257,-0.818052527146474,
136.958704938348));
#236140=CARTESIAN_POINT('Ctrl Pts',(-51.3551920380699,4.73564680419706,
134.819184810706));
#236141=CARTESIAN_POINT('Ctrl Pts',(-51.6336396618827,5.93751807169133,
128.990237384633));
#236142=CARTESIAN_POINT('Ctrl Pts',(-51.9120872856956,1.68310029518491,
124.828380584778));
#236143=CARTESIAN_POINT('Ctrl Pts',(-52.1905349095086,-4.11800442857602,
126.1581574922));
#236144=CARTESIAN_POINT('Ctrl Pts',(-52.4689825333214,-6.13486425817587,
131.757568092191));
#236145=CARTESIAN_POINT('Ctrl Pts',(-52.7474301571343,-2.51408353929296,
136.481027589776));
#236146=CARTESIAN_POINT('Ctrl Pts',(-53.0258777809472,3.41701713239144,
135.987907460498));
#236147=CARTESIAN_POINT('Ctrl Pts',(-53.3043254047601,6.20804598997526,
130.731361012906));
#236148=CARTESIAN_POINT('Ctrl Pts',(-53.5827730285729,3.29418386267868,
125.541897635768));
#236149=CARTESIAN_POINT('Ctrl Pts',(-53.8612206523859,-2.64687230459117,
125.188380653292));
#236150=CARTESIAN_POINT('Ctrl Pts',(-54.1396682761987,-6.15558213084251,
129.995674902111));
#236151=CARTESIAN_POINT('Ctrl Pts',(-54.4181159000117,-4.0076126957546,
135.546111816938));
#236152=CARTESIAN_POINT('Ctrl Pts',(-54.6965635238244,1.82315702396754,
136.739111026966));
#236153=CARTESIAN_POINT('Ctrl Pts',(-54.9750111476374,5.97853450483549,
132.478364539431));
#236154=CARTESIAN_POINT('Ctrl Pts',(-55.2534587714502,4.63993084340721,
126.679290227339));
#236155=CARTESIAN_POINT('Ctrl Pts',(-55.5319063952633,-0.962542589888887,
124.670954082973));
#236156=CARTESIAN_POINT('Ctrl Pts',(-55.810354019076,-5.68048640589689,
128.298918910331));
#236157=CARTESIAN_POINT('Ctrl Pts',(-56.088801642889,-5.1783407220741,134.229262269005));
#236158=CARTESIAN_POINT('Ctrl Pts',(-56.3672492667019,0.0824471093265141,
137.012288325754));
#236159=CARTESIAN_POINT('Ctrl Pts',(-56.6456968905149,5.26747007502141,
134.090532092806));
#236160=CARTESIAN_POINT('Ctrl Pts',(-56.9241445143275,5.6119453719906,128.148944812513));
#236161=CARTESIAN_POINT('Ctrl Pts',(-57.2025921381407,0.799317030873196,
124.64755493279));
#236162=CARTESIAN_POINT('Ctrl Pts',(-57.4810397619534,-4.74784461280872,
126.803968700697));
#236163=CARTESIAN_POINT('Ctrl Pts',(-57.7594873857663,-5.93196900242356,
132.636547210196));
#236164=CARTESIAN_POINT('Ctrl Pts',(-58.0379350095792,-1.66490367160747,
136.785435748359));
#236165=CARTESIAN_POINT('Ctrl Pts',(-58.3163826333922,4.13212679834998,
135.438008433087));
#236166=CARTESIAN_POINT('Ctrl Pts',(-58.5948302572049,6.13193460624012,
129.832485141631));
#236167=CARTESIAN_POINT('Ctrl Pts',(-58.873277881018,2.49679407265481,125.120067933803));
#236168=CARTESIAN_POINT('Ctrl Pts',(-59.1517255048308,-3.43277823852872,
125.631238009216));
#236169=CARTESIAN_POINT('Ctrl Pts',(-59.4301731286437,-6.20779504904446,
130.896255040614));
#236170=CARTESIAN_POINT('Ctrl Pts',(-59.7086207524566,-3.27815147713605,
136.076825586523));
#236171=CARTESIAN_POINT('Ctrl Pts',(-59.9870683762695,2.66395315565763,
136.412258400192));
#236172=CARTESIAN_POINT('Ctrl Pts',(-60.2655160000824,6.15801497974849,
131.594307112665));
#236173=CARTESIAN_POINT('Ctrl Pts',(-60.5439636238952,3.99316187320697,
126.050433587173));
#236174=CARTESIAN_POINT('Ctrl Pts',(-60.8224112477081,-1.84121191800936,
124.875186760365));
#236175=CARTESIAN_POINT('Ctrl Pts',(-61.1008588715211,-5.98360190477769,
129.148561052078));
#236176=CARTESIAN_POINT('Ctrl Pts',(-61.3793064953339,-4.62735405625939,
134.943534254169));
#236177=CARTESIAN_POINT('Ctrl Pts',(-61.6577541191468,0.981206111148332,
136.934809094094));
#236178=CARTESIAN_POINT('Ctrl Pts',(-61.9362017429597,5.68808579699418,
133.292501273148));
#236179=CARTESIAN_POINT('Ctrl Pts',(-62.2146493667725,5.16789251384163,
127.36371374215));
#236180=CARTESIAN_POINT('Ctrl Pts',(-62.4930969905855,-0.10134152394658,
124.596712604715));
#236181=CARTESIAN_POINT('Ctrl Pts',(-62.7715446143984,-5.27744765203657,
127.534236730624));
#236182=CARTESIAN_POINT('Ctrl Pts',(-63.0499922382113,-5.60383720555579,
133.476844954201));
#236183=CARTESIAN_POINT('Ctrl Pts',(-63.3284398620242,-0.780574129835986,
136.963570630527));
#236184=CARTESIAN_POINT('Ctrl Pts',(-63.606887485837,4.75999843803683,134.790283199078));
#236185=CARTESIAN_POINT('Ctrl Pts',(-63.88533510965,5.92636498020503,128.954127638363));
#236186=CARTESIAN_POINT('Ctrl Pts',(-64.1637827334628,1.64669162458969,
124.818245796629));
#236187=CARTESIAN_POINT('Ctrl Pts',(-64.4422303572757,-4.14621088866563,
126.183311037368));
#236188=CARTESIAN_POINT('Ctrl Pts',(-64.7206779810887,-6.12894814889968,
131.794895091487));
#236189=CARTESIAN_POINT('Ctrl Pts',(-64.9991256049015,-2.47948147605779,
136.49622635437));
#236190=CARTESIAN_POINT('Ctrl Pts',(-65.2775732287142,3.44850754387722,
135.967011068231));
#236191=CARTESIAN_POINT('Ctrl Pts',(-65.5560208525274,6.20748659994837,
130.693572227424));
#236192=CARTESIAN_POINT('Ctrl Pts',(-65.83446847634,3.26208872324607,125.521942504845));
#236193=CARTESIAN_POINT('Ctrl Pts',(-66.1129161001531,-2.68100932822562,
125.204596967384));
#236194=CARTESIAN_POINT('Ctrl Pts',(-66.3913637239659,-6.1603907816451,
130.033160660777));
#236195=CARTESIAN_POINT('Ctrl Pts',(-66.6698113477789,-3.97867405855336,
135.570419439246));
#236196=CARTESIAN_POINT('Ctrl Pts',(-66.9482589715917,1.85924975531565,
136.727902995508));
#236197=CARTESIAN_POINT('Ctrl Pts',(-67.2267065954047,5.98861387344954,
132.441940487574));
#236198=CARTESIAN_POINT('Ctrl Pts',(-67.5051542192175,4.61473440193538,
126.651122079325));
#236199=CARTESIAN_POINT('Ctrl Pts',(-67.7836018430304,-0.999860542648545,
124.676926990737));
#236200=CARTESIAN_POINT('Ctrl Pts',(-68.0620494668433,-5.69563249444164,
128.33354406343));
#236201=CARTESIAN_POINT('Ctrl Pts',(-68.3404970906562,-5.15739643095884,
134.260720843274));
#236202=CARTESIAN_POINT('Ctrl Pts',(-68.618944714469,0.120234999752325,
137.011671428276));
#236203=CARTESIAN_POINT('Ctrl Pts',(-68.8973923382821,5.28737633949755,
134.058406622227));
#236204=CARTESIAN_POINT('Ctrl Pts',(-69.1758399620947,5.59567712593856,
128.114832506878));
#236205=CARTESIAN_POINT('Ctrl Pts',(-69.4542875859078,0.761823997666808,
124.642803334499));
#236206=CARTESIAN_POINT('Ctrl Pts',(-69.7327352097205,-4.77210816728929,
126.832944296451));
#236207=CARTESIAN_POINT('Ctrl Pts',(-70.0111828335336,-5.92070605695121,
132.672622843033));
#236208=CARTESIAN_POINT('Ctrl Pts',(-70.2896304573463,-1.62846432284579,
136.795459674095));
#236209=CARTESIAN_POINT('Ctrl Pts',(-70.5680780811594,4.16025656905012,
135.412769153666));
#236210=CARTESIAN_POINT('Ctrl Pts',(-70.8465257049722,6.12590491382102,
129.795176321834));
#236211=CARTESIAN_POINT('Ctrl Pts',(-71.1249733287852,2.46214590988275,
125.104974556385));
#236212=CARTESIAN_POINT('Ctrl Pts',(-71.4034209525978,-3.46420490272305,
125.652230150673));
#236213=CARTESIAN_POINT('Ctrl Pts',(-71.681868576411,-6.20712064554441,
130.93404194847));
#236214=CARTESIAN_POINT('Ctrl Pts',(-71.9603162002238,-3.24599574981168,
136.09668293845));
#236215=CARTESIAN_POINT('Ctrl Pts',(-72.2387638240367,2.69804066428979,
136.395938259856));
#236216=CARTESIAN_POINT('Ctrl Pts',(-72.5172114478495,6.16270951452303,
131.556806891751));
#236217=CARTESIAN_POINT('Ctrl Pts',(-72.7956590716624,3.96414938600637,
126.026214156713));
#236218=CARTESIAN_POINT('Ctrl Pts',(-73.0741066954753,-1.87727036878649,
124.886504593767));
#236219=CARTESIAN_POINT('Ctrl Pts',(-73.3525543192881,-5.99357036442037,
129.185015613353));
#236220=CARTESIAN_POINT('Ctrl Pts',(-73.6310019431012,-4.60207199734241,
134.971625582408));
#236221=CARTESIAN_POINT('Ctrl Pts',(-73.909449566914,1.01850571157763,136.928722630985));
#236222=CARTESIAN_POINT('Ctrl Pts',(-74.187897190727,5.70312642832773,133.257830180947));
#236223=CARTESIAN_POINT('Ctrl Pts',(-74.4663448145398,5.14685257066011,
127.332319060812));
#236224=CARTESIAN_POINT('Ctrl Pts',(-74.7447924383527,-0.139127361718492,
124.597444512675));
#236225=CARTESIAN_POINT('Ctrl Pts',(-75.0232400621657,-5.29725604542678,
127.566422640223));
#236226=CARTESIAN_POINT('Ctrl Pts',(-75.3016876859784,-5.58746520873256,
133.510907586884));
#236227=CARTESIAN_POINT('Ctrl Pts',(-75.5801353097915,-0.743066808063574,
136.968208090913));
#236228=CARTESIAN_POINT('Ctrl Pts',(-75.8585829336042,4.7841736883842,134.761233887624));
#236229=CARTESIAN_POINT('Ctrl Pts',(-76.1370305574171,5.91499228508486,
128.918086453158));
#236230=CARTESIAN_POINT('Ctrl Pts',(-76.41547818123,1.61022193523031,124.808332826166));
#236231=CARTESIAN_POINT('Ctrl Pts',(-76.693925805043,-4.17426370938676,
126.208635817229));
#236232=CARTESIAN_POINT('Ctrl Pts',(-76.9723734288558,-6.12280492919574,
131.832185386163));
#236233=CARTESIAN_POINT('Ctrl Pts',(-77.2508210526686,-2.44478753472383,
136.511214204787));
#236234=CARTESIAN_POINT('Ctrl Pts',(-77.5292686764817,3.47987016964863,
135.945923372052));
#236235=CARTESIAN_POINT('Ctrl Pts',(-77.8077163002943,6.20669718922256,
130.655787547247));
#236236=CARTESIAN_POINT('Ctrl Pts',(-78.0861639241075,3.22987270591563,
125.502183115868));
#236237=CARTESIAN_POINT('Ctrl Pts',(-78.3646115479203,-2.71504700607423,
125.221020782777));
#236238=CARTESIAN_POINT('Ctrl Pts',(-78.6430591717333,-6.16497115690175,
130.070674996542));
#236239=CARTESIAN_POINT('Ctrl Pts',(-78.921506795546,-3.94958799012119,
135.594550453492));
#236240=CARTESIAN_POINT('Ctrl Pts',(-79.199954419359,1.89527359148086,136.71647546501));
#236241=CARTESIAN_POINT('Ctrl Pts',(-79.4784020431719,5.9984713317742,132.405455754592));
#236242=CARTESIAN_POINT('Ctrl Pts',(-79.7568496669848,4.58936695978296,
126.623107831093));
#236243=CARTESIAN_POINT('Ctrl Pts',(-80.0352972907976,-1.0371414452086,
124.683126952807));
#236244=CARTESIAN_POINT('Ctrl Pts',(-80.3137449146107,-5.71056752923021,
128.368260773546));
#236245=CARTESIAN_POINT('Ctrl Pts',(-80.5921925384234,-5.13626103062165,
134.292051340844));
#236246=CARTESIAN_POINT('Ctrl Pts',(-80.8706401622364,0.158018434826916,
137.010824516613));
#236247=CARTESIAN_POINT('Ctrl Pts',(-81.1490877860493,5.30708667829958,
134.026160571776));
#236248=CARTESIAN_POINT('Ctrl Pts',(-81.4275354098621,5.57920153001237,
128.080819862696));
#236249=CARTESIAN_POINT('Ctrl Pts',(-81.705983033675,0.724302734791404,
124.63828005498));
#236250=CARTESIAN_POINT('Ctrl Pts',(-81.984430657488,-4.79619488954742,
126.862067054498));
#236251=CARTESIAN_POINT('Ctrl Pts',(-82.2628782813007,-5.90922371753823,
132.708629246728));
#236252=CARTESIAN_POINT('Ctrl Pts',(-82.5413259051138,-1.59196463073914,
136.805261597452));
#236253=CARTESIAN_POINT('Ctrl Pts',(-82.8197735289264,4.18823217991362,
135.387359107972));
#236254=CARTESIAN_POINT('Ctrl Pts',(-83.0982211527395,6.11964822374235,
129.757904897731));
#236255=CARTESIAN_POINT('Ctrl Pts',(-83.3766687765523,2.42740651138818,
125.090092371815));
#236256=CARTESIAN_POINT('Ctrl Pts',(-83.6551164003652,-3.49550319953123,
125.67341320622));
#236257=CARTESIAN_POINT('Ctrl Pts',(-83.9335640241781,-6.20621623490623,
130.971824050937));
#236258=CARTESIAN_POINT('Ctrl Pts',(-84.2120116479911,-3.21371974092037,
136.116344181428));
#236259=CARTESIAN_POINT('Ctrl Pts',(-84.4904592718038,2.73202819603347,
136.379410921554));
#236260=CARTESIAN_POINT('Ctrl Pts',(-84.7689068956169,6.16717568783019,
131.519278788663));
#236261=CARTESIAN_POINT('Ctrl Pts',(-85.0473545194296,3.9349900057924,126.002171782228));
#236262=CARTESIAN_POINT('Ctrl Pts',(-85.3258021432425,-1.91325925661942,
124.898041715501));
#236263=CARTESIAN_POINT('Ctrl Pts',(-85.6042497670555,-6.00331673010926,
129.221530180052));
#236264=CARTESIAN_POINT('Ctrl Pts',(-85.8826973908683,-4.57661940695503,
134.999562491112));
#236265=CARTESIAN_POINT('Ctrl Pts',(-86.1611450146813,1.05576757090286,
136.922409227389));
#236266=CARTESIAN_POINT('Ctrl Pts',(-86.4395926384942,5.71795572821454,
133.223068174528));
#236267=CARTESIAN_POINT('Ctrl Pts',(-86.718040262307,5.12562190896342,127.301053037252));
#236268=CARTESIAN_POINT('Ctrl Pts',(-86.9964878861199,-0.176908044074368,
124.598406420195));
#236269=CARTESIAN_POINT('Ctrl Pts',(-87.2749355099329,-5.31686814704595,
127.598728532803));
#236270=CARTESIAN_POINT('Ctrl Pts',(-87.5533831337457,-5.57088616633168,
133.544869927476));
#236271=CARTESIAN_POINT('Ctrl Pts',(-87.8318307575586,-0.70553195167748,
136.972617147663));
#236272=CARTESIAN_POINT('Ctrl Pts',(-88.1102783813713,4.80817165941601,
134.732037952774));
#236273=CARTESIAN_POINT('Ctrl Pts',(-88.3887260051845,5.90340040775061,
128.882115164534));
#236274=CARTESIAN_POINT('Ctrl Pts',(-88.6671736289971,1.57369257850503,
124.798642040718));
#236275=CARTESIAN_POINT('Ctrl Pts',(-88.9456212528103,-4.20216185122988,
126.234130893362));
#236276=CARTESIAN_POINT('Ctrl Pts',(-89.2240688766231,-6.11643482670397,
131.869437594414));
#236277=CARTESIAN_POINT('Ctrl Pts',(-89.5025165004358,-2.41000300088966,
136.525990585645));
#236278=CARTESIAN_POINT('Ctrl Pts',(-89.7809641242489,3.51110384754994,
135.924645153375));
#236279=CARTESIAN_POINT('Ctrl Pts',(-90.0594117480617,6.20567778705031,
130.618008372501));
#236280=CARTESIAN_POINT('Ctrl Pts',(-90.3378593718745,3.19753700446471,
125.482620201028));
#236281=CARTESIAN_POINT('Ctrl Pts',(-90.6163069956876,-2.74898407685696,
125.237651490881));
#236282=CARTESIAN_POINT('Ctrl Pts',(-90.8947546195002,-6.16932308688508,
130.108216519297));
#236283=CARTESIAN_POINT('Ctrl Pts',(-91.1732022433134,-3.92035556825405,
135.618503965492));
#236284=CARTESIAN_POINT('Ctrl Pts',(-91.4516498671261,1.93122719758584,
136.70482885892));
#236285=CARTESIAN_POINT('Ctrl Pts',(-91.7300974909391,6.00810651453776,
132.368911692441));
#236286=CARTESIAN_POINT('Ctrl Pts',(-92.0085451147519,4.56382945695037,
126.595248520721));
#236287=CARTESIAN_POINT('Ctrl Pts',(-92.2869927385648,-1.07438391611076,
124.689553739443));
#236288=CARTESIAN_POINT('Ctrl Pts',(-92.5654403623776,-5.72529095683809,
128.403067754236));
#236289=CARTESIAN_POINT('Ctrl Pts',(-92.8438879861907,-5.11493530424405,
134.323252600751));
#236290=CARTESIAN_POINT('Ctrl Pts',(-93.1223356100035,0.195796014469281,
137.009747622148));
#236291=CARTESIAN_POINT('Ctrl Pts',(-93.4007832338166,5.32660036105212,
133.993795136343));
#236292=CARTESIAN_POINT('Ctrl Pts',(-93.6792308576291,5.56251919472255,
128.046908140318));
#236293=CARTESIAN_POINT('Ctrl Pts',(-93.9576784814422,0.686754632612129,
124.633985261843));
#236294=CARTESIAN_POINT('Ctrl Pts',(-94.2361261052551,-4.82010388703947,
126.891335895681));
#236295=CARTESIAN_POINT('Ctrl Pts',(-94.5145737290679,-5.8975224096676,
132.744565087048));
#236296=CARTESIAN_POINT('Ctrl Pts',(-94.7930213528811,-1.55540594779807,
136.814841155217));
#236297=CARTESIAN_POINT('Ctrl Pts',(-95.0714689766937,4.21605259429308,
135.361779237583));
#236298=CARTESIAN_POINT('Ctrl Pts',(-95.3499166005066,6.11316476784841,
129.720672250431));
#236299=CARTESIAN_POINT('Ctrl Pts',(-95.6283642243196,2.39257716445285,
125.075421931555));
#236300=CARTESIAN_POINT('Ctrl Pts',(-95.9068118481323,-3.52667196918255,
125.694786390909));
#236301=CARTESIAN_POINT('Ctrl Pts',(-96.1852594719453,-6.20508185064282,
131.009599947983));
#236302=CARTESIAN_POINT('Ctrl Pts',(-96.4637070957582,-3.18132464646333,
136.135808586901));
#236303=CARTESIAN_POINT('Ctrl Pts',(-96.742154719571,2.76591449146702,136.362676997713));
#236304=CARTESIAN_POINT('Ctrl Pts',(-97.020602343384,6.17141333417382,131.481724194021));
#236305=CARTESIAN_POINT('Ctrl Pts',(-97.299049967197,3.90568481307747,125.978307354616));
#236306=CARTESIAN_POINT('Ctrl Pts',(-97.5774975910097,-1.94917724792726,
124.909797698053));
#236307=CARTESIAN_POINT('Ctrl Pts',(-97.8559452148228,-6.01284064068852,
129.258103399115));
#236308=CARTESIAN_POINT('Ctrl Pts',(-98.1343928386354,-4.55099722825276,
135.027343945068));
#236309=CARTESIAN_POINT('Ctrl Pts',(-98.4128404624484,1.09299030837272,
136.915869117251));
#236310=CARTESIAN_POINT('Ctrl Pts',(-98.6912880862614,5.73257314714861,
133.188216542011));
#236311=CARTESIAN_POINT('Ctrl Pts',(-98.9697357100741,5.10420131546234,
127.269916830042));
#236312=CARTESIAN_POINT('Ctrl Pts',(-99.2481833338871,-0.214682171037078,
124.599598291628));
#236313=CARTESIAN_POINT('Ctrl Pts',(-99.5266309576999,-5.33628323016052,
127.631153211259));
#236314=CARTESIAN_POINT('Ctrl Pts',(-99.8050785815131,-5.55410069269506,
133.578730717485));
#236315=CARTESIAN_POINT('Ctrl Pts',(-100.083526205326,-0.667970951546107,
136.976797637399));
#236316=CARTESIAN_POINT('Ctrl Pts',(-100.361973829139,4.83199146187865,
134.702696476397));
#236317=CARTESIAN_POINT('Ctrl Pts',(-100.640421452952,5.89158977774298,
128.846215105423));
#236318=CARTESIAN_POINT('Ctrl Pts',(-100.918869076765,1.53710490802326,
124.789173799381));
#236319=CARTESIAN_POINT('Ctrl Pts',(-101.197316700577,-4.22990428042106,
126.259795321038));
#236320=CARTESIAN_POINT('Ctrl Pts',(-101.47576432439,-6.10983807746976,
131.906650335846));
#236321=CARTESIAN_POINT('Ctrl Pts',(-101.754211948203,-2.37512916350784,
136.540554949401));
#236322=CARTESIAN_POINT('Ctrl Pts',(-102.032659572016,3.54220742020778,
135.903177200671));
#236323=CARTESIAN_POINT('Ctrl Pts',(-102.311107195829,6.20442843120499,
130.580236103105));
#236324=CARTESIAN_POINT('Ctrl Pts',(-102.589554819642,3.16508281710451,
125.463254485237));
#236325=CARTESIAN_POINT('Ctrl Pts',(-102.868002443455,-2.78281928302352,
125.254488475437));
#236326=CARTESIAN_POINT('Ctrl Pts',(-103.146450067268,-6.1734464103326,
130.145783837928));
#236327=CARTESIAN_POINT('Ctrl Pts',(-103.424897691081,-3.8909778761698,
135.642279087639));
#236328=CARTESIAN_POINT('Ctrl Pts',(-103.703345314893,1.96710924135641,
136.69296360881));
#236329=CARTESIAN_POINT('Ctrl Pts',(-103.981792938706,6.01751906470488,
132.332309655276));
#236330=CARTESIAN_POINT('Ctrl Pts',(-104.260240562519,4.53812283973896,
126.567545180546));
#236331=CARTESIAN_POINT('Ctrl Pts',(-104.538688186332,-1.11158657532129,
124.696207112496));
#236332=CARTESIAN_POINT('Ctrl Pts',(-104.817135810145,-5.73980223168479,
128.437963715717));
#236333=CARTESIAN_POINT('Ctrl Pts',(-105.095583433958,-5.093420042057,134.354323466822));
#236334=CARTESIAN_POINT('Ctrl Pts',(-105.374031057771,0.233566338818549,
137.008440784786));
#236335=CARTESIAN_POINT('Ctrl Pts',(-105.652478681584,5.34591666467016,
133.961311515241));
#236336=CARTESIAN_POINT('Ctrl Pts',(-105.930926305397,5.54563073823764,
128.013098596357));
#236337=CARTESIAN_POINT('Ctrl Pts',(-106.20937392921,0.649181082487974,
124.629919114234));
#236338=CARTESIAN_POINT('Ctrl Pts',(-106.487821553022,-4.84383427380942,
126.920749735436));
#236339=CARTESIAN_POINT('Ctrl Pts',(-106.766269176835,-5.88560256693534,
132.780429032376));
#236340=CARTESIAN_POINT('Ctrl Pts',(-107.044716800648,-1.51878962871805,
136.824197992414));
#236341=CARTESIAN_POINT('Ctrl Pts',(-107.323164424461,4.2437167812931,135.336030490371));
#236342=CARTESIAN_POINT('Ctrl Pts',(-107.601612048274,6.10645478638612,
129.683479759601));
#236343=CARTESIAN_POINT('Ctrl Pts',(-107.880059672087,2.35765915969063,
125.060963779225));
#236344=CARTESIAN_POINT('Ctrl Pts',(-108.1585072959,-3.55771005670707,125.716348912751));
#236345=CARTESIAN_POINT('Ctrl Pts',(-108.436954919713,-6.20371753478999,
131.04736823981));
#236346=CARTESIAN_POINT('Ctrl Pts',(-108.715402543526,-3.14881166685081,
136.155075433609));
#236347=CARTESIAN_POINT('Ctrl Pts',(-108.993850167338,2.79969829492213,
136.345737108415));
#236348=CARTESIAN_POINT('Ctrl Pts',(-109.272297791151,6.17542229652738,
131.444144499421));
#236349=CARTESIAN_POINT('Ctrl Pts',(-109.550745414964,3.87623489377466,
125.954621758183));
#236350=CARTESIAN_POINT('Ctrl Pts',(-109.829193038777,-1.98502301175461,
124.921772105802));
#236351=CARTESIAN_POINT('Ctrl Pts',(-110.10764066259,-6.02214174324697,
129.294733915307));
#236352=CARTESIAN_POINT('Ctrl Pts',(-110.386088286403,-4.52520641067474,
135.054968914823));
#236353=CARTESIAN_POINT('Ctrl Pts',(-110.664535910216,1.13017254468408,
136.909102542919));
#236354=CARTESIAN_POINT('Ctrl Pts',(-110.942983534029,5.74697814347679,
133.153276574838));
#236355=CARTESIAN_POINT('Ctrl Pts',(-111.221431157841,5.08259158390449,
127.238911592946));
#236356=CARTESIAN_POINT('Ctrl Pts',(-111.499878781655,-0.252448342873548,
124.601020082813));
#236357=CARTESIAN_POINT('Ctrl Pts',(-111.778326405467,-5.3555005753377,
127.663695474083));
#236358=CARTESIAN_POINT('Ctrl Pts',(-112.05677402928,-5.53710940981492,
133.612488702192));
#236359=CARTESIAN_POINT('Ctrl Pts',(-112.335221653093,-0.630385199504834,
136.980749405212));
#236360=CARTESIAN_POINT('Ctrl Pts',(-112.613669276906,4.85563221312083,
134.673210545752));
#236361=CARTESIAN_POINT('Ctrl Pts',(-112.892116900719,5.8795608327098,128.810387606114));
#236362=CARTESIAN_POINT('Ctrl Pts',(-113.170564524532,1.50046027955312,
124.779928453004));
#236363=CARTESIAN_POINT('Ctrl Pts',(-113.449012148345,-4.25748996895278,
126.285628149252));
#236364=CARTESIAN_POINT('Ctrl Pts',(-113.727459772158,-6.10301492593933,
131.943822231527));
#236365=CARTESIAN_POINT('Ctrl Pts',(-114.00590739597,-2.3401673148416,136.554906756366));
#236366=CARTESIAN_POINT('Ctrl Pts',(-114.284355019783,3.57317973506622,
135.881520309444));
#236367=CARTESIAN_POINT('Ctrl Pts',(-114.562802643596,6.202949167983,130.542472138726));
#236368=CARTESIAN_POINT('Ctrl Pts',(-114.841250267409,3.13251134643626,
125.444086686097));
#236369=CARTESIAN_POINT('Ctrl Pts',(-115.119697891222,-2.81655137079845,
125.271531112549));
#236370=CARTESIAN_POINT('Ctrl Pts',(-115.398145515035,-6.17734097445314,
130.183375560363));
#236371=CARTESIAN_POINT('Ctrl Pts',(-115.676593138848,-3.86145600246928,
135.665874938939));
#236372=CARTESIAN_POINT('Ctrl Pts',(-115.955040762661,2.00291839317105,
136.680880154352));
#236373=CARTESIAN_POINT('Ctrl Pts',(-116.233488386474,6.02670863349017,
132.295650999397));
#236374=CARTESIAN_POINT('Ctrl Pts',(-116.511936010287,4.51224806071678,
126.539998837124));
#236375=CARTESIAN_POINT('Ctrl Pts',(-116.790383634099,-1.14874804428301,
124.703086825424));
#236376=CARTESIAN_POINT('Ctrl Pts',(-117.068831257912,-5.75410081604829,
128.472947364906));
#236377=CARTESIAN_POINT('Ctrl Pts',(-117.347278881725,-5.07171604131793,
134.385262787713));
#236378=CARTESIAN_POINT('Ctrl Pts',(-117.625726505538,0.271328008281021,
137.006904052952));
#236379=CARTESIAN_POINT('Ctrl Pts',(-117.904174129351,5.3650348733795,133.928710912162));
#236380=CARTESIAN_POINT('Ctrl Pts',(-118.182621753164,5.52853678636705,
127.979392483636));
#236381=CARTESIAN_POINT('Ctrl Pts',(-118.461069376977,0.611583476719488,
124.626081762825));
#236382=CARTESIAN_POINT('Ctrl Pts',(-118.73951700079,-4.86738517051901,
126.95030748382));
#236383=CARTESIAN_POINT('Ctrl Pts',(-119.017964624603,-5.87346463103546,
132.816219753764));
#236384=CARTESIAN_POINT('Ctrl Pts',(-119.296412248415,-1.48211703032935,
136.833331762325));
#236385=CARTESIAN_POINT('Ctrl Pts',(-119.574859872228,4.27122371580729,
135.310113820466));
#236386=CARTESIAN_POINT('Ctrl Pts',(-119.853307496041,6.09951852799569,
129.646328803424));
#236387=CARTESIAN_POINT('Ctrl Pts',(-120.131755119854,2.32265379100196,
125.046718450578));
#236388=CARTESIAN_POINT('Ctrl Pts',(-120.410202743667,-3.58861631197691,
125.738099972737));
#236389=CARTESIAN_POINT('Ctrl Pts',(-120.68865036748,-6.20212333790203,
131.085127526901));
#236390=CARTESIAN_POINT('Ctrl Pts',(-120.967097991293,-3.11618200686478,
136.174144007612));
#236391=CARTESIAN_POINT('Ctrl Pts',(-121.245545615105,2.83337835452712,
136.328591881372));
#236392=CARTESIAN_POINT('Ctrl Pts',(-121.523993238919,6.17920242633619,
131.406541097396));
#236393=CARTESIAN_POINT('Ctrl Pts',(-121.802440862731,3.84664133916317,
125.931115870606));
#236394=CARTESIAN_POINT('Ctrl Pts',(-122.080888486544,-2.02079521982502,
124.933964495032));
#236395=CARTESIAN_POINT('Ctrl Pts',(-122.359336110357,-6.03121969312815,
129.331420371272));
#236396=CARTESIAN_POINT('Ctrl Pts',(-122.63778373417,-4.49924790990888,
135.082436376724));
#236397=CARTESIAN_POINT('Ctrl Pts',(-122.916231357983,1.16731290203685,
136.90210975513));
#236398=CARTESIAN_POINT('Ctrl Pts',(-123.194678981796,5.76117018341619,
133.118249567719));
#236399=CARTESIAN_POINT('Ctrl Pts',(-123.473126605609,5.06079351504635,
127.208038474877));
#236400=CARTESIAN_POINT('Ctrl Pts',(-123.751574229422,-0.290205160143283,
124.602671741062));
#236401=CARTESIAN_POINT('Ctrl Pts',(-124.030021853235,-5.37451947047147,
127.696354115408));
#236402=CARTESIAN_POINT('Ctrl Pts',(-124.308469477047,-5.51991294730918,
133.646142630679));
#236403=CARTESIAN_POINT('Ctrl Pts',(-124.58691710086,-0.592776088308802,
136.984472304668));
#236404=CARTESIAN_POINT('Ctrl Pts',(-124.865364724673,4.87909303712557,
134.64358125345));
#236405=CARTESIAN_POINT('Ctrl Pts',(-125.143812348486,5.86731401838748,
128.774633994209));
#236406=CARTESIAN_POINT('Ctrl Pts',(-125.422259972299,1.46376005097626,
124.770906344175));
#236407=CARTESIAN_POINT('Ctrl Pts',(-125.700707596112,-4.28491789462882,
126.311628420759));
#236408=CARTESIAN_POINT('Ctrl Pts',(-125.979155219925,-6.09596562494584,
131.980951904039));
#236409=CARTESIAN_POINT('Ctrl Pts',(-126.257602843738,-2.30511875041471,
136.569045474729));
#236410=CARTESIAN_POINT('Ctrl Pts',(-126.536050467551,3.60401964443632,
135.859675282198));
#236411=CARTESIAN_POINT('Ctrl Pts',(-126.814498091363,6.20124005219796,
130.50471787872));
#236412=CARTESIAN_POINT('Ctrl Pts',(-127.092945715177,3.09982379940838,
125.42511751388));
#236413=CARTESIAN_POINT('Ctrl Pts',(-127.371393338989,-2.85017909022625,
125.288778770691));
#236414=CARTESIAN_POINT('Ctrl Pts',(-127.649840962802,-6.18100663493216,
130.220990293627));
#236415=CARTESIAN_POINT('Ctrl Pts',(-127.928288586615,-3.83179104109667,
135.689290645038));
#236416=CARTESIAN_POINT('Ctrl Pts',(-128.206736210428,2.03865332610762,
136.6685789433));
#236417=CARTESIAN_POINT('Ctrl Pts',(-128.485183834241,6.03567488037103,
132.258937083203));
#236418=CARTESIAN_POINT('Ctrl Pts',(-128.763631458054,4.48620607868298,
126.512610511197));
#236419=CARTESIAN_POINT('Ctrl Pts',(-129.042079081867,-1.18586694596332,
124.710192623294));
#236420=CARTESIAN_POINT('Ctrl Pts',(-129.32052670568,-5.76818618009069,
128.508017405469));
#236421=CARTESIAN_POINT('Ctrl Pts',(-129.598974329492,-5.04982410627509,
134.416069416958));
#236422=CARTESIAN_POINT('Ctrl Pts',(-129.877421953305,0.30907962358457,
137.005137483589));
#236423=CARTESIAN_POINT('Ctrl Pts',(-130.155869577118,5.38395427874936,
133.895994535135));
#236424=CARTESIAN_POINT('Ctrl Pts',(-130.434317200931,5.51123797253198,
127.945791051148));
#236425=CARTESIAN_POINT('Ctrl Pts',(-130.712764824744,0.573963208500954,
124.622473349811));
#236426=CARTESIAN_POINT('Ctrl Pts',(-130.991212448557,-4.89075570448117,
126.980008045559));
#236427=CARTESIAN_POINT('Ctrl Pts',(-131.26966007237,-5.8611090517438,132.851935924971));
#236428=CARTESIAN_POINT('Ctrl Pts',(-131.548107696183,-1.44538951154951,
136.842242126491));
#236429=CARTESIAN_POINT('Ctrl Pts',(-131.826555319995,4.29857237855583,
135.28403018822));
#236430=CARTESIAN_POINT('Ctrl Pts',(-132.105002943808,6.09235624970348,
129.609220758541));
#236431=CARTESIAN_POINT('Ctrl Pts',(-132.383450567622,2.28756235552218,
125.032686473479));
#236432=CARTESIAN_POINT('Ctrl Pts',(-132.661898191434,-3.6193895897498,
125.760038764874));
#236433=CARTESIAN_POINT('Ctrl Pts',(-132.940345815247,-6.20029931905343,
131.122876410071));
#236434=CARTESIAN_POINT('Ctrl Pts',(-133.21879343906,-3.08343687560774,
136.193013602317));
#236435=CARTESIAN_POINT('Ctrl Pts',(-133.497241062873,2.86695342225543,
136.311241951909));
#236436=CARTESIAN_POINT('Ctrl Pts',(-133.775688686686,6.18275358352724,
131.368915381349));
#236437=CARTESIAN_POINT('Ctrl Pts',(-134.054136310499,3.81690524584148,
125.907790562906));
#236438=CARTESIAN_POINT('Ctrl Pts',(-134.332583934311,-2.05649254658467,
124.946374413949));
#236439=CARTESIAN_POINT('Ctrl Pts',(-134.611031558124,-6.04007415394596,
129.36816140758));
#236440=CARTESIAN_POINT('Ctrl Pts',(-134.889479181937,-4.47312268785726,
135.109745312956));
#236441=CARTESIAN_POINT('Ctrl Pts',(-135.16792680575,1.20441000418008,136.894891013003));
#236442=CARTESIAN_POINT('Ctrl Pts',(-135.446374429563,5.775148741076,133.083136818595));
#236443=CARTESIAN_POINT('Ctrl Pts',(-135.724822053376,5.03880791662344,
127.177298619846));
#236444=CARTESIAN_POINT('Ctrl Pts',(-136.003269677189,-0.327951223754644,
124.604553205172));
#236445=CARTESIAN_POINT('Ctrl Pts',(-136.281717301002,-5.39333921080989,
127.729127925058));
#236446=CARTESIAN_POINT('Ctrl Pts',(-136.560164924815,-5.50251194239939,
133.679691255889));
#236447=CARTESIAN_POINT('Ctrl Pts',(-136.838612548628,-0.555145011576188,
136.987966197812));
#236448=CARTESIAN_POINT('Ctrl Pts',(-137.117060172441,4.90237306454367,
134.613809697415));
#236449=CARTESIAN_POINT('Ctrl Pts',(-137.395507796253,5.8548497885868,128.73895559457));
#236450=CARTESIAN_POINT('Ctrl Pts',(-137.673955420066,1.42700558223168,
124.762107807213));
#236451=CARTESIAN_POINT('Ctrl Pts',(-137.952403043879,-4.3121870410957,
126.33779517211));
#236452=CARTESIAN_POINT('Ctrl Pts',(-138.230850667692,-6.08869043570493,
132.018037977528));
#236453=CARTESIAN_POINT('Ctrl Pts',(-138.509298291505,-2.26998476896503,
136.582970580575));
#236454=CARTESIAN_POINT('Ctrl Pts',(-138.787745915318,3.63472600553235,
135.837642928407));
#236455=CARTESIAN_POINT('Ctrl Pts',(-139.066193539131,6.1993011471828,130.466974722087));
#236456=CARTESIAN_POINT('Ctrl Pts',(-139.344641162943,3.06702138726935,
125.406347671494));
#236457=CARTESIAN_POINT('Ctrl Pts',(-139.623088786757,-2.88370119522,125.306230810748));
#236458=CARTESIAN_POINT('Ctrl Pts',(-139.901536410569,-6.18444325593727,
130.258626643894));
#236459=CARTESIAN_POINT('Ctrl Pts',(-140.179984034382,-3.80198409129777,
135.712525338258));
#236460=CARTESIAN_POINT('Ctrl Pts',(-140.458431658195,2.07431271599591,
136.656060431482));
#236461=CARTESIAN_POINT('Ctrl Pts',(-140.736879282008,6.04441747309895,
132.222169267145));
#236462=CARTESIAN_POINT('Ctrl Pts',(-141.015326905821,4.45999785863389,
126.485381217648));
#236463=CARTESIAN_POINT('Ctrl Pts',(-141.293774529634,-1.22294190490765,
124.717524242802));
#236464=CARTESIAN_POINT('Ctrl Pts',(-141.572222153447,-5.78205780187226,
128.543172537875));
#236465=CARTESIAN_POINT('Ctrl Pts',(-141.85066977726,-5.02774504814366,
134.446742213005));
#236466=CARTESIAN_POINT('Ctrl Pts',(-142.129117401072,0.346819785828787,
137.003141142159));
#236467=CARTESIAN_POINT('Ctrl Pts',(-142.407565024885,5.40267417971275,
133.863163596476));
#236468=CARTESIAN_POINT('Ctrl Pts',(-142.686012648698,5.49373493774783,
127.912295544006));
#236469=CARTESIAN_POINT('Ctrl Pts',(-142.964460272511,0.536321671864061,
124.619094008905));
#236470=CARTESIAN_POINT('Ctrl Pts',(-143.242907896324,-4.91394500969209,
127.00985032009));
#236471=CARTESIAN_POINT('Ctrl Pts',(-143.521355520137,-5.84853628690073,
132.887576222521));
#236472=CARTESIAN_POINT('Ctrl Pts',(-143.79980314395,-1.40860843332932,
136.850928754739));
#236473=CARTESIAN_POINT('Ctrl Pts',(-144.078250767763,4.32576175612421,
135.257780560169));
#236474=CARTESIAN_POINT('Ctrl Pts',(-144.356698391576,6.08496821690962,
129.572157000006));
#236475=CARTESIAN_POINT('Ctrl Pts',(-144.635146015388,2.2523861535788,125.018868367886));
#236476=CARTESIAN_POINT('Ctrl Pts',(-144.913593639201,-3.65002874971022,
125.782164476213));
#236477=CARTESIAN_POINT('Ctrl Pts',(-145.192041263014,-6.19824554583293,
131.160613490521));
#236478=CARTESIAN_POINT('Ctrl Pts',(-145.470488886827,-3.05057748646412,
136.211683518503));
#236479=CARTESIAN_POINT('Ctrl Pts',(-145.74893651064,2.90042225397064,136.293687962933));
#236480=CARTESIAN_POINT('Ctrl Pts',(-146.027384134453,6.18607563651005,
131.33126874552));
#236481=CARTESIAN_POINT('Ctrl Pts',(-146.305831758266,3.78702771569254,
125.884646699409));
#236482=CARTESIAN_POINT('Ctrl Pts',(-146.584279382079,-2.09211366925746,
124.959001402698));
#236483=CARTESIAN_POINT('Ctrl Pts',(-146.862727005891,-6.04870479759444,
129.404955662777));
#236484=CARTESIAN_POINT('Ctrl Pts',(-147.141174629705,-4.4468317125993,
135.136894711575));
#236485=CARTESIAN_POINT('Ctrl Pts',(-147.419622253517,1.24146247646836,
136.887446584034));
#236486=CARTESIAN_POINT('Ctrl Pts',(-147.69806987733,5.78891329847519,133.04793962858));
#236487=CARTESIAN_POINT('Ctrl Pts',(-147.976517501143,5.01663560332014,
127.146693166932));
#236488=CARTESIAN_POINT('Ctrl Pts',(-148.254965124956,-0.365685135012239,
124.606664405427));
#236489=CARTESIAN_POINT('Ctrl Pts',(-148.533412748769,-5.41195909898036,
127.762015688586));
#236490=CARTESIAN_POINT('Ctrl Pts',(-148.811860372582,-5.48490703988586,
133.713133334664));
#236491=CARTESIAN_POINT('Ctrl Pts',(-149.090307996395,-0.517493363741682,
136.991230955176));
#236492=CARTESIAN_POINT('Ctrl Pts',(-149.368755620208,4.92547143272535,
134.583896980843));
#236493=CARTESIAN_POINT('Ctrl Pts',(-149.647203244021,5.84216860517359,
128.703353729273));
#236494=CARTESIAN_POINT('Ctrl Pts',(-149.925650867833,1.39019823527075,
124.753533168151));
#236495=CARTESIAN_POINT('Ctrl Pts',(-150.204098491647,-4.33929639788676,
126.364127433687));
#236496=CARTESIAN_POINT('Ctrl Pts',(-150.482546115459,-6.08118962780021,
132.055079077756));
#236497=CARTESIAN_POINT('Ctrl Pts',(-150.760993739272,-2.23476667239474,
136.596681557904));
#236498=CARTESIAN_POINT('Ctrl Pts',(-151.039441363085,3.66529768052036,
135.81542406449));
#236499=CARTESIAN_POINT('Ctrl Pts',(-151.317888986898,6.19713252478332,
130.429244067412));
#236500=CARTESIAN_POINT('Ctrl Pts',(-151.596336610711,3.03410532552526,
125.387777854462));
#236501=CARTESIAN_POINT('Ctrl Pts',(-151.874784234524,-2.91711644360522,
125.323886586026));
#236502=CARTESIAN_POINT('Ctrl Pts',(-152.153231858337,-6.18765071012318,
130.296283216534));
#236503=CARTESIAN_POINT('Ctrl Pts',(-152.431679482149,-3.77203625758034,
135.735578157629));
#236504=CARTESIAN_POINT('Ctrl Pts',(-152.710127105962,2.10989524146327,
136.643325082775));
#236505=CARTESIAN_POINT('Ctrl Pts',(-152.988574729775,6.0529360877152,132.185348913665));
#236506=CARTESIAN_POINT('Ctrl Pts',(-153.267022353588,4.43362437172323,
126.458311965469));
#236507=CARTESIAN_POINT('Ctrl Pts',(-153.545469977401,-1.25997154729018,
124.725081412269));
#236508=CARTESIAN_POINT('Ctrl Pts',(-153.823917601214,-5.79571516737629,
128.578411459437));
#236509=CARTESIAN_POINT('Ctrl Pts',(-154.102365225027,-5.00547968506979,
134.477280039263));
#236510=CARTESIAN_POINT('Ctrl Pts',(-154.38081284884,0.38454709653853,137.000915102638));
#236511=CARTESIAN_POINT('Ctrl Pts',(-154.659260472653,5.4211938825983,133.830219312748));
#236512=CARTESIAN_POINT('Ctrl Pts',(-154.937708096465,5.47602833059452,
127.8789072034));
#236513=CARTESIAN_POINT('Ctrl Pts',(-155.216155720278,0.498660261630971,
124.615943865326));
#236514=CARTESIAN_POINT('Ctrl Pts',(-155.494603344091,-4.93695222686361,
127.039833201595));
#236515=CARTESIAN_POINT('Ctrl Pts',(-155.773050967904,-5.83574680239484,
132.923139325752));
#236516=CARTESIAN_POINT('Ctrl Pts',(-156.051498591717,-1.37177515860606,
136.85939132518));
#236517=CARTESIAN_POINT('Ctrl Pts',(-156.32994621553,4.3527908409998,135.231365909006));
#236518=CARTESIAN_POINT('Ctrl Pts',(-156.608393839343,6.0773547033811,129.535138901228));
#236519=CARTESIAN_POINT('Ctrl Pts',(-156.886841463156,2.21712648863745,
125.005264645838));
#236520=CARTESIAN_POINT('Ctrl Pts',(-157.165289086968,-3.68053265651321,
125.804476286877));
#236521=CARTESIAN_POINT('Ctrl Pts',(-157.443736710782,-6.19596209434481,
131.19833736989));
#236522=CARTESIAN_POINT('Ctrl Pts',(-157.722184334594,-3.0176050570491,
136.230153064351));
#236523=CARTESIAN_POINT('Ctrl Pts',(-158.000631958407,2.93378360947182,
136.275930564914));
#236524=CARTESIAN_POINT('Ctrl Pts',(-158.27907958222,6.18916846218569,131.293602584915));
#236525=CARTESIAN_POINT('Ctrl Pts',(-158.557527206033,3.7570098558391,125.861685137721));
#236526=CARTESIAN_POINT('Ctrl Pts',(-158.835974829846,-2.12765726788813,
124.971844993383));
#236527=CARTESIAN_POINT('Ctrl Pts',(-159.114422453659,-6.05711130426257,
129.44180177344));
#236528=CARTESIAN_POINT('Ctrl Pts',(-159.392870077472,-4.42037595835707,
135.163883566548));
#236529=CARTESIAN_POINT('Ctrl Pts',(-159.671317701285,1.27846894590735,
136.879776744077));
#236530=CARTESIAN_POINT('Ctrl Pts',(-159.949765325097,5.80246334556346,
133.01265930192));
#236531=CARTESIAN_POINT('Ctrl Pts',(-160.22821294891,4.9942773967397,127.116223250229));
#236532=CARTESIAN_POINT('Ctrl Pts',(-160.506660572723,-0.403405495673234,
124.609005263594));
#236533=CARTESIAN_POINT('Ctrl Pts',(-160.785108196536,-5.43037844501628,
127.795016187323));
#236534=CARTESIAN_POINT('Ctrl Pts',(-161.063555820349,-5.46709889212507,
133.746467627798));
#236535=CARTESIAN_POINT('Ctrl Pts',(-161.342003444162,-0.479822539999598,
136.994266455786));
#236536=CARTESIAN_POINT('Ctrl Pts',(-161.620451067975,4.94838728575097,
134.553844212161));
#236537=CARTESIAN_POINT('Ctrl Pts',(-161.898898691787,5.82927093805496,
128.66782971756));
#236538=CARTESIAN_POINT('Ctrl Pts',(-162.177346315601,1.35333937400316,
124.745182744726));
#236539=CARTESIAN_POINT('Ctrl Pts',(-162.455793939413,-4.36624496045326,
126.390624229737));
#236540=CARTESIAN_POINT('Ctrl Pts',(-162.734241563226,-6.07346347917808,
132.092073832152));
#236541=CARTESIAN_POINT('Ctrl Pts',(-163.012689187039,-2.19946576572379,
136.61017789865));
#236542=CARTESIAN_POINT('Ctrl Pts',(-163.291136810852,3.69573353655413,
135.793019513774));
#236543=CARTESIAN_POINT('Ctrl Pts',(-163.569584434665,6.19473426535967,
130.391527312818));
#236544=CARTESIAN_POINT('Ctrl Pts',(-163.848032058478,3.0010768338922,125.369408750896));
#236545=CARTESIAN_POINT('Ctrl Pts',(-164.126479682291,-2.95042359716811,
125.341745442286));
#236546=CARTESIAN_POINT('Ctrl Pts',(-164.404927306104,-6.19062887863655,
130.333958616169));
#236547=CARTESIAN_POINT('Ctrl Pts',(-164.683374929917,-3.74194864967208,
135.758448248921));
#236548=CARTESIAN_POINT('Ctrl Pts',(-164.961822553729,2.14539958398697,
136.630373369092));
#236549=CARTESIAN_POINT('Ctrl Pts',(-165.240270177542,6.06123040855813,
132.148477387157));
#236550=CARTESIAN_POINT('Ctrl Pts',(-165.518717801355,4.40708659523179,
126.431403757722));
#236551=CARTESIAN_POINT('Ctrl Pts',(-165.797165425168,-1.29695450096345,
124.732863851664));
#236552=CARTESIAN_POINT('Ctrl Pts',(-166.075613048981,-5.80915777052276,
128.613732864363));
#236553=CARTESIAN_POINT('Ctrl Pts',(-166.354060672794,-4.98302884210618,
134.50768176414));
#236554=CARTESIAN_POINT('Ctrl Pts',(-166.632508296607,0.422260157714416,
136.998459447511));
#236555=CARTESIAN_POINT('Ctrl Pts',(-166.91095592042,5.43951270115045,133.797162904712));
#236556=CARTESIAN_POINT('Ctrl Pts',(-167.189403544233,5.45811880719792,
127.845627266545));
#236557=CARTESIAN_POINT('Ctrl Pts',(-167.467851168046,0.460980373357943,
124.613023035806));
#236558=CARTESIAN_POINT('Ctrl Pts',(-167.746298791858,-4.95977650345479,
127.069955579048));
#236559=CARTESIAN_POINT('Ctrl Pts',(-168.024746415672,-5.822741072145,132.958623916859));
#236560=CARTESIAN_POINT('Ctrl Pts',(-168.303194039484,-1.33489105224939,
136.867629524233));
#236561=CARTESIAN_POINT('Ctrl Pts',(-168.581641663297,4.37965863161014,
135.204787213532));
#236562=CARTESIAN_POINT('Ctrl Pts',(-168.86008928711,6.06951599123876,129.498167833929));
#236563=CARTESIAN_POINT('Ctrl Pts',(-169.138536910923,2.18178466725943,
124.991875811423));
#236564=CARTESIAN_POINT('Ctrl Pts',(-169.416984534736,-3.71090017982492,
125.826973370093));
#236565=CARTESIAN_POINT('Ctrl Pts',(-169.695432158549,-6.19344904920226,
131.236046650305));
#236566=CARTESIAN_POINT('Ctrl Pts',(-169.973879782361,-2.98452080916978,
136.248421555465));
#236567=CARTESIAN_POINT('Ctrl Pts',(-170.252327406175,2.96703625254325,
136.257970415857));
#236568=CARTESIAN_POINT('Ctrl Pts',(-170.530775029987,6.19203194594742,
131.25591829527));
#236569=CARTESIAN_POINT('Ctrl Pts',(-170.8092226538,3.72685277860365,125.838906728691));
#236570=CARTESIAN_POINT('Ctrl Pts',(-171.087670277614,-2.16312202539704,
124.984904710079));
#236571=CARTESIAN_POINT('Ctrl Pts',(-171.366117901426,-6.06529336244348,
129.478698374222));
#236572=CARTESIAN_POINT('Ctrl Pts',(-171.644565525239,-4.39375640545797,
135.190710877796));
#236573=CARTESIAN_POINT('Ctrl Pts',(-171.923013149052,1.31542804121008,
136.871881777341));
#236574=CARTESIAN_POINT('Ctrl Pts',(-172.201460772865,5.81579838023838,
132.977297145939));
#236575=CARTESIAN_POINT('Ctrl Pts',(-172.479908396678,4.97173412537368,
127.085889998814));
#236576=CARTESIAN_POINT('Ctrl Pts',(-172.75835602049,-0.441110907994683,
124.611575692932));
#236577=CARTESIAN_POINT('Ctrl Pts',(-173.036803644304,-5.4485965663818,
127.828128198426));
#236578=CARTESIAN_POINT('Ctrl Pts',(-173.315251268116,-5.44908815900415,
133.779692900072));
#236579=CARTESIAN_POINT('Ctrl Pts',(-173.593698891929,-0.442133936257506,
136.997072587158));
#236580=CARTESIAN_POINT('Ctrl Pts',(-173.872146515742,4.97111977446672,
134.523652504987));
#236581=CARTESIAN_POINT('Ctrl Pts',(-174.150594139555,5.81615726515733,
128.632384875785));
#236582=CARTESIAN_POINT('Ctrl Pts',(-174.429041763368,1.31643036424716,
124.737056846366));
#236583=CARTESIAN_POINT('Ctrl Pts',(-174.707489387181,-4.39303173020782,
126.417284578411));
#236584=CARTESIAN_POINT('Ctrl Pts',(-174.985937010994,-6.06551227613263,
132.129020869861));
#236585=CARTESIAN_POINT('Ctrl Pts',(-175.264384634806,-2.16408335703982,
136.623459102702));
#236586=CARTESIAN_POINT('Ctrl Pts',(-175.542832258619,3.72603244582337,
135.770430106468));
#236587=CARTESIAN_POINT('Ctrl Pts',(-175.821279882432,6.19210645777918,
130.353825855915));
#236588=CARTESIAN_POINT('Ctrl Pts',(-176.099727506245,2.96793713625374,
125.351241041473));
#236589=CARTESIAN_POINT('Ctrl Pts',(-176.378175130058,-2.98362142169932,
125.359806717758));
#236590=CARTESIAN_POINT('Ctrl Pts',(-176.656622753871,-6.19337765112022,
130.371651446723));
#236591=CARTESIAN_POINT('Ctrl Pts',(-176.935070377684,-3.71172238248064,
135.781134764673));
#236592=CARTESIAN_POINT('Ctrl Pts',(-177.213518001496,2.18082442793968,
136.617205770365));
#236593=CARTESIAN_POINT('Ctrl Pts',(-177.49196562531,6.06930012827989,132.111556053907));
#236594=CARTESIAN_POINT('Ctrl Pts',(-177.770413249122,4.38038551252508,
126.404657591498));
#236595=CARTESIAN_POINT('Ctrl Pts',(-178.048860872936,-1.33388939551094,
124.740871272604));
#236596=CARTESIAN_POINT('Ctrl Pts',(-178.327308496748,-5.82238511319243,
128.649135443807));
#236597=CARTESIAN_POINT('Ctrl Pts',(-178.605756120561,-4.96039335117553,
134.537946261091));
#236598=CARTESIAN_POINT('Ctrl Pts',(-178.884203744374,0.459957571884186,
136.995774267775));
#236599=CARTESIAN_POINT('Ctrl Pts',(-179.162651368187,5.45762995655925,
133.763995597288));
#236600=CARTESIAN_POINT('Ctrl Pts',(-179.441098991999,5.44000703120181,
127.812456966643));
#236601=CARTESIAN_POINT('Ctrl Pts',(-179.719546615813,0.423283403288203,
124.610331628578));
#236602=CARTESIAN_POINT('Ctrl Pts',(-179.997994239625,-4.98241699370369,
127.100216336253));
#236603=CARTESIAN_POINT('Ctrl Pts',(-180.276441863438,-5.80951957808352,
132.994028680947));
#236604=CARTESIAN_POINT('Ctrl Pts',(-180.554889487251,-1.29795748101432,
136.875643046625));
#236605=CARTESIAN_POINT('Ctrl Pts',(-180.833337111064,4.40636413235919,
135.178045458633));
#236606=CARTESIAN_POINT('Ctrl Pts',(-181.111784734877,6.06145237094964,
129.461245168083));
#236607=CARTESIAN_POINT('Ctrl Pts',(-181.39023235869,2.14636199904753,124.97870236077));
#236608=CARTESIAN_POINT('Ctrl Pts',(-181.668679982503,-3.74113019436597,
125.849654892224));
#236609=CARTESIAN_POINT('Ctrl Pts',(-181.947127606316,-6.19070650352801,
131.273739934436));
#236610=CARTESIAN_POINT('Ctrl Pts',(-182.225575230128,-2.95132596877351,
136.266488314898));
#236611=CARTESIAN_POINT('Ctrl Pts',(-182.504022853942,3.00017895099442,
136.239808181284));
#236612=CARTESIAN_POINT('Ctrl Pts',(-182.782470477755,6.19466598168877,
131.218217272988));
#236613=CARTESIAN_POINT('Ctrl Pts',(-183.060918101567,3.6965576014681,125.81631231638));
#236614=CARTESIAN_POINT('Ctrl Pts',(-183.33936572538,-2.19850662762309,
124.998180068855));
#236615=CARTESIAN_POINT('Ctrl Pts',(-183.617813349193,-6.07325066894868,
129.515644097905));
#236616=CARTESIAN_POINT('Ctrl Pts',(-183.896260973006,-4.36697404029963,
135.217375651221));
#236617=CARTESIAN_POINT('Ctrl Pts',(-184.174708596819,1.35233839284232,
136.863761976378));
#236618=CARTESIAN_POINT('Ctrl Pts',(-184.453156220632,5.8289179083658,132.941854470998));
#236619=CARTESIAN_POINT('Ctrl Pts',(-184.731603844444,4.94900662457131,
127.055694536694));
#236620=CARTESIAN_POINT('Ctrl Pts',(-185.010051468258,-0.478799974789776,
124.614375598192));
#236621=CARTESIAN_POINT('Ctrl Pts',(-185.28849909207,-5.46661278799793,
127.861350494915));
#236622=CARTESIAN_POINT('Ctrl Pts',(-185.566946715884,-5.43087550791776,
133.812807920317));
#236623=CARTESIAN_POINT('Ctrl Pts',(-185.845394339696,-0.404428949079144,
136.999649245311));
#236624=CARTESIAN_POINT('Ctrl Pts',(-186.123841963509,4.99366805651034,
134.493322978084));
#236625=CARTESIAN_POINT('Ctrl Pts',(-186.402289587322,5.80282807241402,
128.59702051737));
#236626=CARTESIAN_POINT('Ctrl Pts',(-186.680737211135,1.27947257368013,
124.729155774178));
#236627=CARTESIAN_POINT('Ctrl Pts',(-186.959184834948,-4.41965571455532,
126.444107491802));
#236628=CARTESIAN_POINT('Ctrl Pts',(-187.237632458761,-6.0573363132998,
132.165918821797));
#236629=CARTESIAN_POINT('Ctrl Pts',(-187.516080082574,-2.12862075745111,
136.636524677919));
#236630=CARTESIAN_POINT('Ctrl Pts',(-187.794527706387,3.75619328558978,
135.74765667963));
#236631=CARTESIAN_POINT('Ctrl Pts',(-188.072975330199,6.18924919941703,
130.316141093742));
#236632=CARTESIAN_POINT('Ctrl Pts',(-188.351422954013,2.93468746061294,
125.333275399398));
#236633=CARTESIAN_POINT('Ctrl Pts',(-188.629870577825,-3.01670868704181,
125.378069743179));
#236634=CARTESIAN_POINT('Ctrl Pts',(-188.908318201638,-6.19589692571743,
130.409360311474));
#236635=CARTESIAN_POINT('Ctrl Pts',(-189.186765825451,-3.68135857605119,
135.80363686423));
#236636=CARTESIAN_POINT('Ctrl Pts',(-189.465213449264,2.21616846064164,
136.603822774524));
#236637=CARTESIAN_POINT('Ctrl Pts',(-189.743661073077,6.07714494785282,
132.07458628205));
#236638=CARTESIAN_POINT('Ctrl Pts',(-190.02210869689,4.35352211302309,126.378074457888));
#236639=CARTESIAN_POINT('Ctrl Pts',(-190.300556320702,-1.37077486229612,
124.749103378371));
#236640=CARTESIAN_POINT('Ctrl Pts',(-190.579003944516,-5.83539670523986,
128.684617885911));
#236641=CARTESIAN_POINT('Ctrl Pts',(-190.857451568328,-4.93757405104588,
134.568072408653));
#236642=CARTESIAN_POINT('Ctrl Pts',(-191.135899192141,0.497637942157669,
136.992859662928));
#236643=CARTESIAN_POINT('Ctrl Pts',(-191.414346815954,5.47554497748281,
133.730718619501));
#236644=CARTESIAN_POINT('Ctrl Pts',(-191.692794439767,5.42169367374449,
127.779397532831));
#236645=CARTESIAN_POINT('Ctrl Pts',(-191.97124206358,0.385570748295746,
124.60786974337));
#236646=CARTESIAN_POINT('Ctrl Pts',(-192.249689687393,-5.00487285865859,
127.130614351886));
#236647=CARTESIAN_POINT('Ctrl Pts',(-192.528137311206,-5.79608281013753,
133.029352306079));
#236648=CARTESIAN_POINT('Ctrl Pts',(-192.806584935019,-1.26097581348702,
136.883431595415));
#236649=CARTESIAN_POINT('Ctrl Pts',(-193.085032558831,4.43290635366497,
135.151141635234));
#236650=CARTESIAN_POINT('Ctrl Pts',(-193.363480182644,6.05316414131348,
129.424372271875));
#236651=CARTESIAN_POINT('Ctrl Pts',(-193.641927806457,2.11085979660312,
124.965744782026));
#236652=CARTESIAN_POINT('Ctrl Pts',(-193.92037543027,-3.77122157995168,
125.872520012798));
#236653=CARTESIAN_POINT('Ctrl Pts',(-194.198823054083,-6.1877345589472,
131.311415825543));
#236654=CARTESIAN_POINT('Ctrl Pts',(-194.477270677896,-2.91802176590892,
136.284352673182));
#236655=CARTESIAN_POINT('Ctrl Pts',(-194.755718301709,3.03321047671203,
136.221444534203));
#236656=CARTESIAN_POINT('Ctrl Pts',(-195.034165925522,6.19707047180361,
131.180500915096));
#236657=CARTESIAN_POINT('Ctrl Pts',(-195.312613549334,3.66612544703105,
125.793902738034));
#236658=CARTESIAN_POINT('Ctrl Pts',(-195.591061173148,-2.23380976337827,
125.011670577786));
#236659=CARTESIAN_POINT('Ctrl Pts',(-195.86950879696,-6.08098292891658,
129.552637575454));
#236660=CARTESIAN_POINT('Ctrl Pts',(-196.147956420774,-4.3400298553121,
135.243876898752));
#236661=CARTESIAN_POINT('Ctrl Pts',(-196.426404044586,1.38919863307876,
136.855417642068));
#236662=CARTESIAN_POINT('Ctrl Pts',(-196.704851668399,5.84182144379631,
132.906332590435));
#236663=CARTESIAN_POINT('Ctrl Pts',(-196.983299292212,4.92609573650846,
127.025637982775));
#236664=CARTESIAN_POINT('Ctrl Pts',(-197.261746916025,-0.516471299475173,
124.617404875624));
#236665=CARTESIAN_POINT('Ctrl Pts',(-197.540194539838,-5.48442644226676,
127.894681845726));
#236666=CARTESIAN_POINT('Ctrl Pts',(-197.81864216365,-5.41246161374207,
133.845811461438));
#236667=CARTESIAN_POINT('Ctrl Pts',(-198.097089787464,-0.36670897563802,
137.001996334766));
#236668=CARTESIAN_POINT('Ctrl Pts',(-198.375537411276,5.01603129634849,
134.462856755322));
#236669=CARTESIAN_POINT('Ctrl Pts',(-198.65398503509,5.78928385374183,128.561737952753));
#236670=CARTESIAN_POINT('Ctrl Pts',(-198.932432658902,1.24246737178614,
124.721479820939));
#236671=CARTESIAN_POINT('Ctrl Pts',(-199.210880282716,-4.44611592693577,
126.471091975977));
#236672=CARTESIAN_POINT('Ctrl Pts',(-199.489327906528,-6.04893589364168,
132.202766320694));
#236673=CARTESIAN_POINT('Ctrl Pts',(-199.767775530341,-2.09307928103787,
136.649374140152));
#236674=CARTESIAN_POINT('Ctrl Pts',(-200.046223154153,3.7862149382325,135.724700077139));
#236675=CARTESIAN_POINT('Ctrl Pts',(-200.324670777967,6.18616259614969,
130.278474422724));
#236676=CARTESIAN_POINT('Ctrl Pts',(-200.603118401779,2.90132903904936,
125.315512490399));
#236677=CARTESIAN_POINT('Ctrl Pts',(-200.881566025592,-3.04968416713424,
125.396533841802));
#236678=CARTESIAN_POINT('Ctrl Pts',(-201.160013649405,-6.1981866090755,
130.447083813107));
#236679=CARTESIAN_POINT('Ctrl Pts',(-201.438461273218,-3.65085835552605,
135.825953713766));
#236680=CARTESIAN_POINT('Ctrl Pts',(-201.716908897031,2.2514303724059,136.590224877478));
#236681=CARTESIAN_POINT('Ctrl Pts',(-201.995356520844,6.08476457658541,
132.037569441512));
#236682=CARTESIAN_POINT('Ctrl Pts',(-202.273804144657,4.32649739215744,
126.35165534194));
#236683=CARTESIAN_POINT('Ctrl Pts',(-202.55225176847,-1.40760953451491,
124.757559863922));
#236684=CARTESIAN_POINT('Ctrl Pts',(-202.830699392283,-5.84819206451709,
128.720178875862));
#236685=CARTESIAN_POINT('Ctrl Pts',(-203.109147016096,-4.91457178729319,
134.59805909049));
#236686=CARTESIAN_POINT('Ctrl Pts',(-203.387594639908,0.535299872273523,
136.989715740974));
#236687=CARTESIAN_POINT('Ctrl Pts',(-203.666042263721,5.49325710007376,
133.697333204442));
#236688=CARTESIAN_POINT('Ctrl Pts',(-203.944489887534,5.40317941343439,
127.746450190138));
#236689=CARTESIAN_POINT('Ctrl Pts',(-204.222937511347,0.347843805837959,
124.605637471411));
#236690=CARTESIAN_POINT('Ctrl Pts',(-204.50138513516,-5.0271432662092,127.161148499539));
#236691=CARTESIAN_POINT('Ctrl Pts',(-204.779832758973,-5.78243126621161,
133.064593483327));
#236692=CARTESIAN_POINT('Ctrl Pts',(-205.058280382786,-1.22394742003769,
136.890994881994));
#236693=CARTESIAN_POINT('Ctrl Pts',(-205.336728006599,4.45928431199552,
135.124076740266));
#236694=CARTESIAN_POINT('Ctrl Pts',(-205.615175630412,6.04465160945437,
129.387550511641));
#236695=CARTESIAN_POINT('Ctrl Pts',(-205.893623254225,2.07527937547198,
124.953003555339));
#236696=CARTESIAN_POINT('Ctrl Pts',(-206.172070878037,-3.80117322153507,
125.89556788454));
#236697=CARTESIAN_POINT('Ctrl Pts',(-206.45051850185,-6.18453332558722,
131.349072927534));
#236698=CARTESIAN_POINT('Ctrl Pts',(-206.728966125663,-2.8846094346739,
136.302013968343));
#236699=CARTESIAN_POINT('Ctrl Pts',(-207.007413749476,3.06612960569919,
136.202880155086));
#236700=CARTESIAN_POINT('Ctrl Pts',(-207.285861373289,6.19924532719362,
131.142770619188));
#236701=CARTESIAN_POINT('Ctrl Pts',(-207.564308997102,3.63555744296752,
125.771678824048));
#236702=CARTESIAN_POINT('Ctrl Pts',(-207.842756620915,-2.26903012449045,
125.025375736976));
#236703=CARTESIAN_POINT('Ctrl Pts',(-208.121204244728,-6.08848985582611,
129.58967743606));
#236704=CARTESIAN_POINT('Ctrl Pts',(-208.399651868541,-4.31292484892225,
135.270213638376));
#236705=CARTESIAN_POINT('Ctrl Pts',(-208.678099492353,1.42600739604885,
136.846849083615));
#236706=CARTESIAN_POINT('Ctrl Pts',(-208.956547116166,5.85450850838505,
132.870732820528));
#236707=CARTESIAN_POINT('Ctrl Pts',(-209.234994739979,4.90300231015654,
126.995721450812));
#236708=CARTESIAN_POINT('Ctrl Pts',(-209.513442363792,-0.554123486127181,
124.620663412976));
#236709=CARTESIAN_POINT('Ctrl Pts',(-209.791889987605,-5.50203686909699,
127.928121015754));
#236710=CARTESIAN_POINT('Ctrl Pts',(-210.070337611418,-5.393847158811,133.878702300482));
#236711=CARTESIAN_POINT('Ctrl Pts',(-210.348785235231,-0.328975413660277,
137.004113768549));
#236712=CARTESIAN_POINT('Ctrl Pts',(-210.627232859043,5.03820866530154,
134.432254965643));
#236713=CARTESIAN_POINT('Ctrl Pts',(-210.905680482857,5.77552511102812,
128.526538489345));
#236714=CARTESIAN_POINT('Ctrl Pts',(-211.184128106669,1.20541612980698,
124.714029271085));
#236715=CARTESIAN_POINT('Ctrl Pts',(-211.462575730482,-4.47241138685473,
126.498237031013));
#236716=CARTESIAN_POINT('Ctrl Pts',(-211.741023354295,-6.04031132844015,
132.239562001151));
#236717=CARTESIAN_POINT('Ctrl Pts',(-212.019470978108,-2.05746024480169,
136.66200701326));
#236718=CARTESIAN_POINT('Ctrl Pts',(-212.297918601921,3.81609629128846,
135.701561149659));
#236719=CARTESIAN_POINT('Ctrl Pts',(-212.576366225734,6.1828467623524,130.240827238612));
#236720=CARTESIAN_POINT('Ctrl Pts',(-212.854813849547,2.86786310767097,
125.297952972686));
#236721=CARTESIAN_POINT('Ctrl Pts',(-213.133261473359,-3.0825466400586,
125.415198329437));
#236722=CARTESIAN_POINT('Ctrl Pts',(-213.411709097173,-6.20024661634941,
130.484820553763));
#236723=CARTESIAN_POINT('Ctrl Pts',(-213.690156720985,-3.62022285110177,
135.848084486325));
#236724=CARTESIAN_POINT('Ctrl Pts',(-213.968604344798,2.28660885659016,
136.576412583105));
#236725=CARTESIAN_POINT('Ctrl Pts',(-214.247051968611,6.09215873212836,
132.00050690397));
#236726=CARTESIAN_POINT('Ctrl Pts',(-214.525499592424,4.29931235134063,
126.325401222624));
#236727=CARTESIAN_POINT('Ctrl Pts',(-214.803947216237,-1.44439204724454,
124.766240415898));
#236728=CARTESIAN_POINT('Ctrl Pts',(-215.08239484005,-5.86077071688603,
128.755817095934));
#236729=CARTESIAN_POINT('Ctrl Pts',(-215.360842463863,-4.89138741227638,
134.627905195436));
#236730=CARTESIAN_POINT('Ctrl Pts',(-215.639290087675,0.572941966656434,
136.986342618411));
#236731=CARTESIAN_POINT('Ctrl Pts',(-215.917737711489,5.51076566800256,
133.66384058922));
#236732=CARTESIAN_POINT('Ctrl Pts',(-216.196185335301,5.38446493632399,
127.713616159441));
#236733=CARTESIAN_POINT('Ctrl Pts',(-216.474632959115,0.310103973899474,
124.603634895418));
#236734=CARTESIAN_POINT('Ctrl Pts',(-216.753080582927,-5.04922739111732,
127.191817647757));
#236735=CARTESIAN_POINT('Ctrl Pts',(-217.031528206741,-5.76856545216855,
133.099750906814));
#236736=CARTESIAN_POINT('Ctrl Pts',(-217.309975830553,-1.18687367276612,
136.898332626102));
#236737=CARTESIAN_POINT('Ctrl Pts',(-217.588423454366,4.48549702990607,
135.096851776628));
#236738=CARTESIAN_POINT('Ctrl Pts',(-217.866871078179,6.03591509080661,
129.350781251827));
#236739=CARTESIAN_POINT('Ctrl Pts',(-218.145318701992,2.03962205410111,
124.94047915284));
#236740=CARTESIAN_POINT('Ctrl Pts',(-218.423766325804,-3.83098400924668,
125.9187976534));
#236741=CARTESIAN_POINT('Ctrl Pts',(-218.702213949618,-6.18110292207006,
131.386709845009));
#236742=CARTESIAN_POINT('Ctrl Pts',(-218.98066157343,-2.85109021317626,
136.319471545938));
#236743=CARTESIAN_POINT('Ctrl Pts',(-219.259109197243,3.09893511812703,
136.18411573184));
#236744=CARTESIAN_POINT('Ctrl Pts',(-219.537556821056,6.20119046726778,
131.105027783371));
#236745=CARTESIAN_POINT('Ctrl Pts',(-219.816004444869,3.6048547219858,125.749641397935));
#236746=CARTESIAN_POINT('Ctrl Pts',(-220.094452068682,-2.30416640585769,
125.039295038577));
#236747=CARTESIAN_POINT('Ctrl Pts',(-220.372899692494,-6.09577117150464,
129.626762307198));
#236748=CARTESIAN_POINT('Ctrl Pts',(-220.651347316308,-4.28566002551621,
135.296384894171));
#236749=CARTESIAN_POINT('Ctrl Pts',(-220.929794940121,1.46276331779004,
136.83805661853));
#236750=CARTESIAN_POINT('Ctrl Pts',(-221.208242563933,5.86697863200795,
132.835056480438));
#236751=CARTESIAN_POINT('Ctrl Pts',(-221.486690187747,4.87972720125093,
126.965946049375));
#236752=CARTESIAN_POINT('Ctrl Pts',(-221.765137811559,-0.591755139529082,
124.624151089502));
#236753=CARTESIAN_POINT('Ctrl Pts',(-222.043585435373,-5.51944341592756,
127.961666765899));
#236754=CARTESIAN_POINT('Ctrl Pts',(-222.322033059185,-5.37503283288975,
133.911479218663));
#236755=CARTESIAN_POINT('Ctrl Pts',(-222.600480682998,-0.29122966137826,
137.006001468201));
#236756=CARTESIAN_POINT('Ctrl Pts',(-222.878928306811,5.06019934158045,
134.401518743003));
#236757=CARTESIAN_POINT('Ctrl Pts',(-223.157375930624,5.7615523541068,128.491423431472));
#236758=CARTESIAN_POINT('Ctrl Pts',(-223.435823554437,1.16832022068962,
124.706804400699));
#236759=CARTESIAN_POINT('Ctrl Pts',(-223.71427117825,-4.49854111992577,
126.525541651043));
#236760=CARTESIAN_POINT('Ctrl Pts',(-223.992718802062,-6.03146293728042,
132.276304499695));
#236761=CARTESIAN_POINT('Ctrl Pts',(-224.271166425875,-2.02176496861996,
136.674422829126));
#236762=CARTESIAN_POINT('Ctrl Pts',(-224.549614049688,3.84583623749284,
135.678240754614));
#236763=CARTESIAN_POINT('Ctrl Pts',(-224.828061673501,6.1793018208946,130.203200936436));
#236764=CARTESIAN_POINT('Ctrl Pts',(-225.106509297314,2.83429090657077,
125.280597496933));
#236765=CARTESIAN_POINT('Ctrl Pts',(-225.384956921127,-3.11529488808334,
125.434062514461));
#236766=CARTESIAN_POINT('Ctrl Pts',(-225.66340454494,-6.20207687120481,
130.522569135094));
#236767=CARTESIAN_POINT('Ctrl Pts',(-225.941852168753,-3.5894531979886,
135.87002836184));
#236768=CARTESIAN_POINT('Ctrl Pts',(-226.220299792565,2.32170260964191,
136.562386403224));
#236769=CARTESIAN_POINT('Ctrl Pts',(-226.498747416378,6.09932714048972,
131.963400042786));
#236770=CARTESIAN_POINT('Ctrl Pts',(-226.777195040191,4.27196799792278,
126.299313072794));
#236771=CARTESIAN_POINT('Ctrl Pts',(-227.055642664004,-1.48112103749588,
124.775144712639));
#236772=CARTESIAN_POINT('Ctrl Pts',(-227.334090287817,-5.87313219624144,
128.79153122554));
#236773=CARTESIAN_POINT('Ctrl Pts',(-227.61253791163,-4.8680217850994,134.65760961753));
#236774=CARTESIAN_POINT('Ctrl Pts',(-227.890985535443,0.610562830463375,
136.982740420231));
#236775=CARTESIAN_POINT('Ctrl Pts',(-228.169433159256,5.52807003248314,
133.630242014917));
#236776=CARTESIAN_POINT('Ctrl Pts',(-228.447880783069,5.36555093588535,
127.680896657417));
#236777=CARTESIAN_POINT('Ctrl Pts',(-228.726328406882,0.272352650944771,
124.601862089598));
#236778=CARTESIAN_POINT('Ctrl Pts',(-229.004776030695,-5.07112441504767,
127.222620660081));
#236779=CARTESIAN_POINT('Ctrl Pts',(-229.283223654507,-5.75448588181141,
133.134823273769));
#236780=CARTESIAN_POINT('Ctrl Pts',(-229.561671278321,-1.14975594545406,
136.905444555836));
#236781=CARTESIAN_POINT('Ctrl Pts',(-229.840118902133,4.51154353607471,
135.069467753152));
#236782=CARTESIAN_POINT('Ctrl Pts',(-230.118566525947,6.0269549091058,129.314065854931));
#236783=CARTESIAN_POINT('Ctrl Pts',(-230.397014149759,2.00388915378425,
124.928172038625));
#236784=CARTESIAN_POINT('Ctrl Pts',(-230.675461773572,-3.86065283843716,
125.942208458593));
#236785=CARTESIAN_POINT('Ctrl Pts',(-230.953909397385,-6.17744347551146,
131.424325183319));
#236786=CARTESIAN_POINT('Ctrl Pts',(-231.232357021197,-2.81746534348149,
136.33672475907));
#236787=CARTESIAN_POINT('Ctrl Pts',(-231.510804645011,3.13162579837364,
136.165151959792));
#236788=CARTESIAN_POINT('Ctrl Pts',(-231.789252268823,6.20290581994918,
131.067273806224));
#236789=CARTESIAN_POINT('Ctrl Pts',(-232.067699892636,3.57401842178686,
125.727791276302));
#236790=CARTESIAN_POINT('Ctrl Pts',(-232.346147516449,-2.33921730549066,
125.053427966802));
#236791=CARTESIAN_POINT('Ctrl Pts',(-232.624595140262,-6.10282660614105,
129.663890814674));
#236792=CARTESIAN_POINT('Ctrl Pts',(-232.903042764075,-4.25823639540172,
135.322389696357));
#236793=CARTESIAN_POINT('Ctrl Pts',(-233.181490387888,1.499465036299,136.829040572621));
#236794=CARTESIAN_POINT('Ctrl Pts',(-233.459938011701,5.87923135258013,
132.799304892167));
#236795=CARTESIAN_POINT('Ctrl Pts',(-233.738385635514,4.85627127225937,
126.9363128818));
#236796=CARTESIAN_POINT('Ctrl Pts',(-234.016833259326,-0.629364865227224,
124.627867775965));
#236797=CARTESIAN_POINT('Ctrl Pts',(-234.29528088314,-5.53664543775268,
127.99531785311));
#236798=CARTESIAN_POINT('Ctrl Pts',(-234.573728506952,-5.35601933315035,
133.944141001422));
#236799=CARTESIAN_POINT('Ctrl Pts',(-234.852176130765,-0.253473117473377,
137.007659363768));
#236800=CARTESIAN_POINT('Ctrl Pts',(-235.130623754578,5.08200251031112,
134.370649226346));
#236801=CARTESIAN_POINT('Ctrl Pts',(-235.409071378391,5.74736610074488,
128.456394080338));
#236802=CARTESIAN_POINT('Ctrl Pts',(-235.687519002204,1.13118101903705,
124.699805477501));
#236803=CARTESIAN_POINT('Ctrl Pts',(-235.965966626017,-4.52450415790052,
126.553004824284));
#236804=CARTESIAN_POINT('Ctrl Pts',(-236.24441424983,-6.0223910480441,132.312992454817));
#236805=CARTESIAN_POINT('Ctrl Pts',(-236.522861873642,-1.98599477519336,
136.686621127679));
#236806=CARTESIAN_POINT('Ctrl Pts',(-236.801309497456,3.87543367482126,
135.654739756147));
#236807=CARTESIAN_POINT('Ctrl Pts',(-237.079757121268,6.1755279031354,130.165596910454));
#236808=CARTESIAN_POINT('Ctrl Pts',(-237.358204745081,2.80061367977841,
125.263446706254));
#236809=CARTESIAN_POINT('Ctrl Pts',(-237.636652368894,-3.14792769771062,
125.453125697856));
#236810=CARTESIAN_POINT('Ctrl Pts',(-237.915099992707,-6.20367730582095,
130.560328158313));
#236811=CARTESIAN_POINT('Ctrl Pts',(-238.19354761652,-3.55855053636696,
135.891784527174));
#236812=CARTESIAN_POINT('Ctrl Pts',(-238.471995240333,2.35671033115007,
136.54814685758));
#236813=CARTESIAN_POINT('Ctrl Pts',(-238.750442864146,6.10626953604027,
131.92625023297));
#236814=CARTESIAN_POINT('Ctrl Pts',(-239.028890487959,4.24446534516054,
126.273391859158));
#236815=CARTESIAN_POINT('Ctrl Pts',(-239.307338111771,-1.51779514426229,
124.784272424193));
#236816=CARTESIAN_POINT('Ctrl Pts',(-239.585785735585,-5.88527604452282,
128.827319941278));
#236817=CARTESIAN_POINT('Ctrl Pts',(-239.864233359397,-4.84447577158576,
134.687171256065));
#236818=CARTESIAN_POINT('Ctrl Pts',(-240.14268098321,0.648161069640796,
136.978909279916));
#236819=CARTESIAN_POINT('Ctrl Pts',(-240.421128607023,5.54516955229552,
133.596538726537));
#236820=CARTESIAN_POINT('Ctrl Pts',(-240.699576230836,5.34643811298351,
127.648292896498));
#236821=CARTESIAN_POINT('Ctrl Pts',(-240.978023854649,0.234591235861842,
124.600319119639));
#236822=CARTESIAN_POINT('Ctrl Pts',(-241.256471478461,-5.09283352659785,
127.253556395099));
#236823=CARTESIAN_POINT('Ctrl Pts',(-241.534919102275,-5.74019307686353,
133.169809284574));
#236824=CARTESIAN_POINT('Ctrl Pts',(-241.813366726087,-1.11259561351327,
136.912330407661));
#236825=CARTESIAN_POINT('Ctrl Pts',(-242.0918143499,4.53742286533832,135.041925684563));
#236826=CARTESIAN_POINT('Ctrl Pts',(-242.370261973713,6.01777139637409,
129.277405681456));
#236827=CARTESIAN_POINT('Ctrl Pts',(-242.648709597526,1.96808199861856,
124.916082668738));
#236828=CARTESIAN_POINT('Ctrl Pts',(-242.927157221339,-3.89017860971679,
125.965799432623));
#236829=CARTESIAN_POINT('Ctrl Pts',(-243.205604845152,-6.1735551215127,
131.461917548614));
#236830=CARTESIAN_POINT('Ctrl Pts',(-243.484052468965,-2.78373607157309,
136.353772968415));
#236831=CARTESIAN_POINT('Ctrl Pts',(-243.762500092778,3.16420043507544,
136.145989541648));
#236832=CARTESIAN_POINT('Ctrl Pts',(-244.040947716591,6.20439132167383,
131.029510086731));
#236833=CARTESIAN_POINT('Ctrl Pts',(-244.319395340403,3.54304968502077,
125.706129268813));
#236834=CARTESIAN_POINT('Ctrl Pts',(-244.597842964216,-2.37418152456686,
125.067773997952));
#236835=CARTESIAN_POINT('Ctrl Pts',(-244.876290588029,-6.10965589829292,
129.701061582678));
#236836=CARTESIAN_POINT('Ctrl Pts',(-245.154738211842,-4.23065497477177,
135.348227081313));
#236837=CARTESIAN_POINT('Ctrl Pts',(-245.433185835655,1.53611119157916,
136.819801279981));
#236838=CARTESIAN_POINT('Ctrl Pts',(-245.711633459468,5.89126621607239,
132.763479380503));
#236839=CARTESIAN_POINT('Ctrl Pts',(-245.990081083281,4.83263539234992,
126.906823046158));
#236840=CARTESIAN_POINT('Ctrl Pts',(-246.268528707094,-0.666951269578287,
124.631813334641));
#236841=CARTESIAN_POINT('Ctrl Pts',(-246.546976330906,-5.55364229714491,
128.029073030433));
#236842=CARTESIAN_POINT('Ctrl Pts',(-246.825423954719,-5.33680736414475,
133.976686438464));
#236843=CARTESIAN_POINT('Ctrl Pts',(-247.103871578532,-0.215707181029578,
137.009087393821));
#236844=CARTESIAN_POINT('Ctrl Pts',(-247.382319202345,5.10361736357064,
134.339647559554));
#236845=CARTESIAN_POINT('Ctrl Pts',(-247.660766826158,5.73296687661779,
128.421451733968));
#236846=CARTESIAN_POINT('Ctrl Pts',(-247.939214449971,1.09399990105564,
124.693032760838));
#236847=CARTESIAN_POINT('Ctrl Pts',(-248.217662073784,-4.55029953871062,
126.580625533077));
#236848=CARTESIAN_POINT('Ctrl Pts',(-248.496109697597,-6.01309599689209,
132.349624507031));
#236849=CARTESIAN_POINT('Ctrl Pts',(-248.77455732141,-1.95015099000055,
136.698601456905));
#236850=CARTESIAN_POINT('Ctrl Pts',(-249.053004945222,3.90488750652966,
135.631059025098));
#236851=CARTESIAN_POINT('Ctrl Pts',(-249.331452569036,6.17152514891849,
130.128016554096));
#236852=CARTESIAN_POINT('Ctrl Pts',(-249.609900192848,2.76683267521693,
125.246501236177));
#236853=CARTESIAN_POINT('Ctrl Pts',(-249.888347816661,-3.18044385971988,
125.472387173231));
#236854=CARTESIAN_POINT('Ctrl Pts',(-250.166795440474,-6.20504786089197,
130.598096224241));
#236855=CARTESIAN_POINT('Ctrl Pts',(-250.445243064287,-3.5275160113489,
135.913352176149));
#236856=CARTESIAN_POINT('Ctrl Pts',(-250.7236906881,2.39163072389511,136.533694473816));
#236857=CARTESIAN_POINT('Ctrl Pts',(-251.002138311913,6.11298566151878,
131.889058851139));
#236858=CARTESIAN_POINT('Ctrl Pts',(-251.280585935725,4.21680541219097,
126.247638542206));
#236859=CARTESIAN_POINT('Ctrl Pts',(-251.559033559539,-1.5544130086051,
124.793623212388));
#236860=CARTESIAN_POINT('Ctrl Pts',(-251.837481183351,-5.89720181167361,
128.863181916876));
#236861=CARTESIAN_POINT('Ctrl Pts',(-252.115928807165,-4.82075024435922,
134.716589015834));
#236862=CARTESIAN_POINT('Ctrl Pts',(-252.394376430977,0.685735291195708,
136.974849339035));
#236863=CARTESIAN_POINT('Ctrl Pts',(-252.67282405479,5.56206359338632,133.562731973716));
#236864=CARTESIAN_POINT('Ctrl Pts',(-252.951271678603,5.32712717665345,
127.615806083426));
#236865=CARTESIAN_POINT('Ctrl Pts',(-253.229719302416,0.196821126400439,
124.599006045371));
#236866=CARTESIAN_POINT('Ctrl Pts',(-253.508166926229,-5.11435391846912,
127.284623701469));
#236867=CARTESIAN_POINT('Ctrl Pts',(-253.786614550041,-5.72568757235024,
133.204707652256));
#236868=CARTESIAN_POINT('Ctrl Pts',(-254.065062173855,-1.07539404373626,
136.918989908584));
#236869=CARTESIAN_POINT('Ctrl Pts',(-254.343509797667,4.56313403947717,
135.014226625117));
#236870=CARTESIAN_POINT('Ctrl Pts',(-254.621957421481,6.00836492926231,
129.240802026269));
#236871=CARTESIAN_POINT('Ctrl Pts',(-254.900405045293,1.9322018468105,124.904211611225));
#236872=CARTESIAN_POINT('Ctrl Pts',(-255.178852669106,-3.91956009939235,
125.989569474605));
#236873=CARTESIAN_POINT('Ctrl Pts',(-255.457300292919,-6.16943824888009,
131.499485975975));
#236874=CARTESIAN_POINT('Ctrl Pts',(-255.735747916732,-2.74990318521692,
136.370614733943));
#236875=CARTESIAN_POINT('Ctrl Pts',(-256.014195540545,3.19665694865877,
136.126630713714));
#236876=CARTESIAN_POINT('Ctrl Pts',(-256.292643164358,6.20564856486739,
130.991735142402));
#236877=CARTESIAN_POINT('Ctrl Pts',(-256.571090788171,3.51194654848645,
125.68466161966));
#236878=CARTESIAN_POINT('Ctrl Pts',(-256.849538411983,-2.40905189372645,
125.082322325773));
#236879=CARTESIAN_POINT('Ctrl Pts',(-257.127986035797,-6.11626988572704,
129.738292634474));
#236880=CARTESIAN_POINT('Ctrl Pts',(-257.406433659609,-4.20289584392431,
135.373859459261));
#236881=CARTESIAN_POINT('Ctrl Pts',(-257.684881283423,1.57266088340656,
136.810408252432));
#236882=CARTESIAN_POINT('Ctrl Pts',(-257.963328907235,5.90315744058412,
132.727450666138));
#236883=CARTESIAN_POINT('Ctrl Pts',(-258.241776531048,4.80867945501638,
126.87772425425));
#236884=CARTESIAN_POINT('Ctrl Pts',(-258.520224154861,-0.704246744852541,
124.635521896935));
#236885=CARTESIAN_POINT('Ctrl Pts',(-258.798671778674,-5.5709361272427,
128.063810879205));
#236886=CARTESIAN_POINT('Ctrl Pts',(-259.077119402487,-5.31644754243966,
134.007449313497));
#236887=CARTESIAN_POINT('Ctrl Pts',(-259.355567026299,-0.179733571114533,
137.013459703814));
#236888=CARTESIAN_POINT('Ctrl Pts',(-259.634014650113,5.12849404027147,
134.30227331953));
#236889=CARTESIAN_POINT('Ctrl Pts',(-259.866054336623,5.61428989304695,
129.384066440553));
#236890=CARTESIAN_POINT('Ctrl Pts',(-260.051696012132,3.39054283699284,
126.521203045511));
#236891=CARTESIAN_POINT('Ctrl Pts',(-260.144521813036,1.754921961264,125.780753115897));
#236892=CARTESIAN_POINT('Ctrl Pts',(-260.190939676638,0.892893391295023,
125.631947563271));
#236893=CARTESIAN_POINT('Ctrl Pts',(210.191733024964,-2.43880115184907,
125.780342085335));
#236894=CARTESIAN_POINT('Ctrl Pts',(210.145323348611,-3.27594855749458,
126.186716565447));
#236895=CARTESIAN_POINT('Ctrl Pts',(210.052505734956,-4.72940422381435,
127.426013481475));
#236896=CARTESIAN_POINT('Ctrl Pts',(209.866872246696,-6.15821517169733,
131.008352419918));
#236897=CARTESIAN_POINT('Ctrl Pts',(209.634832560185,-4.21099667891447,
135.892791108304));
#236898=CARTESIAN_POINT('Ctrl Pts',(209.356384936373,2.01508446636645,137.098708070195));
#236899=CARTESIAN_POINT('Ctrl Pts',(209.07793731256,6.37956871319657,132.510708806665));
#236900=CARTESIAN_POINT('Ctrl Pts',(208.799489688747,4.8866719183268,126.359661034021));
#236901=CARTESIAN_POINT('Ctrl Pts',(208.521042064934,-1.09954563679898,
124.290443595948));
#236902=CARTESIAN_POINT('Ctrl Pts',(208.242594441121,-6.07390144970816,
128.208589139036));
#236903=CARTESIAN_POINT('Ctrl Pts',(207.964146817309,-5.46739734855352,
134.511385201899));
#236904=CARTESIAN_POINT('Ctrl Pts',(207.685699193495,0.163779660617915,
137.407996874876));
#236905=CARTESIAN_POINT('Ctrl Pts',(207.407251569682,5.6442383477931,134.235982835808));
#236906=CARTESIAN_POINT('Ctrl Pts',(207.128803945869,5.93803043711477,127.910585036422));
#236907=CARTESIAN_POINT('Ctrl Pts',(206.850356322057,0.775002953389061,
124.244367681185));
#236908=CARTESIAN_POINT('Ctrl Pts',(206.571908698243,-5.10018277131114,
126.606494049502));
#236909=CARTESIAN_POINT('Ctrl Pts',(206.293461074431,-6.28856642889766,
132.82623846394));
#236910=CARTESIAN_POINT('Ctrl Pts',(206.015013450618,-1.69805588527783,
137.187984519302));
#236911=CARTESIAN_POINT('Ctrl Pts',(205.736565826805,4.45288036648484,135.683487507757));
#236912=CARTESIAN_POINT('Ctrl Pts',(205.458118202992,6.51183958365415,129.695313656966));
#236913=CARTESIAN_POINT('Ctrl Pts',(205.179670579179,2.58673502741873,124.726298504418));
#236914=CARTESIAN_POINT('Ctrl Pts',(204.901222955366,-3.71545195245463,
125.342726181157));
#236915=CARTESIAN_POINT('Ctrl Pts',(204.622775331554,-6.60332046735468,
130.978128730661));
#236916=CARTESIAN_POINT('Ctrl Pts',(204.344327707741,-3.42305986725146,
136.4538470632));
#236917=CARTESIAN_POINT('Ctrl Pts',(204.065880083927,2.90282542147133,136.737963244372));
#236918=CARTESIAN_POINT('Ctrl Pts',(203.787432460115,6.56115601364161,131.569388537382));
#236919=CARTESIAN_POINT('Ctrl Pts',(203.508984836302,4.1901047305044,125.69779051756));
#236920=CARTESIAN_POINT('Ctrl Pts',(203.230537212489,-2.03144808657932,
124.518880964767));
#236921=CARTESIAN_POINT('Ctrl Pts',(202.952089588676,-6.38619936200403,
129.116020142231));
#236922=CARTESIAN_POINT('Ctrl Pts',(202.673641964863,-4.87234540261322,
135.2646617407));
#236923=CARTESIAN_POINT('Ctrl Pts',(202.39519434105,1.1189559521872,137.314504502614));
#236924=CARTESIAN_POINT('Ctrl Pts',(202.116746717238,6.08199145217563,133.381843073553));
#236925=CARTESIAN_POINT('Ctrl Pts',(201.838299093424,5.45597392877388,127.080601183836));
#236926=CARTESIAN_POINT('Ctrl Pts',(201.559851469612,-0.183817095687214,
124.201312298284));
#236927=CARTESIAN_POINT('Ctrl Pts',(201.281403845799,-5.65468918935595,
127.389902241135));
#236928=CARTESIAN_POINT('Ctrl Pts',(201.002956221986,-5.92917816483575,
133.716212626452));
#236929=CARTESIAN_POINT('Ctrl Pts',(200.724508598173,-0.755042063338292,
137.366673267433));
#236930=CARTESIAN_POINT('Ctrl Pts',(200.44606097436,5.11294080853837,134.986689170007));
#236931=CARTESIAN_POINT('Ctrl Pts',(200.167613350547,6.2823808583988,128.763349450982));
#236932=CARTESIAN_POINT('Ctrl Pts',(199.889165726734,1.67861981076543,124.415599285115));
#236933=CARTESIAN_POINT('Ctrl Pts',(199.610718102921,-4.46771083782862,
125.938808675424));
#236934=CARTESIAN_POINT('Ctrl Pts',(199.332270479108,-6.50843348626435,
131.933222605136));
#236935=CARTESIAN_POINT('Ctrl Pts',(199.053822855296,-2.56822371547623,
136.890267516244));
#236936=CARTESIAN_POINT('Ctrl Pts',(198.775375231483,3.73205818513161,136.254661300547));
#236937=CARTESIAN_POINT('Ctrl Pts',(198.49692760767,6.60276093478139,130.610495019181));
#236938=CARTESIAN_POINT('Ctrl Pts',(198.218479983857,3.4058489481713,125.14448175187));
#236939=CARTESIAN_POINT('Ctrl Pts',(197.940032360044,-2.92087183683725,
124.879620661678));
#236940=CARTESIAN_POINT('Ctrl Pts',(197.661584736231,-6.56345409631434,
130.05930615131));
#236941=CARTESIAN_POINT('Ctrl Pts',(197.383137112418,-4.1745426838368,135.923660297497));
#236942=CARTESIAN_POINT('Ctrl Pts',(197.104689488605,2.05056951733907,137.083628129519));
#236943=CARTESIAN_POINT('Ctrl Pts',(196.826241864792,6.39130850797037,132.473255877329));
#236944=CARTESIAN_POINT('Ctrl Pts',(196.54779424098,4.85874721255563,126.329250411482));
#236945=CARTESIAN_POINT('Ctrl Pts',(196.269346617166,-1.13876540820057,
124.297652603739));
#236946=CARTESIAN_POINT('Ctrl Pts',(195.990898993354,-6.0898082506034,128.245401590344));
#236947=CARTESIAN_POINT('Ctrl Pts',(195.712451369541,-5.44461481437399,
134.544708910868));
#236948=CARTESIAN_POINT('Ctrl Pts',(195.434003745728,0.203913652044436,
137.406818876019));
#236949=CARTESIAN_POINT('Ctrl Pts',(195.155556121915,5.66505543396973,134.201592249669));
#236950=CARTESIAN_POINT('Ctrl Pts',(194.877108498102,5.92028802542049,127.874475717408));
#236951=CARTESIAN_POINT('Ctrl Pts',(194.59866087429,0.735065143658737,124.239780275557));
#236952=CARTESIAN_POINT('Ctrl Pts',(194.320213250476,-5.1256466951968,126.637613470433));
#236953=CARTESIAN_POINT('Ctrl Pts',(194.041765626664,-6.2761396229282,132.86448373661));
#236954=CARTESIAN_POINT('Ctrl Pts',(193.763318002851,-1.6591668436545,137.198201498994));
#236955=CARTESIAN_POINT('Ctrl Pts',(193.484870379038,4.48249921013125,135.656291847837));
#236956=CARTESIAN_POINT('Ctrl Pts',(193.206422755225,6.50496747206681,129.655694426079));
#236957=CARTESIAN_POINT('Ctrl Pts',(192.927975131412,2.54968841250072,124.710665118833));
#236958=CARTESIAN_POINT('Ctrl Pts',(192.649527507599,-3.74862973894988,
125.365444281348));
#236959=CARTESIAN_POINT('Ctrl Pts',(192.371079883787,-6.60214029104917,
131.018321851013));
#236960=CARTESIAN_POINT('Ctrl Pts',(192.092632259973,-3.38860644815819,
136.474579499726));
#236961=CARTESIAN_POINT('Ctrl Pts',(191.814184636161,2.93889117796205,136.720183001327));
#236962=CARTESIAN_POINT('Ctrl Pts',(191.535737012347,6.56569138435095,131.529434736241));
#236963=CARTESIAN_POINT('Ctrl Pts',(191.257289388535,4.15894196037717,125.672378777932));
#236964=CARTESIAN_POINT('Ctrl Pts',(190.978841764722,-2.06967194957323,
124.531363418996));
#236965=CARTESIAN_POINT('Ctrl Pts',(190.700394140909,-6.3963584469616,129.154926032595));
#236966=CARTESIAN_POINT('Ctrl Pts',(190.421946517096,-4.84510401107414,
135.294238450423));
#236967=CARTESIAN_POINT('Ctrl Pts',(190.143498893283,1.15856431450073,137.307572482581));
#236968=CARTESIAN_POINT('Ctrl Pts',(189.86505126947,6.09756863406271,133.344772510351));
#236969=CARTESIAN_POINT('Ctrl Pts',(189.586603645657,5.4332052617092,127.047458114672));
#236970=CARTESIAN_POINT('Ctrl Pts',(189.308156021844,-0.224008319322015,
124.202553584261));
#236971=CARTESIAN_POINT('Ctrl Pts',(189.029708398032,-5.67536919831109,
127.424387201254));
#236972=CARTESIAN_POINT('Ctrl Pts',(188.751260774218,-5.91134304125131,
133.752251266956));
#236973=CARTESIAN_POINT('Ctrl Pts',(188.472813150406,-0.71508141444371,
137.371147838333));
#236974=CARTESIAN_POINT('Ctrl Pts',(188.194365526593,5.13830509856852,134.955487759214));
#236975=CARTESIAN_POINT('Ctrl Pts',(187.91591790278,6.26984024615536,128.725144630756));
#236976=CARTESIAN_POINT('Ctrl Pts',(187.637470278967,1.63969850624965,124.405499418827));
#236977=CARTESIAN_POINT('Ctrl Pts',(187.359022655154,-4.49724605717418,
125.966095046791));
#236978=CARTESIAN_POINT('Ctrl Pts',(187.080575031341,-6.5014411967389,131.972820371883));
#236979=CARTESIAN_POINT('Ctrl Pts',(186.802127407528,-2.53112948956026,
136.905788265189));
#236980=CARTESIAN_POINT('Ctrl Pts',(186.523679783716,3.76516656597443,136.231842221641));
#236981=CARTESIAN_POINT('Ctrl Pts',(186.245232159903,6.60145848599114,130.570305731164));
#236982=CARTESIAN_POINT('Ctrl Pts',(185.96678453609,3.3713325565579,125.123854247073));
#236983=CARTESIAN_POINT('Ctrl Pts',(185.688336912277,-2.95688329360047,
124.897510609301));
#236984=CARTESIAN_POINT('Ctrl Pts',(185.409889288464,-6.5678678487195,130.099273563458));
#236985=CARTESIAN_POINT('Ctrl Pts',(185.131441664651,-4.14330270904733,
135.948977074923));
#236986=CARTESIAN_POINT('Ctrl Pts',(184.852994040838,2.08875520864929,137.071029390563));
#236987=CARTESIAN_POINT('Ctrl Pts',(184.574546417025,6.40134913096194,132.434319247607));
#236988=CARTESIAN_POINT('Ctrl Pts',(184.296098793212,4.831415925211,126.299756751549));
#236989=CARTESIAN_POINT('Ctrl Pts',(184.017651169399,-1.17835248801931,
124.304705146227));
#236990=CARTESIAN_POINT('Ctrl Pts',(183.739203545587,-6.10527253047917,
128.282519393244));
#236991=CARTESIAN_POINT('Ctrl Pts',(183.460755921774,-5.42174537657308,
134.577782526619));
#236992=CARTESIAN_POINT('Ctrl Pts',(183.182308297961,0.244100911417136,
137.405455267482));
#236993=CARTESIAN_POINT('Ctrl Pts',(182.903860674148,5.68563038680749,134.167044506474));
#236994=CARTESIAN_POINT('Ctrl Pts',(182.625413050335,5.90234329520773,127.838491527799));
#236995=CARTESIAN_POINT('Ctrl Pts',(182.346965426522,0.695091060812155,
124.23542735186));
#236996=CARTESIAN_POINT('Ctrl Pts',(182.068517802709,-5.15091590138369,
126.668891936874));
#236997=CARTESIAN_POINT('Ctrl Pts',(181.790070178896,-6.263482786439,132.902650210566));
#236998=CARTESIAN_POINT('Ctrl Pts',(181.511622555083,-1.62021497890189,
137.208182855437));
#236999=CARTESIAN_POINT('Ctrl Pts',(181.233174931271,4.51195124234396,135.628915707812));
#237000=CARTESIAN_POINT('Ctrl Pts',(180.954727307458,6.49785469294791,129.61611812487));
#237001=CARTESIAN_POINT('Ctrl Pts',(180.676279683645,2.51254711858197,124.695257343842));
#237002=CARTESIAN_POINT('Ctrl Pts',(180.397832059832,-3.78166851301026,
125.388364025079));
#237003=CARTESIAN_POINT('Ctrl Pts',(180.119384436019,-6.60071552592353,
131.058506988669));
#237004=CARTESIAN_POINT('Ctrl Pts',(179.840936812206,-3.35402743339335,
136.495101852955));
#237005=CARTESIAN_POINT('Ctrl Pts',(179.562489188393,2.97484801707599,136.702183530083));
#237006=CARTESIAN_POINT('Ctrl Pts',(179.28404156458,6.56998346925752,131.489454075275));
#237007=CARTESIAN_POINT('Ctrl Pts',(179.005593940767,4.12762507472721,125.647157201507));
#237008=CARTESIAN_POINT('Ctrl Pts',(178.727146316955,-2.10781911778238,
124.544078323705));
#237009=CARTESIAN_POINT('Ctrl Pts',(178.448698693142,-6.40628051373842,
129.193893042167));
#237010=CARTESIAN_POINT('Ctrl Pts',(178.170251069329,-4.81768308177075,
135.323648786705));
#237011=CARTESIAN_POINT('Ctrl Pts',(177.891803445516,1.19812974544141,137.300399483306));
#237012=CARTESIAN_POINT('Ctrl Pts',(177.613355821703,6.11291986848493,133.307607811431));
#237013=CARTESIAN_POINT('Ctrl Pts',(177.33490819789,5.41023526512845,127.014454258818));
#237014=CARTESIAN_POINT('Ctrl Pts',(177.056460574078,-0.264191242194762,
124.204039502676));
#237015=CARTESIAN_POINT('Ctrl Pts',(176.778012950264,-5.69583890440069,
127.458997407505));
#237016=CARTESIAN_POINT('Ctrl Pts',(176.499565326452,-5.89328887066216,
133.788180672302));
#237017=CARTESIAN_POINT('Ctrl Pts',(176.221117702638,-0.675094267951971,
137.375379074508));
#237018=CARTESIAN_POINT('Ctrl Pts',(175.942670078826,5.16347898681764,134.924132526884));
#237019=CARTESIAN_POINT('Ctrl Pts',(175.664222455013,6.25706730267374,128.687016856641));
#237020=CARTESIAN_POINT('Ctrl Pts',(175.3857748312,1.60071644210391,124.395636664696));
#237021=CARTESIAN_POINT('Ctrl Pts',(175.107327207387,-4.5266146294138,125.993560701866));
#237022=CARTESIAN_POINT('Ctrl Pts',(174.828879583574,-6.49420799391872,
132.012374840923));
#237023=CARTESIAN_POINT('Ctrl Pts',(174.550431959762,-2.49394147171037,
136.92108292349));
#237024=CARTESIAN_POINT('Ctrl Pts',(174.271984335948,3.79813542718566,136.208822025409));
#237025=CARTESIAN_POINT('Ctrl Pts',(173.993536712136,6.59991141772898,130.530125116137));
#237026=CARTESIAN_POINT('Ctrl Pts',(173.715089088322,3.33669123897678,125.103437235529));
#237027=CARTESIAN_POINT('Ctrl Pts',(173.43664146451,-2.99278518196597,124.915619437422));
#237028=CARTESIAN_POINT('Ctrl Pts',(173.158193840697,-6.5720382263662,130.139267102866));
#237029=CARTESIAN_POINT('Ctrl Pts',(172.879746216884,-4.11190920265221,
135.974103216695));
#237030=CARTESIAN_POINT('Ctrl Pts',(172.601298593071,2.12686350036709,137.058198437889));
#237031=CARTESIAN_POINT('Ctrl Pts',(172.322850969258,6.41115254960738,132.395322219168));
#237032=CARTESIAN_POINT('Ctrl Pts',(172.044403345445,4.80390560797255,126.270430011369));
#237033=CARTESIAN_POINT('Ctrl Pts',(171.765955721632,-1.21789590355323,
124.31199853584));
#237034=CARTESIAN_POINT('Ctrl Pts',(171.487508097819,-6.12051057723618,
128.319730643897));
#237035=CARTESIAN_POINT('Ctrl Pts',(171.209060474007,-5.39867503400336,
134.610716316833));
#237036=CARTESIAN_POINT('Ctrl Pts',(170.930612850193,0.284279125540913,
137.403847052956));
#237037=CARTESIAN_POINT('Ctrl Pts',(170.652165226381,5.70599465652041,134.13237215779));
#237038=CARTESIAN_POINT('Ctrl Pts',(170.373717602568,5.88417985149351,127.802617239562));
#237039=CARTESIAN_POINT('Ctrl Pts',(170.095269978755,0.655091221110643,
124.231317842401));
#237040=CARTESIAN_POINT('Ctrl Pts',(169.816822354942,-5.17599423848763,
126.700323644626));
#237041=CARTESIAN_POINT('Ctrl Pts',(169.538374731129,-6.25059385429175,
132.940738931629));
#237042=CARTESIAN_POINT('Ctrl Pts',(169.259927107316,-1.58120307648749,
137.217926915891));
#237043=CARTESIAN_POINT('Ctrl Pts',(168.981479483503,4.54123608254409,135.601360792124));
#237044=CARTESIAN_POINT('Ctrl Pts',(168.703031859691,6.49050113343381,129.576585854424));
#237045=CARTESIAN_POINT('Ctrl Pts',(168.424584235878,2.47531272130571,124.680075943919));
#237046=CARTESIAN_POINT('Ctrl Pts',(168.146136612065,-3.81456715595326,
125.411484460556));
#237047=CARTESIAN_POINT('Ctrl Pts',(167.867688988252,-6.59904616885666,
131.098682708838));
#237048=CARTESIAN_POINT('Ctrl Pts',(167.589241364439,-3.31932413390846,
136.515413333674));
#237049=CARTESIAN_POINT('Ctrl Pts',(167.310793740626,3.01069462210276,136.683965512842));
#237050=CARTESIAN_POINT('Ctrl Pts',(167.032346116813,6.57403210101054,131.449448027918));
#237051=CARTESIAN_POINT('Ctrl Pts',(166.753898493,4.09615523841214,125.622126727152));
#237052=CARTESIAN_POINT('Ctrl Pts',(166.475450869187,-2.14588817997888,
124.557025205477));
#237053=CARTESIAN_POINT('Ctrl Pts',(166.197003245374,-6.41596519343492,
129.232919728208));
#237054=CARTESIAN_POINT('Ctrl Pts',(165.918555621562,-4.79008363144905,
135.352891659104));
#237055=CARTESIAN_POINT('Ctrl Pts',(165.640107997748,1.23765077924384,137.292985770921));
#237056=CARTESIAN_POINT('Ctrl Pts',(165.361660373936,6.12804458641347,133.270350353765));
#237057=CARTESIAN_POINT('Ctrl Pts',(165.083212750123,5.38706479029029,126.981590839339));
#237058=CARTESIAN_POINT('Ctrl Pts',(164.80476512631,-0.304364375363971,
124.205769998417));
#237059=CARTESIAN_POINT('Ctrl Pts',(164.526317502497,-5.71609754908509,
127.493731577419));
#237060=CARTESIAN_POINT('Ctrl Pts',(164.247869878684,-5.8750163220866,133.823999511097));
#237061=CARTESIAN_POINT('Ctrl Pts',(163.969422254871,-0.635082105593798,
137.37936681918));
#237062=CARTESIAN_POINT('Ctrl Pts',(163.690974631059,5.18846154045405,134.892624634889));
#237063=CARTESIAN_POINT('Ctrl Pts',(163.412527007245,6.24406250126218,128.648967541478));
#237064=CARTESIAN_POINT('Ctrl Pts',(163.134079383433,1.56167506282176,124.386011388187));
#237065=CARTESIAN_POINT('Ctrl Pts',(162.85563175962,-4.55581546628373,126.021204622902));
#237066=CARTESIAN_POINT('Ctrl Pts',(162.577184135807,-6.48673414583306,
132.051884546553));
#237067=CARTESIAN_POINT('Ctrl Pts',(162.298736511994,-2.45666103994207,
136.936150924396));
#237068=CARTESIAN_POINT('Ctrl Pts',(162.020288888181,3.83096354709181,136.185601564872));
#237069=CARTESIAN_POINT('Ctrl Pts',(161.741841264368,6.59811978732212,130.489954663008));
#237070=CARTESIAN_POINT('Ctrl Pts',(161.463393640556,3.30192627907479,125.083231473798));
#237071=CARTESIAN_POINT('Ctrl Pts',(161.184946016742,-3.02857617157586,
124.933946475014));
#237072=CARTESIAN_POINT('Ctrl Pts',(160.90649839293,-6.57596507471956,130.179285287561));
#237073=CARTESIAN_POINT('Ctrl Pts',(160.628050769116,-4.08036332794952,
135.999037791754));
#237074=CARTESIAN_POINT('Ctrl Pts',(160.349603145304,2.16489298037573,137.045135746957));
#237075=CARTESIAN_POINT('Ctrl Pts',(160.07115552149,6.42071840063739,132.356266237063));
#237076=CARTESIAN_POINT('Ctrl Pts',(159.792707897678,4.77621728024515,126.241271277656));
#237077=CARTESIAN_POINT('Ctrl Pts',(159.514260273865,-1.25739418950663,
124.319532502318));
#237078=CARTESIAN_POINT('Ctrl Pts',(159.235812650052,-6.13552182622286,
128.357033963427));
#237079=CARTESIAN_POINT('Ctrl Pts',(158.957365026239,-5.37540464154493,
134.643509061136));
#237080=CARTESIAN_POINT('Ctrl Pts',(158.678917402427,0.324446805597038,
137.401994292032));
#237081=CARTESIAN_POINT('Ctrl Pts',(158.400469778613,5.72614748850293,134.097576488416));
#237082=CARTESIAN_POINT('Ctrl Pts',(158.122022154801,5.86579836733105,127.766854182028));
#237083=CARTESIAN_POINT('Ctrl Pts',(157.843574530988,0.615067106763091,
124.22745189946));
#237084=CARTESIAN_POINT('Ctrl Pts',(157.565126907175,-5.20088077722156,
126.731907428977));
#237085=CARTESIAN_POINT('Ctrl Pts',(157.286679283362,-6.23747330409059,
132.978748488409));
#237086=CARTESIAN_POINT('Ctrl Pts',(157.008231659549,-1.54213258201158,
137.227433319288));
#237087=CARTESIAN_POINT('Ctrl Pts',(156.729784035736,4.5703526455712,135.57362812183));
#237088=CARTESIAN_POINT('Ctrl Pts',(156.451336411923,6.48290706601333,129.537099079623));
#237089=CARTESIAN_POINT('Ctrl Pts',(156.172888788111,2.43798660040623,124.665121481617));
#237090=CARTESIAN_POINT('Ctrl Pts',(155.894441164297,-3.84732444870741,
125.434804731043));
#237091=CARTESIAN_POINT('Ctrl Pts',(155.615993540485,-6.59713228170722,
131.138847522794));
#237092=CARTESIAN_POINT('Ctrl Pts',(155.337545916672,-3.28449783564716,
136.535513189234));
#237093=CARTESIAN_POINT('Ctrl Pts',(155.059098292859,3.04642966473303,136.665529624679));
#237094=CARTESIAN_POINT('Ctrl Pts',(154.780650669046,6.57783712958646,131.409418076611));
#237095=CARTESIAN_POINT('Ctrl Pts',(154.502203045233,4.06453361755842,125.597288282381));
#237096=CARTESIAN_POINT('Ctrl Pts',(154.22375542142,-2.18387772549973,124.57020358456));
#237097=CARTESIAN_POINT('Ctrl Pts',(153.945307797607,-6.42541212718171,
129.272004644569));
#237098=CARTESIAN_POINT('Ctrl Pts',(153.666860173794,-4.76230668281685,
135.381965984011));
#237099=CARTESIAN_POINT('Ctrl Pts',(153.388412549982,1.27712595144142,137.285331620145));
#237100=CARTESIAN_POINT('Ctrl Pts',(153.109964926169,6.14294222739622,133.233001517943));
#237101=CARTESIAN_POINT('Ctrl Pts',(152.831517302356,5.36369469578529,126.948869073999));
#237102=CARTESIAN_POINT('Ctrl Pts',(152.553069678543,-0.344526230199219,
124.207745007359));
#237103=CARTESIAN_POINT('Ctrl Pts',(152.27462205473,-5.73614438167267,127.528588423912));
#237104=CARTESIAN_POINT('Ctrl Pts',(151.996174430917,-5.85652607262075,
133.859706456064));
#237105=CARTESIAN_POINT('Ctrl Pts',(151.717726807104,-0.595046410034728,
137.383110924578));
#237106=CARTESIAN_POINT('Ctrl Pts',(151.439279183291,5.21325183374003,134.860965250768));
#237107=CARTESIAN_POINT('Ctrl Pts',(151.160831559478,6.23082632381839,128.610998095198));
#237108=CARTESIAN_POINT('Ctrl Pts',(150.882383935665,1.52257581509584,124.376623945969));
#237109=CARTESIAN_POINT('Ctrl Pts',(150.603936311853,-4.58484748573611,
126.049025785542));
#237110=CARTESIAN_POINT('Ctrl Pts',(150.32548868804,-6.47901992942814,132.091348024725));
#237111=CARTESIAN_POINT('Ctrl Pts',(150.047041064227,-2.41928957569559,
136.950991709558));
#237112=CARTESIAN_POINT('Ctrl Pts',(149.768593440414,3.8636497092349,136.162181700472));
#237113=CARTESIAN_POINT('Ctrl Pts',(149.490145816601,6.59608366116008,130.449795860306));
#237114=CARTESIAN_POINT('Ctrl Pts',(149.211698192788,3.26703896508027,125.06323771061));
#237115=CARTESIAN_POINT('Ctrl Pts',(148.933250568975,-3.06425493618196,
124.95249104296));
#237116=CARTESIAN_POINT('Ctrl Pts',(148.654802945162,-6.57964824826877,
130.219326634649));
#237117=CARTESIAN_POINT('Ctrl Pts',(148.376355321349,-4.04866625388314,
136.02377987614));
#237118=CARTESIAN_POINT('Ctrl Pts',(148.097907697537,2.20284223947883,137.031841801807));
#237119=CARTESIAN_POINT('Ctrl Pts',(147.819460073724,6.43004632958585,132.317152748525));
#237120=CARTESIAN_POINT('Ctrl Pts',(147.541012449911,4.74835196802999,126.212281630895));
#237121=CARTESIAN_POINT('Ctrl Pts',(147.262564826098,-1.29684588225586,
124.327306766486));
#237122=CARTESIAN_POINT('Ctrl Pts',(146.984117202285,-6.15030572119196,
128.394427969547));
#237123=CARTESIAN_POINT('Ctrl Pts',(146.705669578472,-5.35193506149072,
134.676159544383));
#237124=CARTESIAN_POINT('Ctrl Pts',(146.427221954659,0.364602463157475,
137.399897053366));
#237125=CARTESIAN_POINT('Ctrl Pts',(146.148774330846,5.74608813598446,134.062658787717));
#237126=CARTESIAN_POINT('Ctrl Pts',(145.870326707034,5.84719952385297,127.731203680413));
#237127=CARTESIAN_POINT('Ctrl Pts',(145.59187908322,0.575020200877703,124.22382966629));
#237128=CARTESIAN_POINT('Ctrl Pts',(145.313431459408,-5.22557459540567,
126.76364211958));
#237129=CARTESIAN_POINT('Ctrl Pts',(145.034983835595,-6.22412162202233,
133.016677472446));
#237130=CARTESIAN_POINT('Ctrl Pts',(144.756536211782,-1.50300494324566,
137.236701713364));
#237131=CARTESIAN_POINT('Ctrl Pts',(144.478088587969,4.59929985250025,135.545718724575));
#237132=CARTESIAN_POINT('Ctrl Pts',(144.199640964156,6.47507277208744,129.497659263665));
#237133=CARTESIAN_POINT('Ctrl Pts',(143.921193340343,2.40057013901678,124.65039451108));
#237134=CARTESIAN_POINT('Ctrl Pts',(143.64274571653,-3.87993917743928,125.458323972397));
#237135=CARTESIAN_POINT('Ctrl Pts',(143.364298092718,-6.594973935395,131.178999942215));
#237136=CARTESIAN_POINT('Ctrl Pts',(143.085850468904,-3.2495498291107,136.555400674828));
#237137=CARTESIAN_POINT('Ctrl Pts',(142.807402845092,3.08205182079176,136.646876548744));
#237138=CARTESIAN_POINT('Ctrl Pts',(142.528955221279,6.58139841398854,131.369365704677));
#237139=CARTESIAN_POINT('Ctrl Pts',(142.250507597466,4.03276138391676,125.572642787588));
#237140=CARTESIAN_POINT('Ctrl Pts',(141.972059973653,-2.2217863466284,124.583612972623));
#237141=CARTESIAN_POINT('Ctrl Pts',(141.69361234984,-6.43462096491922,129.311146342943));
#237142=CARTESIAN_POINT('Ctrl Pts',(141.415164726027,-4.7343532651591,135.410870684068));
#237143=CARTESIAN_POINT('Ctrl Pts',(141.136717102214,1.31655379926713,137.277437314604));
#237144=CARTESIAN_POINT('Ctrl Pts',(140.858269478402,6.15761223939561,133.195562687939));
#237145=CARTESIAN_POINT('Ctrl Pts',(140.579821854588,5.34012584760095,126.916290175316));
#237146=CARTESIAN_POINT('Ctrl Pts',(140.301374230776,-0.384675318488256,
124.20996445632));
#237147=CARTESIAN_POINT('Ctrl Pts',(140.022926606963,-5.75597865932068,
127.563566655346));
#237148=CARTESIAN_POINT('Ctrl Pts',(139.74447898315,-5.83781880742758,133.895300184066));
#237149=CARTESIAN_POINT('Ctrl Pts',(139.466031359337,-0.554988664812238,
137.386611251964));
#237150=CARTESIAN_POINT('Ctrl Pts',(139.187583735524,5.23784894806212,134.829155547671));
#237151=CARTESIAN_POINT('Ctrl Pts',(138.909136111711,6.21735926081381,128.573109924773));
#237152=CARTESIAN_POINT('Ctrl Pts',(138.630688487898,1.48342014776303,124.367474685896));
#237153=CARTESIAN_POINT('Ctrl Pts',(138.352240864086,-4.61370961197883,
126.077023158863));
#237154=CARTESIAN_POINT('Ctrl Pts',(138.073793240272,-6.47106563055709,
132.130763813104));
#237155=CARTESIAN_POINT('Ctrl Pts',(137.79534561646,-2.38182846378423,136.965604729043));
#237156=CARTESIAN_POINT('Ctrl Pts',(137.516897992647,3.89619270241722,136.138563300043));
#237157=CARTESIAN_POINT('Ctrl Pts',(137.238450368834,6.59380311469226,130.409650196134));
#237158=CARTESIAN_POINT('Ctrl Pts',(136.960002745021,3.23203058975544,125.043456686844));
#237159=CARTESIAN_POINT('Ctrl Pts',(136.681555121208,-3.09982015369448,
124.971252454085));
#237160=CARTESIAN_POINT('Ctrl Pts',(136.403107497395,-6.58308761053252,
130.259389660389));
#237161=CARTESIAN_POINT('Ctrl Pts',(136.124659873582,-4.01681915499975,
136.048328553027));
#237162=CARTESIAN_POINT('Ctrl Pts',(135.846212249769,2.24070987145278,137.018317095051));
#237163=CARTESIAN_POINT('Ctrl Pts',(135.567764625956,6.43913599080291,132.277983202917));
#237164=CARTESIAN_POINT('Ctrl Pts',(135.289317002144,4.72031070388647,126.183462145311));
#237165=CARTESIAN_POINT('Ctrl Pts',(135.010869378331,-1.33624951990408,
124.335321040266));
#237166=CARTESIAN_POINT('Ctrl Pts',(134.732421754518,-6.16486171432077,
128.431911276607));
#237167=CARTESIAN_POINT('Ctrl Pts',(134.453974130705,-5.32826716351462,
134.708666556695));
#237168=CARTESIAN_POINT('Ctrl Pts',(134.175526506892,0.404744610239488,
137.397555414672));
#237169=CARTESIAN_POINT('Ctrl Pts',(133.897078883079,5.76581586005707,134.027620349581));
#237170=CARTESIAN_POINT('Ctrl Pts',(133.618631259266,5.82838401024617,127.695667055759));
#237171=CARTESIAN_POINT('Ctrl Pts',(133.340183635453,0.534951987407334,
124.220451277114));
#237172=CARTESIAN_POINT('Ctrl Pts',(133.06173601164,-5.25007477800144,126.795526540492));
#237173=CARTESIAN_POINT('Ctrl Pts',(132.783288387828,-6.21053930283845,
133.054524478268));
#237174=CARTESIAN_POINT('Ctrl Pts',(132.504840764015,-1.46382161007886,
137.245731754674));
#237175=CARTESIAN_POINT('Ctrl Pts',(132.226393140202,4.62807663068185,135.517633634551));
#237176=CARTESIAN_POINT('Ctrl Pts',(131.947945516389,6.46699854195874,129.458267868007));
#237177=CARTESIAN_POINT('Ctrl Pts',(131.669497892576,2.3630647236181,124.635895578019));
#237178=CARTESIAN_POINT('Ctrl Pts',(131.391050268763,-3.91241013359816,
125.482041313105));
#237179=CARTESIAN_POINT('Ctrl Pts',(131.11260264495,-6.59257120989826,131.219138479237));
#237180=CARTESIAN_POINT('Ctrl Pts',(130.834155021138,-3.2144814093103,136.575075053519));
#237181=CARTESIAN_POINT('Ctrl Pts',(130.555707397324,3.1175597702868,136.628006976231));
#237182=CARTESIAN_POINT('Ctrl Pts',(130.277259773512,6.58471582225214,131.329292396271));
#237183=CARTESIAN_POINT('Ctrl Pts',(129.998812149698,4.0008397148189,125.548191156024));
#237184=CARTESIAN_POINT('Ctrl Pts',(129.720364525886,-2.25961263864694,
124.59725287278));
#237185=CARTESIAN_POINT('Ctrl Pts',(129.441916902073,-6.44359136541048,
129.350343372922));
#237186=CARTESIAN_POINT('Ctrl Pts',(129.16346927826,-4.70622441430021,135.439604688201));
#237187=CARTESIAN_POINT('Ctrl Pts',(128.885021654447,1.35593286170785,137.269303146827));
#237188=CARTESIAN_POINT('Ctrl Pts',(128.606574030634,6.17205407880915,133.158035251063));
#237189=CARTESIAN_POINT('Ctrl Pts',(128.328126406821,5.31635911908928,126.883855350513));
#237190=CARTESIAN_POINT('Ctrl Pts',(128.049678783009,-0.424810152491945,
124.212428263054));
#237191=CARTESIAN_POINT('Ctrl Pts',(127.771231159195,-5.77559964706288,
127.598664975593));
#237192=CARTESIAN_POINT('Ctrl Pts',(127.492783535383,-5.81889521971155,
133.930779376167));
#237193=CARTESIAN_POINT('Ctrl Pts',(127.21433591157,-0.514910354280421,
137.389867671632));
#237194=CARTESIAN_POINT('Ctrl Pts',(126.935888287757,5.26225197196523,134.797196704317));
#237195=CARTESIAN_POINT('Ctrl Pts',(126.657440663944,6.20366181127538,128.535304434163));
#237196=CARTESIAN_POINT('Ctrl Pts',(126.378993040131,1.44420951175126,124.358563947));
#237197=CARTESIAN_POINT('Ctrl Pts',(126.100545416318,-4.64240077551519,
126.105195705413));
#237198=CARTESIAN_POINT('Ctrl Pts',(125.822097792505,-6.46287154396936,
132.170130451126));
#237199=CARTESIAN_POINT('Ctrl Pts',(125.543650168692,-2.34427909234318,
136.979989441362));
#237200=CARTESIAN_POINT('Ctrl Pts',(125.26520254488,3.92859132074607,136.114747238771));
#237201=CARTESIAN_POINT('Ctrl Pts',(124.986754921067,6.59127823242518,130.369519158099));
#237202=CARTESIAN_POINT('Ctrl Pts',(124.708307297254,3.19690245034852,125.023889135492));
#237203=CARTESIAN_POINT('Ctrl Pts',(124.429859673441,-3.13527050623128,
124.990230013179));
#237204=CARTESIAN_POINT('Ctrl Pts',(124.151412049628,-6.58628303406391,
130.299472880227));
#237205=CARTESIAN_POINT('Ctrl Pts',(123.872964425815,-3.98482321140548,
136.072682912751));
#237206=CARTESIAN_POINT('Ctrl Pts',(123.594516802002,2.2784944730983,137.004562127853));
#237207=CARTESIAN_POINT('Ctrl Pts',(123.316069178189,6.44798704746787,132.238759051683));
#237208=CARTESIAN_POINT('Ctrl Pts',(123.037621554376,4.6920945268939,126.154813888819));
#237209=CARTESIAN_POINT('Ctrl Pts',(122.759173930564,-1.37560364233486,
124.343575026687));
#237210=CARTESIAN_POINT('Ctrl Pts',(122.480726306751,-6.17918926623166,
128.46948249565));
#237211=CARTESIAN_POINT('Ctrl Pts',(122.202278682938,-5.30440182463932,
134.741028893516));
#237212=CARTESIAN_POINT('Ctrl Pts',(121.923831059125,0.444871759361186,
137.394969462721));
#237213=CARTESIAN_POINT('Ctrl Pts',(121.645383435312,5.78532992970255,133.992462472369));
#237214=CARTESIAN_POINT('Ctrl Pts',(121.366935811499,5.80935252372653,127.660245624887));
#237215=CARTESIAN_POINT('Ctrl Pts',(121.088488187686,0.494863951094175,
124.21731685712));
#237216=CARTESIAN_POINT('Ctrl Pts',(120.810040563873,-5.27438041714564,
126.827559510225));
#237217=CARTESIAN_POINT('Ctrl Pts',(120.53159294006,-6.19672684983677,133.092288103441));
#237218=CARTESIAN_POINT('Ctrl Pts',(120.253145316248,-1.42458403446405,
137.254523108609));
#237219=CARTESIAN_POINT('Ctrl Pts',(119.974697692435,4.65668191378195,135.489373892464));
#237220=CARTESIAN_POINT('Ctrl Pts',(119.696250068622,6.45868467482089,129.418926352309));
#237221=CARTESIAN_POINT('Ctrl Pts',(119.417802444809,2.32547174398699,124.621625219699));
#237222=CARTESIAN_POINT('Ctrl Pts',(119.139354820996,-3.94473611396066,
125.505955874312));
#237223=CARTESIAN_POINT('Ctrl Pts',(118.860907197183,-6.58992419425096,
131.259261646514));
#237224=CARTESIAN_POINT('Ctrl Pts',(118.58245957337,-3.17929387571916,136.594535596262));
#237225=CARTESIAN_POINT('Ctrl Pts',(118.304011949557,3.15295219745811,136.608921606362));
#237226=CARTESIAN_POINT('Ctrl Pts',(118.025564325744,6.58778923144938,131.289199636326));
#237227=CARTESIAN_POINT('Ctrl Pts',(117.747116701932,3.96876979313418,125.523934293753));
#237228=CARTESIAN_POINT('Ctrl Pts',(117.468669078118,-2.29735519988813,
124.611122779595));
#237229=CARTESIAN_POINT('Ctrl Pts',(117.190221454306,-6.45232299625411,
129.389594282045));
#237230=CARTESIAN_POINT('Ctrl Pts',(116.911773830493,-4.67792117256487,
135.468166931659));
#237231=CARTESIAN_POINT('Ctrl Pts',(116.63332620668,1.39526167955762,137.260929418227));
#237232=CARTESIAN_POINT('Ctrl Pts',(116.354878582867,6.18626721048894,133.120420597908));
#237233=CARTESIAN_POINT('Ctrl Pts',(116.076430959054,5.29239539093549,126.851565801475));
#237234=CARTESIAN_POINT('Ctrl Pts',(115.797983335241,-0.464929244999223,
124.215136336267));
#237235=CARTESIAN_POINT('Ctrl Pts',(115.519535711428,-5.79500661783607,
127.633882084071));
#237236=CARTESIAN_POINT('Ctrl Pts',(115.241088087616,-5.79975601069334,
133.96614271767));
#237237=CARTESIAN_POINT('Ctrl Pts',(114.962640463802,-0.474812963556037,
137.392880062915));
#237238=CARTESIAN_POINT('Ctrl Pts',(114.68419283999,5.28646000118636,134.765089904953));
#237239=CARTESIAN_POINT('Ctrl Pts',(114.405745216177,6.18973448276714,128.497583024264));
#237240=CARTESIAN_POINT('Ctrl Pts',(114.127297592364,1.40494536002493,124.349892059469));
#237241=CARTESIAN_POINT('Ctrl Pts',(113.848849968551,-4.67091991318358,
126.133542381245));
#237242=CARTESIAN_POINT('Ctrl Pts',(113.570402344738,-6.45443797329988,
132.209446480045));
#237243=CARTESIAN_POINT('Ctrl Pts',(113.291954720925,-2.30664285277824,
136.994145313484));
#237244=CARTESIAN_POINT('Ctrl Pts',(113.013507097112,3.96084436367879,136.09073439917));
#237245=CARTESIAN_POINT('Ctrl Pts',(112.735059473299,6.58850910791926,130.329404233275));
#237246=CARTESIAN_POINT('Ctrl Pts',(112.456611849487,3.16165584854565,125.004535781636));
#237247=CARTESIAN_POINT('Ctrl Pts',(112.178164225674,-3.1706046801665,125.00942301702));
#237248=CARTESIAN_POINT('Ctrl Pts',(111.899716601861,-6.58923440045535,
130.339574808866));
#237249=CARTESIAN_POINT('Ctrl Pts',(111.621268978048,-3.9526796087217,136.096842052857));
#237250=CARTESIAN_POINT('Ctrl Pts',(111.342821354235,2.31619464429322,136.990577409908));
#237251=CARTESIAN_POINT('Ctrl Pts',(111.064373730422,6.45659917160154,132.199481748287));
#237252=CARTESIAN_POINT('Ctrl Pts',(110.785926106609,4.66370448261314,126.12633792299));
#237253=CARTESIAN_POINT('Ctrl Pts',(110.507478482796,-1.41490679126679,
124.352068419894));
#237254=CARTESIAN_POINT('Ctrl Pts',(110.229030858983,-6.19328784601188,
128.50714023446));
#237255=CARTESIAN_POINT('Ctrl Pts',(109.950583235171,-5.28033992920373,
134.773245355646));
#237256=CARTESIAN_POINT('Ctrl Pts',(109.672135611358,0.484982423596243,
137.392139293334));
#237257=CARTESIAN_POINT('Ctrl Pts',(109.393687987545,5.80462962181993,133.957186458871));
#237258=CARTESIAN_POINT('Ctrl Pts',(109.115240363732,5.79010576951274,127.624940700352));
#237259=CARTESIAN_POINT('Ctrl Pts',(108.836792739919,0.454757577415474,
124.214426522456));
#237260=CARTESIAN_POINT('Ctrl Pts',(108.558345116106,-5.29849061218381,
126.859739841786));
#237261=CARTESIAN_POINT('Ctrl Pts',(108.279897492293,-6.18268477484283,
133.12996694862));
#237262=CARTESIAN_POINT('Ctrl Pts',(108.00144986848,-1.38529367036394,137.2630754494));
#237263=CARTESIAN_POINT('Ctrl Pts',(107.723002244667,4.68511464182123,135.460940545486));
#237264=CARTESIAN_POINT('Ctrl Pts',(107.444554620855,6.45013147874722,129.379636174388));
#237265=CARTESIAN_POINT('Ctrl Pts',(107.166106997042,2.28779259314522,124.607583964913));
#237266=CARTESIAN_POINT('Ctrl Pts',(106.887659373229,-3.97691592067581,
125.530066769856));
#237267=CARTESIAN_POINT('Ctrl Pts',(106.609211749416,-6.58703298653922,
131.299367957265));
#237268=CARTESIAN_POINT('Ctrl Pts',(106.330764125603,-3.14398853222427,
136.613781581943));
#237269=CARTESIAN_POINT('Ctrl Pts',(106.05231650179,3.18822779082625,136.589621146351));
#237270=CARTESIAN_POINT('Ctrl Pts',(105.773868877977,6.59061852769399,131.249088910493));
#237271=CARTESIAN_POINT('Ctrl Pts',(105.495421254164,3.93655280722527,125.49987309962));
#237272=CARTESIAN_POINT('Ctrl Pts',(105.216973630351,-2.33501263178752,
124.625222179118));
#237273=CARTESIAN_POINT('Ctrl Pts',(104.938526006539,-6.46081553389627,
129.428897615854));
#237274=CARTESIAN_POINT('Ctrl Pts',(104.660078382726,-4.64944458874018,
135.49655635606));
#237275=CARTESIAN_POINT('Ctrl Pts',(104.381630758913,1.43453879547275,137.252316439095));
#237276=CARTESIAN_POINT('Ctrl Pts',(104.1031831351,6.20025110776228,133.082720122298));
#237277=CARTESIAN_POINT('Ctrl Pts',(103.824735511287,5.26823555112421,126.819422724701));
#237278=CARTESIAN_POINT('Ctrl Pts',(103.546287887474,-0.505031109382345,
124.218088575609));
#237279=CARTESIAN_POINT('Ctrl Pts',(103.267840263661,-5.81419885250792,
127.669216675797));
#237280=CARTESIAN_POINT('Ctrl Pts',(102.989392639848,-5.78040188958328,
134.001388898174));
#237281=CARTESIAN_POINT('Ctrl Pts',(102.710945016035,-0.434697978462825,
137.395648314187));
#237282=CARTESIAN_POINT('Ctrl Pts',(102.432497392222,5.31047213868803,134.732836339309));
#237283=CARTESIAN_POINT('Ctrl Pts',(102.15404976841,6.17557779137139,128.459947092858));
#237284=CARTESIAN_POINT('Ctrl Pts',(101.875602144597,1.3656291475316,124.341459344644));
#237285=CARTESIAN_POINT('Ctrl Pts',(101.597154520784,-4.69926596819684,
126.162062135967));
#237286=CARTESIAN_POINT('Ctrl Pts',(101.318706896971,-6.44576523105769,
132.248710442988));
#237287=CARTESIAN_POINT('Ctrl Pts',(101.040259273158,-2.26892113971413,
137.008071820859));
#237288=CARTESIAN_POINT('Ctrl Pts',(100.761811649345,3.99295063606701,136.066525671043));
#237289=CARTESIAN_POINT('Ctrl Pts',(100.483364025532,6.58549584378548,130.289306908136));
#237290=CARTESIAN_POINT('Ctrl Pts',(100.204916401719,3.12629209042249,124.985397342422));
#237291=CARTESIAN_POINT('Ctrl Pts',(99.9264687779064,-3.20582136617937,
125.028830754405));
#237292=CARTESIAN_POINT('Ctrl Pts',(99.6480211540935,-6.5919416003429,130.379693960313));
#237293=CARTESIAN_POINT('Ctrl Pts',(99.3695735302808,-3.92038953804142,
136.120805078117));
#237294=CARTESIAN_POINT('Ctrl Pts',(99.0911259064677,2.35380898804382,136.976363459425));
#237295=CARTESIAN_POINT('Ctrl Pts',(98.812678282655,6.46497204407849,132.160152748165));
#237296=CARTESIAN_POINT('Ctrl Pts',(98.5342306588419,4.63514162304771,126.098035303012));
#237297=CARTESIAN_POINT('Ctrl Pts',(98.2557830350292,-1.45415751030726,
124.36080090516));
#237298=CARTESIAN_POINT('Ctrl Pts',(97.9773354112161,-6.20715693123341,
128.544883097616));
#237299=CARTESIAN_POINT('Ctrl Pts',(97.6988877874034,-5.25608236883021,
134.805314749293));
#237300=CARTESIAN_POINT('Ctrl Pts',(97.4204401635904,0.525075116629235,
137.389065011387));
#237301=CARTESIAN_POINT('Ctrl Pts',(97.1419925397775,5.82371422125203,133.921793616252));
#237302=CARTESIAN_POINT('Ctrl Pts',(96.8635449159648,5.77064446080036,127.589753590393));
#237303=CARTESIAN_POINT('Ctrl Pts',(96.5850972921516,0.414634352527504,
124.211780380221));
#237304=CARTESIAN_POINT('Ctrl Pts',(96.306649668339,-5.32240446970382,126.89206634272));
#237305=CARTESIAN_POINT('Ctrl Pts',(96.0282020445258,-6.16841359819089,
133.1675596176));
#237306=CARTESIAN_POINT('Ctrl Pts',(95.7497544207132,-1.34595197369742,
137.271388460138));
#237307=CARTESIAN_POINT('Ctrl Pts',(95.4713067969001,4.7133737612145,135.432334647225));
#237308=CARTESIAN_POINT('Ctrl Pts',(95.1928591730874,6.44133927067958,129.340398790155));
#237309=CARTESIAN_POINT('Ctrl Pts',(94.9144115492744,2.25002866730758,124.593772333964));
#237310=CARTESIAN_POINT('Ctrl Pts',(94.6359639254615,-4.008948361309,125.554373106298));
#237311=CARTESIAN_POINT('Ctrl Pts',(94.3575163016487,-6.58389769389783,
131.339455925338));
#237312=CARTESIAN_POINT('Ctrl Pts',(94.0790686778357,-3.10856668707799,
136.632812297395));
#237313=CARTESIAN_POINT('Ctrl Pts',(93.8006210540229,3.22338524324122,136.570106311383));
#237314=CARTESIAN_POINT('Ctrl Pts',(93.52217343021,6.59320360614536,131.208961705089));
#237315=CARTESIAN_POINT('Ctrl Pts',(93.2437258063971,3.90418995090443,125.476008465224));
#237316=CARTESIAN_POINT('Ctrl Pts',(92.9652781825842,-2.37258353893516,
124.639550548886));
#237317=CARTESIAN_POINT('Ctrl Pts',(92.6868305587713,-6.46906866364288,
129.468251917951));
#237318=CARTESIAN_POINT('Ctrl Pts',(92.4083829349583,-4.62079571803641,
135.524771909422));
#237319=CARTESIAN_POINT('Ctrl Pts',(92.1299353111456,1.47376275402524,137.24346452859));
#237320=CARTESIAN_POINT('Ctrl Pts',(91.8514876873325,6.21400525245068,133.04493522124));
#237321=CARTESIAN_POINT('Ctrl Pts',(91.5730400635199,5.24388049490719,126.787427311268));
#237322=CARTESIAN_POINT('Ctrl Pts',(91.2945924397067,-0.545114259651984,
124.221284871682));
#237323=CARTESIAN_POINT('Ctrl Pts',(91.016144815894,-5.83317563990314,127.704667441434));
#237324=CARTESIAN_POINT('Ctrl Pts',(90.7376971920811,-5.76083357355547,
134.036516611621));
#237325=CARTESIAN_POINT('Ctrl Pts',(90.4592495682681,-0.394566885476172,
137.398172322869));
#237326=CARTESIAN_POINT('Ctrl Pts',(90.1808019444553,5.33428749469169,134.700437202553));
#237327=CARTESIAN_POINT('Ctrl Pts',(89.9023543206424,6.16119226166949,128.422398034556));
#237328=CARTESIAN_POINT('Ctrl Pts',(89.6239066968295,1.32626233114802,124.333266115003));
#237329=CARTESIAN_POINT('Ctrl Pts',(89.3454590730166,-4.72743789018152,
126.190753912764));
#237330=CARTESIAN_POINT('Ctrl Pts',(89.0670114492037,-6.43685363861442,
132.28792088502));
#237331=CARTESIAN_POINT('Ctrl Pts',(88.7885638253908,-2.23111535094281,
137.021768447433));
#237332=CARTESIAN_POINT('Ctrl Pts',(88.5101162015778,4.02490894820102,136.042121951457));
#237333=CARTESIAN_POINT('Ctrl Pts',(88.2316685777651,6.58223855168135,130.2492286685));
#237334=CARTESIAN_POINT('Ctrl Pts',(87.9532209539521,3.09081248639635,124.966474527032));
#237335=CARTESIAN_POINT('Ctrl Pts',(87.6747733301392,-3.2409192593025,125.048452506173));
#237336=CARTESIAN_POINT('Ctrl Pts',(87.3963257063264,-6.59440453341028,
130.41982884794));
#237337=CARTESIAN_POINT('Ctrl Pts',(87.1178780825135,-3.88795419588509,
136.144571100572));
#237338=CARTESIAN_POINT('Ctrl Pts',(86.8394304587006,2.39133611053674,136.961920803106));
#237339=CARTESIAN_POINT('Ctrl Pts',(86.5609828348878,6.47310535463887,132.120773508667));
#237340=CARTESIAN_POINT('Ctrl Pts',(86.2825352110747,4.60640700660486,126.06990707765));
#237341=CARTESIAN_POINT('Ctrl Pts',(86.004087587262,-1.49335434500641,124.369772158902));
#237342=CARTESIAN_POINT('Ctrl Pts',(85.725639963449,-6.22079600797217,128.582709686544));
#237343=CARTESIAN_POINT('Ctrl Pts',(85.4471923396362,-5.23163004239161,
134.837235886113));
#237344=CARTESIAN_POINT('Ctrl Pts',(85.1687447158232,0.565148352810691,
137.385746730796));
#237345=CARTESIAN_POINT('Ctrl Pts',(84.8902970920103,5.842583020812,133.886285256006));
#237346=CARTESIAN_POINT('Ctrl Pts',(84.6118494681974,5.75096931873532,127.554685598878));
#237347=CARTESIAN_POINT('Ctrl Pts',(84.3334018443846,0.374495763211118,
124.209378528473));
#237348=CARTESIAN_POINT('Ctrl Pts',(84.0549542205716,-5.34612110356891,
126.924537815158));
#237349=CARTESIAN_POINT('Ctrl Pts',(83.7765065967588,-6.15391384870464,
133.205064717373));
#237350=CARTESIAN_POINT('Ctrl Pts',(83.498058972946,-1.30656040228555,137.279461832782));
#237351=CARTESIAN_POINT('Ctrl Pts',(83.2196113491328,4.74145822480973,135.403557257686));
#237352=CARTESIAN_POINT('Ctrl Pts',(82.9411637253203,6.43230837641647,129.301215653567));
#237353=CARTESIAN_POINT('Ctrl Pts',(82.6627161015071,2.21218136583022,124.580190838648));
#237354=CARTESIAN_POINT('Ctrl Pts',(82.3842684776944,-4.04083224888638,
125.578873982957));
#237355=CARTESIAN_POINT('Ctrl Pts',(82.1058208538814,-6.58051843250612,
131.379524065257));
#237356=CARTESIAN_POINT('Ctrl Pts',(81.8273732300686,-3.07302965285007,
136.651627037425));
#237357=CARTESIAN_POINT('Ctrl Pts',(81.5489256062556,3.25842325193051,136.550377824588));
#237358=CARTESIAN_POINT('Ctrl Pts',(81.270477982443,6.59554437101248,131.168819507043));
#237359=CARTESIAN_POINT('Ctrl Pts',(80.9920303586297,3.87168242338918,125.452341274876));
#237360=CARTESIAN_POINT('Ctrl Pts',(80.713582734817,-2.41006652912724,124.654107357959));
#237361=CARTESIAN_POINT('Ctrl Pts',(80.435135111004,-6.47708207967116,129.507655730047));
#237362=CARTESIAN_POINT('Ctrl Pts',(80.1566874871913,-4.59197562204804,
135.552812546207));
#237363=CARTESIAN_POINT('Ctrl Pts',(79.8782398633782,1.51293210175691,137.234374014721));
#237364=CARTESIAN_POINT('Ctrl Pts',(79.5997922395654,6.22752913488936,133.007067294864));
#237365=CARTESIAN_POINT('Ctrl Pts',(79.3213446157525,5.2193311247699,126.755580746775));
#237366=CARTESIAN_POINT('Ctrl Pts',(79.0428969919396,-0.585177210512381,
124.224725106049));
#237367=CARTESIAN_POINT('Ctrl Pts',(78.7644493681267,-5.85193627682986,
127.740233067343));
#237368=CARTESIAN_POINT('Ctrl Pts',(78.4860017443139,-5.74105178772106,
134.071524556339));
#237369=CARTESIAN_POINT('Ctrl Pts',(78.2075541205009,-0.354421171668466,
137.400451995434));
#237370=CARTESIAN_POINT('Ctrl Pts',(77.9291064966881,5.35790518671055,134.667893695246));
#237371=CARTESIAN_POINT('Ctrl Pts',(77.6506588728751,6.14657842672258,128.384937240753));
#237372=CARTESIAN_POINT('Ctrl Pts',(77.3722112490624,1.28684636962602,124.325312674148));
#237373=CARTESIAN_POINT('Ctrl Pts',(77.0937636252493,-4.75543463521666,
126.219616648455));
#237374=CARTESIAN_POINT('Ctrl Pts',(76.8153160014366,-6.42770352619243,
132.327076353179));
#237375=CARTESIAN_POINT('Ctrl Pts',(76.5368683776235,-2.19322688737167,
137.035234685673));
#237376=CARTESIAN_POINT('Ctrl Pts',(76.2584207538107,4.05671811585379,136.017524144697));
#237377=CARTESIAN_POINT('Ctrl Pts',(75.9799731299978,6.57873735230709,130.209170999483));
#237378=CARTESIAN_POINT('Ctrl Pts',(75.7015255061849,3.05521835117689,124.947768036657));
#237379=CARTESIAN_POINT('Ctrl Pts',(75.423077882372,-3.27589705897064,125.068287545233));
#237380=CARTESIAN_POINT('Ctrl Pts',(75.1446302585591,-6.5966231083926,130.459977984534));
#237381=CARTESIAN_POINT('Ctrl Pts',(74.8661826347462,-3.85537478415624,
136.168139239563));
#237382=CARTESIAN_POINT('Ctrl Pts',(74.5877350109334,2.42877462119068,136.94724997613));
#237383=CARTESIAN_POINT('Ctrl Pts',(74.3092873871204,6.48099880189986,132.081345489005));
#237384=CARTESIAN_POINT('Ctrl Pts',(74.0308397633076,4.57750169805637,126.041954289206));
#237385=CARTESIAN_POINT('Ctrl Pts',(73.7523921394947,-1.53249584291112,
124.378981848686));
#237386=CARTESIAN_POINT('Ctrl Pts',(73.4739445156818,-6.23420457082727,
128.620618599563));
#237387=CARTESIAN_POINT('Ctrl Pts',(73.1954968918689,-5.20698385597775,
134.869007583256));
#237388=CARTESIAN_POINT('Ctrl Pts',(72.917049268056,0.605200647212208,137.382184574524));
#237389=CARTESIAN_POINT('Ctrl Pts',(72.6386016442432,5.86123532130951,133.850662693911));
#237390=CARTESIAN_POINT('Ctrl Pts',(72.3601540204302,5.73108107238729,127.519738025268));
#237391=CARTESIAN_POINT('Ctrl Pts',(72.0817063966174,0.334343296816498,
124.207221056211));
#237392=CARTESIAN_POINT('Ctrl Pts',(71.8032587728044,-5.36963963495047,
126.957153055855));
#237393=CARTESIAN_POINT('Ctrl Pts',(71.5248111489915,-6.13918606367764,
133.242480858172));
#237394=CARTESIAN_POINT('Ctrl Pts',(71.2463635251787,-1.26712041579749,
137.287295268168));
#237395=CARTESIAN_POINT('Ctrl Pts',(70.9679159013657,4.76936699192676,135.374609443224));
#237396=CARTESIAN_POINT('Ctrl Pts',(70.689468277553,6.423039130601,129.262088216567));
#237397=CARTESIAN_POINT('Ctrl Pts',(70.4110206537399,2.17425209115883,124.566839982233));
#237398=CARTESIAN_POINT('Ctrl Pts',(70.1325730299272,-4.07256640193864,
125.603568491945));
#237399=CARTESIAN_POINT('Ctrl Pts',(69.8541254061142,-6.57689532758393,
131.419570892283));
#237400=CARTESIAN_POINT('Ctrl Pts',(69.5756777823013,-3.03737874637841,
136.670225104848));
#237401=CARTESIAN_POINT('Ctrl Pts',(69.2972301584884,3.2933405185478,136.530436417012));
#237402=CARTESIAN_POINT('Ctrl Pts',(69.0187825346755,6.5976407355574,131.128663803839));
#237403=CARTESIAN_POINT('Ctrl Pts',(68.7403349108627,3.83903142925813,125.428872405572));
#237404=CARTESIAN_POINT('Ctrl Pts',(68.4618872870498,-2.44746021341752,
124.668892066929));
#237405=CARTESIAN_POINT('Ctrl Pts',(68.1834396632368,-6.48485548504104,
129.547107592018));
#237406=CARTESIAN_POINT('Ctrl Pts',(67.904992039424,-4.56298536871445,135.580677227361));
#237407=CARTESIAN_POINT('Ctrl Pts',(67.6265444156111,1.55204538723279,137.225045234339));
#237408=CARTESIAN_POINT('Ctrl Pts',(67.3480967917982,6.2408222539455,132.969117746385));
#237409=CARTESIAN_POINT('Ctrl Pts',(67.0696491679854,5.19458835039884,126.723884211309));
#237410=CARTESIAN_POINT('Ctrl Pts',(66.7912015441724,-0.625218477415679,
124.228409151229));
#237411=CARTESIAN_POINT('Ctrl Pts',(66.5127539203596,-5.87048006810572,
127.775912235624));
#237412=CARTESIAN_POINT('Ctrl Pts',(66.2343062965465,-5.72105726510147,
134.106411435094));
#237413=CARTESIAN_POINT('Ctrl Pts',(65.9558586727338,-0.314262324654327,
137.402487247406));
#237414=CARTESIAN_POINT('Ctrl Pts',(65.6774110489208,5.3813243395822,134.6352070233));
#237415=CARTESIAN_POINT('Ctrl Pts',(65.398963425108,6.13173682805169,128.347566099575));
#237416=CARTESIAN_POINT('Ctrl Pts',(65.120515801295,1.24738272353907,124.317599316798));
#237417=CARTESIAN_POINT('Ctrl Pts',(64.8420681774823,-4.78325516587229,
126.248649273519));
#237418=CARTESIAN_POINT('Ctrl Pts',(64.5636205536692,-6.41831523285262,
132.366175396547));
#237419=CARTESIAN_POINT('Ctrl Pts',(64.2851729298565,-2.15525715297185,
137.048470036584));
#237420=CARTESIAN_POINT('Ctrl Pts',(64.0067253060435,4.08837696032456,135.992733162246));
#237421=CARTESIAN_POINT('Ctrl Pts',(63.7282776822307,6.57499237540094,130.169135385437));
#237422=CARTESIAN_POINT('Ctrl Pts',(63.4498300584178,3.01951100371835,124.929278564476));
#237423=CARTESIAN_POINT('Ctrl Pts',(63.1713824346048,-3.31075346906837,
125.088335136589));
#237424=CARTESIAN_POINT('Ctrl Pts',(62.892934810792,-6.59859724307971,130.500139882352));
#237425=CARTESIAN_POINT('Ctrl Pts',(62.614487186979,-3.82265251009718,136.191508621766));
#237426=CARTESIAN_POINT('Ctrl Pts',(62.3360395631662,2.46612313270748,136.932351522132));
#237427=CARTESIAN_POINT('Ctrl Pts',(62.0575919393533,6.48865209336687,132.041870150199));
#237428=CARTESIAN_POINT('Ctrl Pts',(61.7791443155403,4.5484267684992,126.014177973478));
#237429=CARTESIAN_POINT('Ctrl Pts',(61.5006966917276,-1.57158055361859,
124.388429633243));
#237430=CARTESIAN_POINT('Ctrl Pts',(61.2222490679146,-6.24738212293903,
128.658608431946));
#237431=CARTESIAN_POINT('Ctrl Pts',(60.9438014441017,-5.18214472286266,
134.900628663412));
#237432=CARTESIAN_POINT('Ctrl Pts',(60.6653538202889,0.645230515680748,
137.378378674564));
#237433=CARTESIAN_POINT('Ctrl Pts',(60.3869061964759,5.87967043157647,133.814927249971));
#237434=CARTESIAN_POINT('Ctrl Pts',(60.108458572663,5.71098045872276,127.484912164554));
#237435=CARTESIAN_POINT('Ctrl Pts',(59.8300109488502,0.294178441208572,
124.205308043382));
#237436=CARTESIAN_POINT('Ctrl Pts',(59.5515633250373,-5.39295919236059,
126.989910856244));
#237437=CARTESIAN_POINT('Ctrl Pts',(59.2731157012244,-6.12423078885343,
133.27980665353));
#237438=CARTESIAN_POINT('Ctrl Pts',(58.9946680774115,-1.2276334756968,137.294888476026));
#237439=CARTESIAN_POINT('Ctrl Pts',(58.7162204535986,4.79709902839574,135.345492276511));
#237440=CARTESIAN_POINT('Ctrl Pts',(58.4377728297857,6.41353187670863,129.223017929039));
#237441=CARTESIAN_POINT('Ctrl Pts',(58.1593252059728,2.13624224877676,124.553720259438));
#237442=CARTESIAN_POINT('Ctrl Pts',(57.8808775821599,-4.10414964454526,
125.628455718198));
#237443=CARTESIAN_POINT('Ctrl Pts',(57.602429958347,-6.57302851338661,131.459594922466));
#237444=CARTESIAN_POINT('Ctrl Pts',(57.3239823345341,-3.00161528872044,
136.688605810505));
#237445=CARTESIAN_POINT('Ctrl Pts',(57.0455347107212,3.32813574922106,136.510282827592));
#237446=CARTESIAN_POINT('Ctrl Pts',(56.7670870869083,6.59949262209846,131.088496083461));
#237447=CARTESIAN_POINT('Ctrl Pts',(56.4886394630955,3.80623817840574,125.405602726962));
#237448=CARTESIAN_POINT('Ctrl Pts',(56.2101918392826,-2.48476320616966,
124.683904127941));
#237449=CARTESIAN_POINT('Ctrl Pts',(55.9317442154696,-6.49238859170611,
129.586606041964));
#237450=CARTESIAN_POINT('Ctrl Pts',(55.6532965916568,-4.53382603227983,
135.608364920346));
#237451=CARTESIAN_POINT('Ctrl Pts',(55.3748489678439,1.59110116109648,137.215478533129));
#237452=CARTESIAN_POINT('Ctrl Pts',(55.096401344031,6.25388411703813,132.931087982032));
#237453=CARTESIAN_POINT('Ctrl Pts',(54.8179537202181,5.1696530886458,126.692338879397));
#237454=CARTESIAN_POINT('Ctrl Pts',(54.5395060964052,-0.665236576618623,
124.23233687071));
#237455=CARTESIAN_POINT('Ctrl Pts',(54.2610584725923,-5.88880632658389,
127.811703624173));
#237456=CARTESIAN_POINT('Ctrl Pts',(53.9826108487795,-5.70085074660091,
134.141175955143));
#237457=CARTESIAN_POINT('Ctrl Pts',(53.7041632249665,-0.274091832533765,
137.40427800337));
#237458=CARTESIAN_POINT('Ctrl Pts',(53.4257156011537,5.40454408550164,134.602378397932));
#237459=CARTESIAN_POINT('Ctrl Pts',(53.1472679773408,6.11666801561766,128.310285995821));
#237460=CARTESIAN_POINT('Ctrl Pts',(52.8688203535278,1.20787285522606,124.310126328773));
#237461=CARTESIAN_POINT('Ctrl Pts',(52.590372729715,-4.81089845124901,126.277850712144));
#237462=CARTESIAN_POINT('Ctrl Pts',(52.3119251059021,-6.40868910648141,
132.405216566294));
#237463=CARTESIAN_POINT('Ctrl Pts',(52.0334774820892,-2.11720755472543,
137.061474009724));
#237464=CARTESIAN_POINT('Ctrl Pts',(51.7550298582764,4.11988430848393,135.967749922743));
#237465=CARTESIAN_POINT('Ctrl Pts',(51.4765822344634,6.57100375973434,130.129123309894));
#237466=CARTESIAN_POINT('Ctrl Pts',(51.1981346106506,2.98369176716867,124.91100679562));
#237467=CARTESIAN_POINT('Ctrl Pts',(50.9196869868376,-3.34548719797895,
125.108594537373));
#237468=CARTESIAN_POINT('Ctrl Pts',(50.6412393630248,-6.60032686431936,
130.540313053181));
#237469=CARTESIAN_POINT('Ctrl Pts',(50.3627917392119,-3.78978858624336,
136.214678381218));
#237470=CARTESIAN_POINT('Ctrl Pts',(50.0843441153989,2.50338026112505,136.917225993175));
#237471=CARTESIAN_POINT('Ctrl Pts',(49.8058964915862,6.49606494544435,132.002348955022));
#237472=CARTESIAN_POINT('Ctrl Pts',(49.5274488677731,4.51918329531533,125.986579159731));
#237473=CARTESIAN_POINT('Ctrl Pts',(49.2490012439603,-1.6106070288309,124.39811516248));
#237474=CARTESIAN_POINT('Ctrl Pts',(48.9705536201474,-6.26032817600901,
128.696677775965));
#237475=CARTESIAN_POINT('Ctrl Pts',(48.6921059963345,-5.15711356346882,
134.932097954848));
#237476=CARTESIAN_POINT('Ctrl Pts',(48.4136583725217,0.685236474895564,
137.374329171949));
#237477=CARTESIAN_POINT('Ctrl Pts',(48.1352107487087,5.89788766849362,133.779080248378));
#237478=CARTESIAN_POINT('Ctrl Pts',(47.8567631248959,5.69066822257687,127.450209307224));
#237479=CARTESIAN_POINT('Ctrl Pts',(47.578315501083,0.254002684709825,124.203639560873));
#237480=CARTESIAN_POINT('Ctrl Pts',(47.29986787727,-5.41607891168467,127.022810002472));
#237481=CARTESIAN_POINT('Ctrl Pts',(47.0214202534572,-6.10904857840509,
133.317040720324));
#237482=CARTESIAN_POINT('Ctrl Pts',(46.7429726296443,-1.18810104518584,
137.302241174989));
#237483=CARTESIAN_POINT('Ctrl Pts',(46.4645250058313,4.82465330659632,135.316206836494));
#237484=CARTESIAN_POINT('Ctrl Pts',(46.1860773820186,6.40378696703385,129.184006238746));
#237485=CARTESIAN_POINT('Ctrl Pts',(45.9076297582056,2.09815324715241,124.54083215642));
#237486=CARTESIAN_POINT('Ctrl Pts',(45.6291821343927,-4.13558080637756,
125.653534739511));
#237487=CARTESIAN_POINT('Ctrl Pts',(45.3507345105798,-6.56891813320061,
131.499594672701));
#237488=CARTESIAN_POINT('Ctrl Pts',(45.072286886767,-2.96574060510383,136.706768473292));
#237489=CARTESIAN_POINT('Ctrl Pts',(44.793839262954,3.36280765460034,136.489917803126));
#237490=CARTESIAN_POINT('Ctrl Pts',(44.5153916391412,6.60109996201359,131.048317834339));
#237491=CARTESIAN_POINT('Ctrl Pts',(44.2369440153282,3.77330388599763,125.38253310131));
#237492=CARTESIAN_POINT('Ctrl Pts',(43.9584963915154,-2.52197412510756,
124.699142984721));
#237493=CARTESIAN_POINT('Ctrl Pts',(43.6800487677024,-6.49968112052436,
129.626149616253));
#237494=CARTESIAN_POINT('Ctrl Pts',(43.4016011438896,-4.50449869325427,
135.635874599185));
#237495=CARTESIAN_POINT('Ctrl Pts',(43.1231535200766,1.6300979761215,137.205674265588));
#237496=CARTESIAN_POINT('Ctrl Pts',(42.8447058962639,6.26671424015497,132.892979411015));
#237497=CARTESIAN_POINT('Ctrl Pts',(42.5662582724509,5.14452626349642,126.660945919963));
#237498=CARTESIAN_POINT('Ctrl Pts',(42.287810648638,-0.705230025235587,
124.236508118946));
#237499=CARTESIAN_POINT('Ctrl Pts',(42.0093630248251,-5.90691437317801,
127.847605906729));
#237500=CARTESIAN_POINT('Ctrl Pts',(41.7309154010123,-5.68043298097947,
134.175816828272));
#237501=CARTESIAN_POINT('Ctrl Pts',(41.4524677771993,-0.233911183839542,
137.405824196969));
#237502=CARTESIAN_POINT('Ctrl Pts',(41.1740201533865,5.42756356405245,134.569409035618));
#237503=CARTESIAN_POINT('Ctrl Pts',(40.8955725295735,6.10137254780096,128.273098310918));
#237504=CARTESIAN_POINT('Ctrl Pts',(40.6171249057607,1.1683182287399,124.302893986988));
#237505=CARTESIAN_POINT('Ctrl Pts',(40.3386772819477,-4.83836346701448,
126.307219882257));
#237506=CARTESIAN_POINT('Ctrl Pts',(40.060229658135,-6.39882550377857,132.444198415735));
#237507=CARTESIAN_POINT('Ctrl Pts',(39.781782034322,-2.07907950257448,137.074246123225));
#237508=CARTESIAN_POINT('Ctrl Pts',(39.5033344105091,4.15123899281517,135.94257535195));
#237509=CARTESIAN_POINT('Ctrl Pts',(39.2248867866962,6.56677165310695,130.089136255519));
#237510=CARTESIAN_POINT('Ctrl Pts',(38.9464391628834,2.94776196882331,124.892953407157));
#237511=CARTESIAN_POINT('Ctrl Pts',(38.6679915390704,-3.38009695863112,
125.129064996863));
#237512=CARTESIAN_POINT('Ctrl Pts',(38.3895439152575,-6.6018119080198,130.58049600839));
#237513=CARTESIAN_POINT('Ctrl Pts',(38.1110962914447,-3.75678423037978,
136.237647659355));
#237514=CARTESIAN_POINT('Ctrl Pts',(37.8326486676317,2.54054462586645,136.901873949744));
#237515=CARTESIAN_POINT('Ctrl Pts',(37.5542010438189,6.50323708344635,131.962783367948));
#237516=CARTESIAN_POINT('Ctrl Pts',(37.275753420006,4.48977236213255,125.959158870647));
#237517=CARTESIAN_POINT('Ctrl Pts',(36.9973057961931,-1.64957382240749,
124.4080380775));
#237518=CARTESIAN_POINT('Ctrl Pts',(36.7188581723802,-6.27304225031618,
128.734825220947));
#237519=CARTESIAN_POINT('Ctrl Pts',(36.4404105485673,-5.13189130533538,
134.96341429146));
#237520=CARTESIAN_POINT('Ctrl Pts',(36.1619629247544,0.725217042420823,
137.370036216732));
#237521=CARTESIAN_POINT('Ctrl Pts',(35.8835153009416,5.91588635701427,133.743123017455));
#237522=CARTESIAN_POINT('Ctrl Pts',(35.6050676771286,5.67014511662727,127.415630739204));
#237523=CARTESIAN_POINT('Ctrl Pts',(35.3266200533158,0.213817516048174,
124.202215670509));
#237524=CARTESIAN_POINT('Ctrl Pts',(35.0481724295028,-5.43899793621292,
127.055849275448));
#237525=CARTESIAN_POINT('Ctrl Pts',(34.76972480569,-6.09363999491508,133.354181678833));
#237526=CARTESIAN_POINT('Ctrl Pts',(34.4912771818771,-1.14852458915375,
137.309353092597));
#237527=CARTESIAN_POINT('Ctrl Pts',(34.2128295580642,4.85202880549439,135.286754208357));
#237528=CARTESIAN_POINT('Ctrl Pts',(33.9343819342512,6.393804762678,129.145054591279));
#237529=CARTESIAN_POINT('Ctrl Pts',(33.6559343104384,2.05998649768791,124.528176150753));
#237530=CARTESIAN_POINT('Ctrl Pts',(33.3774866866255,-4.16685872274224,
125.678804626571));
#237531=CARTESIAN_POINT('Ctrl Pts',(33.0990390628127,-6.56456433933747,
131.539568660782));
#237532=CARTESIAN_POINT('Ctrl Pts',(32.8205914389997,-2.92975602487846,
136.724712420187));
#237533=CARTESIAN_POINT('Ctrl Pts',(32.5421438151868,3.39735494990529,136.469342098247));
#237534=CARTESIAN_POINT('Ctrl Pts',(32.263696191374,6.60246269574222,131.008130545292));
#237535=CARTESIAN_POINT('Ctrl Pts',(31.985248567561,3.74022977242616,125.359664383471));
#237536=CARTESIAN_POINT('Ctrl Pts',(31.7068009437482,-2.55909159136699,
124.714608072585));
#237537=CARTESIAN_POINT('Ctrl Pts',(31.4283533199352,-6.50673280126843,
129.665736849585));
#237538=CARTESIAN_POINT('Ctrl Pts',(31.1499056961224,-4.47500443837311,
135.663205244496));
#237539=CARTESIAN_POINT('Ctrl Pts',(30.8714580723094,1.66903438726656,137.195632795014));
#237540=CARTESIAN_POINT('Ctrl Pts',(30.5930104484966,6.27931214787105,132.854793445461));
#237541=CARTESIAN_POINT('Ctrl Pts',(30.3145628246837,5.11920880603445,126.629706496284));
#237542=CARTESIAN_POINT('Ctrl Pts',(30.0361152008708,-0.745197341294603,
124.240922741373));
#237543=CARTESIAN_POINT('Ctrl Pts',(29.7576675770579,-5.9248035368878,127.883617752917));
#237544=CARTESIAN_POINT('Ctrl Pts',(29.4792199532451,-5.65980472482494,
134.210332770852));
#237545=CARTESIAN_POINT('Ctrl Pts',(29.2007723294321,-0.193721867480399,
137.407125770907));
#237546=CARTESIAN_POINT('Ctrl Pts',(28.9223247056193,5.45038192223944,134.536300158051));
#237547=CARTESIAN_POINT('Ctrl Pts',(28.6438770818064,6.08585099138068,128.236004422871));
#237548=CARTESIAN_POINT('Ctrl Pts',(28.3654294579935,1.12872030979243,124.29590255944));
#237549=CARTESIAN_POINT('Ctrl Pts',(28.0869818341806,-4.86564919544231,
126.336755695574));
#237550=CARTESIAN_POINT('Ctrl Pts',(27.8085342103677,-6.38872479024353,
132.483119500384));
#237551=CARTESIAN_POINT('Ctrl Pts',(27.5300865865548,-2.04087440936798,
137.086785903815));
#237552=CARTESIAN_POINT('Ctrl Pts',(27.2516389627419,4.18243985145892,135.91721038272));
#237553=CARTESIAN_POINT('Ctrl Pts',(26.973191338929,6.56229621234102,130.049175704046));
#237554=CARTESIAN_POINT('Ctrl Pts',(26.6947437151162,2.91172294007416,124.875119068062));
#237555=CARTESIAN_POINT('Ctrl Pts',(26.4162960913032,-3.41458146854746,
125.149745756519));
#237556=CARTESIAN_POINT('Ctrl Pts',(26.1378484674903,-6.60305231915217,
130.620687258984));
#237557=CARTESIAN_POINT('Ctrl Pts',(25.8594008436774,-3.72364066549499,
136.260415605043));
#237558=CARTESIAN_POINT('Ctrl Pts',(25.5809532198646,2.57761484979243,136.886295960714));
#237559=CARTESIAN_POINT('Ctrl Pts',(25.3025055960517,6.51016824160669,131.92317485509));
#237560=CARTESIAN_POINT('Ctrl Pts',(25.0240579722387,4.46019505878377,125.931918122295));
#237561=CARTESIAN_POINT('Ctrl Pts',(24.7456103484259,-1.68847949041943,
124.418198010604));
#237562=CARTESIAN_POINT('Ctrl Pts',(24.467162724613,-6.28552387473587,128.773049353324));
#237563=CARTESIAN_POINT('Ctrl Pts',(24.1887151008001,-5.10647888308236,
134.994576512808));
#237564=CARTESIAN_POINT('Ctrl Pts',(23.9102674769872,0.765170736761864,
137.365499967992));
#237565=CARTESIAN_POINT('Ctrl Pts',(23.6318198531744,5.93366583019039,133.707056889611));
#237566=CARTESIAN_POINT('Ctrl Pts',(23.3533722293614,5.64941190136517,127.381177741815));
#237567=CARTESIAN_POINT('Ctrl Pts',(23.0749246055485,0.173624424299845,
124.201036425055));
#237568=CARTESIAN_POINT('Ctrl Pts',(22.7964769817356,-5.46171541667246,
127.08902745089));
#237569=CARTESIAN_POINT('Ctrl Pts',(22.5180293579228,-6.07800560935413,
133.391228152785));
#237570=CARTESIAN_POINT('Ctrl Pts',(22.2395817341099,-1.10890557412062,
137.316223965318));
#237571=CARTESIAN_POINT('Ctrl Pts',(21.9611341102969,4.87922451068073,135.257135483476));
#237572=CARTESIAN_POINT('Ctrl Pts',(21.6826864864842,6.38358563353538,129.106164430008));
#237573=CARTESIAN_POINT('Ctrl Pts',(21.4042388626712,2.02174341466617,124.515752711409));
#237574=CARTESIAN_POINT('Ctrl Pts',(21.1257912388583,-4.19798223462457,
125.704264442993));
#237575=CARTESIAN_POINT('Ctrl Pts',(20.8473436150454,-6.55996729312864,
131.579515405459));
#237576=CARTESIAN_POINT('Ctrl Pts',(20.5688959912325,-2.89366288146616,
136.742436986267));
#237577=CARTESIAN_POINT('Ctrl Pts',(20.2904483674196,3.43177635497322,136.448556475397));
#237578=CARTESIAN_POINT('Ctrl Pts',(20.0120007436067,6.60358077278748,130.967935705476));
#237579=CARTESIAN_POINT('Ctrl Pts',(19.7335531197938,3.70701706326526,125.336997420853));
#237580=CARTESIAN_POINT('Ctrl Pts',(19.455105495981,-2.59611422954622,124.730298818468));
#237581=CARTESIAN_POINT('Ctrl Pts',(19.176657872168,-6.51354337263571,129.705366275038));
#237582=CARTESIAN_POINT('Ctrl Pts',(18.8982102483552,-4.4453443605568,135.690355843533));
#237583=CARTESIAN_POINT('Ctrl Pts',(18.6197626245423,1.70790895172861,137.1853544935));
#237584=CARTESIAN_POINT('Ctrl Pts',(18.3413150007294,6.29167737336628,132.816531500364));
#237585=CARTESIAN_POINT('Ctrl Pts',(18.0628673769165,5.09370165440758,126.598621765949));
#237586=CARTESIAN_POINT('Ctrl Pts',(17.7844197531036,-0.785137043792105,
124.245580574404));
#237587=CARTESIAN_POINT('Ctrl Pts',(17.5059721292907,-5.94247315482366,
127.919737828307));
#237588=CARTESIAN_POINT('Ctrl Pts',(17.2275245054778,-5.63896674252494,
134.244722503881));
#237589=CARTESIAN_POINT('Ctrl Pts',(16.949076881665,-0.15352537268619,137.408182676953));
#237590=CARTESIAN_POINT('Ctrl Pts',(16.6706292578521,5.47299831451989,134.503052992091));
#237591=CARTESIAN_POINT('Ctrl Pts',(16.3921816340391,6.07010392151387,128.199005706208));
#237592=CARTESIAN_POINT('Ctrl Pts',(16.1137340102263,1.08908056569879,124.289152305198));
#237593=CARTESIAN_POINT('Ctrl Pts',(15.8352863864134,-4.89275462544986,
126.366457057635));
#237594=CARTESIAN_POINT('Ctrl Pts',(15.5568387626005,-6.37838734016194,
132.521978378005));
#237595=CARTESIAN_POINT('Ctrl Pts',(15.2783911387876,-2.00259369080969,
137.099092886824));
#237596=CARTESIAN_POINT('Ctrl Pts',(14.9999435149747,4.21348572825588,135.891655954962));
#237597=CARTESIAN_POINT('Ctrl Pts',(14.7214958911618,6.55757760327567,130.009243136227));
#237598=CARTESIAN_POINT('Ctrl Pts',(14.4430482673489,2.87557601636067,124.857504439193));
#237599=CARTESIAN_POINT('Ctrl Pts',(14.164600643536,-3.44893944989177,125.170636050008));
#237600=CARTESIAN_POINT('Ctrl Pts',(13.8861530197231,-6.60404805175259,
130.660885315664));
#237601=CARTESIAN_POINT('Ctrl Pts',(13.6077053959103,-3.69035911973598,
136.282981374608));
#237602=CARTESIAN_POINT('Ctrl Pts',(13.3292577720973,2.61458955925225,136.870492603333));
#237603=CARTESIAN_POINT('Ctrl Pts',(13.0508101482845,6.5168581630887,131.883524884162));
#237604=CARTESIAN_POINT('Ctrl Pts',(12.7723625244716,4.43045248126686,125.904857924092));
#237605=CARTESIAN_POINT('Ctrl Pts',(12.4939149006587,-1.72732259120293,
124.428594585312));
#237606=CARTESIAN_POINT('Ctrl Pts',(12.2154672768458,-6.29777258675688,
128.811348756686));
#237607=CARTESIAN_POINT('Ctrl Pts',(11.9370196530329,-5.08087723837641,
135.025583464166));
#237608=CARTESIAN_POINT('Ctrl Pts',(11.65857202922,0.805096077419857,137.36072059382));
#237609=CARTESIAN_POINT('Ctrl Pts',(11.3801244054071,5.95122542919731,133.670883201288));
#237610=CARTESIAN_POINT('Ctrl Pts',(11.1016767815943,5.62846934506734,127.346851591727));
#237611=CARTESIAN_POINT('Ctrl Pts',(10.8232291577813,0.13342489883439,124.200101868207));
#237612=CARTESIAN_POINT('Ctrl Pts',(10.5447815339684,-5.4842305112587,127.12234329937));
#237613=CARTESIAN_POINT('Ctrl Pts',(10.2663339101556,-6.06214600106014,
133.428178769409));
#237614=CARTESIAN_POINT('Ctrl Pts',(9.98788628634267,-1.06924546818365,
137.322853538546));
#237615=CARTESIAN_POINT('Ctrl Pts',(9.70943866252976,4.90623941440849,135.227351759386));
#237616=CARTESIAN_POINT('Ctrl Pts',(9.43099103871685,6.37312995827954,129.067337196021));
#237617=CARTESIAN_POINT('Ctrl Pts',(9.15254341490403,1.98342541519871,124.503562298745));
#237618=CARTESIAN_POINT('Ctrl Pts',(8.87409579109107,-4.22895018873139,
125.729913245354));
#237619=CARTESIAN_POINT('Ctrl Pts',(8.59564816727821,-6.55512716491932,
131.61943342649));
#237620=CARTESIAN_POINT('Ctrl Pts',(8.31720054346528,-2.85746251231165,
136.759941514744));
#237621=CARTESIAN_POINT('Ctrl Pts',(8.03875291965246,3.46607059430627,136.427561704794));
#237622=CARTESIAN_POINT('Ctrl Pts',(7.76030529583951,6.60445415171875,130.927734804324));
#237623=CARTESIAN_POINT('Ctrl Pts',(7.48185767202662,3.67366698922382,125.314533053388));
#237624=CARTESIAN_POINT('Ctrl Pts',(7.20341004821377,-2.63304066775796,
124.746214640945));
#237625=CARTESIAN_POINT('Ctrl Pts',(6.92496242440086,-6.52011258225796,
129.745036424131));
#237626=CARTESIAN_POINT('Ctrl Pts',(6.64651480058794,-4.41551955887045,
135.71732539022));
#237627=CARTESIAN_POINT('Ctrl Pts',(6.36806717677509,1.74672022899638,137.174839741911));
#237628=CARTESIAN_POINT('Ctrl Pts',(6.08961955296221,6.30380945844269,132.778194993536));
#237629=CARTESIAN_POINT('Ctrl Pts',(5.81117192914928,5.06800575379271,126.567692880813));
#237630=CARTESIAN_POINT('Ctrl Pts',(5.53272430533639,-0.825047652747706,
124.250481445441));
#237631=CARTESIAN_POINT('Ctrl Pts',(5.25427668152353,-5.95992257223146,
127.955964794454));
#237632=CARTESIAN_POINT('Ctrl Pts',(4.97582905771062,-5.61791980623858,
134.278984753035));
#237633=CARTESIAN_POINT('Ctrl Pts',(4.69738143389771,-0.113323188952861,
137.408994875945));
#237634=CARTESIAN_POINT('Ctrl Pts',(4.41893381008486,5.49541190283514,134.469668769726));
#237635=CARTESIAN_POINT('Ctrl Pts',(4.14048618627195,6.05413192171396,128.162103531929));
#237636=CARTESIAN_POINT('Ctrl Pts',(3.86203856245905,1.0494004653243,124.282643474398));
#237637=CARTESIAN_POINT('Ctrl Pts',(3.58359093864613,-4.91967875263547,
126.396322867843));
#237638=CARTESIAN_POINT('Ctrl Pts',(3.30514331483329,-6.36781353659179,
132.560773608667));
#237639=CARTESIAN_POINT('Ctrl Pts',(3.02669569102039,-1.96423876540577,
137.111166616214));
#237640=CARTESIAN_POINT('Ctrl Pts',(2.74824806720748,4.24437547278969,135.865913015604));
#237641=CARTESIAN_POINT('Ctrl Pts',(2.46980044339459,6.55261600076067,129.969340031779));
#237642=CARTESIAN_POINT('Ctrl Pts',(2.19135281958173,2.83932253712042,124.840110173268));
#237643=CARTESIAN_POINT('Ctrl Pts',(1.91290519576881,-3.48316962951642,
125.191735103234));
#237644=CARTESIAN_POINT('Ctrl Pts',(1.6344575719559,-6.60479906892382,130.701088688872));
#237645=CARTESIAN_POINT('Ctrl Pts',(1.35600994814304,-3.65694082636265,
136.305344131865));
#237646=CARTESIAN_POINT('Ctrl Pts',(1.07756232433016,2.65146738413444,136.854464463202));
#237647=CARTESIAN_POINT('Ctrl Pts',(0.799114700517227,6.52330659999492,
131.843834924404));
#237648=CARTESIAN_POINT('Ctrl Pts',(0.520667076704378,4.40054573170394,
125.877979278764));
#237649=CARTESIAN_POINT('Ctrl Pts',(0.242219452891471,-1.76610168541259,
124.439227416375));
#237650=CARTESIAN_POINT('Ctrl Pts',(-0.03622817092143,-6.30978793249869,
128.849722011837));
#237651=CARTESIAN_POINT('Ctrl Pts',(-0.314675794734322,-5.05508731989592,
135.056433996558));
#237652=CARTESIAN_POINT('Ctrl Pts',(-0.593123418547181,0.844991584946641,
137.355698271319));
#237653=CARTESIAN_POINT('Ctrl Pts',(-0.871571042360099,5.96856450335716,
133.634603292916));
#237654=CARTESIAN_POINT('Ctrl Pts',(-1.15001866617301,5.60731822376822,
127.312653560908));
#237655=CARTESIAN_POINT('Ctrl Pts',(-1.42846628998586,0.0932204292604712,
124.199412034595));
#237656=CARTESIAN_POINT('Ctrl Pts',(-1.70691391379876,-5.50654238566651,
127.155795586355));
#237657=CARTESIAN_POINT('Ctrl Pts',(-1.98536153761166,-6.04606175771675,
133.465032159487));
#237658=CARTESIAN_POINT('Ctrl Pts',(-2.26380916142456,-1.02954574096264,
137.329241566624));
#237659=CARTESIAN_POINT('Ctrl Pts',(-2.5422567852374,4.9330725156305,135.197404139731));
#237660=CARTESIAN_POINT('Ctrl Pts',(-2.82070440905033,6.36243812434939,
129.028574328076));
#237661=CARTESIAN_POINT('Ctrl Pts',(-3.09915203286324,1.94503391917308,
124.491605364478));
#237662=CARTESIAN_POINT('Ctrl Pts',(-3.3775996566761,-4.25976143753379,
125.755750083229));
#237663=CARTESIAN_POINT('Ctrl Pts',(-3.65604728048899,-6.55004413406227,
131.659321244699));
#237664=CARTESIAN_POINT('Ctrl Pts',(-3.9344949043019,-2.82115625883292,
136.777225356981));
#237665=CARTESIAN_POINT('Ctrl Pts',(-4.2129425281148,3.50023639711881,136.406358564405));
#237666=CARTESIAN_POINT('Ctrl Pts',(-4.49139015192765,6.60508280017262,
130.887529331496));
#237667=CARTESIAN_POINT('Ctrl Pts',(-4.76983777574057,3.64018078610111,
125.292272113504));
#237668=CARTESIAN_POINT('Ctrl Pts',(-5.04828539955349,-2.66986953767946,
124.762354950249));
#237669=CARTESIAN_POINT('Ctrl Pts',(-5.32673302336633,-6.52644018671072,
129.784745826872));
#237670=CARTESIAN_POINT('Ctrl Pts',(-5.60518064717923,-4.38553113848304,
135.74411288519));
#237671=CARTESIAN_POINT('Ctrl Pts',(-5.88362827099213,1.7854667809037,137.164088929876));
#237672=CARTESIAN_POINT('Ctrl Pts',(-6.16207589480503,6.31570795354138,
132.739785345549));
#237673=CARTESIAN_POINT('Ctrl Pts',(-6.44052351861788,5.04212205636089,
126.536920986959));
#237674=CARTESIAN_POINT('Ctrl Pts',(-6.71897114243081,-0.864927689259141,
124.255625172881));
#237675=CARTESIAN_POINT('Ctrl Pts',(-6.99741876624371,-5.97715114251656,
127.992297308957));
#237676=CARTESIAN_POINT('Ctrl Pts',(-7.27586639005655,-5.59666469586782,
134.313118248714));
#237677=CARTESIAN_POINT('Ctrl Pts',(-7.55431401386947,-0.0731168059870705,
137.409562337785));
#237678=CARTESIAN_POINT('Ctrl Pts',(-7.83276163768236,5.51762185664139,
134.436148728019));
#237679=CARTESIAN_POINT('Ctrl Pts',(-8.11120926149529,6.03793558382929,
128.125299267457));
#237680=CARTESIAN_POINT('Ctrl Pts',(-8.38965688530811,1.00968147902963,
124.276376308223));
#237681=CARTESIAN_POINT('Ctrl Pts',(-8.66810450912106,-4.94642057931569,
126.426352019512));
#237682=CARTESIAN_POINT('Ctrl Pts',(-8.94655213293394,-6.3570037713493,
132.599503754801));
#237683=CARTESIAN_POINT('Ctrl Pts',(-9.22499975674682,-1.92581105441205,
137.123006644589));
#237684=CARTESIAN_POINT('Ctrl Pts',(-9.50344738055969,4.27510794042973,
135.839982518561));
#237685=CARTESIAN_POINT('Ctrl Pts',(-9.78189500437264,6.54741158865002,
129.929467869325));
#237686=CARTESIAN_POINT('Ctrl Pts',(-10.0603426281855,2.80296384573913,
124.822936914835));
#237687=CARTESIAN_POINT('Ctrl Pts',(-10.3387902519984,-3.51727073900952,
125.213042134361));
#237688=CARTESIAN_POINT('Ctrl Pts',(-10.6172378758113,-6.60530534283666,
130.74129588886));
#237689=CARTESIAN_POINT('Ctrl Pts',(-10.8956854996242,-3.62338702370218,
136.327503048155));
#237690=CARTESIAN_POINT('Ctrl Pts',(-11.174133123437,2.68824695791763,136.838212134247));
#237691=CARTESIAN_POINT('Ctrl Pts',(-11.4525807472499,6.52951331337615,
131.804106446543));
#237692=CARTESIAN_POINT('Ctrl Pts',(-11.7310283710628,4.37047591830066,
125.851283182307));
#237693=CARTESIAN_POINT('Ctrl Pts',(-12.0094759948757,-1.80481533607482,
124.450096109789));
#237694=CARTESIAN_POINT('Ctrl Pts',(-12.2879236186886,-6.32156946672825,
128.88816769684));
#237695=CARTESIAN_POINT('Ctrl Pts',(-12.5663712425015,-5.02911008329581,
135.087126966809));
#237696=CARTESIAN_POINT('Ctrl Pts',(-12.8448188663144,0.884855780999501,
137.350433186591));
#237697=CARTESIAN_POINT('Ctrl Pts',(-13.1232664901273,5.98568241016441,
133.598218508862));
#237698=CARTESIAN_POINT('Ctrl Pts',(-13.4017141139402,5.58595932123025,
127.278584916578));
#237699=CARTESIAN_POINT('Ctrl Pts',(-13.6801617377531,0.0530125053692662,
124.198966949783));
#237700=CARTESIAN_POINT('Ctrl Pts',(-13.958609361566,-5.5286502131212,127.189383072259));
#237701=CARTESIAN_POINT('Ctrl Pts',(-14.2370569853788,-6.02975347533148,
133.501786957402));
#237702=CARTESIAN_POINT('Ctrl Pts',(-14.5155046091917,-0.989807863545592,
137.335387812837));
#237703=CARTESIAN_POINT('Ctrl Pts',(-14.7939522330047,4.95972282003631,
135.167293734234));
#237704=CARTESIAN_POINT('Ctrl Pts',(-15.0723998568175,6.35151052793477,
128.989877262545));
#237705=CARTESIAN_POINT('Ctrl Pts',(-15.3508474806304,1.9065703492003,124.479882351679));
#237706=CARTESIAN_POINT('Ctrl Pts',(-15.6292951044433,-4.29041483930959,
125.781773999224));
#237707=CARTESIAN_POINT('Ctrl Pts',(-15.9077427282562,-6.54471838891106,
131.699177382027));
#237708=CARTESIAN_POINT('Ctrl Pts',(-16.186190352069,-2.78474546637155,
136.794287872519));
#237709=CARTESIAN_POINT('Ctrl Pts',(-16.464637975882,3.53427249738445,136.384947839923));
#237710=CARTESIAN_POINT('Ctrl Pts',(-16.7430855996949,6.60546669485434,
130.847320776822));
#237711=CARTESIAN_POINT('Ctrl Pts',(-17.0215332235078,3.6065596947407,125.270215426085));
#237712=CARTESIAN_POINT('Ctrl Pts',(-17.2999808473206,-2.7065994746034,
124.778719148295));
#237713=CARTESIAN_POINT('Ctrl Pts',(-17.5784284711336,-6.53252595152224,
129.824493011814));
#237714=CARTESIAN_POINT('Ctrl Pts',(-17.8568760949464,-4.35538021062653,
135.770717335825));
#237715=CARTESIAN_POINT('Ctrl Pts',(-18.1353237187593,1.82414717168286,
137.153102455769));
#237716=CARTESIAN_POINT('Ctrl Pts',(-18.4137713425722,6.32737241775927,
132.701303979686));
#237717=CARTESIAN_POINT('Ctrl Pts',(-18.6922189663851,5.01605152124203,
126.506307224649));
#237718=CARTESIAN_POINT('Ctrl Pts',(-18.9706665901979,-0.904775675556959,
124.261011566121));
#237719=CARTESIAN_POINT('Ctrl Pts',(-19.2491142140109,-5.99415822726801,
128.028734025499));
#237720=CARTESIAN_POINT('Ctrl Pts',(-19.5275618378238,-5.57520219902858,
134.347121726088));
#237721=CARTESIAN_POINT('Ctrl Pts',(-19.8060094616367,-0.0329077136511566,
137.409885041447));
#237722=CARTESIAN_POINT('Ctrl Pts',(-20.0844570854496,5.53962735294063,
134.402494109067));
#237723=CARTESIAN_POINT('Ctrl Pts',(-20.3629047092624,6.02151550802112,
128.08859427659));
#237724=CARTESIAN_POINT('Ctrl Pts',(-20.6413523330754,0.969925078616457,
124.270351038909));
#237725=CARTESIAN_POINT('Ctrl Pts',(-20.9197999568882,-4.9729791145623,
126.456543399899));
#237726=CARTESIAN_POINT('Ctrl Pts',(-21.1982475807011,-6.34595844499429,
132.638167381246));
#237727=CARTESIAN_POINT('Ctrl Pts',(-21.476695204514,-1.88731198178147,
137.134612533211));
#237728=CARTESIAN_POINT('Ctrl Pts',(-21.7551428283269,4.30568199237261,
135.813865424697));
#237729=CARTESIAN_POINT('Ctrl Pts',(-22.0335904521398,6.54196455979519,
129.889628126344));
#237730=CARTESIAN_POINT('Ctrl Pts',(-22.3120380759527,2.766501289502,124.805985300257));
#237731=CARTESIAN_POINT('Ctrl Pts',(-22.5904856997656,-3.5512415147419,
125.234556353852));
#237732=CARTESIAN_POINT('Ctrl Pts',(-22.8689333235784,-6.60556685473091,
130.781505425734));
#237733=CARTESIAN_POINT('Ctrl Pts',(-23.1473809473914,-3.58969895510304,
136.349457302372));
#237734=CARTESIAN_POINT('Ctrl Pts',(-23.4258285712042,2.7249269177212,136.821736218705));
#237735=CARTESIAN_POINT('Ctrl Pts',(-23.7042761950172,6.53547807324032,
131.764340922733));
#237736=CARTESIAN_POINT('Ctrl Pts',(-23.98272381883,4.34024415530499,125.824770623956));
#237737=CARTESIAN_POINT('Ctrl Pts',(-24.2611714426429,-1.84346210864104,
124.461200262812));
#237738=CARTESIAN_POINT('Ctrl Pts',(-24.5396190664558,-6.33311675287646,
128.926684387076));
#237739=CARTESIAN_POINT('Ctrl Pts',(-24.8180666902687,-5.00294649117208,
135.117661237576));
#237740=CARTESIAN_POINT('Ctrl Pts',(-25.0965143140816,0.924687188395989,
137.344925534737));
#237741=CARTESIAN_POINT('Ctrl Pts',(-25.3749619378945,6.00257851530871,
133.561730197376));
#237742=CARTESIAN_POINT('Ctrl Pts',(-25.6534095617074,5.56439342891538,
127.244646921163));
#237743=CARTESIAN_POINT('Ctrl Pts',(-25.9318571855203,0.0128026170801758,
124.198766630261));
#237744=CARTESIAN_POINT('Ctrl Pts',(-26.2103048093331,-5.5505531744091,
127.223104512485));
#237745=CARTESIAN_POINT('Ctrl Pts',(-26.4887524331461,-6.01322175821376,
133.538441801192));
#237746=CARTESIAN_POINT('Ctrl Pts',(-26.7672000569589,-0.950033308434149,
137.341292049436));
#237747=CARTESIAN_POINT('Ctrl Pts',(-27.0456476807718,4.98618934008908,
135.137021658645));
#237748=CARTESIAN_POINT('Ctrl Pts',(-27.3240953045847,6.34034757396176,
128.951247433362));
#237749=CARTESIAN_POINT('Ctrl Pts',(-27.6025429283976,1.86803613056208,
124.468393694749));
#237750=CARTESIAN_POINT('Ctrl Pts',(-27.8809905522105,-4.32090925818572,
125.807984029013));
#237751=CARTESIAN_POINT('Ctrl Pts',(-28.1594381760234,-6.53915012681315,
131.739000361591));
#237752=CARTESIAN_POINT('Ctrl Pts',(-28.4378857998363,-2.74823148414282,
136.811128429099));
#237753=CARTESIAN_POINT('Ctrl Pts',(-28.7163334236492,3.56817763388296,
136.36333032473));
#237754=CARTESIAN_POINT('Ctrl Pts',(-28.994781047462,6.60560582153853,130.807110630244));
#237755=CARTESIAN_POINT('Ctrl Pts',(-29.273228671275,3.5728049609845,125.248363808452));
#237756=CARTESIAN_POINT('Ctrl Pts',(-29.5516762950878,-2.74322911748845,
124.795306628702));
#237757=CARTESIAN_POINT('Ctrl Pts',(-29.8301239189007,-6.53836965118233,
129.86427650611));
#237758=CARTESIAN_POINT('Ctrl Pts',(-30.1085715427137,-4.32506789255462,
135.797137756284));
#237759=CARTESIAN_POINT('Ctrl Pts',(-30.3870191665265,1.862759968018,137.141880726698));
#237760=CARTESIAN_POINT('Ctrl Pts',(-30.6654667903394,6.33880241886542,
132.662752321889));
#237761=CARTESIAN_POINT('Ctrl Pts',(-30.9439144141524,4.98979511448915,
126.475852728289));
#237762=CARTESIAN_POINT('Ctrl Pts',(-31.2223620379652,-0.944590135059391,
124.266640425567));
#237763=CARTESIAN_POINT('Ctrl Pts',(-31.5008096617781,-6.01094319628198,
128.065273593905));
#237764=CARTESIAN_POINT('Ctrl Pts',(-31.7792572855909,-5.55353311102158,
134.380993925146));
#237765=CARTESIAN_POINT('Ctrl Pts',(-32.0577049094039,0.00730259809219468,
137.409962974972));
#237766=CARTESIAN_POINT('Ctrl Pts',(-32.3361525332168,5.56142757631112,
134.368706159956));
#237767=CARTESIAN_POINT('Ctrl Pts',(-32.6146001570296,6.0048723027414,128.051989919443));
#237768=CARTESIAN_POINT('Ctrl Pts',(-32.8930477808425,0.930132737272799,
124.264567889721));
#237769=CARTESIAN_POINT('Ctrl Pts',(-33.1714954046555,-4.99935337423901,
126.486895890252));
#237770=CARTESIAN_POINT('Ctrl Pts',(-33.4499430284683,-6.33467796681538,
132.676763055306));
#237771=CARTESIAN_POINT('Ctrl Pts',(-33.7283906522812,-1.84874297411136,
137.145983852021));
#237772=CARTESIAN_POINT('Ctrl Pts',(-34.0068382760941,4.33609649568588,
135.787562701789));
#237773=CARTESIAN_POINT('Ctrl Pts',(-34.285285899907,6.53627511603778,129.849822279112));
#237774=CARTESIAN_POINT('Ctrl Pts',(-34.5637335237199,2.72993621954223,
124.789255957683));
#237775=CARTESIAN_POINT('Ctrl Pts',(-34.8421811475328,-3.58508069791401,
125.256276964487));
#237776=CARTESIAN_POINT('Ctrl Pts',(-35.1206287713457,-6.60558359491616,
130.821715809516));
#237777=CARTESIAN_POINT('Ctrl Pts',(-35.3990763951586,-3.55587786888901,
136.37120608099));
#237778=CARTESIAN_POINT('Ctrl Pts',(-35.6775240189714,2.76150590435573,
136.805037327097));
#237779=CARTESIAN_POINT('Ctrl Pts',(-35.9559716427844,6.54120065856107,
131.724539826499));
#237780=CARTESIAN_POINT('Ctrl Pts',(-36.2344192665972,4.30985156296601,
125.798442586144));
#237781=CARTESIAN_POINT('Ctrl Pts',(-36.5128668904101,-1.8820405710409,
124.472539463974));
#237782=CARTESIAN_POINT('Ctrl Pts',(-36.791314514223,-6.3444293630544,128.965270655295));
#237783=CARTESIAN_POINT('Ctrl Pts',(-37.0697621380359,-4.9765975130263,
135.148035677403));
#237784=CARTESIAN_POINT('Ctrl Pts',(-37.3482097618488,0.964484331168655,
137.339175519844));
#237785=CARTESIAN_POINT('Ctrl Pts',(-37.6266573856617,6.0192521926987,133.525139710547));
#237786=CARTESIAN_POINT('Ctrl Pts',(-37.9051050094746,5.54262134595571,
127.210840832248));
#237787=CARTESIAN_POINT('Ctrl Pts',(-38.1835526332875,-0.0274077456145885,
124.198811083455));
#237788=CARTESIAN_POINT('Ctrl Pts',(-38.4620002571004,-5.5722504579079,
127.256958657474));
#237789=CARTESIAN_POINT('Ctrl Pts',(-38.7404478809132,-5.99646721895241,
133.574995332598));
#237790=CARTESIAN_POINT('Ctrl Pts',(-39.0188955047262,-0.910223549489097,
137.346954057637));
#237791=CARTESIAN_POINT('Ctrl Pts',(-39.297343128539,5.0124710950622,135.106589034709));
#237792=CARTESIAN_POINT('Ctrl Pts',(-39.5757907523519,6.32894967607775,
128.912686271968));
#237793=CARTESIAN_POINT('Ctrl Pts',(-39.8542383761648,1.82943269115809,
124.457139819403));
#237794=CARTESIAN_POINT('Ctrl Pts',(-40.1326859999777,-4.35124356418029,
125.834379201373));
#237795=CARTESIAN_POINT('Ctrl Pts',(-40.4111336237906,-6.53333955410249,
131.778788707735));
#237796=CARTESIAN_POINT('Ctrl Pts',(-40.6895812476035,-2.7116156651858,
136.827746402689));
#237797=CARTESIAN_POINT('Ctrl Pts',(-40.9680288714165,3.60195055024708,
136.34150681987));
#237798=CARTESIAN_POINT('Ctrl Pts',(-41.2464764952292,6.60550017506977,
130.766900381762));
#237799=CARTESIAN_POINT('Ctrl Pts',(-41.5249241190422,3.53891783562657,
125.226718070324));
#237800=CARTESIAN_POINT('Ctrl Pts',(-41.803371742855,-2.77975710900975,
124.812116776814));
#237801=CARTESIAN_POINT('Ctrl Pts',(-42.081819366668,-6.5439710691505,129.904094835568));
#237802=CARTESIAN_POINT('Ctrl Pts',(-42.3602669904808,-4.2945953075014,
135.82337316755));
#237803=CARTESIAN_POINT('Ctrl Pts',(-42.6387146142937,1.90130373909722,
137.130424158489));
#237804=CARTESIAN_POINT('Ctrl Pts',(-42.9171622381066,6.34999753331677,
132.624131800705));
#237805=CARTESIAN_POINT('Ctrl Pts',(-43.1956098619195,4.96335380904355,
126.44555862638));
#237806=CARTESIAN_POINT('Ctrl Pts',(-43.4740574857324,-0.984369592426984,
124.272511542639));
#237807=CARTESIAN_POINT('Ctrl Pts',(-43.7525051095453,-6.02750542758532,
128.101914660188));
#237808=CARTESIAN_POINT('Ctrl Pts',(-44.0309527333582,-5.53165823480283,
134.414733590743));
#237809=CARTESIAN_POINT('Ctrl Pts',(-44.3094003571711,0.0475126392350714,
137.409796135472));
#237810=CARTESIAN_POINT('Ctrl Pts',(-44.5878479809839,5.58302171893757,
134.334786132711));
#237811=CARTESIAN_POINT('Ctrl Pts',(-44.8662956047969,5.98800658471021,
128.015487552405));
#237812=CARTESIAN_POINT('Ctrl Pts',(-45.1447432286098,0.890305929518511,
124.259027074959));
#237813=CARTESIAN_POINT('Ctrl Pts',(-45.4231908524226,-5.02554238103793,
126.517408365848));
#237814=CARTESIAN_POINT('Ctrl Pts',(-45.7016384762356,-6.32316275481482,
132.715289346806));
#237815=CARTESIAN_POINT('Ctrl Pts',(-45.9800861000484,-1.81010546059046,
137.15712017965));
#237816=CARTESIAN_POINT('Ctrl Pts',(-46.2585337238614,4.36635032334889,
135.761075324496));
#237817=CARTESIAN_POINT('Ctrl Pts',(-46.5369813476741,6.53034346820225,
129.810051802649));
#237818=CARTESIAN_POINT('Ctrl Pts',(-46.8154289714873,2.6932699907919,124.772749507024));
#237819=CARTESIAN_POINT('Ctrl Pts',(-47.0938765952999,-3.61878703460243,
125.278203161403));
#237820=CARTESIAN_POINT('Ctrl Pts',(-47.3723242191129,-6.60535556277213,
130.861925550195));
#237821=CARTESIAN_POINT('Ctrl Pts',(-47.6507718429257,-3.52192501831287,
136.392748578105));
#237822=CARTESIAN_POINT('Ctrl Pts',(-47.9292194667387,2.79798256237344,
136.788116078208));
#237823=CARTESIAN_POINT('Ctrl Pts',(-48.2076670905515,6.54668085728591,
131.684704632686));
#237824=CARTESIAN_POINT('Ctrl Pts',(-48.4861147143645,4.27929926749242,
125.772300044465));
#237825=CARTESIAN_POINT('Ctrl Pts',(-48.7645623381774,-1.92054929373528,
124.484113293097));
#237826=CARTESIAN_POINT('Ctrl Pts',(-49.0430099619902,-6.35550687806913,
129.003925071669));
#237827=CARTESIAN_POINT('Ctrl Pts',(-49.3214575858032,-4.95006412522954,
135.178249160753));
#237828=CARTESIAN_POINT('Ctrl Pts',(-49.5999052096159,1.00424573461974,
137.333183354982));
#237829=CARTESIAN_POINT('Ctrl Pts',(-49.878352833429,6.03570282448511,133.488448404247));
#237830=CARTESIAN_POINT('Ctrl Pts',(-50.1568004572417,5.52064387912377,
127.17716790253));
#237831=CARTESIAN_POINT('Ctrl Pts',(-50.4352480810547,-0.0676170927052693,
124.199100307716));
#237832=CARTESIAN_POINT('Ctrl Pts',(-50.7136957048675,-5.5937412596168,
127.290944252747));
#237833=CARTESIAN_POINT('Ctrl Pts',(-50.9921433286805,-5.97949047839309,
133.611446197116));
#237834=CARTESIAN_POINT('Ctrl Pts',(-51.2705909524933,-0.870380061875472,
137.352373627632));
#237835=CARTESIAN_POINT('Ctrl Pts',(-51.5490385763063,5.03856711107574,
135.075996990117));
#237836=CARTESIAN_POINT('Ctrl Pts',(-51.8274862001192,6.31731725663583,
128.874195207264));
#237837=CARTESIAN_POINT('Ctrl Pts',(-52.105933823932,1.79076146145295,124.446121142656));
#237838=CARTESIAN_POINT('Ctrl Pts',(-52.3843814477449,-4.38141663324442,
125.860958538224));
#237839=CARTESIAN_POINT('Ctrl Pts',(-52.6628290715579,-6.52728688609205,
131.818540946088));
#237840=CARTESIAN_POINT('Ctrl Pts',(-52.9412766953706,-2.67489936631311,
136.844141177504));
#237841=CARTESIAN_POINT('Ctrl Pts',(-53.2197243191836,3.63558999500893,
136.319478134021));
#237842=CARTESIAN_POINT('Ctrl Pts',(-53.4981719429964,6.60514975936288,
130.726691521383));
#237843=CARTESIAN_POINT('Ctrl Pts',(-53.7766195668094,3.50489957436681,
125.205279013792));
#237844=CARTESIAN_POINT('Ctrl Pts',(-54.0550671906223,-2.8161820956091,
124.829148969725));
#237845=CARTESIAN_POINT('Ctrl Pts',(-54.3335148144351,-6.54932999786417,
129.943946524707));
#237846=CARTESIAN_POINT('Ctrl Pts',(-54.6119624382481,-4.26396358463975,
135.849422597461));
#237847=CARTESIAN_POINT('Ctrl Pts',(-54.890410062061,1.93977705666721,137.11873317567));
#237848=CARTESIAN_POINT('Ctrl Pts',(-55.1688576858738,6.3609573462743,132.58544384723));
#237849=CARTESIAN_POINT('Ctrl Pts',(-55.4473053096868,4.93672858469731,
126.415426041482));
#237850=CARTESIAN_POINT('Ctrl Pts',(-55.7257529334997,-1.02411257361735,
124.278624699781));
#237851=CARTESIAN_POINT('Ctrl Pts',(-56.0042005573125,-6.0438443074584,
128.138655866601));
#237852=CARTESIAN_POINT('Ctrl Pts',(-56.2826481811254,-5.50957838095395,
134.448339472641));
#237853=CARTESIAN_POINT('Ctrl Pts',(-56.5610958049383,0.0877209197796484,
137.40938452913));
#237854=CARTESIAN_POINT('Ctrl Pts',(-56.8395434287512,5.60440898064107,
134.300735284249));
#237855=CARTESIAN_POINT('Ctrl Pts',(-57.117991052564,5.97091897889293,127.979088528083));
#237856=CARTESIAN_POINT('Ctrl Pts',(-57.396438676377,0.850446131150592,
124.253728799937));
#237857=CARTESIAN_POINT('Ctrl Pts',(-57.6748863001899,-5.05154516451579,
126.548079696037));
#237858=CARTESIAN_POINT('Ctrl Pts',(-57.9533339240027,-6.31141323569307,
132.753744828139));
#237859=CARTESIAN_POINT('Ctrl Pts',(-58.2317815478157,-1.77140087294607,
137.168021103437));
#237860=CARTESIAN_POINT('Ctrl Pts',(-58.5102291716285,4.39644235429495,
135.734404274317));
#237861=CARTESIAN_POINT('Ctrl Pts',(-58.7886767954414,6.52416983608798,
129.770318170665));
#237862=CARTESIAN_POINT('Ctrl Pts',(-59.0671244192543,2.65650396193163,
124.756466559932));
#237863=CARTESIAN_POINT('Ctrl Pts',(-59.3455720430672,-3.6523592758065,
125.300334132115));
#237864=CARTESIAN_POINT('Ctrl Pts',(-59.62401966688,-6.60488276674858,130.902133157784));
#237865=CARTESIAN_POINT('Ctrl Pts',(-59.902467290693,-3.48784166150989,
136.414083995446));
#237866=CARTESIAN_POINT('Ctrl Pts',(-60.1809149145059,2.83435554011865,
136.770973099059));
#237867=CARTESIAN_POINT('Ctrl Pts',(-60.4593625383188,6.55191846634393,
131.644836817403));
#237868=CARTESIAN_POINT('Ctrl Pts',(-60.7378101621316,4.24858840101079,
125.746343967642));
#237869=CARTESIAN_POINT('Ctrl Pts',(-61.0162577859445,-1.95898684976931,
124.49592132131));
#237870=CARTESIAN_POINT('Ctrl Pts',(-61.2947054097575,-6.36634888743926,
129.042646203845));
#237871=CARTESIAN_POINT('Ctrl Pts',(-61.5731530335703,-4.92334731098624,
135.208300568055));
#237872=CARTESIAN_POINT('Ctrl Pts',(-61.8516006573832,1.04396992537583,
137.326949262193));
#237873=CARTESIAN_POINT('Ctrl Pts',(-62.1300482811962,6.05192980108374,
133.451657638088));
#237874=CARTESIAN_POINT('Ctrl Pts',(-62.408495905009,5.49846184280268,127.143629379772));
#237875=CARTESIAN_POINT('Ctrl Pts',(-62.6869435288219,-0.107823934219708,
124.199634292325));
#237876=CARTESIAN_POINT('Ctrl Pts',(-62.9653911526347,-5.61502478318622,
127.325060038955));
#237877=CARTESIAN_POINT('Ctrl Pts',(-63.2438387764477,-5.96229216561512,
133.647793044045));
#237878=CARTESIAN_POINT('Ctrl Pts',(-63.5222864002605,-0.830504322008783,
137.357550558596));
#237879=CARTESIAN_POINT('Ctrl Pts',(-63.8007340240734,5.06447642113188,
135.045246658467));
#237880=CARTESIAN_POINT('Ctrl Pts',(-64.0791816478864,6.30545074667997,
128.835775665549));
#237881=CARTESIAN_POINT('Ctrl Pts',(-64.3576292716992,1.75202387442331,
124.435338072814));
#237882=CARTESIAN_POINT('Ctrl Pts',(-64.6360768955121,-4.41142734730395,
125.887721054655));
#237883=CARTESIAN_POINT('Ctrl Pts',(-64.914524519325,-6.52099234706562,
131.858255603616));
#237884=CARTESIAN_POINT('Ctrl Pts',(-65.1929721431379,-2.63808394806071,
136.860312146029));
#237885=CARTESIAN_POINT('Ctrl Pts',(-65.4714197669508,3.66909472164654,
136.297245083462));
#237886=CARTESIAN_POINT('Ctrl Pts',(-65.7498673907637,6.60455458740261,
130.686485539062));
#237887=CARTESIAN_POINT('Ctrl Pts',(-66.0283150145766,3.4707514377644,125.184047433287));
#237888=CARTESIAN_POINT('Ctrl Pts',(-66.3067626383895,-2.85250272754526,
124.846402576302));
#237889=CARTESIAN_POINT('Ctrl Pts',(-66.5852102622024,-6.55444623874626,
129.983830096806));
#237890=CARTESIAN_POINT('Ctrl Pts',(-66.8636578860152,-4.23317385903938,
135.875285080744));
#237891=CARTESIAN_POINT('Ctrl Pts',(-67.1421055098281,1.978178495085,137.106808211453));
#237892=CARTESIAN_POINT('Ctrl Pts',(-67.4205531336411,6.37168145161813,
132.546689895061));
#237893=CARTESIAN_POINT('Ctrl Pts',(-67.6990007574539,4.90992042805787,
126.385456090168));
#237894=CARTESIAN_POINT('Ctrl Pts',(-67.9774483812669,-1.06381760593968,
124.284979670466));
#237895=CARTESIAN_POINT('Ctrl Pts',(-68.2558960050797,-6.05995923045808,
128.175495851683));
#237896=CARTESIAN_POINT('Ctrl Pts',(-68.5343436288926,-5.48729436765201,
134.481810325563));
#237897=CARTESIAN_POINT('Ctrl Pts',(-68.8127912527054,0.12792594979327,
137.408728171199));
#237898=CARTESIAN_POINT('Ctrl Pts',(-69.0912388765185,5.62558856890878,
134.266554876337));
#237899=CARTESIAN_POINT('Ctrl Pts',(-69.3696865003312,5.9536101184771,127.942794195258));
#237900=CARTESIAN_POINT('Ctrl Pts',(-69.6481341241442,0.810554819188534,
124.248673260987));
#237901=CARTESIAN_POINT('Ctrl Pts',(-69.9265817479571,-5.07736076112986,
126.578908744281));
#237902=CARTESIAN_POINT('Ctrl Pts',(-70.2050293717699,-6.29942984483285,
132.792128074323));
#237903=CARTESIAN_POINT('Ctrl Pts',(-70.4834769955829,-1.73263064539088,
137.178686219444));
#237904=CARTESIAN_POINT('Ctrl Pts',(-70.7619246193956,4.42637147345276,
135.707550539556));
#237905=CARTESIAN_POINT('Ctrl Pts',(-71.0403722432087,6.51775444846118,
129.730622855503));
#237906=CARTESIAN_POINT('Ctrl Pts',(-71.3188198670216,2.6196394953401,124.740407719779));
#237907=CARTESIAN_POINT('Ctrl Pts',(-71.5972674908343,-3.68579617749442,
125.322669056552));
#237908=CARTESIAN_POINT('Ctrl Pts',(-71.8757151146474,-6.6041652243652,
130.942337142376));
#237909=CARTESIAN_POINT('Ctrl Pts',(-72.1541627384602,-3.45362906145158,
136.435211542427));
#237910=CARTESIAN_POINT('Ctrl Pts',(-72.4326103622731,2.87062348977667,
136.753609024891));
#237911=CARTESIAN_POINT('Ctrl Pts',(-72.711057986086,6.55691329165398,131.604937857965));
#237912=CARTESIAN_POINT('Ctrl Pts',(-72.9895056098989,4.21772010152317,
125.720575317484));
#237913=CARTESIAN_POINT('Ctrl Pts',(-73.2679532337117,-1.99735181482566,
124.50796311106));
#237914=CARTESIAN_POINT('Ctrl Pts',(-73.5464008575247,-6.37695498941029,
129.081432616995));
#237915=CARTESIAN_POINT('Ctrl Pts',(-73.8248484813376,-4.89644806029751,
135.238188785743));
#237916=CARTESIAN_POINT('Ctrl Pts',(-74.1032961051504,1.08365543144292,
137.320473472483));
#237917=CARTESIAN_POINT('Ctrl Pts',(-74.3817437289633,6.06793252119795,
133.414768775364));
#237918=CARTESIAN_POINT('Ctrl Pts',(-74.6601913527762,5.47607605895596,
127.110226506756));
#237919=CARTESIAN_POINT('Ctrl Pts',(-74.9386389765891,-0.148026780279403,
124.200413017498));
#237920=CARTESIAN_POINT('Ctrl Pts',(-75.217086600402,-5.63610023994771,
127.359304751927));
#237921=CARTESIAN_POINT('Ctrl Pts',(-75.4955342242149,-5.94487291790794,
133.684034526541));
#237922=CARTESIAN_POINT('Ctrl Pts',(-75.7739818480278,-0.790597807498519,
137.362484658699));
#237923=CARTESIAN_POINT('Ctrl Pts',(-76.0524294718406,5.09019806515201,
135.014339179226));
#237924=CARTESIAN_POINT('Ctrl Pts',(-76.3308770956536,6.29335058592772,
128.797429070474));
#237925=CARTESIAN_POINT('Ctrl Pts',(-76.6093247194664,1.71322136550425,
124.424791009442));
#237926=CARTESIAN_POINT('Ctrl Pts',(-76.8877723432794,-4.44127459430165,
125.914665758975));
#237927=CARTESIAN_POINT('Ctrl Pts',(-77.1662199670922,-6.51445617026952,
131.89793120868));
#237928=CARTESIAN_POINT('Ctrl Pts',(-77.4446675909052,-2.60117077463652,
136.876258709042));
#237929=CARTESIAN_POINT('Ctrl Pts',(-77.7231152147181,3.7024634886308,136.274808492052));
#237930=CARTESIAN_POINT('Ctrl Pts',(-78.0015628385308,6.60371468124315,
130.646283924643));
#237931=CARTESIAN_POINT('Ctrl Pts',(-78.2800104623438,3.43647469119047,
125.163024115555));
#237932=CARTESIAN_POINT('Ctrl Pts',(-78.5584580861567,-2.88871765894464,
124.863876957204));
#237933=CARTESIAN_POINT('Ctrl Pts',(-78.8369057099696,-6.55931960221255,
130.023744073965));
#237934=CARTESIAN_POINT('Ctrl Pts',(-79.1153533337825,-4.20222727162433,
135.900959659057));
#237935=CARTESIAN_POINT('Ctrl Pts',(-79.3938009575953,2.01650663137172,
137.094649707722));
#237936=CARTESIAN_POINT('Ctrl Pts',(-79.6722485814083,6.38216945196263,
132.507871380239));
#237937=CARTESIAN_POINT('Ctrl Pts',(-79.9506962052212,4.88293033251105,
126.355649882987));
#237938=CARTESIAN_POINT('Ctrl Pts',(-80.229143829034,-1.10348321810992,
124.29157621921));
#237939=CARTESIAN_POINT('Ctrl Pts',(-80.507591452847,-6.07584959944043,
128.212433250316));
#237940=CARTESIAN_POINT('Ctrl Pts',(-80.7860390766598,-5.46480702063872,
134.515144909234));
#237941=CARTESIAN_POINT('Ctrl Pts',(-81.0644867004727,0.168126239464741,
137.407827085998));
#237942=CARTESIAN_POINT('Ctrl Pts',(-81.3429343242857,5.64655969892388,
134.232246175545));
#237943=CARTESIAN_POINT('Ctrl Pts',(-81.6213819480984,5.93608064484842,
127.906605898828));
#237944=CARTESIAN_POINT('Ctrl Pts',(-81.8998295719115,0.770633471818905,
124.243860645443));
#237945=CARTESIAN_POINT('Ctrl Pts',(-82.1782771957242,-5.10298821427442,
126.609894368197));
#237946=CARTESIAN_POINT('Ctrl Pts',(-82.4567248195372,-6.28721302628274,
132.830437663053));
#237947=CARTESIAN_POINT('Ctrl Pts',(-82.7351724433501,-1.69379621456928,
137.189115132473));
#237948=CARTESIAN_POINT('Ctrl Pts',(-83.0136200671628,4.45613657178832,
135.680515115291));
#237949=CARTESIAN_POINT('Ctrl Pts',(-83.2920676909759,6.51109754304618,
129.690967328089));
#237950=CARTESIAN_POINT('Ctrl Pts',(-83.5705153147887,2.58267795704331,
124.724573581631));
#237951=CARTESIAN_POINT('Ctrl Pts',(-83.8489629386017,-3.71909650065006,
125.345207107088));
#237952=CARTESIAN_POINT('Ctrl Pts',(-84.1274105624144,-6.60320296221082,
130.982536014198));
#237953=CARTESIAN_POINT('Ctrl Pts',(-84.4058581862275,-3.41928848589759,
136.456130436155));
#237954=CARTESIAN_POINT('Ctrl Pts',(-84.6843058100402,2.90678506742617,
136.736024499134));
#237955=CARTESIAN_POINT('Ctrl Pts',(-84.9627534338533,6.56166514813073,
131.565009232842));
#237956=CARTESIAN_POINT('Ctrl Pts',(-85.241201057666,4.1866955128661,125.694995048862));
#237957=CARTESIAN_POINT('Ctrl Pts',(-85.519648681479,-2.03564276727566,
124.520238216135));
#237958=CARTESIAN_POINT('Ctrl Pts',(-85.7980963052919,-6.38732479096924,
129.120282873878));
#237959=CARTESIAN_POINT('Ctrl Pts',(-86.0765439291047,-4.8693673699251,
135.267912706297));
#237960=CARTESIAN_POINT('Ctrl Pts',(-86.3549915529177,1.12330078225909,
137.313756225814));
#237961=CARTESIAN_POINT('Ctrl Pts',(-86.6334391767305,6.08371039184151,
133.377783183006));
#237962=CARTESIAN_POINT('Ctrl Pts',(-86.9118868005434,5.45348735709659,
127.076960521238));
#237963=CARTESIAN_POINT('Ctrl Pts',(-87.1903344243564,-0.188224141151809,
124.201436454379));
#237964=CARTESIAN_POINT('Ctrl Pts',(-87.4687820481692,-5.65696684894189,
127.39367712271));
#237965=CARTESIAN_POINT('Ctrl Pts',(-87.7472296719821,-5.92723338074904,
133.720169301662));
#237966=CARTESIAN_POINT('Ctrl Pts',(-88.0256772957949,-0.750661997095914,
137.367175745102));
#237967=CARTESIAN_POINT('Ctrl Pts',(-88.3041249196079,5.11573109001074,
134.983275697681));
#237968=CARTESIAN_POINT('Ctrl Pts',(-88.5825725434208,6.28101722275544,
128.759156842984));
#237969=CARTESIAN_POINT('Ctrl Pts',(-88.8610201672337,1.67435537253749,
124.414480343369));
#237970=CARTESIAN_POINT('Ctrl Pts',(-89.1394677910466,-4.47095726823472,
125.941791652735));
#237971=CARTESIAN_POINT('Ctrl Pts',(-89.4179154148595,-6.50767859790483,
131.93756629108));
#237972=CARTESIAN_POINT('Ctrl Pts',(-89.6963630386723,-2.56416121387375,
136.891980275641));
#237973=CARTESIAN_POINT('Ctrl Pts',(-89.9748106624853,3.73569505946763,
136.252169191183));
#237974=CARTESIAN_POINT('Ctrl Pts',(-90.253258286298,6.60263007200808,130.606088167816));
#237975=CARTESIAN_POINT('Ctrl Pts',(-90.5317059101111,3.40207060478355,
125.142209839621));
#237976=CARTESIAN_POINT('Ctrl Pts',(-90.8101535339238,-2.9248255478482,
124.881571464914));
#237977=CARTESIAN_POINT('Ctrl Pts',(-91.0886011577368,-6.56394990767886,
130.063686977158));
#237978=CARTESIAN_POINT('Ctrl Pts',(-91.3670487815497,-4.17112496913288,
135.926445381018));
#237979=CARTESIAN_POINT('Ctrl Pts',(-91.6454964053626,2.05476004526333,
137.082258115016));
#237980=CARTESIAN_POINT('Ctrl Pts',(-91.9239440291755,6.39242095867105,
132.468989741201));
#237981=CARTESIAN_POINT('Ctrl Pts',(-92.2023916529884,4.85575929818535,
126.326008524418));
#237982=CARTESIAN_POINT('Ctrl Pts',(-92.4808392768012,-1.14310794030347,
124.298414101576));
#237983=CARTESIAN_POINT('Ctrl Pts',(-92.7592869006141,-6.09151482558059,
128.249466693771));
#237984=CARTESIAN_POINT('Ctrl Pts',(-93.0377345244271,-5.44211717319261,
134.548341988427));
#237985=CARTESIAN_POINT('Ctrl Pts',(-93.3161821482399,0.208320299155509,
137.406681306919));
#237986=CARTESIAN_POINT('Ctrl Pts',(-93.5946297720528,5.6673215935918,134.197810453193));
#237987=CARTESIAN_POINT('Ctrl Pts',(-93.8730773958657,5.91833120756931,
127.870524979765));
#237988=CARTESIAN_POINT('Ctrl Pts',(-94.1515250196785,0.730683568342929,
124.239291131637));
#237989=CARTESIAN_POINT('Ctrl Pts',(-94.4299726434915,-5.12842657431339,
126.641035419604));
#237990=CARTESIAN_POINT('Ctrl Pts',(-94.7084202673044,-6.27476323274215,
132.868672174754));
#237991=CARTESIAN_POINT('Ctrl Pts',(-94.9868678911172,-1.6548990195065,
137.199307456074));
#237992=CARTESIAN_POINT('Ctrl Pts',(-95.2653155149302,4.48573654634406,
135.653299003326));
#237993=CARTESIAN_POINT('Ctrl Pts',(-95.543763138743,6.50419936651746,129.651353057874));
#237994=CARTESIAN_POINT('Ctrl Pts',(-95.822210762556,2.54562071666526,124.708964732227));
#237995=CARTESIAN_POINT('Ctrl Pts',(-96.1006583863688,-3.75225901131679,
125.367947448562));
#237996=CARTESIAN_POINT('Ctrl Pts',(-96.3791060101818,-6.60199601594203,
131.022728283664));
#237997=CARTESIAN_POINT('Ctrl Pts',(-96.6575536339946,-3.38482120735248,
136.476839901474));
#237998=CARTESIAN_POINT('Ctrl Pts',(-96.9360012578075,2.94283893308538,
136.718220173391));
#237999=CARTESIAN_POINT('Ctrl Pts',(-97.2144488816204,6.5661738596919,131.525052421605));
#238000=CARTESIAN_POINT('Ctrl Pts',(-97.4928965054334,4.15551578466796,
125.669604109659));
#238001=CARTESIAN_POINT('Ctrl Pts',(-97.771344129246,-2.07385828823457,
124.532746181678));
#238002=CARTESIAN_POINT('Ctrl Pts',(-98.0497917530593,-6.39745790785863,
129.15919553488));
#238003=CARTESIAN_POINT('Ctrl Pts',(-98.3282393768718,-4.84210624335443,
135.297471228287));
#238004=CARTESIAN_POINT('Ctrl Pts',(-98.606687000685,1.16290450875192,137.306797771098));
#238005=CARTESIAN_POINT('Ctrl Pts',(-98.8851346244975,6.09926282835875,
133.340702231527));
#238006=CARTESIAN_POINT('Ctrl Pts',(-99.1635822483109,5.43069657425812,
127.043832655902));
#238007=CARTESIAN_POINT('Ctrl Pts',(-99.4420298721233,-0.228414527308866,
124.202704565042));
#238008=CARTESIAN_POINT('Ctrl Pts',(-99.7204774959365,-5.67762383694899,
127.428175877623));
#238009=CARTESIAN_POINT('Ctrl Pts',(-99.9989251197493,-5.90937420777732,
133.756196030418));
#238010=CARTESIAN_POINT('Ctrl Pts',(-100.277372743562,-0.710698370637635,
137.371623643978));
#238011=CARTESIAN_POINT('Ctrl Pts',(-100.555820367375,5.14107454957247,
134.9520573649));
#238012=CARTESIAN_POINT('Ctrl Pts',(-100.834267991188,6.26845111417983,
128.720960401273));
#238013=CARTESIAN_POINT('Ctrl Pts',(-101.112715615001,1.63542733571746,
124.404406456659));
#238014=CARTESIAN_POINT('Ctrl Pts',(-101.391163238814,-4.50047426920288,
125.969097730777));
#238015=CARTESIAN_POINT('Ctrl Pts',(-101.669610862627,-6.50065988111587,
131.977159382129));
#238016=CARTESIAN_POINT('Ctrl Pts',(-101.94805848644,-2.52705663717401,
136.907476263252));
#238017=CARTESIAN_POINT('Ctrl Pts',(-102.226506110253,3.76878820275105,
136.229328019765));
#238018=CARTESIAN_POINT('Ctrl Pts',(-102.504953734065,6.60130079988703,
130.565899758046));
#238019=CARTESIAN_POINT('Ctrl Pts',(-102.783401357878,3.36754045339959,
125.121605376767));
#238020=CARTESIAN_POINT('Ctrl Pts',(-103.061848981691,-2.96082505626518,
124.899485443752));
#238021=CARTESIAN_POINT('Ctrl Pts',(-103.340296605504,-6.56833698356739,
130.103657326284));
#238022=CARTESIAN_POINT('Ctrl Pts',(-103.618744229317,-4.13986810407194,
135.951741302244));
#238023=CARTESIAN_POINT('Ctrl Pts',(-103.89719185313,2.0929373192654,137.06963389251));
#238024=CARTESIAN_POINT('Ctrl Pts',(-104.175639476943,6.40243559186997,
132.430046418718));
#238025=CARTESIAN_POINT('Ctrl Pts',(-104.454087100755,4.82840833191319,
126.296533112833));
#238026=CARTESIAN_POINT('Ctrl Pts',(-104.732534724569,-1.18269030421136,
124.305493064181));
#238027=CARTESIAN_POINT('Ctrl Pts',(-105.010982348381,-6.10695432839948,
128.286594809759));
#238028=CARTESIAN_POINT('Ctrl Pts',(-105.289429972194,-5.41922566609253,
134.581400333014));
#238029=CARTESIAN_POINT('Ctrl Pts',(-105.567877596007,0.248506639461218,
137.40529087642));
#238030=CARTESIAN_POINT('Ctrl Pts',(-105.84632521982,5.68787348357469,134.163248985309));
#238031=CARTESIAN_POINT('Ctrl Pts',(-106.124772843633,5.90036246435008,
127.834552775061));
#238032=CARTESIAN_POINT('Ctrl Pts',(-106.403220467446,0.690706589119241,
124.234964888896));
#238033=CARTESIAN_POINT('Ctrl Pts',(-106.681668091259,-5.1536748986197,
126.672330744555));
#238034=CARTESIAN_POINT('Ctrl Pts',(-106.960115715072,-6.26208092554253,
132.906830192629));
#238035=CARTESIAN_POINT('Ctrl Pts',(-107.238563338885,-1.61594050155245,
137.209262812568));
#238036=CARTESIAN_POINT('Ctrl Pts',(-107.517010962697,4.51517030028232,
135.625903212168));
#238037=CARTESIAN_POINT('Ctrl Pts',(-107.79545858651,6.49706017448951,129.611781512777));
#238038=CARTESIAN_POINT('Ctrl Pts',(-108.073906210323,2.50846914737518,
124.69358174996));
#238039=CARTESIAN_POINT('Ctrl Pts',(-108.352353834136,-3.78528248064593,
125.390889238328));
#238040=CARTESIAN_POINT('Ctrl Pts',(-108.630801457949,-6.60054443028347,
131.062912461436));
#238041=CARTESIAN_POINT('Ctrl Pts',(-108.909249081762,-3.35022850301195,
136.497339170987));
#238042=CARTESIAN_POINT('Ctrl Pts',(-109.187696705575,2.97878375076591,
136.700196707408));
#238043=CARTESIAN_POINT('Ctrl Pts',(-109.466144329388,6.57043925926657,
131.485068904869));
#238044=CARTESIAN_POINT('Ctrl Pts',(-109.7445919532,4.12418207230337,125.644403440746));
#238045=CARTESIAN_POINT('Ctrl Pts',(-110.023039577014,-2.11199696161116,
124.5454865442));
#238046=CARTESIAN_POINT('Ctrl Pts',(-110.301487200826,-6.40735396459295,
129.198169158078));
#238047=CARTESIAN_POINT('Ctrl Pts',(-110.579934824639,-4.81466569075636,
135.326863256411));
#238048=CARTESIAN_POINT('Ctrl Pts',(-110.858382448452,1.20246514338981,
137.299598366182));
#238049=CARTESIAN_POINT('Ctrl Pts',(-111.136830072265,6.11458925444912,
133.303527294979));
#238050=CARTESIAN_POINT('Ctrl Pts',(-111.415277696078,5.407704554961,127.010844138312));
#238051=CARTESIAN_POINT('Ctrl Pts',(-111.693725319891,-0.268596449482207,
124.204217302498));
#238052=CARTESIAN_POINT('Ctrl Pts',(-111.972172943703,-5.69807043851701,
127.462799738304));
#238053=CARTESIAN_POINT('Ctrl Pts',(-112.250620567517,-5.89129606077132,
133.792113377828));
#238054=CARTESIAN_POINT('Ctrl Pts',(-112.529068191329,-0.670708408989202,
137.375828190507));
#238055=CARTESIAN_POINT('Ctrl Pts',(-112.807515815142,5.16622750472631,
134.920685337692));
#238056=CARTESIAN_POINT('Ctrl Pts',(-113.085963438955,6.25565272584325,
128.682841160722));
#238057=CARTESIAN_POINT('Ctrl Pts',(-113.364411062768,1.5964386975353,124.394569722605));
#238058=CARTESIAN_POINT('Ctrl Pts',(-113.642858686581,-4.52982450344111,
125.996582981263));
#238059=CARTESIAN_POINT('Ctrl Pts',(-113.921306310394,-6.49340027998504,
132.016709014688));
#238060=CARTESIAN_POINT('Ctrl Pts',(-114.199753934207,-2.48985841946147,
136.922746097669));
#238061=CARTESIAN_POINT('Ctrl Pts',(-114.47820155802,3.80174169220082,136.206285824184));
#238062=CARTESIAN_POINT('Ctrl Pts',(-114.756649181833,6.59972691413776,
130.525720184532));
#238063=CARTESIAN_POINT('Ctrl Pts',(-115.035096805645,3.3328855165654,125.101211490497));
#238064=CARTESIAN_POINT('Ctrl Pts',(-115.313544429458,-2.99671485022117,
124.917618229914));
#238065=CARTESIAN_POINT('Ctrl Pts',(-115.591992053271,-6.57248066731354,
130.143653640229));
#238066=CARTESIAN_POINT('Ctrl Pts',(-115.870439677084,-4.10845783467579,
135.976846485386));
#238067=CARTESIAN_POINT('Ctrl Pts',(-116.148887300897,2.13103703870585,
137.056777507999));
#238068=CARTESIAN_POINT('Ctrl Pts',(-116.42733492471,6.41221298046361,132.391042855849));
#238069=CARTESIAN_POINT('Ctrl Pts',(-116.705782548523,4.8008784471946,126.267224740454));
#238070=CARTESIAN_POINT('Ctrl Pts',(-116.984230172336,-1.22222884309565,
124.312812844714));
#238071=CARTESIAN_POINT('Ctrl Pts',(-117.262677796149,-6.12216753577917,
128.323816222486));
#238072=CARTESIAN_POINT('Ctrl Pts',(-117.541125419961,-5.39613334759327,
134.614318718005));
#238073=CARTESIAN_POINT('Ctrl Pts',(-117.819573043774,0.288683771261777,
137.403655846021));
#238074=CARTESIAN_POINT('Ctrl Pts',(-118.098020667587,5.70821460731317,
134.128563052582));
#238075=CARTESIAN_POINT('Ctrl Pts',(-118.3764682914,5.88217508103065,127.79869061768));
#238076=CARTESIAN_POINT('Ctrl Pts',(-118.654915915213,0.650704015508265,
124.230882077529));
#238077=CARTESIAN_POINT('Ctrl Pts',(-118.933363539026,-5.17873225160735,
126.703779183394));
#238078=CARTESIAN_POINT('Ctrl Pts',(-119.211811162839,-6.24916657463125,
132.944910302722));
#238079=CARTESIAN_POINT('Ctrl Pts',(-119.490258786652,-1.57692210432836,
137.218980833058));
#238080=CARTESIAN_POINT('Ctrl Pts',(-119.768706410464,4.54443674292479,
135.598328756974));
#238081=CARTESIAN_POINT('Ctrl Pts',(-120.047154034278,6.48968023150711,
129.572254159139));
#238082=CARTESIAN_POINT('Ctrl Pts',(-120.32560165809,2.47122462583917,124.67842520485));
#238083=CARTESIAN_POINT('Ctrl Pts',(-120.604049281903,-3.81816568494053,
125.414031626265));
#238084=CARTESIAN_POINT('Ctrl Pts',(-120.882496905716,-6.59884825902321,
131.103087058474));
#238085=CARTESIAN_POINT('Ctrl Pts',(-121.160944529529,-3.31551165472302,
136.517627485086));
#238086=CARTESIAN_POINT('Ctrl Pts',(-121.439392153342,3.0146181885189,136.68195476905));
#238087=CARTESIAN_POINT('Ctrl Pts',(-121.717839777155,6.57446118879764,
131.445060164237));
#238088=CARTESIAN_POINT('Ctrl Pts',(-121.996287400968,4.0926955368563,125.619393975946));
#238089=CARTESIAN_POINT('Ctrl Pts',(-122.274735024781,-2.15005737416446,
124.5584588316));
#238090=CARTESIAN_POINT('Ctrl Pts',(-122.553182648593,-6.41701259446945,
129.237202299292));
#238091=CARTESIAN_POINT('Ctrl Pts',(-122.831630272406,-4.7870467289504,
135.356087701536));
#238092=CARTESIAN_POINT('Ctrl Pts',(-123.110077896219,1.24198122024032,
137.292158277842));
#238093=CARTESIAN_POINT('Ctrl Pts',(-123.388525520032,6.1296891021858,133.266259750888));
#238094=CARTESIAN_POINT('Ctrl Pts',(-123.666973143845,5.38451215118288,
126.97799619087));
#238095=CARTESIAN_POINT('Ctrl Pts',(-123.945420767658,-0.30876841871475,
124.20597461069));
#238096=CARTESIAN_POINT('Ctrl Pts',(-124.223868391471,-5.71830589598935,
127.497547421752));
#238097=CARTESIAN_POINT('Ctrl Pts',(-124.502316015284,-5.87299960962311,
133.827920012961));
#238098=CARTESIAN_POINT('Ctrl Pts',(-124.780763639097,-0.630693593994696,
137.379789228888));
#238099=CARTESIAN_POINT('Ctrl Pts',(-125.059211262909,5.19118902341993,
134.889160778557));
#238100=CARTESIAN_POINT('Ctrl Pts',(-125.337658886723,6.24262253199412,
128.644800533857));
#238101=CARTESIAN_POINT('Ctrl Pts',(-125.616106510535,1.55739090273089,
124.384970505708));
#238102=CARTESIAN_POINT('Ctrl Pts',(-125.894554134348,-4.55900688336737,
126.024246385717));
#238103=CARTESIAN_POINT('Ctrl Pts',(-126.173001758161,-6.48590006351826,
132.056213723232));
#238104=CARTESIAN_POINT('Ctrl Pts',(-126.451449381974,-2.45256793912933,
136.937789213063));
#238105=CARTESIAN_POINT('Ctrl Pts',(-126.729897005787,3.83455430671493,
136.183043458277));
#238106=CARTESIAN_POINT('Ctrl Pts',(-127.0083446296,6.5979084730801,130.485550936142));
#238107=CARTESIAN_POINT('Ctrl Pts',(-127.286792253413,3.29810707843306,
125.081028936517));
#238108=CARTESIAN_POINT('Ctrl Pts',(-127.565239877225,-3.03249359980603,
124.935969151478));
#238109=CARTESIAN_POINT('Ctrl Pts',(-127.843687501038,-6.57638080537151,
130.183674436914));
#238110=CARTESIAN_POINT('Ctrl Pts',(-128.122135124851,-4.07689532486387,
136.001760000162));
#238111=CARTESIAN_POINT('Ctrl Pts',(-128.400582748664,2.1690577917847,137.043689437881));
#238112=CARTESIAN_POINT('Ctrl Pts',(-128.679030372477,6.42175276214748,
132.351980497887));
#238113=CARTESIAN_POINT('Ctrl Pts',(-128.95747799629,4.77317066415926,126.238084493312));
#238114=CARTESIAN_POINT('Ctrl Pts',(-129.235925620103,-1.26172209184052,
124.320373171937));
#238115=CARTESIAN_POINT('Ctrl Pts',(-129.514373243916,-6.13715388399014,
128.361129552696));
#238116=CARTESIAN_POINT('Ctrl Pts',(-129.792820867728,-5.37284107338758,
134.647095923599));
#238117=CARTESIAN_POINT('Ctrl Pts',(-130.071268491542,0.328850205779251,
137.401776276312));
#238118=CARTESIAN_POINT('Ctrl Pts',(-130.349716115354,5.72834421106097,
134.093753940311));
#238119=CARTESIAN_POINT('Ctrl Pts',(-130.628163739167,5.86376973154965,
127.762939836503));
#238120=CARTESIAN_POINT('Ctrl Pts',(-130.90661136298,0.610677329821333,
124.227042848828));
#238121=CARTESIAN_POINT('Ctrl Pts',(-131.185058986793,-5.20359770476699,
126.735379570785));
#238122=CARTESIAN_POINT('Ctrl Pts',(-131.463506610606,-6.23602065855449,
132.982911093959));
#238123=CARTESIAN_POINT('Ctrl Pts',(-131.741954234419,-1.53784527367628,
137.228461157434));
#238124=CARTESIAN_POINT('Ctrl Pts',(-132.020401858232,4.57353478979242,
135.57057665953));
#238125=CARTESIAN_POINT('Ctrl Pts',(-132.298849482045,6.48205981103755,
129.532772461657));
#238126=CARTESIAN_POINT('Ctrl Pts',(-132.577297105858,2.43388853216508,
124.66349565853));
#238127=CARTESIAN_POINT('Ctrl Pts',(-132.85574472967,-3.85090740570176,
125.437373754826));
#238128=CARTESIAN_POINT('Ctrl Pts',(-133.134192353483,-6.59690756501448,
131.143250586095));
#238129=CARTESIAN_POINT('Ctrl Pts',(-133.412639977296,-3.28067194892964,
136.53770409198));
#238130=CARTESIAN_POINT('Ctrl Pts',(-133.691087601109,3.0503409184865,136.663495034279));
#238131=CARTESIAN_POINT('Ctrl Pts',(-133.969535224922,6.5782394992522,131.405027682246));
#238132=CARTESIAN_POINT('Ctrl Pts',(-134.247982848735,4.06105734507014,
125.59457664199));
#238133=CARTESIAN_POINT('Ctrl Pts',(-134.526430472548,-2.18803811555026,
124.57166256319));
#238134=CARTESIAN_POINT('Ctrl Pts',(-134.804878096361,-6.42643343958478,
129.276293512134));
#238135=CARTESIAN_POINT('Ctrl Pts',(-135.083325720174,-4.75925038136761,
135.385143480741));
#238136=CARTESIAN_POINT('Ctrl Pts',(-135.361773343986,1.28145127501926,
137.284477781773));
#238137=CARTESIAN_POINT('Ctrl Pts',(-135.640220967799,6.14456181203885,
133.228900980221));
#238138=CARTESIAN_POINT('Ctrl Pts',(-135.918668591612,5.36112022232688,
126.945290030769));
#238139=CARTESIAN_POINT('Ctrl Pts',(-136.197116215425,-0.348928946420584,
124.207976424505));
#238140=CARTESIAN_POINT('Ctrl Pts',(-136.475563839238,-5.73832945953392,
127.53241764038));
#238141=CARTESIAN_POINT('Ctrl Pts',(-136.754011463051,-5.85448553231475,
133.863614608987));
#238142=CARTESIAN_POINT('Ctrl Pts',(-137.032459086864,-0.590655408416443,
137.383506612345));
#238143=CARTESIAN_POINT('Ctrl Pts',(-137.310906710677,5.21595818069537,
134.857484855651));
#238144=CARTESIAN_POINT('Ctrl Pts',(-137.58935433449,6.22936101547165,128.606839930282));
#238145=CARTESIAN_POINT('Ctrl Pts',(-137.867801958302,1.51828539823306,
124.375609161675));
#238146=CARTESIAN_POINT('Ctrl Pts',(-138.146249582115,-4.58802032761614,
126.052086919061));
#238147=CARTESIAN_POINT('Ctrl Pts',(-138.424697205928,-6.47815950964009,
132.095672043897));
#238148=CARTESIAN_POINT('Ctrl Pts',(-138.703144829741,-2.41518657799051,
136.952605052004));
#238149=CARTESIAN_POINT('Ctrl Pts',(-138.981592453554,3.86722483040823,
136.159601783301));
#238150=CARTESIAN_POINT('Ctrl Pts',(-139.260040077367,6.59584554409815,
130.445393501362));
#238151=CARTESIAN_POINT('Ctrl Pts',(-139.53848770118,3.26320642772972,125.061058462695));
#238152=CARTESIAN_POINT('Ctrl Pts',(-139.816935324993,-3.06815997922566,
124.954537528447));
#238153=CARTESIAN_POINT('Ctrl Pts',(-140.095382948806,-6.58003725322031,
130.223718233352));
#238154=CARTESIAN_POINT('Ctrl Pts',(-140.373830572619,-4.04518174419624,
136.026480923393));
#238155=CARTESIAN_POINT('Ctrl Pts',(-140.652278196431,2.20699816962987,
137.030370167137));
#238156=CARTESIAN_POINT('Ctrl Pts',(-140.930725820244,6.43105458342049,
132.312860792301));
#238157=CARTESIAN_POINT('Ctrl Pts',(-141.209173444057,4.74528600953044,
126.209113451214));
#238158=CARTESIAN_POINT('Ctrl Pts',(-141.48762106787,-1.30116858700904,
124.328173765698));
#238159=CARTESIAN_POINT('Ctrl Pts',(-141.766068691683,-6.15191281770628,
128.398533417733));
#238160=CARTESIAN_POINT('Ctrl Pts',(-142.044516315496,-5.34934970658085,
134.679730735221));
#238161=CARTESIAN_POINT('Ctrl Pts',(-142.322963939309,0.369004454631186,
137.399652236939));
#238162=CARTESIAN_POINT('Ctrl Pts',(-142.601411563122,5.74826154890666,
134.058822938361));
#238163=CARTESIAN_POINT('Ctrl Pts',(-142.879859186934,5.84514709792562,
127.727301756295));
#238164=CARTESIAN_POINT('Ctrl Pts',(-143.158306810748,0.570628015260733,
124.223447345055));
#238165=CARTESIAN_POINT('Ctrl Pts',(-143.43675443456,-5.22827033670001,
126.767130735766));
#238166=CARTESIAN_POINT('Ctrl Pts',(-143.715202058373,-6.22264366443886,
133.020831158207));
#238167=CARTESIAN_POINT('Ctrl Pts',(-143.993649682186,-1.49871145760156,
137.237703434405));
#238168=CARTESIAN_POINT('Ctrl Pts',(-144.272097305999,4.60246336264661,
135.542647948195));
#238169=CARTESIAN_POINT('Ctrl Pts',(-144.550544929812,6.47419919545755,
129.493337883343));
#238170=CARTESIAN_POINT('Ctrl Pts',(-144.828992553625,2.39646224985712,
124.648793664219));
#238171=CARTESIAN_POINT('Ctrl Pts',(-145.107440177438,-3.8835064296727,
125.460914759058));
#238172=CARTESIAN_POINT('Ctrl Pts',(-145.38588780125,-6.59472242016944,
131.183401556022));
#238173=CARTESIAN_POINT('Ctrl Pts',(-145.664335425064,-3.24571067663155,
136.557568247724));
#238174=CARTESIAN_POINT('Ctrl Pts',(-145.942783048876,3.08595061694992,
136.644818187128));
#238175=CARTESIAN_POINT('Ctrl Pts',(-146.221230672689,6.58177405062243,
131.364972942318));
#238176=CARTESIAN_POINT('Ctrl Pts',(-146.499678296502,4.02926866931097,
125.569952358496));
#238177=CARTESIAN_POINT('Ctrl Pts',(-146.778125920315,-2.22593777837984,
124.585097249699));
#238178=CARTESIAN_POINT('Ctrl Pts',(-147.056573544128,-6.43561615084533,
129.315441348065));
#238179=CARTESIAN_POINT('Ctrl Pts',(-147.335021167941,-4.73127767801157,
135.414029517352));
#238180=CARTESIAN_POINT('Ctrl Pts',(-147.613468791753,1.32087384515067,
137.276557162581));
#238181=CARTESIAN_POINT('Ctrl Pts',(-147.891916415567,6.15920683289404,
133.191452367319));
#238182=CARTESIAN_POINT('Ctrl Pts',(-148.170364039379,5.33752963518947,
126.91272686995));
#238183=CARTESIAN_POINT('Ctrl Pts',(-148.448811663193,-0.389076544435395,
124.210222669761));
#238184=CARTESIAN_POINT('Ctrl Pts',(-148.727259287005,-5.75814038716998,
127.567409102056));
#238185=CARTESIAN_POINT('Ctrl Pts',(-149.005706910818,-5.83575451489182,
133.899195843233));
#238186=CARTESIAN_POINT('Ctrl Pts',(-149.284154534631,-0.550595335885521,
137.386980203127));
#238187=CARTESIAN_POINT('Ctrl Pts',(-149.562602158444,5.24053405872261,
134.825658742734));
#238188=CARTESIAN_POINT('Ctrl Pts',(-149.841049782257,6.21586866768539,
128.568960756646));
#238189=CARTESIAN_POINT('Ctrl Pts',(-150.119497406069,1.47912363311174,
124.366486037389));
#238190=CARTESIAN_POINT('Ctrl Pts',(-150.397945029883,-4.61686376108527,
126.080103549656));
#238191=CARTESIAN_POINT('Ctrl Pts',(-150.676392653695,-6.4701789051783,
132.135082514543));
#238192=CARTESIAN_POINT('Ctrl Pts',(-150.954840277509,-2.37771572122463,
136.967193065487));
#238193=CARTESIAN_POINT('Ctrl Pts',(-151.233287901321,3.89975205266408,
136.135961667893));
#238194=CARTESIAN_POINT('Ctrl Pts',(-151.511735525134,6.59353820363339,
130.405249368239));
#238195=CARTESIAN_POINT('Ctrl Pts',(-151.790183148947,3.22818485771248,
125.041300809049));
#238196=CARTESIAN_POINT('Ctrl Pts',(-152.06863077276,-3.10371266684865,
124.97332267276));
#238197=CARTESIAN_POINT('Ctrl Pts',(-152.347078396573,-6.58344987536885,
130.263783545709));
#238198=CARTESIAN_POINT('Ctrl Pts',(-152.625526020386,-4.01331826783166,
136.051008339035));
#238199=CARTESIAN_POINT('Ctrl Pts',(-152.903973644199,2.24485676634579,
137.016820189321));
#238200=CARTESIAN_POINT('Ctrl Pts',(-153.182421268012,6.44011809960154,
132.273685188686));
#238201=CARTESIAN_POINT('Ctrl Pts',(-153.460868891824,4.71722551658265,
126.180312687687));
#238202=CARTESIAN_POINT('Ctrl Pts',(-153.739316515637,-1.34056686689732,
124.336214336947));
#238203=CARTESIAN_POINT('Ctrl Pts',(-154.01776413945,-6.16644379003131,
128.436026431582));
#238204=CARTESIAN_POINT('Ctrl Pts',(-154.296211763263,-5.32566011765276,
134.712221943579));
#238205=CARTESIAN_POINT('Ctrl Pts',(-154.574659387076,0.409145029887599,
137.397283806609));
#238206=CARTESIAN_POINT('Ctrl Pts',(-154.853107010889,5.7679658828075,134.023771341112));
#238207=CARTESIAN_POINT('Ctrl Pts',(-155.131554634702,5.82630787022557,
127.691777697632));
#238208=CARTESIAN_POINT('Ctrl Pts',(-155.410002258515,0.530557555869813,
124.220095699443));
#238209=CARTESIAN_POINT('Ctrl Pts',(-155.688449882327,-5.25274923315307,
126.799031501784));
#238210=CARTESIAN_POINT('Ctrl Pts',(-155.96689750614,-6.20903608797397,
133.058669090323));
#238211=CARTESIAN_POINT('Ctrl Pts',(-156.245345129953,-1.4595221062231,
137.246707321489));
#238212=CARTESIAN_POINT('Ctrl Pts',(-156.523792753766,4.63122138952822,
135.514543657883));
#238213=CARTESIAN_POINT('Ctrl Pts',(-156.802240377579,6.46609867604585,
129.453951885458));
#238214=CARTESIAN_POINT('Ctrl Pts',(-157.080688001392,2.35894716575843,
124.634319766706));
#238215=CARTESIAN_POINT('Ctrl Pts',(-157.359135625205,-3.9159615488849,
125.484653766641));
#238216=CARTESIAN_POINT('Ctrl Pts',(-157.637583249018,-6.59229290546042,
131.223538480449));
#238217=CARTESIAN_POINT('Ctrl Pts',(-157.916030872831,-3.21062913332988,
136.577219216243));
#238218=CARTESIAN_POINT('Ctrl Pts',(-158.194478496644,3.12144596437753,
136.625924919674));
#238219=CARTESIAN_POINT('Ctrl Pts',(-158.472926120456,6.58506471193526,
131.324897428694));
#238220=CARTESIAN_POINT('Ctrl Pts',(-158.751373744269,3.99733068751967,
125.545522037924));
#238221=CARTESIAN_POINT('Ctrl Pts',(-159.029821368082,-2.26375495826568,
124.598762393297));
#238222=CARTESIAN_POINT('Ctrl Pts',(-159.308268991895,-6.44456038798308,
129.354644356446));
#238223=CARTESIAN_POINT('Ctrl Pts',(-159.586716615708,-4.7031296554214,
135.442744740987));
#238224=CARTESIAN_POINT('Ctrl Pts',(-159.865164239521,1.36024746981527,
137.268396713766));
#238225=CARTESIAN_POINT('Ctrl Pts',(-160.143611863334,6.17362362207528,
133.153915299856));
#238226=CARTESIAN_POINT('Ctrl Pts',(-160.422059487147,5.31374126392856,
126.880307915048));
#238227=CARTESIAN_POINT('Ctrl Pts',(-160.70050711096,-0.429209725076344,
124.212713263223));
#238228=CARTESIAN_POINT('Ctrl Pts',(-160.978954734773,-5.77773794479658,
127.602520510164));
#238229=CARTESIAN_POINT('Ctrl Pts',(-161.257402358585,-5.81680725143943,
133.934662397221));
#238230=CARTESIAN_POINT('Ctrl Pts',(-161.535849982398,-0.51051486084124,
137.390209872519));
#238231=CARTESIAN_POINT('Ctrl Pts',(-161.814297606211,5.26491574683228,
134.793683619137));
#238232=CARTESIAN_POINT('Ctrl Pts',(-162.092745230024,6.20214598860049,
128.531164416574));
#238233=CARTESIAN_POINT('Ctrl Pts',(-162.371192853837,1.43990705852047,
124.357601470914));
#238234=CARTESIAN_POINT('Ctrl Pts',(-162.64964047765,-4.64553611496906,
126.108295239334));
#238235=CARTESIAN_POINT('Ctrl Pts',(-162.928088101462,-6.46195854585841,
132.1744436748));
#238236=CARTESIAN_POINT('Ctrl Pts',(-163.206535725276,-2.34015675732853,
136.981552712947));
#238237=CARTESIAN_POINT('Ctrl Pts',(-163.484983349088,3.93213476817268,
136.112123988049));
#238238=CARTESIAN_POINT('Ctrl Pts',(-163.763430972902,6.5909865371863,130.365120024332));
#238239=CARTESIAN_POINT('Ctrl Pts',(-164.041878596714,3.19304366611785,
125.021756707701));
#238240=CARTESIAN_POINT('Ctrl Pts',(-164.320326220527,-3.13915034525769,
124.99232388833));
#238241=CARTESIAN_POINT('Ctrl Pts',(-164.59877384434,-6.58661854536123,
130.303868889347));
#238242=CARTESIAN_POINT('Ctrl Pts',(-164.877221468153,-3.98130607648258,
136.075341338217));
#238243=CARTESIAN_POINT('Ctrl Pts',(-165.155669091966,2.28263217906914,
137.003040006531));
#238244=CARTESIAN_POINT('Ctrl Pts',(-165.434116715779,6.44894297483741,
132.23445513871));
#238245=CARTESIAN_POINT('Ctrl Pts',(-165.712564339591,4.6889902251094,126.151683269957));
#238246=CARTESIAN_POINT('Ctrl Pts',(-165.991011963405,-1.37991547158711,
124.344494587733));
#238247=CARTESIAN_POINT('Ctrl Pts',(-166.269459587217,-6.18074626251326,
128.473607204924));
#238248=CARTESIAN_POINT('Ctrl Pts',(-166.54790721103,-5.3017731844313,134.744568344699));
#238249=CARTESIAN_POINT('Ctrl Pts',(-166.826354834843,0.449270444124704,
137.394671073086));
#238250=CARTESIAN_POINT('Ctrl Pts',(-167.104802458656,5.78745648261092,
133.988600447415));
#238251=CARTESIAN_POINT('Ctrl Pts',(-167.383250082469,5.8072527465451,127.656368976875));
#238252=CARTESIAN_POINT('Ctrl Pts',(-167.661697706282,0.490467436472931,
124.216988036188));
#238253=CARTESIAN_POINT('Ctrl Pts',(-167.940145330095,-5.27703348705155,
126.831080686747));
#238254=CARTESIAN_POINT('Ctrl Pts',(-168.218592953908,-6.19519843339338,
133.096423488211));
#238255=CARTESIAN_POINT('Ctrl Pts',(-168.49704057772,-1.42027867171577,
137.255472485049));
#238256=CARTESIAN_POINT('Ctrl Pts',(-168.775488201534,4.65980780479824,
135.486264830004));
#238257=CARTESIAN_POINT('Ctrl Pts',(-169.053935825346,6.45775855296945,
129.414615927465));
#238258=CARTESIAN_POINT('Ctrl Pts',(-169.332383449159,2.32134467000579,
124.620074502325));
#238259=CARTESIAN_POINT('Ctrl Pts',(-169.610831072972,-3.94827156070164,
125.508589897919));
#238260=CARTESIAN_POINT('Ctrl Pts',(-169.889278696785,-6.58961911091297,
131.263659872085));
#238261=CARTESIAN_POINT('Ctrl Pts',(-170.167726320598,-3.17542861898582,
136.596656269364));
#238262=CARTESIAN_POINT('Ctrl Pts',(-170.446173944411,3.15682564547787,
136.606815932013));
#238263=CARTESIAN_POINT('Ctrl Pts',(-170.724621568223,6.58811136125304,
131.284802626386));
#238264=CARTESIAN_POINT('Ctrl Pts',(-171.003069192037,3.96524458316956,
125.521286585549));
#238265=CARTESIAN_POINT('Ctrl Pts',(-171.28151681585,-2.30148825387982,
124.612657487621));
#238266=CARTESIAN_POINT('Ctrl Pts',(-171.559964439662,-6.45326581956532,
129.393901084596));
#238267=CARTESIAN_POINT('Ctrl Pts',(-171.838412063475,-4.67480735663214,
135.471288087592));
#238268=CARTESIAN_POINT('Ctrl Pts',(-172.116859687288,1.39957069001038,
137.259996737715));
#238269=CARTESIAN_POINT('Ctrl Pts',(-172.395307311101,6.18781164536257,
133.116291168777));
#238270=CARTESIAN_POINT('Ctrl Pts',(-172.673754934914,5.289755990031,126.848034367363));
#238271=CARTESIAN_POINT('Ctrl Pts',(-172.952202558727,-0.469327001192524,
124.215448112602));
#238272=CARTESIAN_POINT('Ctrl Pts',(-173.23065018254,-5.79712140621875,
127.637750563632));
#238273=CARTESIAN_POINT('Ctrl Pts',(-173.509097806352,-5.79764444405506,
133.970012956726));
#238274=CARTESIAN_POINT('Ctrl Pts',(-173.787545430165,-0.470415468481743,
137.393195500846));
#238275=CARTESIAN_POINT('Ctrl Pts',(-174.065993053978,5.28910234155359,
134.76156066971));
#238276=CARTESIAN_POINT('Ctrl Pts',(-174.344440677791,6.18819348671444,
128.493452310623));
#238277=CARTESIAN_POINT('Ctrl Pts',(-174.622888301604,1.40063712764339,
124.34895579147));
#238278=CARTESIAN_POINT('Ctrl Pts',(-174.901335925417,-4.67403632680454,
126.13666094344));
#238279=CARTESIAN_POINT('Ctrl Pts',(-175.17978354923,-6.45349873628761,
132.213754066126));
#238280=CARTESIAN_POINT('Ctrl Pts',(-175.458231173043,-2.30251107806296,
136.995683462282));
#238281=CARTESIAN_POINT('Ctrl Pts',(-175.736678796856,3.96437177698222,
136.088089627079));
#238282=CARTESIAN_POINT('Ctrl Pts',(-176.015126420669,6.58819063930867,
130.325006956645));
#238283=CARTESIAN_POINT('Ctrl Pts',(-176.293574044481,3.15778415511627,
125.002426882869));
#238284=CARTESIAN_POINT('Ctrl Pts',(-176.572021668294,-3.17447170129595,
125.011540471058));
#238285=CARTESIAN_POINT('Ctrl Pts',(-176.850469292107,-6.58954314578118,
130.343972778891));
#238286=CARTESIAN_POINT('Ctrl Pts',(-177.12891691592,-3.94914635637289,
136.099479019269));
#238287=CARTESIAN_POINT('Ctrl Pts',(-177.407364539733,2.32032300801719,
136.989030129397));
#238288=CARTESIAN_POINT('Ctrl Pts',(-177.685812163546,6.45752888212044,
132.195172096054));
#238289=CARTESIAN_POINT('Ctrl Pts',(-177.964259787359,4.66058118137817,
126.123226258898));
#238290=CARTESIAN_POINT('Ctrl Pts',(-178.242707411172,-1.41921294300185,
124.353014211231));
#238291=CARTESIAN_POINT('Ctrl Pts',(-178.521155034985,-6.19481970517025,
128.511274345191));
#238292=CARTESIAN_POINT('Ctrl Pts',(-178.799602658797,-5.27768979205393,
134.776768739972));
#238293=CARTESIAN_POINT('Ctrl Pts',(-179.078050282611,0.489379210479558,
137.391814133187));
#238294=CARTESIAN_POINT('Ctrl Pts',(-179.356497906423,5.80673262608622,
133.95331156054));
#238295=CARTESIAN_POINT('Ctrl Pts',(-179.634945530236,5.7879824329786,127.621076906106));
#238296=CARTESIAN_POINT('Ctrl Pts',(-179.913393154049,0.450359142625426,
124.214124470449));
#238297=CARTESIAN_POINT('Ctrl Pts',(-180.191840777862,-5.30112219853358,
126.863277103057));
#238298=CARTESIAN_POINT('Ctrl Pts',(-180.470288401675,-6.18113121345664,
133.134092952866));
#238299=CARTESIAN_POINT('Ctrl Pts',(-180.748736025488,-1.38098260826046,
137.263998600285));
#238300=CARTESIAN_POINT('Ctrl Pts',(-181.0271836493,4.68822154917632,135.457812512445));
#238301=CARTESIAN_POINT('Ctrl Pts',(-181.305631273113,6.44917913527537,
129.375331466973));
#238302=CARTESIAN_POINT('Ctrl Pts',(-181.584078896926,2.28365615597197,
124.606058398942));
#238303=CARTESIAN_POINT('Ctrl Pts',(-181.862526520739,-3.98043526786393,
125.532722265928));
#238304=CARTESIAN_POINT('Ctrl Pts',(-182.140974144552,-6.58670113560653,
131.303764244219));
#238305=CARTESIAN_POINT('Ctrl Pts',(-182.419421768365,-3.14011043796568,
136.615878686839));
#238306=CARTESIAN_POINT('Ctrl Pts',(-182.697869392178,3.19208834924215,
136.587491932238));
#238307=CARTESIAN_POINT('Ctrl Pts',(-182.976317015991,6.59091388568205,
131.244690021124));
#238308=CARTESIAN_POINT('Ctrl Pts',(-183.254764639804,3.93301154522339,
125.497246899427));
#238309=CARTESIAN_POINT('Ctrl Pts',(-183.533212263617,-2.33913626699958,
124.626782017781));
#238310=CARTESIAN_POINT('Ctrl Pts',(-183.811659887429,-6.46173212300977,
129.433210077844));
#238311=CARTESIAN_POINT('Ctrl Pts',(-184.090107511242,-4.64631183113728,
135.499658499484));
#238312=CARTESIAN_POINT('Ctrl Pts',(-184.368555135055,1.43884204859816,
137.251357545694));
#238313=CARTESIAN_POINT('Ctrl Pts',(-184.647002758868,6.20177037701405,
133.078581368264));
#238314=CARTESIAN_POINT('Ctrl Pts',(-184.925450382681,5.26557470227994,
126.815907422802));
#238315=CARTESIAN_POINT('Ctrl Pts',(-185.203898006494,-0.50942688622466,
124.218427116558));
#238316=CARTESIAN_POINT('Ctrl Pts',(-185.482345630307,-5.81629005317544,
127.673097957001));
#238317=CARTESIAN_POINT('Ctrl Pts',(-185.76079325412,-5.77826680282389,
134.005246211819));
#238318=CARTESIAN_POINT('Ctrl Pts',(-186.039240877932,-0.430298644703365,
137.395936977472));
#238319=CARTESIAN_POINT('Ctrl Pts',(-186.317688501746,5.31309294664177,
134.729291084778));
#238320=CARTESIAN_POINT('Ctrl Pts',(-186.596136125558,6.17401167904375,
128.455825836229));
#238321=CARTESIAN_POINT('Ctrl Pts',(-186.874583749371,1.36131529564269,
124.340549319425));
#238322=CARTESIAN_POINT('Ctrl Pts',(-187.153031373184,-4.70236334050424,
126.165199610876));
#238323=CARTESIAN_POINT('Ctrl Pts',(-187.431478996997,-6.44479978994851,
132.253012231859));
#238324=CARTESIAN_POINT('Ctrl Pts',(-187.70992662081,-2.26478007840253,
137.009584789872));
#238325=CARTESIAN_POINT('Ctrl Pts',(-187.988374244623,3.99646188453734,
136.063859475589));
#238326=CARTESIAN_POINT('Ctrl Pts',(-188.266821868436,6.58515061360439,
130.284911651585));
#238327=CARTESIAN_POINT('Ctrl Pts',(-188.545269492249,3.12240763126122,
124.983312050825));
#238328=CARTESIAN_POINT('Ctrl Pts',(-188.823717116061,-3.20967542611822,
125.030971708867));
#238329=CARTESIAN_POINT('Ctrl Pts',(-189.102164739874,-6.59222356825658,
130.384093728275));
#238330=CARTESIAN_POINT('Ctrl Pts',(-189.380612363687,-3.91684029919248,
136.123420487763));
#238331=CARTESIAN_POINT('Ctrl Pts',(-189.6590599875,2.35792785654334,136.974791077059));
#238332=CARTESIAN_POINT('Ctrl Pts',(-189.937507611313,6.46587550329532,
132.155837516369));
#238333=CARTESIAN_POINT('Ctrl Pts',(-190.215955235126,4.63199943809816,
126.094942708994));
#238334=CARTESIAN_POINT('Ctrl Pts',(-190.494402858939,-1.45845782495887,
124.361772891742));
#238335=CARTESIAN_POINT('Ctrl Pts',(-190.772850482752,-6.2086635965042,
128.549026456613));
#238336=CARTESIAN_POINT('Ctrl Pts',(-191.051298106565,-5.25341083294129,
134.808821936201));
#238337=CARTESIAN_POINT('Ctrl Pts',(-191.329745730377,0.529469842708527,
137.388713092773));
#238338=CARTESIAN_POINT('Ctrl Pts',(-191.60819335419,5.82579359894846,133.91790598813));
#238339=CARTESIAN_POINT('Ctrl Pts',(-191.886640978003,5.76849764359442,
127.585902793086));
#238340=CARTESIAN_POINT('Ctrl Pts',(-192.165088601816,0.410234160553658,
124.211505108333));
#238341=CARTESIAN_POINT('Ctrl Pts',(-192.443536225629,-5.32501447498302,
126.895619557667));
#238342=CARTESIAN_POINT('Ctrl Pts',(-192.721983849442,-6.16683494942961,
133.171676088433));
#238343=CARTESIAN_POINT('Ctrl Pts',(-193.000431473255,-1.34163537198624,
137.272285351261));
#238344=CARTESIAN_POINT('Ctrl Pts',(-193.278879097068,4.71646156978089,
135.429187759513));
#238345=CARTESIAN_POINT('Ctrl Pts',(-193.557326720881,6.44036074087642,
129.336099959682));
#238346=CARTESIAN_POINT('Ctrl Pts',(-193.835774344694,2.24588302022023,
124.592271975924));
#238347=CARTESIAN_POINT('Ctrl Pts',(-194.114221968506,-4.01245147853337,
125.557049976435));
#238348=CARTESIAN_POINT('Ctrl Pts',(-194.392669592319,-6.58353908766677,
131.343850110767));
#238349=CARTESIAN_POINT('Ctrl Pts',(-194.671117216133,-3.10467589899933,
136.634885756375));
#238350=CARTESIAN_POINT('Ctrl Pts',(-194.949564839945,3.22723276899961,
136.567953636405));
#238351=CARTESIAN_POINT('Ctrl Pts',(-195.228012463758,6.59347218137276,
131.204561099293));
#238352=CARTESIAN_POINT('Ctrl Pts',(-195.506460087571,3.90063276808784,
125.473403870355));
#238353=CARTESIAN_POINT('Ctrl Pts',(-195.784907711384,-2.3766976025655,
124.641135460387));
#238354=CARTESIAN_POINT('Ctrl Pts',(-196.063355335197,-6.46995898459376,
129.472569879579));
#238355=CARTESIAN_POINT('Ctrl Pts',(-196.34180295901,-4.61764413484867,
135.527854925386));
#238356=CARTESIAN_POINT('Ctrl Pts',(-196.620250582823,1.47806009036541,
137.242479457832));
#238357=CARTESIAN_POINT('Ctrl Pts',(-196.898698206635,6.21549929978325,
133.040787295662));
#238358=CARTESIAN_POINT('Ctrl Pts',(-197.177145830448,5.24119829672186,
126.783928271841));
#238359=CARTESIAN_POINT('Ctrl Pts',(-197.455593454261,-0.5495078942556,
124.2216501647));
#238360=CARTESIAN_POINT('Ctrl Pts',(-197.734041078074,-5.83524317536515,
127.708561380459));
#238361=CARTESIAN_POINT('Ctrl Pts',(-198.012488701887,-5.75867504579123,
134.040360856918));
#238362=CARTESIAN_POINT('Ctrl Pts',(-198.2909363257,-0.390165876051177,
137.398434200813));
#238363=CARTESIAN_POINT('Ctrl Pts',(-198.569383949513,5.33688667311775,
134.696876060105));
#238364=CARTESIAN_POINT('Ctrl Pts',(-198.847831573325,6.15960109109908,
128.418286387655));
#238365=CARTESIAN_POINT('Ctrl Pts',(-199.126279197139,1.32194301960288,
124.332382366286));
#238366=CARTESIAN_POINT('Ctrl Pts',(-199.404726820951,-4.73051610640191,
126.193910184127));
#238367=CARTESIAN_POINT('Ctrl Pts',(-199.683174444764,-6.43586202918244,
132.292216717274));
#238368=CARTESIAN_POINT('Ctrl Pts',(-199.961622068577,-2.22696515648391,
137.023256180599));
#238369=CARTESIAN_POINT('Ctrl Pts',(-200.24006969239,4.02840390172748,136.039434431435));
#238370=CARTESIAN_POINT('Ctrl Pts',(-200.518517316203,6.58186657272242,
130.244835594899));
#238371=CARTESIAN_POINT('Ctrl Pts',(-200.796964940016,3.08691540544346,
124.964412919876));
#238372=CARTESIAN_POINT('Ctrl Pts',(-201.075412563829,-3.24476021523692,
125.050616881724));
#238373=CARTESIAN_POINT('Ctrl Pts',(-201.353860187642,-6.59465971346335,
130.424230250803));
#238374=CARTESIAN_POINT('Ctrl Pts',(-201.632307811455,-3.88438910205457,
136.147164856536));
#238375=CARTESIAN_POINT('Ctrl Pts',(-201.910755435267,2.39544533118521,
136.960323377152));
#238376=CARTESIAN_POINT('Ctrl Pts',(-202.18920305908,6.47398252907625,132.116452857208));
#238377=CARTESIAN_POINT('Ctrl Pts',(-202.467650682893,4.60324605437475,
126.066833668302));
#238378=CARTESIAN_POINT('Ctrl Pts',(-202.746098306706,-1.49764866322506,
124.370770304711));
#238379=CARTESIAN_POINT('Ctrl Pts',(-203.024545930519,-6.22227742352606,
128.586862140274));
#238380=CARTESIAN_POINT('Ctrl Pts',(-203.302993554332,-5.22893720675747,
134.840726745644));
#238381=CARTESIAN_POINT('Ctrl Pts',(-203.581441178145,0.569540855237039,
137.385368066758));
#238382=CARTESIAN_POINT('Ctrl Pts',(-203.859888801958,5.84463869488665,
133.882385042152));
#238383=CARTESIAN_POINT('Ctrl Pts',(-204.138336425771,5.7487991004088,127.550847941203));
#238384=CARTESIAN_POINT('Ctrl Pts',(-204.416784049583,0.370093977104817,
124.209130046901));
#238385=CARTESIAN_POINT('Ctrl Pts',(-204.695231673396,-5.34870943106288,
126.928106852114));
#238386=CARTESIAN_POINT('Ctrl Pts',(-204.973679297209,-6.15231017106575,
133.209171502253));
#238387=CARTESIAN_POINT('Ctrl Pts',(-205.252126921022,-1.30223842092043,
137.280332430907));
#238388=CARTESIAN_POINT('Ctrl Pts',(-205.530574544835,4.74452682016742,
135.400391631911));
#238389=CARTESIAN_POINT('Ctrl Pts',(-205.809022168648,6.43130369654214,
129.296922859329));
#238390=CARTESIAN_POINT('Ctrl Pts',(-206.087469792461,2.20802666244648,
124.578715744137));
#238391=CARTESIAN_POINT('Ctrl Pts',(-206.365917416273,-4.04431900633787,
125.581572127967));
#238392=CARTESIAN_POINT('Ctrl Pts',(-206.644365040087,-6.58013308426553,
131.383915986335));
#238393=CARTESIAN_POINT('Ctrl Pts',(-206.922812663899,-3.06912631512495,
136.653676773657));
#238394=CARTESIAN_POINT('Ctrl Pts',(-207.201260287713,3.26225760245914,
136.548201768512));
#238395=CARTESIAN_POINT('Ctrl Pts',(-207.479707911525,6.59578615352751,
131.164417347887));
#238396=CARTESIAN_POINT('Ctrl Pts',(-207.758155535338,3.86810945157081,
125.449758381845));
#238397=CARTESIAN_POINT('Ctrl Pts',(-208.036603159151,-2.41417086872696,
124.655717283569));
#238398=CARTESIAN_POINT('Ctrl Pts',(-208.315050782964,-6.47794609946865,
129.511979031309));
#238399=CARTESIAN_POINT('Ctrl Pts',(-208.593498406777,-4.58880533005852,
135.555876320469));
#238400=CARTESIAN_POINT('Ctrl Pts',(-208.87194603059,1.51722336207232,137.233362803106));
#238401=CARTESIAN_POINT('Ctrl Pts',(-209.150393654402,6.22899790494034,
133.00291035145));
#238402=CARTESIAN_POINT('Ctrl Pts',(-209.428841278216,5.21662767663345,
126.752098099478));
#238403=CARTESIAN_POINT('Ctrl Pts',(-209.707288902028,-0.589568540070009,
124.225117137599));
#238404=CARTESIAN_POINT('Ctrl Pts',(-209.985736525842,-5.85398007047323,
127.744139519898));
#238405=CARTESIAN_POINT('Ctrl Pts',(-210.264184149654,-5.73886989893714,
134.07535559084));
#238406=CARTESIAN_POINT('Ctrl Pts',(-210.542631773467,-0.350018649658268,
137.400687078332));
#238407=CARTESIAN_POINT('Ctrl Pts',(-210.82107939728,5.36048263929459,134.664316796842));
#238408=CARTESIAN_POINT('Ctrl Pts',(-211.099527021093,6.14496225687153,
128.38083535594));
#238409=CARTESIAN_POINT('Ctrl Pts',(-211.377974644906,1.28252175847855,
124.324455234681));
#238410=CARTESIAN_POINT('Ctrl Pts',(-211.656422268719,-4.75849358128477,
126.222791599316));
#238411=CARTESIAN_POINT('Ctrl Pts',(-211.934869892531,-6.4266857851828,
132.331366069634));
#238412=CARTESIAN_POINT('Ctrl Pts',(-212.213317516344,-2.18906771355195,
137.036697127864));
#238413=CARTESIAN_POINT('Ctrl Pts',(-212.491765140157,4.06019664492976,
136.014815399695));
#238414=CARTESIAN_POINT('Ctrl Pts',(-212.770212763971,6.57833863835413,
130.204780271616));
#238415=CARTESIAN_POINT('Ctrl Pts',(-213.048660387783,3.05130879283982,
124.945730190337));
#238416=CARTESIAN_POINT('Ctrl Pts',(-213.327108011596,-3.27972476857289,
125.070475261673));
#238417=CARTESIAN_POINT('Ctrl Pts',(-213.605555635409,-6.59685149112928,
130.464380859201));
#238418=CARTESIAN_POINT('Ctrl Pts',(-213.884003259222,-3.85179396744981,
136.170711245733));
#238419=CARTESIAN_POINT('Ctrl Pts',(-214.162450883035,2.43287404171984,
136.94562756578));
#238420=CARTESIAN_POINT('Ctrl Pts',(-214.440898506847,6.48184965905313,
132.077019577989));
#238421=CARTESIAN_POINT('Ctrl Pts',(-214.71934613066,4.57432209567675,126.038900178414));
#238422=CARTESIAN_POINT('Ctrl Pts',(-214.997793754473,-1.53678400556905,
124.380006116735));
#238423=CARTESIAN_POINT('Ctrl Pts',(-215.276241378286,-6.23566068176903,
128.624779994154));
#238424=CARTESIAN_POINT('Ctrl Pts',(-215.554689002099,-5.20426982038336,
134.872481986055));
#238425=CARTESIAN_POINT('Ctrl Pts',(-215.833136625912,0.609590763220439,
137.381779179092));
#238426=CARTESIAN_POINT('Ctrl Pts',(-216.111584249725,5.86326721558844,
133.846750038845));
#238427=CARTESIAN_POINT('Ctrl Pts',(-216.390031873537,5.72888753335829,
127.51591364943));
#238428=CARTESIAN_POINT('Ctrl Pts',(-216.668479497351,0.329940079686948,
124.206999374164));
#238429=CARTESIAN_POINT('Ctrl Pts',(-216.946927121163,-5.37220618874772,
126.960737782571));
#238430=CARTESIAN_POINT('Ctrl Pts',(-217.225374744977,-6.13755741658593,
133.246577804923));
#238431=CARTESIAN_POINT('Ctrl Pts',(-217.503822368789,-1.26279321493052,
137.288139541036));
#238432=CARTESIAN_POINT('Ctrl Pts',(-217.782269992602,4.77241626036792,
135.37142519669));
#238433=CARTESIAN_POINT('Ctrl Pts',(-218.060717616415,6.4220083378839,129.257801617636));
#238434=CARTESIAN_POINT('Ctrl Pts',(-218.339165240228,2.17008848543354,
124.565390205911));
#238435=CARTESIAN_POINT('Ctrl Pts',(-218.617612864041,-4.07603667041411,
125.606287811847));
#238436=CARTESIAN_POINT('Ctrl Pts',(-218.896060487854,-6.57648325161253,
131.423960386264));
#238437=CARTESIAN_POINT('Ctrl Pts',(-219.174508111666,-3.03346300364714,
136.672251042379));
#238438=CARTESIAN_POINT('Ctrl Pts',(-219.45295573548,3.29716155176439,136.528237060474));
#238439=CARTESIAN_POINT('Ctrl Pts',(-219.731403359293,6.59785571640026,
131.124260254445));
#238440=CARTESIAN_POINT('Ctrl Pts',(-220.009850983105,3.83544280083539,
125.426311310091));
#238441=CARTESIAN_POINT('Ctrl Pts',(-220.288298606918,-2.45155467689987,
124.67052694699));
#238442=CARTESIAN_POINT('Ctrl Pts',(-220.566746230731,-6.48569317166813,
129.551436072715));
#238443=CARTESIAN_POINT('Ctrl Pts',(-220.845193854544,-4.55979648539947,
135.58372164639));
#238444=CARTESIAN_POINT('Ctrl Pts',(-221.123641478357,1.55633041250914,
137.224007919343));
#238445=CARTESIAN_POINT('Ctrl Pts',(-221.40208910217,6.24226569228925,132.964951939167));
#238446=CARTESIAN_POINT('Ctrl Pts',(-221.680536725983,5.19186375248807,
126.720418085194));
#238447=CARTESIAN_POINT('Ctrl Pts',(-221.958984349796,-0.629607339204784,
124.228827906785));
#238448=CARTESIAN_POINT('Ctrl Pts',(-222.237431973609,-5.87250004419688,
127.779831056953));
#238449=CARTESIAN_POINT('Ctrl Pts',(-222.515879597421,-5.71885209614835,
134.110229116839));
#238450=CARTESIAN_POINT('Ctrl Pts',(-222.794327221234,-0.309858453196267,
137.402695526548));
#238451=CARTESIAN_POINT('Ctrl Pts',(-223.072774845047,5.38387997081673,
134.631614501482));
#238452=CARTESIAN_POINT('Ctrl Pts',(-223.35122246886,6.13009571880702,128.343474128844));
#238453=CARTESIAN_POINT('Ctrl Pts',(-223.629670092673,1.24305297303857,
124.316768218352));
#238454=CARTESIAN_POINT('Ctrl Pts',(-223.908117716486,-4.78629472843886,
126.25184278623));
#238455=CARTESIAN_POINT('Ctrl Pts',(-224.186565340298,-6.41727139797729,
132.370458838244));
#238456=CARTESIAN_POINT('Ctrl Pts',(-224.465012964112,-2.15108915391133,
137.049907133607));
#238457=CARTESIAN_POINT('Ctrl Pts',(-224.743460587925,4.09183893605206,
135.990003292637));
#238458=CARTESIAN_POINT('Ctrl Pts',(-225.021908211737,6.57456694122844,
130.164747166004));
#238459=CARTESIAN_POINT('Ctrl Pts',(-225.300355835551,3.01558911286705,
124.927264554503));
#238460=CARTESIAN_POINT('Ctrl Pts',(-225.578803459363,-3.31456779050113,
125.090546112851));
#238461=CARTESIAN_POINT('Ctrl Pts',(-225.857251083176,-6.5987988200372,
130.504544065675));
#238462=CARTESIAN_POINT('Ctrl Pts',(-226.135698706989,-3.8190561032033,
136.194058782834));
#238463=CARTESIAN_POINT('Ctrl Pts',(-226.414146330802,2.47021260121173,
136.930704187504));
#238464=CARTESIAN_POINT('Ctrl Pts',(-226.692593954615,6.48947660170784,
132.037539139922));
#238465=CARTESIAN_POINT('Ctrl Pts',(-226.971041578427,4.54522863379049,
126.011143274415));
#238466=CARTESIAN_POINT('Ctrl Pts',(-227.24948920224,-1.57586240181677,
124.389479985577));
#238467=CARTESIAN_POINT('Ctrl Pts',(-227.527936826054,-6.24881287531301,
128.662778613197));
#238468=CARTESIAN_POINT('Ctrl Pts',(-227.806384449866,-5.17940958787633,
134.904086480733));
#238469=CARTESIAN_POINT('Ctrl Pts',(-228.084832073679,0.649618082593193,
137.377946562762));
#238470=CARTESIAN_POINT('Ctrl Pts',(-228.363279697492,5.88167847076755,
133.811002298682));
#238471=CARTESIAN_POINT('Ctrl Pts',(-228.641727321305,5.70876368027354,
127.481101212267));
#238472=CARTESIAN_POINT('Ctrl Pts',(-228.920174945118,0.289773956218704,
124.205113169075));
#238473=CARTESIAN_POINT('Ctrl Pts',(-229.198622568931,-5.39550387735667,
126.993511139885));
#238474=CARTESIAN_POINT('Ctrl Pts',(-229.477070192744,-6.12257723265909,
133.283893610337));
#238475=CARTESIAN_POINT('Ctrl Pts',(-229.755517816557,-1.22330121567356,
137.295706392352));
#238476=CARTESIAN_POINT('Ctrl Pts',(-230.033965440369,4.80012885692891,
135.34228952721));
#238477=CARTESIAN_POINT('Ctrl Pts',(-230.312413064183,6.41247500934538,
129.218737684256));
#238478=CARTESIAN_POINT('Ctrl Pts',(-230.590860687995,2.13206989499296,
124.552295855027));
#238479=CARTESIAN_POINT('Ctrl Pts',(-230.869308311808,-4.10760329545278,
125.631196112227));
#238480=CARTESIAN_POINT('Ctrl Pts',(-231.147755935621,-6.5725897249546,
131.463981826697));
#238481=CARTESIAN_POINT('Ctrl Pts',(-231.426203559434,-2.99768728608136,
136.690607874263));
#238482=CARTESIAN_POINT('Ctrl Pts',(-231.704651183247,3.33194332353496,
136.508060252089));
#238483=CARTESIAN_POINT('Ctrl Pts',(-231.98309880706,6.59968079330357,131.084091307006));
#238484=CARTESIAN_POINT('Ctrl Pts',(-232.261546430872,3.80263402635669,
125.403063523931));
#238485=CARTESIAN_POINT('Ctrl Pts',(-232.539994054686,-2.48884764181187,
124.685563901874));
#238486=CARTESIAN_POINT('Ctrl Pts',(-232.818441678498,-6.49319991412244,
129.5909395417));
#238487=CARTESIAN_POINT('Ctrl Pts',(-233.096889302311,-4.53061867580467,
135.611389871331));
#238488=CARTESIAN_POINT('Ctrl Pts',(-233.375336926124,1.59537979255065,
137.214415153187));
#238489=CARTESIAN_POINT('Ctrl Pts',(-233.653784549937,6.25530217018742,
132.926913465378));
#238490=CARTESIAN_POINT('Ctrl Pts',(-233.93223217375,5.16690744192206,126.688889402902));
#238491=CARTESIAN_POINT('Ctrl Pts',(-234.210679797563,-0.669622808008655,
124.232782334755));
#238492=CARTESIAN_POINT('Ctrl Pts',(-234.489127421376,-5.89080241027189,
127.815634669064));
#238493=CARTESIAN_POINT('Ctrl Pts',(-234.767575045188,-5.69862237919218,
134.144980142666));
#238494=CARTESIAN_POINT('Ctrl Pts',(-235.046022669002,-0.269686774814632,
137.404459471037));
#238495=CARTESIAN_POINT('Ctrl Pts',(-235.324470292814,5.40707780068583,
134.598770385822));
#238496=CARTESIAN_POINT('Ctrl Pts',(-235.602917916627,6.11500202779203,
128.306204090801));
#238497=CARTESIAN_POINT('Ctrl Pts',(-235.88136554044,1.20353812581378,124.309321602146));
#238498=CARTESIAN_POINT('Ctrl Pts',(-236.159813164253,-4.81391851768082,
126.281062668365));
#238499=CARTESIAN_POINT('Ctrl Pts',(-236.438260788066,-6.40761921642086,
132.40949357451));
#238500=CARTESIAN_POINT('Ctrl Pts',(-236.716708411879,-2.11303088487057,
137.062885708328));
#238501=CARTESIAN_POINT('Ctrl Pts',(-236.995156035692,4.12332960257798,
135.964999029683));
#238502=CARTESIAN_POINT('Ctrl Pts',(-237.273603659505,6.57055162110693,
130.124737761504));
#238503=CARTESIAN_POINT('Ctrl Pts',(-237.552051283318,2.97975768913041,
124.909016696624));
#238504=CARTESIAN_POINT('Ctrl Pts',(-237.83049890713,-3.34928798990126,
125.110828691528));
#238505=CARTESIAN_POINT('Ctrl Pts',(-238.108946530943,-6.60050162802816,
130.544718381962));
#238506=CARTESIAN_POINT('Ctrl Pts',(-238.387394154756,-3.7861767224282,
136.217206602688));
#238507=CARTESIAN_POINT('Ctrl Pts',(-238.665841778569,2.5074596260677,136.915553795314));
#238508=CARTESIAN_POINT('Ctrl Pts',(-238.944289402382,6.49686307441993,
131.998013005973));
#238509=CARTESIAN_POINT('Ctrl Pts',(-239.222737026195,4.51596674678651,
125.983563984846));
#238510=CARTESIAN_POINT('Ctrl Pts',(-239.501184650008,-1.61488240390346,
124.399191560181));
#238511=CARTESIAN_POINT('Ctrl Pts',(-239.77963227382,-6.26173351679718,
128.700856589348));
#238512=CARTESIAN_POINT('Ctrl Pts',(-240.058079897633,-5.15435743044315,
134.935539058562));
#238513=CARTESIAN_POINT('Ctrl Pts',(-240.336527521446,0.689621330129741,
137.373870359787));
#238514=CARTESIAN_POINT('Ctrl Pts',(-240.614975145259,5.89987177818775,
133.775143146303));
#238515=CARTESIAN_POINT('Ctrl Pts',(-240.893422769072,5.68842828685113,
127.446411919705));
#238516=CARTESIAN_POINT('Ctrl Pts',(-241.171870392886,0.249597095069331,
124.203471501526));
#238517=CARTESIAN_POINT('Ctrl Pts',(-241.450318016698,-5.41860163358522,
127.026425709627));
#238518=CARTESIAN_POINT('Ctrl Pts',(-241.728765640511,-6.10737017438111,
133.321117535742));
#238519=CARTESIAN_POINT('Ctrl Pts',(-242.007213264324,-1.18376388654087,
137.303032704464));
#238520=CARTESIAN_POINT('Ctrl Pts',(-242.285660888137,4.82766358294966,
135.312985703106));
#238521=CARTESIAN_POINT('Ctrl Pts',(-242.56410851195,6.40270406418687,129.179732506718));
#238522=CARTESIAN_POINT('Ctrl Pts',(-242.842556135762,2.09397229991911,
124.539433176702));
#238523=CARTESIAN_POINT('Ctrl Pts',(-243.121003759575,-4.13901771174057,
125.65629610612));
#238524=CARTESIAN_POINT('Ctrl Pts',(-243.399451383388,-6.56845264856689,
131.503978824623));
#238525=CARTESIAN_POINT('Ctrl Pts',(-243.677899007202,-2.9618004881116,
136.70874658909));
#238526=CARTESIAN_POINT('Ctrl Pts',(-243.956346631013,3.36660162892119,
136.487672091016));
#238527=CARTESIAN_POINT('Ctrl Pts',(-244.234794254827,6.60126131660758,
131.043911994042));
#238528=CARTESIAN_POINT('Ctrl Pts',(-244.513241878639,3.76968434387551,
125.380015884821));
#238529=CARTESIAN_POINT('Ctrl Pts',(-244.791689502453,-2.52604838156001,
124.70082759102));
#238530=CARTESIAN_POINT('Ctrl Pts',(-245.070137126265,-6.50046604866569,
129.630487974449));
#238531=CARTESIAN_POINT('Ctrl Pts',(-245.348584750079,-4.50127298246883,
135.638879970036));
#238532=CARTESIAN_POINT('Ctrl Pts',(-245.627032373891,1.63437005520677,
137.204584860103));
#238533=CARTESIAN_POINT('Ctrl Pts',(-245.905479997704,6.26810685556324,
132.888796339615));
#238534=CARTESIAN_POINT('Ctrl Pts',(-246.183927621517,5.14175966970064,
126.65751322091));
#238535=CARTESIAN_POINT('Ctrl Pts',(-246.46237524533,-0.709613463692526,
124.236980274974));
#238536=CARTESIAN_POINT('Ctrl Pts',(-246.740822869143,-5.90888649049716,
127.851549029514));
#238537=CARTESIAN_POINT('Ctrl Pts',(-247.019270492956,-5.67818149768794,
134.179607380607));
#238538=CARTESIAN_POINT('Ctrl Pts',(-247.297718116769,-0.229505103091092,
137.405978846438));
#238539=CARTESIAN_POINT('Ctrl Pts',(-247.576165740581,5.43007526929941,
134.565785666913));
#238540=CARTESIAN_POINT('Ctrl Pts',(-247.854613364394,6.09968174312738,
128.269026622868));
#238541=CARTESIAN_POINT('Ctrl Pts',(-248.133060988207,1.16397868104094,
124.302115661998));
#238542=CARTESIAN_POINT('Ctrl Pts',(-248.41150861202,-4.84136392540264,
126.31045016297));
#238543=CARTESIAN_POINT('Ctrl Pts',(-248.689956235833,-6.39772959817725,
132.448468831983));
#238544=CARTESIAN_POINT('Ctrl Pts',(-248.968403859646,-2.07489431669385,
137.075632371099));
#238545=CARTESIAN_POINT('Ctrl Pts',(-249.246851483459,4.15466747760909,
135.939803537374));
#238546=CARTESIAN_POINT('Ctrl Pts',(-249.525299107272,6.56629282677857,
130.08475354068));
#238547=CARTESIAN_POINT('Ctrl Pts',(-249.803746731085,2.94381584937754,
124.890987292882));
#238548=CARTESIAN_POINT('Ctrl Pts',(-250.082194354898,-3.38388408020374,
125.131322246124));
#238549=CARTESIAN_POINT('Ctrl Pts',(-250.36064197871,-6.60195985200274,
130.584902319384));
#238550=CARTESIAN_POINT('Ctrl Pts',(-250.639089602524,-3.75315704348482,
136.240153847548));
#238551=CARTESIAN_POINT('Ctrl Pts',(-250.917537226336,2.54461373609029,
136.900176950603));
#238552=CARTESIAN_POINT('Ctrl Pts',(-251.19598485015,6.50400880347224,131.958442640812));
#238553=CARTESIAN_POINT('Ctrl Pts',(-251.474432473962,4.48653751899202,
125.956163331638));
#238554=CARTESIAN_POINT('Ctrl Pts',(-251.752880097775,-1.65384256596459,
124.409140480742));
#238555=CARTESIAN_POINT('Ctrl Pts',(-252.031327721588,-6.27442212737671,
128.739012511497));
#238556=CARTESIAN_POINT('Ctrl Pts',(-252.309775345401,-5.12911427652582,
134.966838554275));
#238557=CARTESIAN_POINT('Ctrl Pts',(-252.588222969213,0.729599023732927,
137.369550720794));
#238558=CARTESIAN_POINT('Ctrl Pts',(-252.866670593027,5.91784646323776,
133.739173911277));
#238559=CARTESIAN_POINT('Ctrl Pts',(-253.145118216839,5.66788210748017,
127.411847055674));
#238560=CARTESIAN_POINT('Ctrl Pts',(-253.423565840652,0.209410983396998,
124.20207443517));
#238561=CARTESIAN_POINT('Ctrl Pts',(-253.702013464465,-5.44149859849489,
127.059480266814));
#238562=CARTESIAN_POINT('Ctrl Pts',(-253.980461088278,-6.0919368110008,
133.358248211846));
#238563=CARTESIAN_POINT('Ctrl Pts',(-254.258908712091,-1.1441826817532,
137.310118186916));
#238564=CARTESIAN_POINT('Ctrl Pts',(-254.537356335904,4.85501939763767,
135.283514846073));
#238565=CARTESIAN_POINT('Ctrl Pts',(-254.815803959717,6.39269590315201,
129.140787462715));
#238566=CARTESIAN_POINT('Ctrl Pts',(-255.09425158353,2.05579703890082,124.526802775315));
#238567=CARTESIAN_POINT('Ctrl Pts',(-255.372699207342,-4.17027861730954,
125.681586622223));
#238568=CARTESIAN_POINT('Ctrl Pts',(-255.651146831155,-6.5640724361261,
131.5439503534));
#238569=CARTESIAN_POINT('Ctrl Pts',(-255.929594454968,-2.925803447894,136.726665654721));
#238570=CARTESIAN_POINT('Ctrl Pts',(-256.208042078781,3.40113425532747,
136.467074956607));
#238571=CARTESIAN_POINT('Ctrl Pts',(-256.486489702594,6.60259898059897,
131.003720738236));
#238572=CARTESIAN_POINT('Ctrl Pts',(-256.764937326407,3.73659166461274,
125.357175036369));
#238573=CARTESIAN_POINT('Ctrl Pts',(-257.04338495022,-2.56314926818932,
124.716306516944));
#238574=CARTESIAN_POINT('Ctrl Pts',(-257.321832574033,-6.5075031063131,
129.670100547101));
#238575=CARTESIAN_POINT('Ctrl Pts',(-257.600280197845,-4.47173821150659,
135.666151948257));
#238576=CARTESIAN_POINT('Ctrl Pts',(-257.878727821659,1.67325768403046,
137.194590998305));
#238577=CARTESIAN_POINT('Ctrl Pts',(-258.157175445471,6.28075871394982,
132.850463013089));
#238578=CARTESIAN_POINT('Ctrl Pts',(-258.435623069284,5.1162713672671,126.626553096149));
#238579=CARTESIAN_POINT('Ctrl Pts',(-258.714070693097,-0.749294580734974,
124.240926059104));
#238580=CARTESIAN_POINT('Ctrl Pts',(-258.99251831691,-5.92728653745133,
127.888508918958));
#238581=CARTESIAN_POINT('Ctrl Pts',(-259.270965940723,-5.656519339957,134.212338033208));
#238582=CARTESIAN_POINT('Ctrl Pts',(-259.549413564536,-0.191230405826049,
137.41063083554));
#238583=CARTESIAN_POINT('Ctrl Pts',(-259.827861188349,5.45654320709978,
134.526020746857));
#238584=CARTESIAN_POINT('Ctrl Pts',(-260.059900874859,5.97341346954355,
129.293215926205));
#238585=CARTESIAN_POINT('Ctrl Pts',(-260.245542550368,3.60742224527213,
126.247226657536));
#238586=CARTESIAN_POINT('Ctrl Pts',(-260.338368351272,1.86717727106152,
125.459413119698));
#238587=CARTESIAN_POINT('Ctrl Pts',(-260.384786214875,0.950008195528324,
125.301089073499));
#238588=CARTESIAN_POINT('Ctrl Pts',(209.997886486728,-2.58542267678463,
125.478296443779));
#238589=CARTESIAN_POINT('Ctrl Pts',(209.951476810375,-3.47289965896197,
125.909102290886));
#238590=CARTESIAN_POINT('Ctrl Pts',(209.85865919672,-5.01373755653622,127.222906143875));
#238591=CARTESIAN_POINT('Ctrl Pts',(209.67302570846,-6.52844908712303,131.020616473957));
#238592=CARTESIAN_POINT('Ctrl Pts',(209.440986021949,-4.4641631800594,136.198709217918));
#238593=CARTESIAN_POINT('Ctrl Pts',(209.162538398136,2.13623200523086,137.47712630299));
#238594=CARTESIAN_POINT('Ctrl Pts',(208.884090774324,6.76311047611758,132.61329501932));
#238595=CARTESIAN_POINT('Ctrl Pts',(208.60564315051,5.180460236421,126.09244423763));
#238596=CARTESIAN_POINT('Ctrl Pts',(208.327195526698,-1.16565068102074,
123.898824768668));
#238597=CARTESIAN_POINT('Ctrl Pts',(208.048747902884,-6.43906639651766,
128.052530506575));
#238598=CARTESIAN_POINT('Ctrl Pts',(207.770300279072,-5.79609906993421,
134.734252735451));
#238599=CARTESIAN_POINT('Ctrl Pts',(207.491852655259,0.173626147510206,
137.805009652024));
#238600=CARTESIAN_POINT('Ctrl Pts',(207.213405031446,5.98357180802623,134.442293088818));
#238601=CARTESIAN_POINT('Ctrl Pts',(206.934957407633,6.29502677410122,127.736610299611));
#238602=CARTESIAN_POINT('Ctrl Pts',(206.65650978382,0.821596385081328,123.849978754804));
#238603=CARTESIAN_POINT('Ctrl Pts',(206.378062160007,-5.40680743188727,
126.354116934927));
#238604=CARTESIAN_POINT('Ctrl Pts',(206.099614536195,-6.66663710465116,
132.947794423038));
#238605=CARTESIAN_POINT('Ctrl Pts',(205.821166912381,-1.80014356190772,
137.571770081489));
#238606=CARTESIAN_POINT('Ctrl Pts',(205.542719288569,4.72058899422897,135.976822216287));
#238607=CARTESIAN_POINT('Ctrl Pts',(205.264271664756,6.90333351468265,129.628637390042));
#238608=CARTESIAN_POINT('Ctrl Pts',(204.985824040943,2.74225038547515,124.360883417158));
#238609=CARTESIAN_POINT('Ctrl Pts',(204.70737641713,-3.93882614214087,125.014370927945));
#238610=CARTESIAN_POINT('Ctrl Pts',(204.428928793317,-7.00031425910704,
130.988575726592));
#238611=CARTESIAN_POINT('Ctrl Pts',(204.150481169504,-3.62885534891233,
136.793496040797));
#238612=CARTESIAN_POINT('Ctrl Pts',(203.872033545692,3.07734423765085,137.09469337995));
#238613=CARTESIAN_POINT('Ctrl Pts',(203.593585921878,6.95561486460971,131.615382266785));
#238614=CARTESIAN_POINT('Ctrl Pts',(203.315138298066,4.44201520086038,125.390781848689));
#238615=CARTESIAN_POINT('Ctrl Pts',(203.036690674253,-2.15357941165663,
124.140995867004));
#238616=CARTESIAN_POINT('Ctrl Pts',(202.75824305044,-6.77013976170558,129.014516559232));
#238617=CARTESIAN_POINT('Ctrl Pts',(202.479795426627,-5.16527240588502,
135.532816506767));
#238618=CARTESIAN_POINT('Ctrl Pts',(202.201347802814,1.18622795093483,137.705896487686));
#238619=CARTESIAN_POINT('Ctrl Pts',(201.922900179001,6.44764277258624,133.536802163981));
#238620=CARTESIAN_POINT('Ctrl Pts',(201.644452555188,5.78398887041165,126.856727545651));
#238621=CARTESIAN_POINT('Ctrl Pts',(201.366004931376,-0.194868239746226,
123.804334868162));
#238622=CARTESIAN_POINT('Ctrl Pts',(201.087557307562,-5.99465095761073,
127.184623883922));
#238623=CARTESIAN_POINT('Ctrl Pts',(200.80910968375,-6.2856423003101,133.891274124028));
#238624=CARTESIAN_POINT('Ctrl Pts',(200.530662059936,-0.80043543977546,
137.76120165575));
#238625=CARTESIAN_POINT('Ctrl Pts',(200.252214436124,5.42033248649604,135.238132133988));
#238626=CARTESIAN_POINT('Ctrl Pts',(199.973766812311,6.66007965562565,128.640643190398));
#238627=CARTESIAN_POINT('Ctrl Pts',(199.695319188498,1.77953898422249,124.031504858911));
#238628=CARTESIAN_POINT('Ctrl Pts',(199.416871564685,-4.73631107837294,
125.646290097223));
#238629=CARTESIAN_POINT('Ctrl Pts',(199.138423940872,-6.89972264160091,
132.00109015798));
#238630=CARTESIAN_POINT('Ctrl Pts',(198.859976317059,-2.72262616738874,
137.256154234582));
#238631=CARTESIAN_POINT('Ctrl Pts',(198.581528693247,3.95643074697165,136.582335164788));
#238632=CARTESIAN_POINT('Ctrl Pts',(198.303081069434,6.999721087252,130.598839755845));
#238633=CARTESIAN_POINT('Ctrl Pts',(198.024633445621,3.61060970373355,124.804207978572));
#238634=CARTESIAN_POINT('Ctrl Pts',(197.746185821808,-3.09647560942607,
124.523423352781));
#238635=CARTESIAN_POINT('Ctrl Pts',(197.467738197995,-6.9580511087663,130.014513232485));
#238636=CARTESIAN_POINT('Ctrl Pts',(197.189290574182,-4.4255175588443,136.231434272887));
#238637=CARTESIAN_POINT('Ctrl Pts',(196.910842950369,2.17385042910367,137.461139751337));
#238638=CARTESIAN_POINT('Ctrl Pts',(196.632395326556,6.77555607120273,132.573590407591));
#238639=CARTESIAN_POINT('Ctrl Pts',(196.353947702743,5.15085668818228,126.060205318492));
#238640=CARTESIAN_POINT('Ctrl Pts',(196.07550007893,-1.20722835793932,123.90646718437));
#238641=CARTESIAN_POINT('Ctrl Pts',(195.797052455118,-6.45592951949867,
128.091556134528));
#238642=CARTESIAN_POINT('Ctrl Pts',(195.518604831305,-5.77194684232935,
134.769579876729));
#238643=CARTESIAN_POINT('Ctrl Pts',(195.240157207492,0.216173007661386,
137.80376083149));
#238644=CARTESIAN_POINT('Ctrl Pts',(194.961709583679,6.00564042424985,134.405834929363));
#238645=CARTESIAN_POINT('Ctrl Pts',(194.683261959866,6.2762176827981,127.698330076496));
#238646=CARTESIAN_POINT('Ctrl Pts',(194.404814336053,0.779257501134259,
123.845115552844));
#238647=CARTESIAN_POINT('Ctrl Pts',(194.12636671224,-5.43380225522669,126.387107265649));
#238648=CARTESIAN_POINT('Ctrl Pts',(193.847919088427,-6.65346319503207,
132.988339014042));
#238649=CARTESIAN_POINT('Ctrl Pts',(193.569471464615,-1.75891649835014,
137.58260130935));
#238650=CARTESIAN_POINT('Ctrl Pts',(193.291023840801,4.75198853246758,135.947991544374));
#238651=CARTESIAN_POINT('Ctrl Pts',(193.012576216989,6.89604824949333,129.586636238002));
#238652=CARTESIAN_POINT('Ctrl Pts',(192.734128593176,2.70297651592057,124.344310147306));
#238653=CARTESIAN_POINT('Ctrl Pts',(192.455680969363,-3.97399858803937,
125.038454847768));
#238654=CARTESIAN_POINT('Ctrl Pts',(192.17723334555,-6.99906313021511,131.031185270517));
#238655=CARTESIAN_POINT('Ctrl Pts',(191.898785721737,-3.59233057896577,
136.815474918205));
#238656=CARTESIAN_POINT('Ctrl Pts',(191.620338097924,3.11557827924791,137.075844182864));
#238657=CARTESIAN_POINT('Ctrl Pts',(191.341890474111,6.96042290329331,131.573026430018));
#238658=CARTESIAN_POINT('Ctrl Pts',(191.063442850298,4.40897891477476,125.363842346942));
#238659=CARTESIAN_POINT('Ctrl Pts',(190.784995226486,-2.19410130582752,
124.154228770475));
#238660=CARTESIAN_POINT('Ctrl Pts',(190.506547602672,-6.78090961418206,
129.055761484483));
#238661=CARTESIAN_POINT('Ctrl Pts',(190.22809997886,-5.13639325295408,135.564171377977));
#238662=CARTESIAN_POINT('Ctrl Pts',(189.949652355047,1.22821758097839,137.698547712335));
#238663=CARTESIAN_POINT('Ctrl Pts',(189.671204731234,6.46415645975623,133.497502906364));
#238664=CARTESIAN_POINT('Ctrl Pts',(189.392757107421,5.75985134361714,126.821591904301));
#238665=CARTESIAN_POINT('Ctrl Pts',(189.114309483608,-0.237475772924818,
123.80565078066));
#238666=CARTESIAN_POINT('Ctrl Pts',(188.835861859795,-6.01657425548534,
127.221182091151));
#238667=CARTESIAN_POINT('Ctrl Pts',(188.557414235982,-6.2667349232476,133.929479419415));
#238668=CARTESIAN_POINT('Ctrl Pts',(188.278966612169,-0.758072343566082,
137.76594523932));
#238669=CARTESIAN_POINT('Ctrl Pts',(188.000518988357,5.44722168595988,135.205054884148));
#238670=CARTESIAN_POINT('Ctrl Pts',(187.722071364544,6.64678509766207,128.600141483854));
#238671=CARTESIAN_POINT('Ctrl Pts',(187.443623740731,1.73827771811677,124.02079778535));
#238672=CARTESIAN_POINT('Ctrl Pts',(187.165176116918,-4.76762196479028,
125.675216934184));
#238673=CARTESIAN_POINT('Ctrl Pts',(186.886728493105,-6.89230997333645,
132.043068555446));
#238674=CARTESIAN_POINT('Ctrl Pts',(186.608280869292,-2.68330182444739,
137.272608096043));
#238675=CARTESIAN_POINT('Ctrl Pts',(186.329833245479,3.99152961452714,136.558144195375));
#238676=CARTESIAN_POINT('Ctrl Pts',(186.051385621667,6.99834033481346,130.556234274655));
#238677=CARTESIAN_POINT('Ctrl Pts',(185.772937997853,3.5740181753383,124.782340341422));
#238678=CARTESIAN_POINT('Ctrl Pts',(185.494490374041,-3.13465208677821,
124.542388849921));
#238679=CARTESIAN_POINT('Ctrl Pts',(185.216042750227,-6.96273021741339,
130.056883498557));
#238680=CARTESIAN_POINT('Ctrl Pts',(184.937595126415,-4.39239942652681,
136.258273103275));
#238681=CARTESIAN_POINT('Ctrl Pts',(184.659147502602,2.21433185669671,137.447783572063));
#238682=CARTESIAN_POINT('Ctrl Pts',(184.380699878789,6.78620033974098,132.532312894923));
#238683=CARTESIAN_POINT('Ctrl Pts',(184.102252254976,5.12188223488049,126.028938490053));
#238684=CARTESIAN_POINT('Ctrl Pts',(183.823804631163,-1.24919542597752,
123.913943728027));
#238685=CARTESIAN_POINT('Ctrl Pts',(183.54535700735,-6.47232351695142,128.130905471908));
#238686=CARTESIAN_POINT('Ctrl Pts',(183.266909383538,-5.74770248642891,
134.804641889104));
#238687=CARTESIAN_POINT('Ctrl Pts',(182.988461759724,0.258776338245136,
137.80231524236));
#238688=CARTESIAN_POINT('Ctrl Pts',(182.710014135912,6.02745234999885,134.369210164519));
#238689=CARTESIAN_POINT('Ctrl Pts',(182.431566512099,6.25719410952084,127.66018250561));
#238690=CARTESIAN_POINT('Ctrl Pts',(182.153118888286,0.73688016331929,123.840500929948));
#238691=CARTESIAN_POINT('Ctrl Pts',(181.874671264473,-5.46059065437546,
126.420266203747));
#238692=CARTESIAN_POINT('Ctrl Pts',(181.59622364066,-6.64004542538295,133.028800068927));
#238693=CARTESIAN_POINT('Ctrl Pts',(181.317776016847,-1.71762283471616,
137.593182748215));
#238694=CARTESIAN_POINT('Ctrl Pts',(181.039328393035,4.78321123051439,135.918969541833));
#238695=CARTESIAN_POINT('Ctrl Pts',(180.760880769221,6.88850784776155,129.544680596588));
#238696=CARTESIAN_POINT('Ctrl Pts',(180.482433145409,2.66360227523266,124.32797605183));
#238697=CARTESIAN_POINT('Ctrl Pts',(180.203985521595,-4.00902366402984,
125.062752534008));
#238698=CARTESIAN_POINT('Ctrl Pts',(179.925537897783,-6.99755270774298,
131.073786351827));
#238699=CARTESIAN_POINT('Ctrl Pts',(179.64709027397,-3.5556726624947,136.837231082039));
#238700=CARTESIAN_POINT('Ctrl Pts',(179.368642650157,3.15369685531979,137.056762577506));
#238701=CARTESIAN_POINT('Ctrl Pts',(179.090195026344,6.96497302975191,131.530642118605));
#238702=CARTESIAN_POINT('Ctrl Pts',(178.811747402531,4.37577924769062,125.337104441072));
#238703=CARTESIAN_POINT('Ctrl Pts',(178.533299778718,-2.23454189429802,
124.167708099424));
#238704=CARTESIAN_POINT('Ctrl Pts',(178.254852154906,-6.79142819886702,
129.097071203448));
#238705=CARTESIAN_POINT('Ctrl Pts',(177.976404531092,-5.10732376838957,
135.595349873321));
#238706=CARTESIAN_POINT('Ctrl Pts',(177.69795690728,1.27016169860089,137.690943469992));
#238707=CARTESIAN_POINT('Ctrl Pts',(177.419509283467,6.48043061542571,133.458103853558));
#238708=CARTESIAN_POINT('Ctrl Pts',(177.141061659654,5.73550038331004,126.786603845811));
#238709=CARTESIAN_POINT('Ctrl Pts',(176.862614035841,-0.280074506296806,
123.807226032976));
#238710=CARTESIAN_POINT('Ctrl Pts',(176.584166412028,-6.0382746070172,127.257873074351));
#238711=CARTESIAN_POINT('Ctrl Pts',(176.305718788215,-6.24759533000263,
133.967568912391));
#238712=CARTESIAN_POINT('Ctrl Pts',(176.027271164402,-0.71568115671533,
137.770430858802));
#238713=CARTESIAN_POINT('Ctrl Pts',(175.748823540589,5.4739090366252,135.171814564968));
#238714=CARTESIAN_POINT('Ctrl Pts',(175.470375916777,6.63324424063007,128.559721455457));
#238715=CARTESIAN_POINT('Ctrl Pts',(175.191928292964,1.69695203949225,124.010342079205));
#238716=CARTESIAN_POINT('Ctrl Pts',(174.913480669151,-4.79875618522306,
125.704333833448));
#238717=CARTESIAN_POINT('Ctrl Pts',(174.635033045338,-6.88464190799096,
132.085001052137));
#238718=CARTESIAN_POINT('Ctrl Pts',(174.356585421525,-2.64387805077028,
137.288822274217));
#238719=CARTESIAN_POINT('Ctrl Pts',(174.078137797712,4.02648057448505,136.533740017397));
#238720=CARTESIAN_POINT('Ctrl Pts',(173.799690173899,6.99670025630013,130.513637987877));
#238721=CARTESIAN_POINT('Ctrl Pts',(173.521242550086,3.53729421038521,124.76069585245));
#238722=CARTESIAN_POINT('Ctrl Pts',(173.242794926273,-3.17271240844464,
124.561586386726));
#238723=CARTESIAN_POINT('Ctrl Pts',(172.96434730246,-6.96715131953175,130.099281462668));
#238724=CARTESIAN_POINT('Ctrl Pts',(172.685899678648,-4.35911853223319,
136.284909836929));
#238725=CARTESIAN_POINT('Ctrl Pts',(172.407452054835,2.25473123140845,137.434181218309));
#238726=CARTESIAN_POINT('Ctrl Pts',(172.129004431022,6.79659314313001,132.490971352347));
#238727=CARTESIAN_POINT('Ctrl Pts',(171.850556807209,5.09271798834896,125.997848616637));
#238728=CARTESIAN_POINT('Ctrl Pts',(171.572109183396,-1.29111620461978,
123.921675598615));
#238729=CARTESIAN_POINT('Ctrl Pts',(171.293661559583,-6.48847768007612,
128.170353875152));
#238730=CARTESIAN_POINT('Ctrl Pts',(171.01521393577,-5.72324514729908,134.839555669585));
#238731=CARTESIAN_POINT('Ctrl Pts',(170.736766311957,0.301370079776633,
137.800610341449));
#238732=CARTESIAN_POINT('Ctrl Pts',(170.458318688145,6.04904092628448,134.332453302864));
#238733=CARTESIAN_POINT('Ctrl Pts',(170.179871064331,6.23793867361471,127.6221514434));
#238734=CARTESIAN_POINT('Ctrl Pts',(169.901423440519,0.694475520138818,
123.836144355433));
#238735=CARTESIAN_POINT('Ctrl Pts',(169.622975816706,-5.4871767093294,126.453587596077));
#238736=CARTESIAN_POINT('Ctrl Pts',(169.344528192893,-6.62638160640872,
133.06917869639));
#238737=CARTESIAN_POINT('Ctrl Pts',(169.06608056908,-1.67626552393645,137.603512624779));
#238738=CARTESIAN_POINT('Ctrl Pts',(168.787632945267,4.81425668490999,135.88975801558));
#238739=CARTESIAN_POINT('Ctrl Pts',(168.509185321454,6.88071218983824,129.50277163308));
#238740=CARTESIAN_POINT('Ctrl Pts',(168.230737697641,2.62412933378287,124.311881941165));
#238741=CARTESIAN_POINT('Ctrl Pts',(167.952290073828,-4.0439001841742,125.087262977647));
#238742=CARTESIAN_POINT('Ctrl Pts',(167.673842450016,-6.99578298838191,
131.116377449467));
#238743=CARTESIAN_POINT('Ctrl Pts',(167.395394826203,-3.51888298926545,
136.858763695638));
#238744=CARTESIAN_POINT('Ctrl Pts',(167.11694720239,3.19169856999505,137.037449287095));
#238745=CARTESIAN_POINT('Ctrl Pts',(166.838499578577,6.96926506657354,131.488230894564));
#238746=CARTESIAN_POINT('Ctrl Pts',(166.560051954764,4.34241743449723,125.310569126392));
#238747=CARTESIAN_POINT('Ctrl Pts',(166.281604330951,-2.27489968099678,
124.181433351974));
#238748=CARTESIAN_POINT('Ctrl Pts',(166.003156707138,-6.80169512468258,
129.13844418665));
#238749=CARTESIAN_POINT('Ctrl Pts',(165.724709083325,-5.0780650300646,135.626350836796));
#238750=CARTESIAN_POINT('Ctrl Pts',(165.446261459512,1.31205874991464,137.683084042787));
#238751=CARTESIAN_POINT('Ctrl Pts',(165.1678138357,6.49646463635559,133.418606465321));
#238752=CARTESIAN_POINT('Ctrl Pts',(164.889366211887,5.71093689192698,126.751764666776));
#238753=CARTESIAN_POINT('Ctrl Pts',(164.610918588074,-0.322662861405092,
123.809060566689));
#238754=CARTESIAN_POINT('Ctrl Pts',(164.332470964261,-6.05975120806294,
127.29469547395));
#238755=CARTESIAN_POINT('Ctrl Pts',(164.054023340448,-6.22822422981513,
134.00554119152));
#238756=CARTESIAN_POINT('Ctrl Pts',(163.775575716635,-0.673263450036036,
137.774658347991));
#238757=CARTESIAN_POINT('Ctrl Pts',(163.497128092822,5.50039354957815,135.138412408175));
#238758=CARTESIAN_POINT('Ctrl Pts',(163.218680469009,6.61945758629338,128.51938460299));
#238759=CARTESIAN_POINT('Ctrl Pts',(162.940232845196,1.65556347968583,124.000138127916));
#238760=CARTESIAN_POINT('Ctrl Pts',(162.661785221384,-4.82971258598073,
125.733639716082));
#238761=CARTESIAN_POINT('Ctrl Pts',(162.383337597571,-6.87671872970774,
132.126886094224));
#238762=CARTESIAN_POINT('Ctrl Pts',(162.104889973758,-2.60435630721971,
137.304796168278));
#238763=CARTESIAN_POINT('Ctrl Pts',(161.826442349945,4.06128233172446,136.509123535159));
#238764=CARTESIAN_POINT('Ctrl Pts',(161.547994726132,6.99480091248578,130.471052473933));
#238765=CARTESIAN_POINT('Ctrl Pts',(161.269547102319,3.50043916969439,124.739275313697));
#238766=CARTESIAN_POINT('Ctrl Pts',(160.991099478506,-3.21065516408591,
124.581015251828));
#238767=CARTESIAN_POINT('Ctrl Pts',(160.712651854693,-6.97131425129578,
130.141705553748));
#238768=CARTESIAN_POINT('Ctrl Pts',(160.434204230881,-4.32567610919938,
136.311343486817));
#238769=CARTESIAN_POINT('Ctrl Pts',(160.155756607067,2.29504705622523,137.420333194114));
#238770=CARTESIAN_POINT('Ctrl Pts',(159.877308983254,6.80673409626067,132.449567311792));
#238771=CARTESIAN_POINT('Ctrl Pts',(159.598861359442,5.06336502927952,125.966936850291));
#238772=CARTESIAN_POINT('Ctrl Pts',(159.320413735629,-1.33298914047637,
123.929662509627));
#238773=CARTESIAN_POINT('Ctrl Pts',(159.041966111816,-6.50439141027418,
128.209899882485));
#238774=CARTESIAN_POINT('Ctrl Pts',(158.763518488003,-5.69857573121565,
134.874319924428));
#238775=CARTESIAN_POINT('Ctrl Pts',(158.48507086419,0.343952653928878,137.798646191931));
#238776=CARTESIAN_POINT('Ctrl Pts',(158.206623240377,6.07040535313402,134.295565706438));
#238777=CARTESIAN_POINT('Ctrl Pts',(157.928175616564,6.2184520885971,127.584238299121));
#238778=CARTESIAN_POINT('Ctrl Pts',(157.649727992752,0.652045142912632,
123.832045990734));
#238779=CARTESIAN_POINT('Ctrl Pts',(157.371280368939,-5.51355943493244,
126.487070207899));
#238780=CARTESIAN_POINT('Ctrl Pts',(157.092832745126,-6.61247224442723,
133.109473400187));
#238781=CARTESIAN_POINT('Ctrl Pts',(156.814385121313,-1.63484609852131,
137.613590556265));
#238782=CARTESIAN_POINT('Ctrl Pts',(156.5359374975,4.84512374525377,135.860358048054));
#238783=CARTESIAN_POINT('Ctrl Pts',(156.257489873687,6.87266156459436,129.46091090043));
#238784=CARTESIAN_POINT('Ctrl Pts',(155.979042249874,2.58455915425555,124.296028411687));
#238785=CARTESIAN_POINT('Ctrl Pts',(155.700594626061,-4.07862685611001,
125.111985270442));
#238786=CARTESIAN_POINT('Ctrl Pts',(155.422147002248,-6.99375403770952,
131.158956985208));
#238787=CARTESIAN_POINT('Ctrl Pts',(155.143699378435,-3.48196292253304,
136.880071961106));
#238788=CARTESIAN_POINT('Ctrl Pts',(154.865251754623,3.22958201510593,137.017905027291));
#238789=CARTESIAN_POINT('Ctrl Pts',(154.58680413081,6.97329885471516,131.445794329457));
#238790=CARTESIAN_POINT('Ctrl Pts',(154.308356506997,4.30889471142897,125.284237386175));
#238791=CARTESIAN_POINT('Ctrl Pts',(154.029908883184,-2.31517317045128,
124.195404019528));
#238792=CARTESIAN_POINT('Ctrl Pts',(153.751461259371,-6.81171001118396,
129.179878900999));
#238793=CARTESIAN_POINT('Ctrl Pts',(153.473013635558,-5.04861812217248,
135.65717311965));
#238794=CARTESIAN_POINT('Ctrl Pts',(153.194566011745,1.3539071824088,137.674969721956));
#238795=CARTESIAN_POINT('Ctrl Pts',(152.916118387933,6.51225792839928,133.379012205241));
#238796=CARTESIAN_POINT('Ctrl Pts',(152.637670764119,5.68616177967723,126.717075658174));
#238797=CARTESIAN_POINT('Ctrl Pts',(152.359223140307,-0.365239260122265,
123.811154313817));
#238798=CARTESIAN_POINT('Ctrl Pts',(152.080775516494,-6.08100326279917,
127.331647925483));
#238799=CARTESIAN_POINT('Ctrl Pts',(151.802327892681,-6.20862234048841,
134.043394849727));
#238800=CARTESIAN_POINT('Ctrl Pts',(151.523880268868,-0.630820795332096,
137.778627550233));
#238801=CARTESIAN_POINT('Ctrl Pts',(151.245432645055,5.52667424342534,135.104849651499));
#238802=CARTESIAN_POINT('Ctrl Pts',(150.966985021242,6.60542564552152,128.479132421149));
#238803=CARTESIAN_POINT('Ctrl Pts',(150.688537397429,1.61411357236584,123.990186309594));
#238804=CARTESIAN_POINT('Ctrl Pts',(150.410089773616,-4.86049001996232,
125.763133496143));
#238805=CARTESIAN_POINT('Ctrl Pts',(150.131642149803,-6.8685407320831,132.168722129643));
#238806=CARTESIAN_POINT('Ctrl Pts',(149.853194525991,-2.56473805828847,
137.32052918631));
#238807=CARTESIAN_POINT('Ctrl Pts',(149.574746902178,4.09593359665354,136.484295660832));
#238808=CARTESIAN_POINT('Ctrl Pts',(149.296299278365,6.99264237375128,130.428479310845));
#238809=CARTESIAN_POINT('Ctrl Pts',(149.017851654552,3.46345441894284,124.718079518912));
#238810=CARTESIAN_POINT('Ctrl Pts',(148.739404030739,-3.24847894771935,
124.600674725279));
#238811=CARTESIAN_POINT('Ctrl Pts',(148.460956406926,-6.97521885844655,
130.184154199754));
#238812=CARTESIAN_POINT('Ctrl Pts',(148.182508783113,-4.29207339664657,
136.337573073429));
#238813=CARTESIAN_POINT('Ctrl Pts',(147.9040611593,2.33527783722936,137.406240012622));
#238814=CARTESIAN_POINT('Ctrl Pts',(147.625613535487,6.81662282335624,132.408102307496));
#238815=CARTESIAN_POINT('Ctrl Pts',(147.347165911675,5.03382444535687,125.936204336462));
#238816=CARTESIAN_POINT('Ctrl Pts',(147.068718287862,-1.37481268193005,
123.937904165105));
#238817=CARTESIAN_POINT('Ctrl Pts',(146.790270664049,-6.52006411785656,
128.249542028514));
#238818=CARTESIAN_POINT('Ctrl Pts',(146.511823040236,-5.67369515231286,
134.908933365434));
#238819=CARTESIAN_POINT('Ctrl Pts',(146.233375416423,0.386522482789046,
137.796422866589));
#238820=CARTESIAN_POINT('Ctrl Pts',(145.95492779261,6.09154483888081,134.258548742122));
#238821=CARTESIAN_POINT('Ctrl Pts',(145.676480168797,6.19873507655051,127.546444477659));
#238822=CARTESIAN_POINT('Ctrl Pts',(145.398032544984,0.609590603913882,
123.828205987717));
#238823=CARTESIAN_POINT('Ctrl Pts',(145.119584921171,-5.53973785356302,
126.520712798507));
#238824=CARTESIAN_POINT('Ctrl Pts',(144.841137297358,-6.59831785485502,
133.149682687181));
#238825=CARTESIAN_POINT('Ctrl Pts',(144.562689673546,-1.59336609328267,
137.623416169231));
#238826=CARTESIAN_POINT('Ctrl Pts',(144.284242049733,4.87581126775532,135.830770728684));
#238827=CARTESIAN_POINT('Ctrl Pts',(144.00579442592,6.86435627034879,129.419099949804));
#238828=CARTESIAN_POINT('Ctrl Pts',(143.727346802107,2.54489320293839,124.280416050852));
#238829=CARTESIAN_POINT('Ctrl Pts',(143.448899178294,-4.11320239302776,
125.136918496298));
#238830=CARTESIAN_POINT('Ctrl Pts',(143.170451554481,-6.99146593090932,
131.201523381251));
#238831=CARTESIAN_POINT('Ctrl Pts',(142.892003930668,-3.44491383038404,
136.901155088855));
#238832=CARTESIAN_POINT('Ctrl Pts',(142.613556306855,3.26734578686757,136.998130522314));
#238833=CARTESIAN_POINT('Ctrl Pts',(142.335108683042,6.97707424470332,131.403333995789));
#238834=CARTESIAN_POINT('Ctrl Pts',(142.05666105923,4.27521232068256,125.258110196154));
#238835=CARTESIAN_POINT('Ctrl Pts',(141.778213435417,-2.35536087031262,
124.209619584399));
#238836=CARTESIAN_POINT('Ctrl Pts',(141.499765811604,-6.8214724872659,129.221373811115));
#238837=CARTESIAN_POINT('Ctrl Pts',(141.221318187791,-5.01898413587917,
135.687815579753));
#238838=CARTESIAN_POINT('Ctrl Pts',(140.942870563978,1.39570544537436,137.666600808179));
#238839=CARTESIAN_POINT('Ctrl Pts',(140.664422940165,6.52780990633047,133.339322540502));
#238840=CARTESIAN_POINT('Ctrl Pts',(140.385975316352,5.66117596461176,126.68253810542));
#238841=CARTESIAN_POINT('Ctrl Pts',(140.10752769254,-0.407802124764288,
123.813507196776));
#238842=CARTESIAN_POINT('Ctrl Pts',(139.829080068726,-6.10202998372316,
127.368729059661));
#238843=CARTESIAN_POINT('Ctrl Pts',(139.550632444914,-6.18879038837768,
134.081128484328));
#238844=CARTESIAN_POINT('Ctrl Pts',(139.272184821101,-0.588354765331746,
137.78233831845));
#238845=CARTESIAN_POINT('Ctrl Pts',(138.993737197288,5.55275014432601,135.071127538621));
#238846=CARTESIAN_POINT('Ctrl Pts',(138.715289573475,6.59114893827324,128.438966401494));
#238847=CARTESIAN_POINT('Ctrl Pts',(138.436841949662,1.57260385347371,123.980486993006));
#238848=CARTESIAN_POINT('Ctrl Pts',(138.158394325849,-4.8910873466988,125.792814080728));
#238849=CARTESIAN_POINT('Ctrl Pts',(137.879946702036,-6.86010821815569,
132.210507608145));
#238850=CARTESIAN_POINT('Ctrl Pts',(137.601499078223,-2.52502477204539,
137.336020745319));
#238851=CARTESIAN_POINT('Ctrl Pts',(137.32305145441,4.13043308525698,136.459257314423));
#238852=CARTESIAN_POINT('Ctrl Pts',(137.044603830598,6.99022472008204,130.385920076178));
#238853=CARTESIAN_POINT('Ctrl Pts',(136.766156206785,3.42634132861412,124.69710925351));
#238854=CARTESIAN_POINT('Ctrl Pts',(136.487708582972,-3.28618235777073,
124.620564078594));
#238855=CARTESIAN_POINT('Ctrl Pts',(136.209260959159,-6.97886499629743,
130.226625827737));
#238856=CARTESIAN_POINT('Ctrl Pts',(135.930813335346,-4.25831163973555,
136.363597624819));
#238857=CARTESIAN_POINT('Ctrl Pts',(135.652365711533,2.37542208365453,137.391902196061));
#238858=CARTESIAN_POINT('Ctrl Pts',(135.37391808772,6.82625895798624,132.366577875963));
#238859=CARTESIAN_POINT('Ctrl Pts',(135.095470463907,5.00409733121823,125.905652213954));
#238860=CARTESIAN_POINT('Ctrl Pts',(134.817022840094,-1.4165852791943,123.946400259653));
#238861=CARTESIAN_POINT('Ctrl Pts',(134.538575216282,-6.53549522206528,
128.289278844285));
#238862=CARTESIAN_POINT('Ctrl Pts',(134.260127592469,-5.64860433254967,
134.943394709987));
#238863=CARTESIAN_POINT('Ctrl Pts',(133.981679968656,0.429077988916399,
137.793940447809));
#238864=CARTESIAN_POINT('Ctrl Pts',(133.703232344843,6.1124586001935,134.221403781595));
#238865=CARTESIAN_POINT('Ctrl Pts',(133.42478472103,6.17878836809604,127.508771379477));
#238866=CARTESIAN_POINT('Ctrl Pts',(133.146337097217,0.567113476311158,
123.824624488677));
#238867=CARTESIAN_POINT('Ctrl Pts',(132.867889473404,-5.5657109951702,126.554514121259));
#238868=CARTESIAN_POINT('Ctrl Pts',(132.589441849591,-6.58391896218814,
133.189805067404));
#238869=CARTESIAN_POINT('Ctrl Pts',(132.310994225778,-1.55182704527753,
137.632989099587));
#238870=CARTESIAN_POINT('Ctrl Pts',(132.032546601965,4.90631811527725,135.800997153839));
#238871=CARTESIAN_POINT('Ctrl Pts',(131.754098978153,6.85579661485726,129.377340330521));
#238872=CARTESIAN_POINT('Ctrl Pts',(131.47565135434,2.50513294966777,124.265045437181));
#238873=CARTESIAN_POINT('Ctrl Pts',(131.197203730527,-4.14762551371829,
125.162061731307));
#238874=CARTESIAN_POINT('Ctrl Pts',(130.918756106714,-6.98891875276791,
131.244075060281));
#238875=CARTESIAN_POINT('Ctrl Pts',(130.640308482901,-3.4077370856862,136.922012297644));
#238876=CARTESIAN_POINT('Ctrl Pts',(130.361860859088,3.30498848592948,136.978126504915));
#238877=CARTESIAN_POINT('Ctrl Pts',(130.083413235275,6.98059109663955,131.360851466943));
#238878=CARTESIAN_POINT('Ctrl Pts',(129.804965611462,4.24137151037132,125.232188524482));
#238879=CARTESIAN_POINT('Ctrl Pts',(129.526517987649,-2.39546129141071,
124.224079519825));
#238880=CARTESIAN_POINT('Ctrl Pts',(129.248070363836,-6.83098219117618,
129.262927379388));
#238881=CARTESIAN_POINT('Ctrl Pts',(128.969622740024,-4.98916416928312,
135.718277081636));
#238882=CARTESIAN_POINT('Ctrl Pts',(128.691175116211,1.43745198996158,137.657977611568));
#238883=CARTESIAN_POINT('Ctrl Pts',(128.412727492398,6.54311999386511,133.299538941816));
#238884=CARTESIAN_POINT('Ctrl Pts',(128.134279868585,5.63598037258881,126.648153288314));
#238885=CARTESIAN_POINT('Ctrl Pts',(127.855832244772,-0.450349878148651,
123.81611912838));
#238886=CARTESIAN_POINT('Ctrl Pts',(127.577384620959,-6.12283059168226,
127.40593750243));
#238887=CARTESIAN_POINT('Ctrl Pts',(127.298936997146,-6.16872910836309,
134.118740697091));
#238888=CARTESIAN_POINT('Ctrl Pts',(127.020489373333,-0.545866933628919,
137.785790515136));
#238889=CARTESIAN_POINT('Ctrl Pts',(126.742041749521,5.57862028602806,135.037247319125));
#238890=CARTESIAN_POINT('Ctrl Pts',(126.463594125708,6.57662799357718,128.398888032392));
#238891=CARTESIAN_POINT('Ctrl Pts',(126.185146501895,1.53103586116759,123.971040537565));
#238892=CARTESIAN_POINT('Ctrl Pts',(125.906698878082,-4.92150343239493,
125.822680370014));
#238893=CARTESIAN_POINT('Ctrl Pts',(125.628251254269,-6.85142150039552,
132.252240981353));
#238894=CARTESIAN_POINT('Ctrl Pts',(125.349803630456,-2.48521792008072,
137.351270271259));
#238895=CARTESIAN_POINT('Ctrl Pts',(125.071356006643,4.16477951914341,136.434009423738));
#238896=CARTESIAN_POINT('Ctrl Pts',(124.79290838283,6.98754804106521,130.343376346978));
#238897=CARTESIAN_POINT('Ctrl Pts',(124.514460759018,3.38910127394743,124.676365294554));
#238898=CARTESIAN_POINT('Ctrl Pts',(124.236013135205,-3.32376399712637,
124.640682574762));
#238899=CARTESIAN_POINT('Ctrl Pts',(123.957565511392,-6.98225252973936,
130.269118863895));
#238900=CARTESIAN_POINT('Ctrl Pts',(123.679117887579,-4.22439208952083,
136.389416176637));
#238901=CARTESIAN_POINT('Ctrl Pts',(123.400670263766,2.41547830794073,137.377320275725));
#238902=CARTESIAN_POINT('Ctrl Pts',(123.122222639953,6.83564214308024,132.324995555895));
#238903=CARTESIAN_POINT('Ctrl Pts',(122.84377501614,4.97418478841272,125.875281614887));
#238904=CARTESIAN_POINT('Ctrl Pts',(122.565327392328,-1.45830538437,123.955150478444));
#238905=CARTESIAN_POINT('Ctrl Pts',(122.286879768514,-6.55068415109515,
128.329108857337));
#238906=CARTESIAN_POINT('Ctrl Pts',(122.008432144702,-5.62330420167569,
134.977702681109));
#238907=CARTESIAN_POINT('Ctrl Pts',(121.729984520888,0.471617595401148,
137.791199027578));
#238908=CARTESIAN_POINT('Ctrl Pts',(121.451536897076,6.13314586210485,134.184132201278));
#238909=CARTESIAN_POINT('Ctrl Pts',(121.173089273263,6.15861270236637,127.471220400567));
#238910=CARTESIAN_POINT('Ctrl Pts',(120.89464164945,0.52461533410983,123.821301626325));
#238911=CARTESIAN_POINT('Ctrl Pts',(120.616194025637,-5.5914778973097,126.588472923636));
#238912=CARTESIAN_POINT('Ctrl Pts',(120.337746401824,-6.56927609998288,
133.229839054105));
#238913=CARTESIAN_POINT('Ctrl Pts',(120.059298778011,-1.51023049375061,
137.642308992603));
#238914=CARTESIAN_POINT('Ctrl Pts',(119.780851154198,4.93664315737715,135.77103842679));
#238915=CARTESIAN_POINT('Ctrl Pts',(119.502403530385,6.84698291530094,129.33563359));
#238916=CARTESIAN_POINT('Ctrl Pts',(119.223955906573,2.46527986777437,124.249917140239));
#238917=CARTESIAN_POINT('Ctrl Pts',(118.94550828276,-4.18189494262004,125.187414043775));
#238918=CARTESIAN_POINT('Ctrl Pts',(118.667060658947,-6.98611259767199,
131.28661044553));
#238919=CARTESIAN_POINT('Ctrl Pts',(118.388613035134,-3.37043406603744,
136.942642814599));
#238920=CARTESIAN_POINT('Ctrl Pts',(118.110165411321,3.34250871742766,136.95789371635));
#238921=CARTESIAN_POINT('Ctrl Pts',(117.831717787508,6.98384928020556,131.318348317123));
#238922=CARTESIAN_POINT('Ctrl Pts',(117.553270163695,4.20737353447909,125.206473331696));
#238923=CARTESIAN_POINT('Ctrl Pts',(117.274822539882,-2.43547294780967,
124.238783289987));
#238924=CARTESIAN_POINT('Ctrl Pts',(116.99637491607,-6.84023877052931,129.304538066038));
#238925=CARTESIAN_POINT('Ctrl Pts',(116.717927292256,-4.95915932737393,
135.748556496538));
#238926=CARTESIAN_POINT('Ctrl Pts',(116.439479668444,1.47914526923655,137.649100451659));
#238927=CARTESIAN_POINT('Ctrl Pts',(116.161032044631,6.55818762368211,133.259662883379));
#238928=CARTESIAN_POINT('Ctrl Pts',(115.882584420818,5.61057593724064,126.613922481));
#238929=CARTESIAN_POINT('Ctrl Pts',(115.604136797005,-0.49288094365267,
123.818990011842));
#238930=CARTESIAN_POINT('Ctrl Pts',(115.325689173192,-6.14340431590201,
127.443271875017));
#238931=CARTESIAN_POINT('Ctrl Pts',(115.047241549379,-6.14843924382291,
134.156230094282));
#238932=CARTESIAN_POINT('Ctrl Pts',(114.768793925566,-0.5033588746261,137.78898401237));
#238933=CARTESIAN_POINT('Ctrl Pts',(114.490346301753,5.60428370990391,135.003210248456));
#238934=CARTESIAN_POINT('Ctrl Pts',(114.211898677941,6.56186334951224,128.358898798961));
#238935=CARTESIAN_POINT('Ctrl Pts',(113.933451054127,1.48941113576461,123.961847293312));
#238936=CARTESIAN_POINT('Ctrl Pts',(113.655003430315,-4.95173714997151,
125.852731257293));
#238937=CARTESIAN_POINT('Ctrl Pts',(113.376555806502,-6.84248090069202,
132.293920702821));
#238938=CARTESIAN_POINT('Ctrl Pts',(113.098108182689,-2.4453189774521,137.366277199056));
#238939=CARTESIAN_POINT('Ctrl Pts',(112.819660558876,4.19897162559319,136.408552924347));
#238940=CARTESIAN_POINT('Ctrl Pts',(112.541212935063,6.98461243588604,130.300849699721));
#238941=CARTESIAN_POINT('Ctrl Pts',(112.26276531125,3.35173563488669,124.655848410718));
#238942=CARTESIAN_POINT('Ctrl Pts',(111.984317687437,-3.3612224731848,124.661029468288));
#238943=CARTESIAN_POINT('Ctrl Pts',(111.705870063624,-6.98538133324609,
130.311631733633));
#238944=CARTESIAN_POINT('Ctrl Pts',(111.427422439812,-4.1903160029037,136.415027772168));
#238945=CARTESIAN_POINT('Ctrl Pts',(111.148974815999,2.45544502578993,137.362494791951));
#238946=CARTESIAN_POINT('Ctrl Pts',(110.870527192186,6.84477203094083,132.28335688814));
#238947=CARTESIAN_POINT('Ctrl Pts',(110.592079568373,4.94408792536061,125.845093664656));
#238948=CARTESIAN_POINT('Ctrl Pts',(110.31363194456,-1.49997145150339,123.964154497236));
#238949=CARTESIAN_POINT('Ctrl Pts',(110.035184320747,-6.56563034211481,
128.369030591753));
#238950=CARTESIAN_POINT('Ctrl Pts',(109.756736696934,-5.59779569719655,
135.011856007506));
#238951=CARTESIAN_POINT('Ctrl Pts',(109.478289073121,0.514139725922464,
137.788198707481));
#238952=CARTESIAN_POINT('Ctrl Pts',(109.199841449309,6.15360585804082,134.146735382281));
#238953=CARTESIAN_POINT('Ctrl Pts',(108.921393825496,6.13820882697821,127.433792932393));
#238954=CARTESIAN_POINT('Ctrl Pts',(108.642946201683,0.482097752094529,
123.818237523792));
#238955=CARTESIAN_POINT('Ctrl Pts',(108.36449857787,-5.61703760517944,126.622587947283));
#238956=CARTESIAN_POINT('Ctrl Pts',(108.086050954057,-6.5543898108359,133.26978316381));
#238957=CARTESIAN_POINT('Ctrl Pts',(107.807603330244,-1.46857798007734,
137.651375502926));
#238958=CARTESIAN_POINT('Ctrl Pts',(107.529155706431,4.96678527034939,135.740895657668));
#238959=CARTESIAN_POINT('Ctrl Pts',(107.250708082618,6.83791549827476,129.2939812737));
#238960=CARTESIAN_POINT('Ctrl Pts',(106.972260458805,2.42533543402888,124.23503172061));
#238961=CARTESIAN_POINT('Ctrl Pts',(106.693812834992,-4.21600940986681,
125.212974494265));
#238962=CARTESIAN_POINT('Ctrl Pts',(106.415365211179,-6.98304756960462,
131.329127960835));
#238963=CARTESIAN_POINT('Ctrl Pts',(106.136917587367,-3.33300615371489,
136.96304587525));
#238964=CARTESIAN_POINT('Ctrl Pts',(105.858469963554,3.37990509103613,136.937432906355));
#238965=CARTESIAN_POINT('Ctrl Pts',(105.580022339741,6.98684867466819,131.275826121299));
#238966=CARTESIAN_POINT('Ctrl Pts',(105.301574715928,4.1732196528133,125.180965570684));
#238967=CARTESIAN_POINT('Ctrl Pts',(105.023127092115,-2.4753943568629,124.253730350031));
#238968=CARTESIAN_POINT('Ctrl Pts',(104.744679468302,-6.84924188231931,
129.346204329164));
#238969=CARTESIAN_POINT('Ctrl Pts',(104.466231844489,-4.92897072199215,
135.778652702442));
#238970=CARTESIAN_POINT('Ctrl Pts',(104.187784220676,1.52078373823962,137.639969657397));
#238971=CARTESIAN_POINT('Ctrl Pts',(103.909336596864,6.57301223744494,133.219695842813));
#238972=CARTESIAN_POINT('Ctrl Pts',(103.63088897305,5.58496359993783,126.579846951912));
#238973=CARTESIAN_POINT('Ctrl Pts',(103.352441349238,-0.535393745272065,
123.82211974078));
#238974=CARTESIAN_POINT('Ctrl Pts',(103.073993725425,-6.1637503940156,127.480730793984));
#238975=CARTESIAN_POINT('Ctrl Pts',(102.795546101612,-6.12792154660547,
134.193595286717));
#238976=CARTESIAN_POINT('Ctrl Pts',(102.517098477799,-0.460832163475232,
137.791918691816));
#238977=CARTESIAN_POINT('Ctrl Pts',(102.238650853986,5.6297394649859,134.96901758787));
#238978=CARTESIAN_POINT('Ctrl Pts',(101.960203230173,6.54685555318778,128.319000183017));
#238979=CARTESIAN_POINT('Ctrl Pts',(101.68175560636,1.44773121968427,123.952907600908));
#238980=CARTESIAN_POINT('Ctrl Pts',(101.403307982548,-4.981787379107,125.882965629019));
#238981=CARTESIAN_POINT('Ctrl Pts',(101.124860358735,-6.83328675034245,
132.335545228093));
#238982=CARTESIAN_POINT('Ctrl Pts',(100.846412734922,-2.4053294226295,137.38104097262));
#238983=CARTESIAN_POINT('Ctrl Pts',(100.567965111109,4.23300813760519,136.382888759548));
#238984=CARTESIAN_POINT('Ctrl Pts',(100.289517487296,6.98141801332452,130.258341710245));
#238985=CARTESIAN_POINT('Ctrl Pts',(100.011069863483,3.31424579602927,124.635559362262));
#238986=CARTESIAN_POINT('Ctrl Pts',(99.7326222396699,-3.39855639790849,
124.681604005209));
#238987=CARTESIAN_POINT('Ctrl Pts',(99.4541746158571,-6.98825129087862,
130.354162861621));
#238988=CARTESIAN_POINT('Ctrl Pts',(99.1757269920442,-4.15608464258612,
136.440431462363));
#238989=CARTESIAN_POINT('Ctrl Pts',(98.8972793682313,2.49532075622072,137.347426294104));
#238990=CARTESIAN_POINT('Ctrl Pts',(98.6188317444184,6.85364828325664,132.241663415635));
#238991=CARTESIAN_POINT('Ctrl Pts',(98.3403841206056,4.91380785731226,125.815089481885));
#238992=CARTESIAN_POINT('Ctrl Pts',(98.0619364967926,-1.54158193664305,
123.97341198238));
#238993=CARTESIAN_POINT('Ctrl Pts',(97.7834888729798,-6.58033324128762,
128.409042568218));
#238994=CARTESIAN_POINT('Ctrl Pts',(97.5050412491668,-5.57207976433927,
135.045853423614));
#238995=CARTESIAN_POINT('Ctrl Pts',(97.226593625354,0.55664280480716,137.784939598694));
#238996=CARTESIAN_POINT('Ctrl Pts',(96.948146001541,6.17383782984873,134.109214710358));
#238997=CARTESIAN_POINT('Ctrl Pts',(96.6696983777281,6.11757749800464,127.396490361844));
#238998=CARTESIAN_POINT('Ctrl Pts',(96.3912507539153,0.43956230576973,123.815432294619));
#238999=CARTESIAN_POINT('Ctrl Pts',(96.1128031301024,-5.64238917165504,
126.656857928054));
#239000=CARTESIAN_POINT('Ctrl Pts',(95.8343555062895,-6.53926064636413,
133.309635916377));
#239001=CARTESIAN_POINT('Ctrl Pts',(95.5559078824767,-1.42687104770695,
137.660188294596));
#239002=CARTESIAN_POINT('Ctrl Pts',(95.2774602586637,4.99674333726689,135.710569963425));
#239003=CARTESIAN_POINT('Ctrl Pts',(94.9990126348508,6.82859469977515,129.252384925061));
#239004=CARTESIAN_POINT('Ctrl Pts',(94.720565011038,2.38530112858694,124.22038972988));
#239005=CARTESIAN_POINT('Ctrl Pts',(94.442117387225,-4.24996765133445,125.238742135624));
#239006=CARTESIAN_POINT('Ctrl Pts',(94.1636697634123,-6.97972378214161,
131.371626030693));
#239007=CARTESIAN_POINT('Ctrl Pts',(93.885222139599,-3.29545473562348,136.983220723554));
#239008=CARTESIAN_POINT('Ctrl Pts',(93.6067745157866,3.41717622101856,136.91674483311));
#239009=CARTESIAN_POINT('Ctrl Pts',(93.3283268919733,6.98958916888377,131.233286455149));
#239010=CARTESIAN_POINT('Ctrl Pts',(93.0498792681607,4.13891113095855,125.155666186642));
#239011=CARTESIAN_POINT('Ctrl Pts',(92.7714316443476,-2.51522403926791,
124.268920146089));
#239012=CARTESIAN_POINT('Ctrl Pts',(92.4929840205349,-6.85799119293255,
129.387924624807));
#239013=CARTESIAN_POINT('Ctrl Pts',(92.2145363967218,-4.89859947178764,
135.808564584124));
#239014=CARTESIAN_POINT('Ctrl Pts',(91.9360887729091,1.562365854042,137.63058556713));
#239015=CARTESIAN_POINT('Ctrl Pts',(91.6576411490961,6.58759328582208,133.179639301113));
#239016=CARTESIAN_POINT('Ctrl Pts',(91.3791935252832,5.55914430975498,126.545927963732));
#239017=CARTESIAN_POINT('Ctrl Pts',(91.1007459014705,-0.57788670767935,
123.825508199223));
#239018=CARTESIAN_POINT('Ctrl Pts',(90.8222982776573,-6.18386807209161,
127.518312871276));
#239019=CARTESIAN_POINT('Ctrl Pts',(90.5438506538447,-6.10717677700159,
134.230834889814));
#239020=CARTESIAN_POINT('Ctrl Pts',(90.2654030300316,-0.41828837601907,
137.794594444728));
#239021=CARTESIAN_POINT('Ctrl Pts',(89.9869554062187,5.65498660800168,134.934670604388));
#239022=CARTESIAN_POINT('Ctrl Pts',(89.708507782406,6.53160516072318,128.279193663018));
#239023=CARTESIAN_POINT('Ctrl Pts',(89.430060158593,1.40599765739116,123.944221791613));
#239024=CARTESIAN_POINT('Ctrl Pts',(89.1516125347801,-5.01165300627911,
125.913382364846));
#239025=CARTESIAN_POINT('Ctrl Pts',(88.8731649109673,-6.82383939003939,
132.377113014756));
#239026=CARTESIAN_POINT('Ctrl Pts',(88.5947172871542,-2.36525073744058,
137.395561044874));
#239027=CARTESIAN_POINT('Ctrl Pts',(88.3162696633415,4.26688779394398,136.357017880338));
#239028=CARTESIAN_POINT('Ctrl Pts',(88.0378220395285,6.97796489175107,130.2158539537));
#239029=CARTESIAN_POINT('Ctrl Pts',(87.7593744157156,3.2766331465752,124.615498901007));
#239030=CARTESIAN_POINT('Ctrl Pts',(87.4809267919028,-3.43576438787495,
124.702405423128));
#239031=CARTESIAN_POINT('Ctrl Pts',(87.2024791680898,-6.99086229628967,
130.396710671853));
#239032=CARTESIAN_POINT('Ctrl Pts',(86.924031544277,-4.1216992770237,136.465626305881));
#239033=CARTESIAN_POINT('Ctrl Pts',(86.6455839204641,2.53510402162323,137.332115340552));
#239034=CARTESIAN_POINT('Ctrl Pts',(86.3671362966513,6.8622705711149,132.199916683345));
#239035=CARTESIAN_POINT('Ctrl Pts',(86.0886886728382,4.88334570630671,125.785270178391));
#239036=CARTESIAN_POINT('Ctrl Pts',(85.8102410490255,-1.58313529789712,
123.982922590838));
#239037=CARTESIAN_POINT('Ctrl Pts',(85.5317934252125,-6.59479230379227,
128.449143304076));
#239038=CARTESIAN_POINT('Ctrl Pts',(85.2533458013996,-5.5461573560172,135.079693669646));
#239039=CARTESIAN_POINT('Ctrl Pts',(84.9748981775869,0.599125257088023,
137.781421821987));
#239040=CARTESIAN_POINT('Ctrl Pts',(84.6964505537737,6.19384102782544,134.071571575853));
#239041=CARTESIAN_POINT('Ctrl Pts',(84.418002929961,6.09671947994716,127.359314071181));
#239042=CARTESIAN_POINT('Ctrl Pts',(84.1395553061481,0.397010571302045,
123.812886042756));
#239043=CARTESIAN_POINT('Ctrl Pts',(83.8611076823352,-5.66753165732491,
126.691281596061));
#239044=CARTESIAN_POINT('Ctrl Pts',(83.5826600585222,-6.52388916718428,
133.349395835046));
#239045=CARTESIAN_POINT('Ctrl Pts',(83.3042124347095,-1.38511124210516,
137.66874704105));
#239046=CARTESIAN_POINT('Ctrl Pts',(83.0257648108964,5.02651624802251,135.68006246779));
#239047=CARTESIAN_POINT('Ctrl Pts',(82.7473171870836,6.81902086518772,129.210846085452));
#239048=CARTESIAN_POINT('Ctrl Pts',(82.4688695632707,2.34517843493451,124.205991710613));
#239049=CARTESIAN_POINT('Ctrl Pts',(82.1904219394578,-4.28376840868787,
125.264716013022));
#239050=CARTESIAN_POINT('Ctrl Pts',(81.9119743156449,-6.97614135844701,
131.414103080323));
#239051=CARTESIAN_POINT('Ctrl Pts',(81.6335266918322,-3.25778120324508,
137.003166611925));
#239052=CARTESIAN_POINT('Ctrl Pts',(81.355079068019,3.45432072627939,136.895830263219));
#239053=CARTESIAN_POINT('Ctrl Pts',(81.0766314442065,6.99207066130227,131.190730894994));
#239054=CARTESIAN_POINT('Ctrl Pts',(80.7981838203932,4.10444924022979,125.130576117049));
#239055=CARTESIAN_POINT('Ctrl Pts',(80.5197361965806,-2.55496051912119,
124.284352115297));
#239056=CARTESIAN_POINT('Ctrl Pts',(80.2412885727675,-6.86648637816013,
129.429697407007));
#239057=CARTESIAN_POINT('Ctrl Pts',(79.9628409489547,-4.86804670217826,
135.838291033188));
#239058=CARTESIAN_POINT('Ctrl Pts',(79.6843933251418,1.6038900758031,137.620948528586));
#239059=CARTESIAN_POINT('Ctrl Pts',(79.405945701329,6.60193022850756,133.139494742587));
#239060=CARTESIAN_POINT('Ctrl Pts',(79.1274980775159,5.53311902343524,126.512166773338));
#239061=CARTESIAN_POINT('Ctrl Pts',(78.8490504537032,-0.620358256282274,
123.829155261608));
#239062=CARTESIAN_POINT('Ctrl Pts',(78.5706028298902,-6.2037566046621,127.556016714277));
#239063=CARTESIAN_POINT('Ctrl Pts',(78.2921552060774,-6.08620570371632,
134.267947523646));
#239064=CARTESIAN_POINT('Ctrl Pts',(78.0137075822645,-0.375729088733312,
137.797011171955));
#239065=CARTESIAN_POINT('Ctrl Pts',(77.7352599584516,5.68002420340909,134.90017057075));
#239066=CARTESIAN_POINT('Ctrl Pts',(77.4568123346387,6.51611273722737,128.23948071401));
#239067=CARTESIAN_POINT('Ctrl Pts',(77.1783647108257,1.36421199533782,123.935790187287));
#239068=CARTESIAN_POINT('Ctrl Pts',(76.8999170870129,-5.04133292480603,
125.94398033767));
#239069=CARTESIAN_POINT('Ctrl Pts',(76.6214694632,-6.81413916985829,132.418622522501));
#239070=CARTESIAN_POINT('Ctrl Pts',(76.3430218393871,-2.32508440701577,
137.409836877774));
#239071=CARTESIAN_POINT('Ctrl Pts',(76.0645742155741,4.30060933918641,136.33094124537));
#239072=CARTESIAN_POINT('Ctrl Pts',(75.7861265917614,6.97425319912241,130.173388004487));
#239073=CARTESIAN_POINT('Ctrl Pts',(75.5076789679483,3.23889908027492,124.595667770297));
#239074=CARTESIAN_POINT('Ctrl Pts',(75.2292313441357,-3.47284506432852,
124.72343295124));
#239075=CARTESIAN_POINT('Ctrl Pts',(74.9507837203226,-6.99321425272744,
130.439273587703));
#239076=CARTESIAN_POINT('Ctrl Pts',(74.6723360965098,-4.08716118037883,
136.490611369118));
#239077=CARTESIAN_POINT('Ctrl Pts',(74.3938884726969,2.57479334781394,137.316562498648));
#239078=CARTESIAN_POINT('Ctrl Pts',(74.1154408488841,6.87063857501356,132.158118238212));
#239079=CARTESIAN_POINT('Ctrl Pts',(73.836993225071,4.85270260113016,125.755636859138));
#239080=CARTESIAN_POINT('Ctrl Pts',(73.5585456012583,-1.62462999549052,
123.992685970191));
#239081=CARTESIAN_POINT('Ctrl Pts',(73.2800979774453,-6.60900699384299,
128.489331313375));
#239082=CARTESIAN_POINT('Ctrl Pts',(73.0016503536324,-5.52002943279461,
135.113375491641));
#239083=CARTESIAN_POINT('Ctrl Pts',(72.7232027298196,0.641585508562261,
137.777645507711));
#239084=CARTESIAN_POINT('Ctrl Pts',(72.4447551060067,6.21361471074508,134.033807373642));
#239085=CARTESIAN_POINT('Ctrl Pts',(72.1663074821937,6.07563554570727,127.322265437984));
#239086=CARTESIAN_POINT('Ctrl Pts',(71.8878598583809,0.354444125461637,
123.810598862555));
#239087=CARTESIAN_POINT('Ctrl Pts',(71.609412234568,-5.69246413052499,126.725857675724));
#239088=CARTESIAN_POINT('Ctrl Pts',(71.330964610755,-6.5082759428922,133.3890614465));
#239089=CARTESIAN_POINT('Ctrl Pts',(71.0525169869423,-1.34330011069692,
137.677051425141));
#239090=CARTESIAN_POINT('Ctrl Pts',(70.7740693631292,5.05610289937005,135.649374301231));
#239091=CARTESIAN_POINT('Ctrl Pts',(70.4956217393166,6.80919434927445,129.16936629411));
#239092=CARTESIAN_POINT('Ctrl Pts',(70.2171741155033,2.30496883983272,124.191838196331));
#239093=CARTESIAN_POINT('Ctrl Pts',(69.9387264916908,-4.31741042942741,
125.290895163988));
#239094=CARTESIAN_POINT('Ctrl Pts',(69.6602788678776,-6.97230043126892,
131.456557535721));
#239095=CARTESIAN_POINT('Ctrl Pts',(69.3818312440649,-3.21998695258627,
137.02288280126));
#239096=CARTESIAN_POINT('Ctrl Pts',(69.1033836202519,3.49133723041524,136.874689971681));
#239097=CARTESIAN_POINT('Ctrl Pts',(68.8249359964391,6.9942930599711,131.148161017746));
#239098=CARTESIAN_POINT('Ctrl Pts',(68.5464883726262,4.0698352576252,125.105696291628));
#239099=CARTESIAN_POINT('Ctrl Pts',(68.2680407488133,-2.59460232397255,
124.300025685817));
#239100=CARTESIAN_POINT('Ctrl Pts',(67.9895931250004,-6.87472712320984,
129.471521127857));
#239101=CARTESIAN_POINT('Ctrl Pts',(67.7111455011875,-4.83731354530826,
135.867830948109));
#239102=CARTESIAN_POINT('Ctrl Pts',(67.4326978773747,1.64535486482719,137.61105889887));
#239103=CARTESIAN_POINT('Ctrl Pts',(67.1542502535617,6.61602253424027,133.099263654809));
#239104=CARTESIAN_POINT('Ctrl Pts',(66.8758026297489,5.50688870535577,126.478564631767));
#239105=CARTESIAN_POINT('Ctrl Pts',(66.5973550059358,-0.662806817281494,
123.833060792792));
#239106=CARTESIAN_POINT('Ctrl Pts',(66.3189073821232,-6.22341525475008,
127.593840925854));
#239107=CARTESIAN_POINT('Ctrl Pts',(66.0404597583101,-6.0650091038406,134.304931812993));
#239108=CARTESIAN_POINT('Ctrl Pts',(65.7620121344974,-0.333155878668442,
137.799168783944));
#239109=CARTESIAN_POINT('Ctrl Pts',(65.4835645106842,5.70485132343066,134.865518765369));
#239110=CARTESIAN_POINT('Ctrl Pts',(65.2051168868716,6.50037885677781,128.199862807569));
#239111=CARTESIAN_POINT('Ctrl Pts',(64.9266692630585,1.32237578190785,123.927613100363));
#239112=CARTESIAN_POINT('Ctrl Pts',(64.6482216392459,-5.07082603488719,
125.974758413674));
#239113=CARTESIAN_POINT('Ctrl Pts',(64.3697740154327,-6.80418644924447,
132.460072213177));
#239114=CARTESIAN_POINT('Ctrl Pts',(64.09132639162,-2.28483191973344,137.423867942321));
#239115=CARTESIAN_POINT('Ctrl Pts',(63.812878767807,4.33417152376786,136.304659820925));
#239116=CARTESIAN_POINT('Ctrl Pts',(63.5344311439942,6.97028307297671,130.130945436197));
#239117=CARTESIAN_POINT('Ctrl Pts',(63.2559835201813,3.20104499537862,124.576066704985));
#239118=CARTESIAN_POINT('Ctrl Pts',(62.9775358963684,-3.5097970532309,124.744685810362));
#239119=CARTESIAN_POINT('Ctrl Pts',(62.6990882725555,-6.9953070730393,130.481850031987));
#239120=CARTESIAN_POINT('Ctrl Pts',(62.4206406487427,-4.05247163247362,
136.51538572624));
#239121=CARTESIAN_POINT('Ctrl Pts',(62.1421930249296,2.61438726408988,137.300768344709));
#239122=CARTESIAN_POINT('Ctrl Pts',(61.8637454011169,6.87875198487314,132.116269629093));
#239123=CARTESIAN_POINT('Ctrl Pts',(61.5852977773038,4.82187967727427,125.726190622201));
#239124=CARTESIAN_POINT('Ctrl Pts',(61.3068501534911,-1.66606449182178,
124.002701758653));
#239125=CARTESIAN_POINT('Ctrl Pts',(61.0284025296781,-6.62297678470872,
128.529605106938));
#239126=CARTESIAN_POINT('Ctrl Pts',(60.7499549058653,-5.49369696285183,
135.146897641504));
#239127=CARTESIAN_POINT('Ctrl Pts',(60.4715072820523,0.684021985849089,
137.773610795799));
#239128=CARTESIAN_POINT('Ctrl Pts',(60.1930596582395,6.23315814588628,133.995923503096));
#239129=CARTESIAN_POINT('Ctrl Pts',(59.9146120344266,6.05432647655821,127.285345835106));
#239130=CARTESIAN_POINT('Ctrl Pts',(59.6361644106137,0.311864545564345,
123.808570838767));
#239131=CARTESIAN_POINT('Ctrl Pts',(59.3577167868007,-5.71718566737322,
126.760584885814));
#239132=CARTESIAN_POINT('Ctrl Pts',(59.0792691629879,-6.49242155204172,
133.428631280914));
#239133=CARTESIAN_POINT('Ctrl Pts',(58.800821539175,-1.30143920280946,137.685101139145));
#239134=CARTESIAN_POINT('Ctrl Pts',(58.5223739153621,5.08550219496502,135.618506600908));
#239135=CARTESIAN_POINT('Ctrl Pts',(58.2439262915492,6.79911551616065,129.127947088084));
#239136=CARTESIAN_POINT('Ctrl Pts',(57.9654786677363,2.26467383326308,124.1779297115));
#239137=CARTESIAN_POINT('Ctrl Pts',(57.6870310439234,-4.35089246693584,
125.317278618444));
#239138=CARTESIAN_POINT('Ctrl Pts',(57.4085834201106,-6.96820114293417,
131.498987823723));
#239139=CARTESIAN_POINT('Ctrl Pts',(57.1301357962976,-3.18207338412696,
137.042368560968));
#239140=CARTESIAN_POINT('Ctrl Pts',(56.8516881724848,3.52822436176609,136.853324741857));
#239141=CARTESIAN_POINT('Ctrl Pts',(56.5732405486719,6.9962562825383,131.105578400848));
#239142=CARTESIAN_POINT('Ctrl Pts',(56.294792924859,4.03507046577855,125.081027632309));
#239143=CARTESIAN_POINT('Ctrl Pts',(56.0163453010462,-2.63414798488075,
124.315940276861));
#239144=CARTESIAN_POINT('Ctrl Pts',(55.7378976772331,-6.8827131227178,129.513394237565));
#239145=CARTESIAN_POINT('Ctrl Pts',(55.4594500534204,-4.80640114000575,
135.897183234276));
#239146=CARTESIAN_POINT('Ctrl Pts',(55.1810024296073,1.68675868462211,137.600917044446));
#239147=CARTESIAN_POINT('Ctrl Pts',(54.9025548057946,6.62986968082513,133.058947528554));
#239148=CARTESIAN_POINT('Ctrl Pts',(54.6241071819816,5.4804543274898,126.445122784157));
#239149=CARTESIAN_POINT('Ctrl Pts',(54.3456595581689,-0.705230817730614,
123.837224648055));
#239150=CARTESIAN_POINT('Ctrl Pts',(54.0672119343557,-6.24284329389726,
127.63178410442));
#239151=CARTESIAN_POINT('Ctrl Pts',(53.7887643105431,-6.04358776282204,
134.341786387386));
#239152=CARTESIAN_POINT('Ctrl Pts',(53.51031668673,-0.290570323389535,137.801067200743));
#239153=CARTESIAN_POINT('Ctrl Pts',(53.2318690629172,5.72946704808866,134.830716472279));
#239154=CARTESIAN_POINT('Ctrl Pts',(52.9534214391043,6.48440410239917,128.160341411752));
#239155=CARTESIAN_POINT('Ctrl Pts',(52.6749738152913,1.28049056735643,123.919690833848));
#239156=CARTESIAN_POINT('Ctrl Pts',(52.3965261914786,-5.10013124364513,
126.005715452363));
#239157=CARTESIAN_POINT('Ctrl Pts',(52.1180785676656,-6.79398159699943,
132.501460550851));
#239158=CARTESIAN_POINT('Ctrl Pts',(51.8396309438527,-2.24449476716385,
137.43765371859));
#239159=CARTESIAN_POINT('Ctrl Pts',(51.5611833200399,4.36757310402998,136.278174580871));
#239160=CARTESIAN_POINT('Ctrl Pts',(51.2827356962269,6.96605466042841,130.088527821552));
#239161=CARTESIAN_POINT('Ctrl Pts',(51.0042880724141,3.16307229458231,124.556696431394));
#239162=CARTESIAN_POINT('Ctrl Pts',(50.7258404486012,-3.54661898531293,
124.766163212963));
#239163=CARTESIAN_POINT('Ctrl Pts',(50.4473928247883,-6.99714067967511,
130.52443842702));
#239164=CARTESIAN_POINT('Ctrl Pts',(50.1689452009753,-4.0176319187415,136.539948459229));
#239165=CARTESIAN_POINT('Ctrl Pts',(49.8904975771625,2.65388430328469,137.284733463992));
#239166=CARTESIAN_POINT('Ctrl Pts',(49.6120499533496,6.88661050004828,132.074372406703));
#239167=CARTESIAN_POINT('Ctrl Pts',(49.3336023295367,4.79087807689359,125.696932558722));
#239168=CARTESIAN_POINT('Ctrl Pts',(49.0551547057238,-1.7074372515208,124.012969585086));
#239169=CARTESIAN_POINT('Ctrl Pts',(48.776707081911,-6.63670115873435,128.569963192402));
#239170=CARTESIAN_POINT('Ctrl Pts',(48.498259458098,-5.46716092194746,135.180258877061));
#239171=CARTESIAN_POINT('Ctrl Pts',(48.2198118342852,0.72643311645002,137.769317835757));
#239172=CARTESIAN_POINT('Ctrl Pts',(47.9413642104722,6.25247060906043,133.957921368012));
#239173=CARTESIAN_POINT('Ctrl Pts',(47.6629165866595,6.03279306211481,127.248556630613));
#239174=CARTESIAN_POINT('Ctrl Pts',(47.3844689628464,0.269273409411107,
123.806802046542));
#239175=CARTESIAN_POINT('Ctrl Pts',(47.1060213390337,-5.74169535180415,
126.7954619395));
#239176=CARTESIAN_POINT('Ctrl Pts',(46.8275737152206,-6.47632658212296,
133.468103872012));
#239177=CARTESIAN_POINT('Ctrl Pts',(46.5491260914079,-1.25953006961336,
137.69289588478));
#239178=CARTESIAN_POINT('Ctrl Pts',(46.2706784675948,5.11471304540623,135.587460510634));
#239179=CARTESIAN_POINT('Ctrl Pts',(45.9922308437821,6.78878473932087,129.086590002178));
#239180=CARTESIAN_POINT('Ctrl Pts',(45.7137832199691,2.22429490837156,124.164266771503));
#239181=CARTESIAN_POINT('Ctrl Pts',(45.4353355961562,-4.38421328052394,
125.343865398741));
#239182=CARTESIAN_POINT('Ctrl Pts',(45.1568879723434,-6.96384364534361,
131.541392372057));
#239183=CARTESIAN_POINT('Ctrl Pts',(44.8784403485304,-3.1440419027679,137.061623168999));
#239184=CARTESIAN_POINT('Ctrl Pts',(44.5999927247176,3.56498075346585,136.831735365442));
#239185=CARTESIAN_POINT('Ctrl Pts',(44.3215451009046,6.99796025625624,131.062984622213));
#239186=CARTESIAN_POINT('Ctrl Pts',(44.0430974770918,4.00015615291162,125.056571053198));
#239187=CARTESIAN_POINT('Ctrl Pts',(43.7646498532789,-2.67359603646683,
124.332095298706));
#239188=CARTESIAN_POINT('Ctrl Pts',(43.486202229466,-6.8904440807599,129.555315184507));
#239189=CARTESIAN_POINT('Ctrl Pts',(43.2077546056531,-4.77531063174146,
135.926346804027));
#239190=CARTESIAN_POINT('Ctrl Pts',(42.9293069818402,1.72810000095366,137.590523341125));
#239191=CARTESIAN_POINT('Ctrl Pts',(42.6508593580274,6.64347115515083,133.018547857752));
#239192=CARTESIAN_POINT('Ctrl Pts',(42.3724117342144,5.4538168693733,126.411842469708));
#239193=CARTESIAN_POINT('Ctrl Pts',(42.0939641104015,-0.74762868559244,
123.841646673103));
#239194=CARTESIAN_POINT('Ctrl Pts',(41.8155164865887,-6.26204000219037,
127.669844843974));
#239195=CARTESIAN_POINT('Ctrl Pts',(41.5370688627757,-6.02194247443641,
134.378509881167));
#239196=CARTESIAN_POINT('Ctrl Pts',(41.2586212389629,-0.247974000920424,
137.802706352008));
#239197=CARTESIAN_POINT('Ctrl Pts',(40.9801736151499,5.75387046523817,134.795764981093));
#239198=CARTESIAN_POINT('Ctrl Pts',(40.7017259913371,6.46818906604193,128.120917991039));
#239199=CARTESIAN_POINT('Ctrl Pts',(40.4232783675241,1.23855790375582,123.912023681303));
#239200=CARTESIAN_POINT('Ctrl Pts',(40.1448307437113,-5.12924746516435,
126.036850306614));
#239201=CARTESIAN_POINT('Ctrl Pts',(39.8663831198984,-6.78352499126783,
132.542786001862));
#239202=CARTESIAN_POINT('Ctrl Pts',(39.5879354960856,-2.20407444401526,
137.451193695743));
#239203=CARTESIAN_POINT('Ctrl Pts',(39.3094878722726,4.40081284226458,136.251486506627));
#239204=CARTESIAN_POINT('Ctrl Pts',(39.0310402484598,6.96156811816289,130.046136732356));
#239205=CARTESIAN_POINT('Ctrl Pts',(38.7525926246468,3.12498238497894,124.537557667297));
#239206=CARTESIAN_POINT('Ctrl Pts',(38.474145000834,-3.58330949612422,124.78786436319));
#239207=CARTESIAN_POINT('Ctrl Pts',(38.195697377021,-6.9987150046898,130.567037194673));
#239208=CARTESIAN_POINT('Ctrl Pts',(37.9172497532082,-3.98264333018119,
136.564298657899));
#239209=CARTESIAN_POINT('Ctrl Pts',(37.6388021293952,2.69328300182069,137.268458450676));
#239210=CARTESIAN_POINT('Ctrl Pts',(37.3603545055824,6.89421382933879,132.032428123559));
#239211=CARTESIAN_POINT('Ctrl Pts',(37.0819068817695,4.7596989487639,125.667863752866));
#239212=CARTESIAN_POINT('Ctrl Pts',(36.8034592579566,-1.74874674150458,
124.02348906901));
#239213=CARTESIAN_POINT('Ctrl Pts',(36.5250116341437,-6.65017960735793,
128.610404074285));
#239214=CARTESIAN_POINT('Ctrl Pts',(36.2465640103308,-5.44042229338459,
135.213457962098));
#239215=CARTESIAN_POINT('Ctrl Pts',(35.968116386518,0.768817328804687,137.764766786667));
#239216=CARTESIAN_POINT('Ctrl Pts',(35.689668762705,6.27155138463682,133.919802376575));
#239217=CARTESIAN_POINT('Ctrl Pts',(35.4112211388921,6.01103610030595,127.211899187745));
#239218=CARTESIAN_POINT('Ctrl Pts',(35.1327735150793,0.226672295232647,
123.805292551423));
#239219=CARTESIAN_POINT('Ctrl Pts',(34.8543258912663,-5.76599227560232,
126.830487544402));
#239220=CARTESIAN_POINT('Ctrl Pts',(34.5758782674535,-6.45999162954105,
133.507477757125));
#239221=CARTESIAN_POINT('Ctrl Pts',(34.2974306436406,-1.21757426406734,
137.700435373207));
#239222=CARTESIAN_POINT('Ctrl Pts',(34.0189830198277,5.1437343682746,135.556237180835));
#239223=CARTESIAN_POINT('Ctrl Pts',(33.7405353960148,6.778202401566,129.045296568894));
#239224=CARTESIAN_POINT('Ctrl Pts',(33.4620877722019,2.18383356141425,124.150849882625));
#239225=CARTESIAN_POINT('Ctrl Pts',(33.1836401483891,-4.41737163547663,
125.370654519698));
#239226=CARTESIAN_POINT('Ctrl Pts',(32.9051925245761,-6.95922809996586,
131.58376960941));
#239227=CARTESIAN_POINT('Ctrl Pts',(32.6267449007632,-3.10589391777991,
137.080645911863));
#239228=CARTESIAN_POINT('Ctrl Pts',(32.3482972769504,3.60160504349277,136.80992264244));
#239229=CARTESIAN_POINT('Ctrl Pts',(32.0698496531375,6.99940491798352,131.020381260171));
#239230=CARTESIAN_POINT('Ctrl Pts',(31.7914020293246,3.96509361278713,125.032327460544));
#239231=CARTESIAN_POINT('Ctrl Pts',(31.5129544055117,-2.71294501696876,
124.348490152723));
#239232=CARTESIAN_POINT('Ctrl Pts',(31.2345067816988,-6.89791971086261,
129.597282415287));
#239233=CARTESIAN_POINT('Ctrl Pts',(30.9560591578859,-4.74404317258561,
135.955320576696));
#239234=CARTESIAN_POINT('Ctrl Pts',(30.677611534073,1.76937728190418,137.579878174048));
#239235=CARTESIAN_POINT('Ctrl Pts',(30.3991639102601,6.65682645320975,132.978066139427));
#239236=CARTESIAN_POINT('Ctrl Pts',(30.1207162864473,5.42697731806706,126.378724921634));
#239237=CARTESIAN_POINT('Ctrl Pts',(29.8422686626343,-0.789998849798377,
123.846326704078));
#239238=CARTESIAN_POINT('Ctrl Pts',(29.5638210388214,-6.28100466828836,
127.708021734164));
#239239=CARTESIAN_POINT('Ctrl Pts',(29.2853734150086,-6.00007404075783,
134.415100933532));
#239240=CARTESIAN_POINT('Ctrl Pts',(29.0069257911957,-0.205368489683527,
137.804086176998));
#239241=CARTESIAN_POINT('Ctrl Pts',(28.7284781673828,5.77806067060162,134.760665586949));
#239242=CARTESIAN_POINT('Ctrl Pts',(28.4500305435699,6.45173434856014,128.08159400628));
#239243=CARTESIAN_POINT('Ctrl Pts',(28.171582919757,1.19657934493693,123.904611926838));
#239244=CARTESIAN_POINT('Ctrl Pts',(27.8931352959441,-5.15817362053239,
126.068161822712));
#239245=CARTESIAN_POINT('Ctrl Pts',(27.6146876721312,-6.77281701952304,
132.584047034882));
#239246=CARTESIAN_POINT('Ctrl Pts',(27.3362400483183,-2.16357244807759,
137.464487372053));
#239247=CARTESIAN_POINT('Ctrl Pts',(27.0577924245054,4.4338895067609,136.22459658713));
#239248=CARTESIAN_POINT('Ctrl Pts',(26.7793448006925,6.95682361243065,130.003773739425));
#239249=CARTESIAN_POINT('Ctrl Pts',(26.5008971768797,3.08677667800406,124.518651121888));
#239250=CARTESIAN_POINT('Ctrl Pts',(26.2224495530668,-3.61986722608435,
124.809788456898));
#239251=CARTESIAN_POINT('Ctrl Pts',(25.9440019292538,-7.00002998974624,
130.609644756432));
#239252=CARTESIAN_POINT('Ctrl Pts',(25.665554305441,-3.94750716330764,136.588435419948));
#239253=CARTESIAN_POINT('Ctrl Pts',(25.3871066816281,2.7325818997646,137.251943907838));
#239254=CARTESIAN_POINT('Ctrl Pts',(25.1086590578152,6.90156169100052,131.990438333922));
#239255=CARTESIAN_POINT('Ctrl Pts',(24.8302114340022,4.72834344823931,125.638985281792));
#239256=CARTESIAN_POINT('Ctrl Pts',(24.5517638101894,-1.78999143103474,
124.034259820624));
#239257=CARTESIAN_POINT('Ctrl Pts',(24.2733161863765,-6.66341163113055,
128.650926254035));
#239258=CARTESIAN_POINT('Ctrl Pts',(23.9948685625636,-5.41348206797292,
135.246493666413));
#239259=CARTESIAN_POINT('Ctrl Pts',(23.7164209387507,0.811173052350488,
137.759957817164));
#239260=CARTESIAN_POINT('Ctrl Pts',(23.4379733149379,6.29039976557031,133.881567941299));
#239261=CARTESIAN_POINT('Ctrl Pts',(23.159525691125,5.98905639734383,127.175374864857));
#239262=CARTESIAN_POINT('Ctrl Pts',(22.8810780673121,0.184062781628937,
123.804042409345));
#239263=CARTESIAN_POINT('Ctrl Pts',(22.6026304434992,-5.79007553843628,
126.865660402631));
#239264=CARTESIAN_POINT('Ctrl Pts',(22.3241828196863,-6.44341729959363,
133.546751477239));
#239265=CARTESIAN_POINT('Ctrl Pts',(22.0457351958734,-1.17557334085921,
137.707719325048));
#239266=CARTESIAN_POINT('Ctrl Pts',(21.7672875720605,5.17256508817436,135.524837768503));
#239267=CARTESIAN_POINT('Ctrl Pts',(21.4888399482477,6.76736889502847,129.004068318375));
#239268=CARTESIAN_POINT('Ctrl Pts',(21.2103923244347,2.14329129170119,124.137679542035));
#239269=CARTESIAN_POINT('Ctrl Pts',(20.9319447006219,-4.45036630309889,
125.397644988631));
#239270=CARTESIAN_POINT('Ctrl Pts',(20.6534970768089,-6.95435467783159,
131.626117965476));
#239271=CARTESIAN_POINT('Ctrl Pts',(20.3750494529961,-3.06763084275059,
137.099436084669));
#239272=CARTESIAN_POINT('Ctrl Pts',(20.0966018291831,3.6380958747203,136.787887381128));
#239273=CARTESIAN_POINT('Ctrl Pts',(19.8181542053702,7.00059021418742,130.977769893405));
#239274=CARTESIAN_POINT('Ctrl Pts',(19.5397065815574,3.92988414466092,125.0082977527));
#239275=CARTESIAN_POINT('Ctrl Pts',(19.2612589577445,-2.75219346829522,
124.365124231394));
#239276=CARTESIAN_POINT('Ctrl Pts',(18.9828113339316,-6.90513973601376,
129.639294374793));
#239277=CARTESIAN_POINT('Ctrl Pts',(18.7043637101187,-4.71259992116536,
135.98410347865));
#239278=CARTESIAN_POINT('Ctrl Pts',(18.4259160863058,1.81058899792882,137.568981937677));
#239279=CARTESIAN_POINT('Ctrl Pts',(18.1474684624929,6.6699350801164,132.937503873645));
#239280=CARTESIAN_POINT('Ctrl Pts',(17.86902083868,5.39993666812053,126.345771367118));
#239281=CARTESIAN_POINT('Ctrl Pts',(17.5905732148672,-0.832339740306418,
123.851264567558));
#239282=CARTESIAN_POINT('Ctrl Pts',(17.3121255910542,-6.29973658944851,
127.746313360329));
#239283=CARTESIAN_POINT('Ctrl Pts',(17.0336779672413,-5.97798327212915,
134.451558188587));
#239284=CARTESIAN_POINT('Ctrl Pts',(16.7552303434285,-0.162755368441711,
137.805206624583));
#239285=CARTESIAN_POINT('Ctrl Pts',(16.4767827196156,5.80203676780203,134.72541959047));
#239286=CARTESIAN_POINT('Ctrl Pts',(16.1983350958026,6.43504055968944,128.042370914639));
#239287=CARTESIAN_POINT('Ctrl Pts',(15.9198874719898,1.15455644643036,123.897455845098));
#239288=CARTESIAN_POINT('Ctrl Pts',(15.6414398481769,-5.18690863788001,
126.0996488404));
#239289=CARTESIAN_POINT('Ctrl Pts',(15.362992224364,-6.7618580785529,132.625242120967));
#239290=CARTESIAN_POINT('Ctrl Pts',(15.0845446005511,-2.12299028016722,
137.477534254917));
#239291=CARTESIAN_POINT('Ctrl Pts',(14.8060969767383,4.466801871851,136.197505818795));
#239292=CARTESIAN_POINT('Ctrl Pts',(14.5276493529253,6.95182131904109,129.961440412534));
#239293=CARTESIAN_POINT('Ctrl Pts',(14.2492017291125,3.04845658938423,124.499977495755));
#239294=CARTESIAN_POINT('Ctrl Pts',(13.9707541052995,-3.65629082053323,
124.831934681683));
#239295=CARTESIAN_POINT('Ctrl Pts',(13.6923064814867,-7.00108558611715,
130.652259533458));
#239296=CARTESIAN_POINT('Ctrl Pts',(13.4138588576738,-3.91222472010448,
136.612357850978));
#239297=CARTESIAN_POINT('Ctrl Pts',(13.1354112338608,2.77177954088132,137.23519044743));
#239298=CARTESIAN_POINT('Ctrl Pts',(12.856963610048,6.90865381275575,131.94840459374));
#239299=CARTESIAN_POINT('Ctrl Pts',(12.5785159862351,4.6968127372094,125.6102982156));
#239300=CARTESIAN_POINT('Ctrl Pts',(12.3000683624222,-1.83116979177416,
124.045281440813));
#239301=CARTESIAN_POINT('Ctrl Pts',(12.0216207386093,-6.67639673973472,
128.691528230086));
#239302=CARTESIAN_POINT('Ctrl Pts',(11.7431731147965,-5.38634124399241,
135.279364765853));
#239303=CARTESIAN_POINT('Ctrl Pts',(11.4647254909835,0.853498717580522,
137.75489110545));
#239304=CARTESIAN_POINT('Ctrl Pts',(11.1862778671706,6.30901505342741,133.843219478972));
#239305=CARTESIAN_POINT('Ctrl Pts',(10.9078302433578,5.96685476769427,127.13898501537));
#239306=CARTESIAN_POINT('Ctrl Pts',(10.6293826195448,0.141446447510913,
123.803051666633));
#239307=CARTESIAN_POINT('Ctrl Pts',(10.350934995732,-5.81394424789186,126.900979210845));
#239308=CARTESIAN_POINT('Ctrl Pts',(10.0724873719191,-6.42660420644864,
133.585923577051));
#239309=CARTESIAN_POINT('Ctrl Pts',(9.79403974810624,-1.1335288563486,137.714747470394));
#239310=CARTESIAN_POINT('Ctrl Pts',(9.51559212429333,5.20120413677258,135.493263437154));
#239311=CARTESIAN_POINT('Ctrl Pts',(9.23714450048043,6.75628462114785,128.962906778349));
#239312=CARTESIAN_POINT('Ctrl Pts',(8.95869687666756,2.10266960154115,124.124756237763));
#239313=CARTESIAN_POINT('Ctrl Pts',(8.68024925285465,-4.48319606076117,
125.4248358054));
#239314=CARTESIAN_POINT('Ctrl Pts',(8.40180162904178,-6.94922355952728,
131.66843587102));
#239315=CARTESIAN_POINT('Ctrl Pts',(8.12335400522884,-3.0292540955323,137.117992991138));
#239316=CARTESIAN_POINT('Ctrl Pts',(7.84490638141603,3.67445189496732,136.765630398031));
#239317=CARTESIAN_POINT('Ctrl Pts',(7.56645875760307,7.00151610094645,130.935152100895));
#239318=CARTESIAN_POINT('Ctrl Pts',(7.2880111337902,3.89452905323253,124.984482820099));
#239319=CARTESIAN_POINT('Ctrl Pts',(7.00956350997733,-2.79133993608059,
124.381996918337));
#239320=CARTESIAN_POINT('Ctrl Pts',(6.73111588616443,-6.91210388867261,
129.681349506257));
#239321=CARTESIAN_POINT('Ctrl Pts',(6.45266826235151,-4.68098204262199,
136.012694443327));
#239322=CARTESIAN_POINT('Ctrl Pts',(6.17422063853866,1.85173362191231,137.557835035774));
#239323=CARTESIAN_POINT('Ctrl Pts',(5.89577301472578,6.68279655012581,132.896862563455));
#239324=CARTESIAN_POINT('Ctrl Pts',(5.61732539091285,5.37269592153495,126.312983027266));
#239325=CARTESIAN_POINT('Ctrl Pts',(5.33887776709996,-0.874649788159289,
123.856460080569));
#239326=CARTESIAN_POINT('Ctrl Pts',(5.06043014328709,-6.31823507155263,
127.784718303561));
#239327=CARTESIAN_POINT('Ctrl Pts',(4.7819825194742,-5.95567098713191,134.487880295395));
#239328=CARTESIAN_POINT('Ctrl Pts',(4.50353489566127,-0.120136216239877,
137.806067653244));
#239329=CARTESIAN_POINT('Ctrl Pts',(4.22508727184843,5.82579786839633,134.690028297709));
#239330=CARTESIAN_POINT('Ctrl Pts',(3.94663964803551,6.41810831802433,128.003250169541));
#239331=CARTESIAN_POINT('Ctrl Pts',(3.66819202422262,1.11249076541009,123.890555701254));
#239332=CARTESIAN_POINT('Ctrl Pts',(3.3897444004097,-5.21545145242058,126.131310192911));
#239333=CARTESIAN_POINT('Ctrl Pts',(3.11129677659686,-6.75064857444498,
132.666369733619));
#239334=CARTESIAN_POINT('Ctrl Pts',(2.83284915278395,-2.08232944407128,
137.490333860877));
#239335=CARTESIAN_POINT('Ctrl Pts',(2.55440152897106,4.49954871795507,136.170215205482));
#239336=CARTESIAN_POINT('Ctrl Pts',(2.27595390515816,6.94656142335602,129.919138320362));
#239337=CARTESIAN_POINT('Ctrl Pts',(1.9975062813453,3.01002353908442,124.481537480858));
#239338=CARTESIAN_POINT('Ctrl Pts',(1.71905865753238,-3.69257892978116,
124.854302216906));
#239339=CARTESIAN_POINT('Ctrl Pts',(1.44061103371947,-7.00188175468703,
130.694879946647));
#239340=CARTESIAN_POINT('Ctrl Pts',(1.16216340990662,-3.87679730797559,
136.636065064534));
#239341=CARTESIAN_POINT('Ctrl Pts',(0.883715786093727,2.81087447268782,
137.218198690258));
#239342=CARTESIAN_POINT('Ctrl Pts',(0.605268162280799,6.91548993180329,
131.906328460586));
#239343=CARTESIAN_POINT('Ctrl Pts',(0.326820538467947,4.66510798405627,
125.5818036173));
#239344=CARTESIAN_POINT('Ctrl Pts',(0.0483729146550416,-1.87228029784353,
124.056553521165));
#239345=CARTESIAN_POINT('Ctrl Pts',(-0.23007470915786,-6.68913445200245,
128.732208497919));
#239346=CARTESIAN_POINT('Ctrl Pts',(-0.508522332970751,-5.35900082715629,
135.312070042369));
#239347=CARTESIAN_POINT('Ctrl Pts',(-0.786969956783612,0.895792756101716,
137.749566839272));
#239348=CARTESIAN_POINT('Ctrl Pts',(-1.06541758059653,6.32739655841135,
133.804758410613));
#239349=CARTESIAN_POINT('Ctrl Pts',(-1.34386520440944,5.94443203404716,
127.102730987725));
#239350=CARTESIAN_POINT('Ctrl Pts',(-1.62231282822229,0.0988248720430084,
123.802320359999));
#239351=CARTESIAN_POINT('Ctrl Pts',(-1.90076045203519,-5.83759751950527,
126.936442660293));
#239352=CARTESIAN_POINT('Ctrl Pts',(-2.17920807584809,-6.40955297312139,
133.624992605024));
#239353=CARTESIAN_POINT('Ctrl Pts',(-2.45765569966099,-1.09144236850938,
137.721519548813));
#239354=CARTESIAN_POINT('Ctrl Pts',(-2.73610332347384,5.22965045283876,
135.461515356786));
#239355=CARTESIAN_POINT('Ctrl Pts',(-3.01455094728676,6.74494999065597,
128.921813474073));
#239356=CARTESIAN_POINT('Ctrl Pts',(-3.29299857109967,2.06196999618574,
124.112080448687));
#239357=CARTESIAN_POINT('Ctrl Pts',(-3.57144619491253,-4.51585969194472,
125.452225962441));
#239358=CARTESIAN_POINT('Ctrl Pts',(-3.84989381872542,-6.94383493518842,
131.710721757939));
#239359=CARTESIAN_POINT('Ctrl Pts',(-4.12834144253832,-2.99076509818949,
137.136315943637));
#239360=CARTESIAN_POINT('Ctrl Pts',(-4.40678906635123,3.71067175704807,
136.743152517891));
#239361=CARTESIAN_POINT('Ctrl Pts',(-4.68523669016409,7.00218254395157,
130.892529461858));
#239362=CARTESIAN_POINT('Ctrl Pts',(-4.963684313977,3.85902964859785,124.960883545208));
#239363=CARTESIAN_POINT('Ctrl Pts',(-5.24213193778992,-2.83038296973812,
124.399107588329));
#239364=CARTESIAN_POINT('Ctrl Pts',(-5.52057956160276,-6.91881191077996,
129.723446251312));
#239365=CARTESIAN_POINT('Ctrl Pts',(-5.79902718541567,-4.6491907085676,
136.041092411279));
#239366=CARTESIAN_POINT('Ctrl Pts',(-6.07747480922856,1.89280962922548,
137.546437881394));
#239367=CARTESIAN_POINT('Ctrl Pts',(-6.35592243304147,6.69541038665145,
132.856143714835));
#239368=CARTESIAN_POINT('Ctrl Pts',(-6.63437005685431,5.34525608772619,
126.280361117063));
#239369=CARTESIAN_POINT('Ctrl Pts',(-6.91281768066725,-0.916927425542613,
123.86191305059));
#239370=CARTESIAN_POINT('Ctrl Pts',(-7.19126530448013,-6.33649942913263,
127.823235140749));
#239371=CARTESIAN_POINT('Ctrl Pts',(-7.469712928293,-5.93313801255607,134.524065908027));
#239372=CARTESIAN_POINT('Ctrl Pts',(-7.74816055210589,-0.0775126123463511,
137.806669231077));
#239373=CARTESIAN_POINT('Ctrl Pts',(-8.02660817591882,5.84934309190818,
134.654493020103));
#239374=CARTESIAN_POINT('Ctrl Pts',(-8.3050557997317,6.40093825099524,127.964233220621));
#239375=CARTESIAN_POINT('Ctrl Pts',(-8.58350342354456,1.07038386063539,
123.883911750995));
#239376=CARTESIAN_POINT('Ctrl Pts',(-8.86195104735747,-5.2438010064896,
126.163144707024));
#239377=CARTESIAN_POINT('Ctrl Pts',(-9.14039867117038,-6.73918892257159,
132.707428348838));
#239378=CARTESIAN_POINT('Ctrl Pts',(-9.41884629498326,-2.04159144649203,
137.50288571564));
#239379=CARTESIAN_POINT('Ctrl Pts',(-9.69729391879612,4.53212883162697,
136.142725758454));
#239380=CARTESIAN_POINT('Ctrl Pts',(-9.97574154260907,6.94104412028278,
129.876869030427));
#239381=CARTESIAN_POINT('Ctrl Pts',(-10.254189166422,2.97147895125515,124.463331760497));
#239382=CARTESIAN_POINT('Ctrl Pts',(-10.5326367902348,-3.72873020915888,
124.876890233732));
#239383=CARTESIAN_POINT('Ctrl Pts',(-10.8110844140478,-7.00241846595355,
130.737504416682));
#239384=CARTESIAN_POINT('Ctrl Pts',(-11.0895320378606,-3.84122623969676,
136.659556182137));
#239385=CARTESIAN_POINT('Ctrl Pts',(-11.3679796616735,2.84986524650705,
137.200969265957));
#239386=CARTESIAN_POINT('Ctrl Pts',(-11.6464272854864,6.92206979482823,
131.864211493609));
#239387=CARTESIAN_POINT('Ctrl Pts',(-11.9248749092993,4.6332303636112,125.553502542771));
#239388=CARTESIAN_POINT('Ctrl Pts',(-12.2033225331122,-1.91332142587795,
124.068075643991));
#239389=CARTESIAN_POINT('Ctrl Pts',(-12.4817701569251,-6.70162429593314,
128.77296555011));
#239390=CARTESIAN_POINT('Ctrl Pts',(-12.760217780738,-5.33146183057377,
135.344608284054));
#239391=CARTESIAN_POINT('Ctrl Pts',(-13.0386654045509,0.938053600692905,
137.743985215925));
#239392=CARTESIAN_POINT('Ctrl Pts',(-13.3171130283637,6.34554359938892,
133.766186161411));
#239393=CARTESIAN_POINT('Ctrl Pts',(-13.5955606521767,5.92178902728497,
127.066614125326));
#239394=CARTESIAN_POINT('Ctrl Pts',(-13.8740082759896,0.0561996345831295,
123.801848516541));
#239395=CARTESIAN_POINT('Ctrl Pts',(-14.1524558998025,-5.86103447679583,
126.972049436864));
#239396=CARTESIAN_POINT('Ctrl Pts',(-14.4309035236153,-6.39226423145161,
133.663957113442));
#239397=CARTESIAN_POINT('Ctrl Pts',(-14.7093511474282,-1.04931543687181,
137.728035309365));
#239398=CARTESIAN_POINT('Ctrl Pts',(-14.9877987712411,5.25790298228423,
135.429594703837));
#239399=CARTESIAN_POINT('Ctrl Pts',(-15.266246395054,6.73336542356173,128.880789928272));
#239400=CARTESIAN_POINT('Ctrl Pts',(-15.5446940188669,2.02119398377386,
124.099652644515));
#239401=CARTESIAN_POINT('Ctrl Pts',(-15.8231416426798,-4.54835598628669,
125.479814444798));
#239402=CARTESIAN_POINT('Ctrl Pts',(-16.1015892664927,-6.93818900449243,
131.752974059312));
#239403=CARTESIAN_POINT('Ctrl Pts',(-16.3800368903055,-2.95216527694612,
137.154404263204));
#239404=CARTESIAN_POINT('Ctrl Pts',(-16.6584845141185,3.74675411882228,
136.720454573632));
#239405=CARTESIAN_POINT('Ctrl Pts',(-16.9369321379314,7.00258951850748,
130.849903555692));
#239406=CARTESIAN_POINT('Ctrl Pts',(-17.2153797617442,3.82338724620039,
124.93750080251));
#239407=CARTESIAN_POINT('Ctrl Pts',(-17.4938273855571,-2.86932112251383,
124.416455607327));
#239408=CARTESIAN_POINT('Ctrl Pts',(-17.77227500937,-6.92526355376757,129.765583050046));
#239409=CARTESIAN_POINT('Ctrl Pts',(-18.0507226331829,-4.61722709704176,
136.069296330209));
#239410=CARTESIAN_POINT('Ctrl Pts',(-18.3291702569958,1.93381549778173,
137.534790896862));
#239411=CARTESIAN_POINT('Ctrl Pts',(-18.6076178808087,6.70777612228299,
132.81534883664));
#239412=CARTESIAN_POINT('Ctrl Pts',(-18.8860655046216,5.31761818348739,
126.247906845325));
#239413=CARTESIAN_POINT('Ctrl Pts',(-19.1645131284344,-0.959171085842972,
123.867623275557));
#239414=CARTESIAN_POINT('Ctrl Pts',(-19.4429607522474,-6.35452898539608,
127.861862444637));
#239415=CARTESIAN_POINT('Ctrl Pts',(-19.7214083760603,-5.91038518336925,
134.560113685611));
#239416=CARTESIAN_POINT('Ctrl Pts',(-19.9998559998732,-0.0348861361944895,
137.807011335788));
#239417=CARTESIAN_POINT('Ctrl Pts',(-20.278303623686,5.87267156586067,134.618815074426));
#239418=CARTESIAN_POINT('Ctrl Pts',(-20.5567512474989,6.38353099484532,
127.925321513668));
#239419=CARTESIAN_POINT('Ctrl Pts',(-20.8351988713118,1.02823729239309,
123.877524240513));
#239420=CARTESIAN_POINT('Ctrl Pts',(-21.1136464951247,-5.27195624958391,
126.1951512031));
#239421=CARTESIAN_POINT('Ctrl Pts',(-21.3920941189376,-6.72747954757436,
132.748416445183));
#239422=CARTESIAN_POINT('Ctrl Pts',(-21.6705417427505,-2.00077779699093,
137.515189354092));
#239423=CARTESIAN_POINT('Ctrl Pts',(-21.9489893665634,4.56454100559805,
136.115038496344));
#239424=CARTESIAN_POINT('Ctrl Pts',(-22.2274369903762,6.93526961426714,
129.834634109035));
#239425=CARTESIAN_POINT('Ctrl Pts',(-22.5058846141892,2.93282425418085,
124.445361009293));
#239426=CARTESIAN_POINT('Ctrl Pts',(-22.784332238002,-3.76474331906749,
124.899697895151));
#239427=CARTESIAN_POINT('Ctrl Pts',(-23.062779861815,-7.0026957000287,130.780131364099));
#239428=CARTESIAN_POINT('Ctrl Pts',(-23.3412274856278,-3.80551283336702,
136.682830333316));
#239429=CARTESIAN_POINT('Ctrl Pts',(-23.6196751094408,2.88875041752152,
137.183502812971));
#239430=CARTESIAN_POINT('Ctrl Pts',(-23.8981227332536,6.92839315801137,
131.822055253468));
#239431=CARTESIAN_POINT('Ctrl Pts',(-24.1765703570665,4.60118105711114,
125.525396040718));
#239432=CARTESIAN_POINT('Ctrl Pts',(-24.4550179808794,-1.95429165508329,
124.079847382335));
#239433=CARTESIAN_POINT('Ctrl Pts',(-24.7334656046923,-6.71386580871103,
128.813797876394));
#239434=CARTESIAN_POINT('Ctrl Pts',(-25.0119132285052,-5.30372527471246,
135.376978285193));
#239435=CARTESIAN_POINT('Ctrl Pts',(-25.290360852318,0.980279685362951,
137.738146442235));
#239436=CARTESIAN_POINT('Ctrl Pts',(-25.568808476131,6.36345550391485,133.727504160674));
#239437=CARTESIAN_POINT('Ctrl Pts',(-25.8472560999438,5.89892658645264,
127.030635766497));
#239438=CARTESIAN_POINT('Ctrl Pts',(-26.1257037237567,0.0135723146251221,
123.801636153745));
#239439=CARTESIAN_POINT('Ctrl Pts',(-26.4041513475696,-5.88425425129846,
127.007798221134));
#239440=CARTESIAN_POINT('Ctrl Pts',(-26.6825989713826,-6.37473862207999,
133.70281565846));
#239441=CARTESIAN_POINT('Ctrl Pts',(-26.9610465951954,-1.00714962246484,
137.734294510605));
#239442=CARTESIAN_POINT('Ctrl Pts',(-27.2394942190083,5.28596067820108,
135.397502661138));
#239443=CARTESIAN_POINT('Ctrl Pts',(-27.5179418428212,6.72153134913555,
128.839837661092));
#239444=CARTESIAN_POINT('Ctrl Pts',(-27.7963894666341,1.98034307527561,
124.087473285763));
#239445=CARTESIAN_POINT('Ctrl Pts',(-28.0748370904469,-4.58068373962494,
125.507600230172));
#239446=CARTESIAN_POINT('Ctrl Pts',(-28.3532847142599,-6.93228597665136,
131.795191209466));
#239447=CARTESIAN_POINT('Ctrl Pts',(-28.6317323380727,-2.91345606213275,
137.172257279568));
#239448=CARTESIAN_POINT('Ctrl Pts',(-28.9101799618857,3.78269764324474,
136.697537406337));
#239449=CARTESIAN_POINT('Ctrl Pts',(-29.1886275856985,7.00273700953358,
130.807275961916));
#239450=CARTESIAN_POINT('Ctrl Pts',(-29.4670752095115,3.78760316678249,
124.914335458459));
#239451=CARTESIAN_POINT('Ctrl Pts',(-29.7455228333243,-2.90815295154017,
124.434040332496));
#239452=CARTESIAN_POINT('Ctrl Pts',(-30.0239704571372,-6.93145857856742,
129.807758341064));
#239453=CARTESIAN_POINT('Ctrl Pts',(-30.3024180809501,-4.5850923924679,
136.097305155009));
#239454=CARTESIAN_POINT('Ctrl Pts',(-30.580865704763,1.97474970809384,137.52289451376));
#239455=CARTESIAN_POINT('Ctrl Pts',(-30.8593133285759,6.71989329880362,
132.774479440534));
#239456=CARTESIAN_POINT('Ctrl Pts',(-31.1377609523888,5.28978323295099,
126.215621414657));
#239457=CARTESIAN_POINT('Ctrl Pts',(-31.4162085762017,-1.00137920370602,
123.873590543879));
#239458=CARTESIAN_POINT('Ctrl Pts',(-31.6946562000146,-6.37232307225107,
127.900598783877));
#239459=CARTESIAN_POINT('Ctrl Pts',(-31.9731038238274,-5.88741334268594,
134.596022292384));
#239460=CARTESIAN_POINT('Ctrl Pts',(-32.2515514476404,0.00774163267598956,
137.807093954702));
#239461=CARTESIAN_POINT('Ctrl Pts',(-32.5299990714533,5.89578242580862,
134.582995782735));
#239462=CARTESIAN_POINT('Ctrl Pts',(-32.8084466952661,6.36588719460685,
127.886516490566));
#239463=CARTESIAN_POINT('Ctrl Pts',(-33.086894319079,0.9860526224398,123.8713934065));
#239464=CARTESIAN_POINT('Ctrl Pts',(-33.365341942892,-5.29991613840065,
126.227328495126));
#239465=CARTESIAN_POINT('Ctrl Pts',(-33.6437895667048,-6.71552088334846,
132.789332503824));
#239466=CARTESIAN_POINT('Ctrl Pts',(-33.9222371905177,-1.95989000793276,
137.527244320318));
#239467=CARTESIAN_POINT('Ctrl Pts',(-34.2006848143306,4.59678403882356,
136.08715444511));
#239468=CARTESIAN_POINT('Ctrl Pts',(-34.4791324381435,6.9292381192855,129.792435121214));
#239469=CARTESIAN_POINT('Ctrl Pts',(-34.7575800619564,2.89406088022529,
124.427625893158));
#239470=CARTESIAN_POINT('Ctrl Pts',(-35.0360276857693,-3.80061692502793,
124.922724356021));
#239471=CARTESIAN_POINT('Ctrl Pts',(-35.3144753095821,-7.00271344663942,
130.822759209339));
#239472=CARTESIAN_POINT('Ctrl Pts',(-35.592922933395,-3.76965841235978,
136.705886655638));
#239473=CARTESIAN_POINT('Ctrl Pts',(-35.8713705572079,2.92752854482695,
137.165799978524));
#239474=CARTESIAN_POINT('Ctrl Pts',(-36.1498181810209,6.9344597870381,131.779861302279));
#239475=CARTESIAN_POINT('Ctrl Pts',(-36.4282658048337,4.56896125215494,
125.49748515264));
#239476=CARTESIAN_POINT('Ctrl Pts',(-36.7067134286466,-1.99518946729269,
124.091868299989));
#239477=CARTESIAN_POINT('Ctrl Pts',(-36.9851610524595,-6.72585853672236,
128.854703963711));
#239478=CARTESIAN_POINT('Ctrl Pts',(-37.2636086762724,-5.27579218736066,
135.409178846303));
#239479=CARTESIAN_POINT('Ctrl Pts',(-37.5420563000852,1.02246944540875,
137.732050734562));
#239480=CARTESIAN_POINT('Ctrl Pts',(-37.8205039238982,6.38113160825695,
133.688713841779));
#239481=CARTESIAN_POINT('Ctrl Pts',(-38.0989515477111,5.87584555872632,
126.994797244432));
#239482=CARTESIAN_POINT('Ctrl Pts',(-38.377399171524,-0.0290555082599903,
123.801683279478));
#239483=CARTESIAN_POINT('Ctrl Pts',(-38.6558467953367,-5.90725598259587,
127.04368768842));
#239484=CARTESIAN_POINT('Ctrl Pts',(-38.9342944191497,-6.35697679442443,
133.741566800161));
#239485=CARTESIAN_POINT('Ctrl Pts',(-39.2127420429625,-0.964946487758246,
137.740296920595));
#239486=CARTESIAN_POINT('Ctrl Pts',(-39.4911896667755,5.31382250090111,
135.365240417872));
#239487=CARTESIAN_POINT('Ctrl Pts',(-39.7696372905882,6.70944820589337,
128.798958190032));
#239488=CARTESIAN_POINT('Ctrl Pts',(-40.0480849144012,1.93941878443644,
124.07554282374));
#239489=CARTESIAN_POINT('Ctrl Pts',(-40.3265325382142,-4.61284175404266,
125.535582288951));
#239490=CARTESIAN_POINT('Ctrl Pts',(-40.604980162027,-6.9261260704041,131.837371644027));
#239491=CARTESIAN_POINT('Ctrl Pts',(-40.8834277858398,-2.87463888813357,
137.18987433118));
#239492=CARTESIAN_POINT('Ctrl Pts',(-41.1618754096529,3.81850099841496,
136.674401865208));
#239493=CARTESIAN_POINT('Ctrl Pts',(-41.4403230334656,7.00262501156454,
130.76464826011));
#239494=CARTESIAN_POINT('Ctrl Pts',(-41.7187706572786,3.75167873633635,
124.891388371457));
#239495=CARTESIAN_POINT('Ctrl Pts',(-41.9972182810916,-2.94687701788942,
124.451861112224));
#239496=CARTESIAN_POINT('Ctrl Pts',(-42.2756659049044,-6.93739675562063,
129.849970561546));
#239497=CARTESIAN_POINT('Ctrl Pts',(-42.5541135287174,-4.55278778560923,
136.125117847804));
#239498=CARTESIAN_POINT('Ctrl Pts',(-42.8325611525302,2.01561074332903,
137.510749172913));
#239499=CARTESIAN_POINT('Ctrl Pts',(-43.1110087763431,6.73176146720674,
132.733537040953));
#239500=CARTESIAN_POINT('Ctrl Pts',(-43.389456400156,5.26175226755184,126.183506021407));
#239501=CARTESIAN_POINT('Ctrl Pts',(-43.6679040239687,-1.0435502150944,
123.879814634434));
#239502=CARTESIAN_POINT('Ctrl Pts',(-43.9463516477818,-6.38988103033122,
127.93944272308));
#239503=CARTESIAN_POINT('Ctrl Pts',(-44.2247992715946,-5.86422334173611,
134.631790397739));
#239504=CARTESIAN_POINT('Ctrl Pts',(-44.5032468954075,0.050369114677416,
137.806917084757));
#239505=CARTESIAN_POINT('Ctrl Pts',(-44.7816945192204,5.91867481537061,
134.547036472328));
#239506=CARTESIAN_POINT('Ctrl Pts',(-45.0601421430334,6.34800750407734,
127.847819589252));
#239507=CARTESIAN_POINT('Ctrl Pts',(-45.3385897668461,0.943831413943965,
123.865519476137));
#239508=CARTESIAN_POINT('Ctrl Pts',(-45.6170373906592,-5.32767963687585,
126.25967539076));
#239509=CARTESIAN_POINT('Ctrl Pts',(-45.895485014472,-6.7033133730266,132.830175008601));
#239510=CARTESIAN_POINT('Ctrl Pts',(-46.1739326382849,-1.91892959442962,
137.539050167615));
#239511=CARTESIAN_POINT('Ctrl Pts',(-46.4523802620978,4.62885673652604,
136.059074638009));
#239512=CARTESIAN_POINT('Ctrl Pts',(-46.7308278859106,6.92294985883713,
129.750273630666));
#239513=CARTESIAN_POINT('Ctrl Pts',(-47.0092755097235,2.8551902657795,124.410127069272));
#239514=CARTESIAN_POINT('Ctrl Pts',(-47.2877231335364,-3.83634969773052,
124.945968763085));
#239515=CARTESIAN_POINT('Ctrl Pts',(-47.5661707573492,-7.00247170512816,
130.865386372813));
#239516=CARTESIAN_POINT('Ctrl Pts',(-47.8446183811622,-3.73366430527375,
136.728724294741));
#239517=CARTESIAN_POINT('Ctrl Pts',(-48.123066004975,2.96619819148554,137.147861418602));
#239518=CARTESIAN_POINT('Ctrl Pts',(-48.4015136287881,6.9402694571073,131.737631203552));
#239519=CARTESIAN_POINT('Ctrl Pts',(-48.6799612526008,4.53657214265928,
125.469770912784));
#239520=CARTESIAN_POINT('Ctrl Pts',(-48.9584088764139,-2.03601334702262,
124.104137951514));
#239521=CARTESIAN_POINT('Ctrl Pts',(-49.2368565002267,-6.7376020355722,
128.895682296272));
#239522=CARTESIAN_POINT('Ctrl Pts',(-49.5153041240395,-5.24766360358919,
135.441208774179));
#239523=CARTESIAN_POINT('Ctrl Pts',(-49.7937517478526,1.06462131747325,
137.725698318783));
#239524=CARTESIAN_POINT('Ctrl Pts',(-50.0721993716652,6.39857125742062,
133.649816642113));
#239525=CARTESIAN_POINT('Ctrl Pts',(-50.3506469954783,5.85254679938199,
126.959099887138));
#239526=CARTESIAN_POINT('Ctrl Pts',(-50.6290946192911,-0.0716822544825644,
123.801989891996));
#239527=CARTESIAN_POINT('Ctrl Pts',(-50.907542243104,-5.93003881835047,
127.079716508824));
#239528=CARTESIAN_POINT('Ctrl Pts',(-51.1859898669169,-6.33897940665598,
133.780209102606));
#239529=CARTESIAN_POINT('Ctrl Pts',(-51.4644374907297,-0.922707596604453,
137.746042316915));
#239530=CARTESIAN_POINT('Ctrl Pts',(-51.7428851145428,5.34148741795441,
135.332809169526));
#239531=CARTESIAN_POINT('Ctrl Pts',(-52.0213327383556,6.69711644158035,
128.758153029896));
#239532=CARTESIAN_POINT('Ctrl Pts',(-52.2997803621686,1.89842262772099,
124.063861700536));
#239533=CARTESIAN_POINT('Ctrl Pts',(-52.5782279859813,-4.64482883791282,
125.563759584248));
#239534=CARTESIAN_POINT('Ctrl Pts',(-52.8566756097944,-6.91970951400822,
131.879513799985));
#239535=CARTESIAN_POINT('Ctrl Pts',(-53.135123233607,-2.83571519333325,
137.207254765232));
#239536=CARTESIAN_POINT('Ctrl Pts',(-53.4135708574202,3.85416285762642,
136.651048807542));
#239537=CARTESIAN_POINT('Ctrl Pts',(-53.6920184812329,7.0022535287505,130.72202202986));
#239538=CARTESIAN_POINT('Ctrl Pts',(-53.9704661050458,3.71561528605495,
124.868660391816));
#239539=CARTESIAN_POINT('Ctrl Pts',(-54.2489137288587,-2.98549188662705,
124.469917286158));
#239540=CARTESIAN_POINT('Ctrl Pts',(-54.5273613526715,-6.94307786488582,
129.892218147303));
#239541=CARTESIAN_POINT('Ctrl Pts',(-54.8058089764845,-4.5203144735249,
136.152733377983));
#239542=CARTESIAN_POINT('Ctrl Pts',(-55.0842566002972,2.05639708936689,
137.498355324372));
#239543=CARTESIAN_POINT('Ctrl Pts',(-55.3627042241104,6.74338018771311,
132.69252315503));
#239544=CARTESIAN_POINT('Ctrl Pts',(-55.6411518479232,5.23352632598741,
126.151561855625));
#239545=CARTESIAN_POINT('Ctrl Pts',(-55.919599471736,-1.08568255734582,
123.886295316588));
#239546=CARTESIAN_POINT('Ctrl Pts',(-56.1980470955489,-6.40720220901991,
127.978392822871));
#239547=CARTESIAN_POINT('Ctrl Pts',(-56.4764947193619,-5.8408160398338,
134.667416676276));
#239548=CARTESIAN_POINT('Ctrl Pts',(-56.7549423431748,0.0929947302327828,
137.806480732508));
#239549=CARTESIAN_POINT('Ctrl Pts',(-57.0333899669875,5.94134788626073,
134.510938475691));
#239550=CARTESIAN_POINT('Ctrl Pts',(-57.3118375908005,6.32989258579528,
127.809232243652));
#239551=CARTESIAN_POINT('Ctrl Pts',(-57.5902852146133,0.901575231427987,
123.859902667085));
#239552=CARTESIAN_POINT('Ctrl Pts',(-57.8687328384263,-5.35524571622284,
126.292190691378));
#239553=CARTESIAN_POINT('Ctrl Pts',(-58.1471804622391,-6.69085746896258,
132.870942446081));
#239554=CARTESIAN_POINT('Ctrl Pts',(-58.4256280860521,-1.87789807428466,
137.550606458515));
#239555=CARTESIAN_POINT('Ctrl Pts',(-58.7040757098649,4.6607579102399,136.030800115547));
#239556=CARTESIAN_POINT('Ctrl Pts',(-58.9825233336777,6.91640506593584,
129.708151199698));
#239557=CARTESIAN_POINT('Ctrl Pts',(-59.2609709574908,2.81621385120844,
124.392865186062));
#239558=CARTESIAN_POINT('Ctrl Pts',(-59.5394185813036,-3.87194031308425,
124.969430255013));
#239559=CARTESIAN_POINT('Ctrl Pts',(-59.8178662051166,-7.00197048445272,
130.908011274954));
#239560=CARTESIAN_POINT('Ctrl Pts',(-60.0963138289294,-3.69753184588372,
136.751342404371));
#239561=CARTESIAN_POINT('Ctrl Pts',(-60.3747614527424,3.00475792457964,
137.129687797925));
#239562=CARTESIAN_POINT('Ctrl Pts',(-60.6532090765552,6.94582195293937,
131.695366522141));
#239563=CARTESIAN_POINT('Ctrl Pts',(-60.9316567003681,4.50401492881459,
125.442254348109));
#239564=CARTESIAN_POINT('Ctrl Pts',(-61.210104324181,-2.07676178152925,
124.116655882255));
#239565=CARTESIAN_POINT('Ctrl Pts',(-61.4885519479939,-6.74909587010084,
128.93673135561));
#239566=CARTESIAN_POINT('Ctrl Pts',(-61.7669995718066,-5.21934056571308,
135.473066881942));
#239567=CARTESIAN_POINT('Ctrl Pts',(-62.0454471956197,1.10673373960332,
137.719089430292));
#239568=CARTESIAN_POINT('Ctrl Pts',(-62.3238948194324,6.41577380517329,
133.610814003028));
#239569=CARTESIAN_POINT('Ctrl Pts',(-62.6023424432454,5.82903117176375,
126.923545017394));
#239570=CARTESIAN_POINT('Ctrl Pts',(-62.8807900670583,-0.114306344492842,
123.802555979936));
#239571=CARTESIAN_POINT('Ctrl Pts',(-63.1592376908712,-5.95260191433588,
127.115883347286));
#239572=CARTESIAN_POINT('Ctrl Pts',(-63.4376853146842,-6.32074712567447,
133.818741133891));
#239573=CARTESIAN_POINT('Ctrl Pts',(-63.716132938497,-0.880434514181572,
137.751530486667));
#239574=CARTESIAN_POINT('Ctrl Pts',(-63.99458056231,5.36895440422691,135.300210117855));
#239575=CARTESIAN_POINT('Ctrl Pts',(-64.2730281861228,6.6845365131549,128.717423692735));
#239576=CARTESIAN_POINT('Ctrl Pts',(-64.5514758099358,1.85735612425694,
124.052430348997));
#239577=CARTESIAN_POINT('Ctrl Pts',(-64.8299234337484,-4.67664380594228,
125.592131071942));
#239578=CARTESIAN_POINT('Ctrl Pts',(-65.1083710575615,-6.91303654523158,
131.921616115747));
#239579=CARTESIAN_POINT('Ctrl Pts',(-65.3868186813742,-2.79668642006362,
137.224397937687));
#239580=CARTESIAN_POINT('Ctrl Pts',(-65.6652663051872,3.88968189941585,
136.627479098696));
#239581=CARTESIAN_POINT('Ctrl Pts',(-65.9437139290001,7.00162257485687,
130.679398850698));
#239582=CARTESIAN_POINT('Ctrl Pts',(-66.2221615528129,3.67941415228271,
124.846152361731));
#239583=CARTESIAN_POINT('Ctrl Pts',(-66.500609176626,-3.02399612686491,
124.48820818522));
#239584=CARTESIAN_POINT('Ctrl Pts',(-66.7790568004388,-6.94850169584742,
129.934499532835));
#239585=CARTESIAN_POINT('Ctrl Pts',(-67.0575044242516,-4.48767365952541,
136.180150722241));
#239586=CARTESIAN_POINT('Ctrl Pts',(-67.3359520480646,2.09710723485436,
137.485713427398));
#239587=CARTESIAN_POINT('Ctrl Pts',(-67.6143996718775,6.75474902978674,
132.651439302549));
#239588=CARTESIAN_POINT('Ctrl Pts',(-67.8928472956903,5.20510645418034,
126.119790101011));
#239589=CARTESIAN_POINT('Ctrl Pts',(-68.1712949195033,-1.12777466923081,
123.893032350195));
#239590=CARTESIAN_POINT('Ctrl Pts',(-68.449742543316,-6.42428596647451,
128.017447639935));
#239591=CARTESIAN_POINT('Ctrl Pts',(-68.728190167129,-5.81719230434518,
134.702899807851));
#239592=CARTESIAN_POINT('Ctrl Pts',(-69.0066377909419,0.135616899834216,
137.805784914121));
#239593=CARTESIAN_POINT('Ctrl Pts',(-69.2850854147548,5.96380079832,134.474703130449));
#239594=CARTESIAN_POINT('Ctrl Pts',(-69.5635330385676,6.31154311101565,
127.770755883637));
#239595=CARTESIAN_POINT('Ctrl Pts',(-69.8419806623805,0.859285640710264,
123.854543187474));
#239596=CARTESIAN_POINT('Ctrl Pts',(-70.1204282861936,-5.38261335497044,
126.324873192109));
#239597=CARTESIAN_POINT('Ctrl Pts',(-70.3988759100064,-6.67815363271447,
132.911633305611));
#239598=CARTESIAN_POINT('Ctrl Pts',(-70.6773235338194,-1.83679696793597,
137.561912764793));
#239599=CARTESIAN_POINT('Ctrl Pts',(-70.9557711576322,4.69248637785542,
136.002331925448));
#239600=CARTESIAN_POINT('Ctrl Pts',(-71.2342187814451,6.90960398310133,
129.666069389173));
#239601=CARTESIAN_POINT('Ctrl Pts',(-71.5126664052579,2.77713308079745,
124.375840883174));
#239602=CARTESIAN_POINT('Ctrl Pts',(-71.7911140290708,-3.90738745226578,
124.993107962432));
#239603=CARTESIAN_POINT('Ctrl Pts',(-72.0695616528837,-7.00120980318599,
130.950632336283));
#239604=CARTESIAN_POINT('Ctrl Pts',(-72.3480092766965,-3.66126237309149,
136.773740146404));
#239605=CARTESIAN_POINT('Ctrl Pts',(-72.6264569005095,3.04320631526353,
137.111279789924));
#239606=CARTESIAN_POINT('Ctrl Pts',(-72.9049045243223,6.95111706878496,
131.653068824177));
#239607=CARTESIAN_POINT('Ctrl Pts',(-73.1833521481353,4.47129081703998,
125.414936478256));
#239608=CARTESIAN_POINT('Ctrl Pts',(-73.4617997719481,-2.11743326086482,
124.129421628353));
#239609=CARTESIAN_POINT('Ctrl Pts',(-73.7402473957612,-6.76033961440018,
128.977849620639));
#239610=CARTESIAN_POINT('Ctrl Pts',(-74.018695019574,-5.19082412325261,
135.504751989078));
#239611=CARTESIAN_POINT('Ctrl Pts',(-74.2971426433868,1.14880515130821,
137.712224313981));
#239612=CARTESIAN_POINT('Ctrl Pts',(-74.5755902671998,6.43273861406817,
133.571707369781));
#239613=CARTESIAN_POINT('Ctrl Pts',(-74.8540378910127,5.80529954725181,
126.8881339527));
#239614=CARTESIAN_POINT('Ctrl Pts',(-75.1324855148255,-0.156926198840311,
123.803381522322));
#239615=CARTESIAN_POINT('Ctrl Pts',(-75.4109331386384,-5.97494443446864,
127.15218686363));
#239616=CARTESIAN_POINT('Ctrl Pts',(-75.6893807624512,-6.30228062708332,
133.857161466198));
#239617=CARTESIAN_POINT('Ctrl Pts',(-75.9678283862644,-0.838128806933456,
137.756761226486));
#239618=CARTESIAN_POINT('Ctrl Pts',(-76.2462760100769,5.3962224419198,135.267444470826));
#239619=CARTESIAN_POINT('Ctrl Pts',(-76.52472363389,6.67170888677059,128.676771687789));
#239620=CARTESIAN_POINT('Ctrl Pts',(-76.8031712577027,1.81622079577817,
124.041249192718));
#239621=CARTESIAN_POINT('Ctrl Pts',(-77.0816188815158,-4.70828547921653,
125.620695700721));
#239622=CARTESIAN_POINT('Ctrl Pts',(-77.3600665053286,-6.90610741134329,
131.963677031195));
#239623=CARTESIAN_POINT('Ctrl Pts',(-77.6385141291417,-2.75755401454922,
137.241303213299));
#239624=CARTESIAN_POINT('Ctrl Pts',(-77.9169617529544,3.92505680761298,
136.603693612052));
#239625=CARTESIAN_POINT('Ctrl Pts',(-78.1954093767674,7.00073217326374,
130.636780302039));
#239626=CARTESIAN_POINT('Ctrl Pts',(-78.4738570005803,3.6430766764653,124.823865115242));
#239627=CARTESIAN_POINT('Ctrl Pts',(-78.7523046243931,-3.06238831181505,
124.506733131632));
#239628=CARTESIAN_POINT('Ctrl Pts',(-79.0307522482061,-6.95366804752337,
129.976813151389));
#239629=CARTESIAN_POINT('Ctrl Pts',(-79.3091998720188,-4.45486655312747,
136.207368864621));
#239630=CARTESIAN_POINT('Ctrl Pts',(-79.5876474958318,2.13773967126259,
137.472823950436));
#239631=CARTESIAN_POINT('Ctrl Pts',(-79.8660951196445,6.76586757215105,
132.610287005887));
#239632=CARTESIAN_POINT('Ctrl Pts',(-80.1445427434577,5.17649370523912,
126.08819193488));
#239633=CARTESIAN_POINT('Ctrl Pts',(-80.4229903672703,-1.16982499101125,
123.900025485612));
#239634=CARTESIAN_POINT('Ctrl Pts',(-80.7014379910835,-6.44113166965063,
128.056605727087));
#239635=CARTESIAN_POINT('Ctrl Pts',(-80.9798856148961,-5.7933530106558,
134.738238477622));
#239636=CARTESIAN_POINT('Ctrl Pts',(-81.2583332387092,0.17823404410257,
137.804829655383));
#239637=CARTESIAN_POINT('Ctrl Pts',(-81.5367808625219,5.98603271954817,
134.438331779315));
#239638=CARTESIAN_POINT('Ctrl Pts',(-81.815228486335,6.29295975968447,127.732391934959));
#239639=CARTESIAN_POINT('Ctrl Pts',(-82.0936761101477,0.816964208846405,
123.849441235906));
#239640=CARTESIAN_POINT('Ctrl Pts',(-82.3721237339607,-5.40978153900143,
126.357721681897));
#239641=CARTESIAN_POINT('Ctrl Pts',(-82.6505713577735,-6.66520233502723,
132.952246079378));
#239642=CARTESIAN_POINT('Ctrl Pts',(-82.9290189815866,-1.79562779839943,
137.572968667493));
#239643=CARTESIAN_POINT('Ctrl Pts',(-83.2074666053992,4.72404096366304,
135.97367112261));
#239644=CARTESIAN_POINT('Ctrl Pts',(-83.4859142292123,6.90254686235,129.624029758449));
#239645=CARTESIAN_POINT('Ctrl Pts',(-83.7643618530252,2.73794940269844,
124.359054791448));
#239646=CARTESIAN_POINT('Ctrl Pts',(-84.0428094768383,-3.94268980176888,
125.017001007954));
#239647=CARTESIAN_POINT('Ctrl Pts',(-84.3212571006508,-7.00018968951541,
130.99324797746));
#239648=CARTESIAN_POINT('Ctrl Pts',(-84.5997047244641,-3.62485723087481,
136.795916690882));
#239649=CARTESIAN_POINT('Ctrl Pts',(-84.8781523482765,3.08154193881888,
137.092638076712));
#239650=CARTESIAN_POINT('Ctrl Pts',(-85.1565999720898,6.95615460843127,
131.61073967702));
#239651=CARTESIAN_POINT('Ctrl Pts',(-85.4350475959023,4.4384010199398,125.387818315495));
#239652=CARTESIAN_POINT('Ctrl Pts',(-85.7134952197154,-2.1580262779319,
124.142434716771));
#239653=CARTESIAN_POINT('Ctrl Pts',(-85.9919428435283,-6.7713328518292,
129.019035567703));
#239654=CARTESIAN_POINT('Ctrl Pts',(-86.2703904673411,-5.16211533289519,
135.536262921482));
#239655=CARTESIAN_POINT('Ctrl Pts',(-86.5488380911541,1.19083399361533,
137.70510322424));
#239656=CARTESIAN_POINT('Ctrl Pts',(-86.827285714967,6.4494650554685,133.532498191482));
#239657=CARTESIAN_POINT('Ctrl Pts',(-87.1057333387799,5.78135280522977,
126.852868005224));
#239658=CARTESIAN_POINT('Ctrl Pts',(-87.3841809625928,-0.199540238229241,
123.804466488563));
#239659=CARTESIAN_POINT('Ctrl Pts',(-87.6626285864056,-5.99706555083783,
127.188625712615));
#239660=CARTESIAN_POINT('Ctrl Pts',(-87.9410762102187,-6.28358059516641,
133.895468675847));
#239661=CARTESIAN_POINT('Ctrl Pts',(-88.2195238340314,-0.795792042514341,
137.761734342542));
#239662=CARTESIAN_POINT('Ctrl Pts',(-88.4979714578443,5.42329052060546,
135.234513442586));
#239663=CARTESIAN_POINT('Ctrl Pts',(-88.7764190816572,6.65863403776028,
128.636198521433));
#239664=CARTESIAN_POINT('Ctrl Pts',(-89.0548667054699,1.77501816656995,
124.03031864602));
#239665=CARTESIAN_POINT('Ctrl Pts',(-89.3333143292831,-4.73975268523957,
125.649452412109));
#239666=CARTESIAN_POINT('Ctrl Pts',(-89.6117619530957,-6.8989223691057,
132.005694987746));
#239667=CARTESIAN_POINT('Ctrl Pts',(-89.8902095769088,-2.71831942685781,
137.257969965635));
#239668=CARTESIAN_POINT('Ctrl Pts',(-90.1686572007216,3.9602862713853,136.579693228991));
#239669=CARTESIAN_POINT('Ctrl Pts',(-90.4471048245344,6.99958235696585,
130.59416796313));
#239670=CARTESIAN_POINT('Ctrl Pts',(-90.7255524483476,3.60660420510239,
124.801799478213));
#239671=CARTESIAN_POINT('Ctrl Pts',(-91.0040000721602,-3.10066701883943,
124.525491438947));
#239672=CARTESIAN_POINT('Ctrl Pts',(-91.2824476959735,-6.95857672847263,
130.019157435019));
#239673=CARTESIAN_POINT('Ctrl Pts',(-91.560895319786,-4.4218943700117,136.234386796543));
#239674=CARTESIAN_POINT('Ctrl Pts',(-91.8393429435991,2.17829289294083,
137.459687371113));
#239675=CARTESIAN_POINT('Ctrl Pts',(-92.1177905674117,6.77673540280433,
132.56906778996));
#239676=CARTESIAN_POINT('Ctrl Pts',(-92.3962381912249,5.14768913942031,
126.056768528114));
#239677=CARTESIAN_POINT('Ctrl Pts',(-92.6746858150375,-1.21183196449619,
123.907274463707));
#239678=CARTESIAN_POINT('Ctrl Pts',(-92.9531334388505,-6.45773869432309,
128.095865633305));
#239679=CARTESIAN_POINT('Ctrl Pts',(-93.2315810626634,-5.76929904214118,
134.773431376103));
#239680=CARTESIAN_POINT('Ctrl Pts',(-93.5100286864763,0.220844583841736,
137.803614991691));
#239681=CARTESIAN_POINT('Ctrl Pts',(-93.7884763102892,6.00804282613147,
134.401825770043));
#239682=CARTESIAN_POINT('Ctrl Pts',(-94.0669239341021,6.27414322041607,
127.694141819211));
#239683=CARTESIAN_POINT('Ctrl Pts',(-94.3453715579151,0.774612504073732,
123.844597001431));
#239684=CARTESIAN_POINT('Ctrl Pts',(-94.6238191817278,-5.43674926158731,
126.390734943524));
#239685=CARTESIAN_POINT('Ctrl Pts',(-94.9022668055408,-6.65200405581671,
132.99277926246));
#239686=CARTESIAN_POINT('Ctrl Pts',(-95.1807144293538,-1.75439209121494,
137.583773756932));
#239687=CARTESIAN_POINT('Ctrl Pts',(-95.4591620531666,4.75542049839504,
135.94481876907));
#239688=CARTESIAN_POINT('Ctrl Pts',(-95.7376096769794,6.89523396518648,
129.582033865318));
#239689=CARTESIAN_POINT('Ctrl Pts',(-96.0160573007924,2.69866426887766,
124.342507532899));
#239690=CARTESIAN_POINT('Ctrl Pts',(-96.2945049246052,-3.97784605345104,
125.041108506217));
#239691=CARTESIAN_POINT('Ctrl Pts',(-96.5729525484182,-6.99891018124123,
131.035856619345));
#239692=CARTESIAN_POINT('Ctrl Pts',(-96.8514001722308,-3.58831776824163,
136.817871216047));
#239693=CARTESIAN_POINT('Ctrl Pts',(-97.129847796044,3.11976337470375,137.073763349068));
#239694=CARTESIAN_POINT('Ctrl Pts',(-97.4082954198568,6.96093438520996,
131.56838064919));
#239695=CARTESIAN_POINT('Ctrl Pts',(-97.6867430436697,4.40534675625846,
125.360900864701));
#239696=CARTESIAN_POINT('Ctrl Pts',(-97.9651906674826,-2.1985393285419,
124.155694665303));
#239697=CARTESIAN_POINT('Ctrl Pts',(-98.2436382912955,-6.78207517502872,
129.060287670645));
#239698=CARTESIAN_POINT('Ctrl Pts',(-98.5220859151084,-5.13321525845608,
135.567598511506));
#239699=CARTESIAN_POINT('Ctrl Pts',(-98.8005335389213,1.23281870913114,
137.697726424945));
#239700=CARTESIAN_POINT('Ctrl Pts',(-99.0789811627341,6.4659525095689,133.493187921042));
#239701=CARTESIAN_POINT('Ctrl Pts',(-99.3574287865471,5.7571918330539,126.817748481762));
#239702=CARTESIAN_POINT('Ctrl Pts',(-99.6358764103599,-0.242146883580649,
123.805810838454));
#239703=CARTESIAN_POINT('Ctrl Pts',(-99.9143240341728,-6.01896444373747,
127.225198543987));
#239704=CARTESIAN_POINT('Ctrl Pts',(-100.192771657986,-6.26464772285957,
133.93366134335));
#239705=CARTESIAN_POINT('Ctrl Pts',(-100.471219281798,-0.753425789729175,
137.766449650557));
#239706=CARTESIAN_POINT('Ctrl Pts',(-100.749666905611,5.45015763726631,
135.201418253402));
#239707=CARTESIAN_POINT('Ctrl Pts',(-101.028114529424,6.64531245061667,
128.595705697122));
#239708=CARTESIAN_POINT('Ctrl Pts',(-101.306562153237,1.73374976341167,
124.019639113937));
#239709=CARTESIAN_POINT('Ctrl Pts',(-101.58500977705,-4.77104425798471,
125.678400140516));
#239710=CARTESIAN_POINT('Ctrl Pts',(-101.863457400863,-6.89148168476197,
132.047668428412));
#239711=CARTESIAN_POINT('Ctrl Pts',(-102.141905024676,-2.67898411084018,
137.274397577103));
#239712=CARTESIAN_POINT('Ctrl Pts',(-102.420352648489,3.99536898529432,
136.555478838857));
#239713=CARTESIAN_POINT('Ctrl Pts',(-102.698800272302,6.99817316856906,
130.551563412989));
#239714=CARTESIAN_POINT('Ctrl Pts',(-102.977247896115,3.56999808969468,
124.779956268296));
#239715=CARTESIAN_POINT('Ctrl Pts',(-103.255695519928,-3.13883082950684,
124.544482412068));
#239716=CARTESIAN_POINT('Ctrl Pts',(-103.53414314374,-6.96322755680218,
130.061530814641));
#239717=CARTESIAN_POINT('Ctrl Pts',(-103.812590767553,-4.38875833197407,
136.261203516848));
#239718=CARTESIAN_POINT('Ctrl Pts',(-104.091038391366,2.21876539717438,
137.44630417621));
#239719=CARTESIAN_POINT('Ctrl Pts',(-104.369486015179,6.78735211903507,
132.52778318216));
#239720=CARTESIAN_POINT('Ctrl Pts',(-104.647933638992,5.11869382408742,
126.02552104512));
#239721=CARTESIAN_POINT('Ctrl Pts',(-104.926381262805,-1.25379403310144,
123.914779015865));
#239722=CARTESIAN_POINT('Ctrl Pts',(-105.204828886617,-6.47410642511416,
128.135225903801));
#239723=CARTESIAN_POINT('Ctrl Pts',(-105.483276510431,-5.74503129012806,
134.808477199207));
#239724=CARTESIAN_POINT('Ctrl Pts',(-105.761724134243,0.263446940103889,
137.802140968053));
#239725=CARTESIAN_POINT('Ctrl Pts',(-106.040171758056,6.02983030247923,
134.365186455377));
#239726=CARTESIAN_POINT('Ctrl Pts',(-106.318619381869,6.25509419046252,
127.656006953765));
#239727=CARTESIAN_POINT('Ctrl Pts',(-106.597067005682,0.732232095750508,
123.840010663559));
#239728=CARTESIAN_POINT('Ctrl Pts',(-106.875514629495,-5.46351552342998,
126.423911753675));
#239729=CARTESIAN_POINT('Ctrl Pts',(-107.153962253308,-6.63855928414971,
133.033231352883));
#239730=CARTESIAN_POINT('Ctrl Pts',(-107.432409877121,-1.71309137438684,
137.594327632723));
#239731=CARTESIAN_POINT('Ctrl Pts',(-107.710857500934,4.78662381927155,
135.915775933963));
#239732=CARTESIAN_POINT('Ctrl Pts',(-107.989305124746,6.8876655625929,129.540083265954));
#239733=CARTESIAN_POINT('Ctrl Pts',(-108.26775274856,2.65927913505975,124.326199720693));
#239734=CARTESIAN_POINT('Ctrl Pts',(-108.546200372372,-4.0128549045848,
125.065429563905));
#239735=CARTESIAN_POINT('Ctrl Pts',(-108.824647996185,-6.99737132577695,
131.078456683062));
#239736=CARTESIAN_POINT('Ctrl Pts',(-109.103095619998,-3.5516453391731,
136.839602908365));
#239737=CARTESIAN_POINT('Ctrl Pts',(-109.381543243811,3.1578692066097,137.054656306401));
#239738=CARTESIAN_POINT('Ctrl Pts',(-109.659990867624,6.96545622200577,
131.525993310316));
#239739=CARTESIAN_POINT('Ctrl Pts',(-109.938438491437,4.37212925083209,
125.334185123311));
#239740=CARTESIAN_POINT('Ctrl Pts',(-110.21688611525,-2.23897091146772,
124.169200982596));
#239741=CARTESIAN_POINT('Ctrl Pts',(-110.495333739063,-6.79256618593892,
129.10160440085));
#239742=CARTESIAN_POINT('Ctrl Pts',(-110.773781362875,-5.10412497083799,
135.598757597999));
#239743=CARTESIAN_POINT('Ctrl Pts',(-111.052228986688,1.27475774209554,
137.690094189444));
#239744=CARTESIAN_POINT('Ctrl Pts',(-111.330676610501,6.48220036542147,
133.453778015119));
#239745=CARTESIAN_POINT('Ctrl Pts',(-111.609124234314,5.73281752601749,
126.782776683677));
#239746=CARTESIAN_POINT('Ctrl Pts',(-111.887571858127,-0.284744556090853,
123.807414522182));
#239747=CARTESIAN_POINT('Ctrl Pts',(-112.16601948194,-6.04064030169634,
127.261904002525));
#239748=CARTESIAN_POINT('Ctrl Pts',(-112.444467105753,-6.24548271172772,
133.971738053464));
#239749=CARTESIAN_POINT('Ctrl Pts',(-112.722914729566,-0.71103161847358,
137.770906975801));
#239750=CARTESIAN_POINT('Ctrl Pts',(-113.001362353379,5.47682279633179,
135.16816012963));
#239751=CARTESIAN_POINT('Ctrl Pts',(-113.279809977192,6.63174461897671,
128.55529471533));
#239752=CARTESIAN_POINT('Ctrl Pts',(-113.558257601004,1.69241711551747,
124.009210992206));
#239753=CARTESIAN_POINT('Ctrl Pts',(-113.836705224817,-4.80215903792943,
125.707537813274));
#239754=CARTESIAN_POINT('Ctrl Pts',(-114.11515284863,-6.88378563403075,
132.089595797848));
#239755=CARTESIAN_POINT('Ctrl Pts',(-114.393600472443,-2.63954952408134,
137.290585438973));
#239756=CARTESIAN_POINT('Ctrl Pts',(-114.672048096256,4.03030364933543,
136.531051338922));
#239757=CARTESIAN_POINT('Ctrl Pts',(-114.950495720069,6.99650466029252,
130.508968230339));
#239758=CARTESIAN_POINT('Ctrl Pts',(-115.228943343882,3.53325968669456,
124.758336294896));
#239759=CARTESIAN_POINT('Ctrl Pts',(-115.507390967695,-3.17687832964389,
124.563705347279));
#239760=CARTESIAN_POINT('Ctrl Pts',(-115.785838591507,-6.96762036017394,
130.103931720095));
#239761=CARTESIAN_POINT('Ctrl Pts',(-116.06428621532,-4.35545966688232,
136.287818031834));
#239762=CARTESIAN_POINT('Ctrl Pts',(-116.342733839133,2.25915568424066,
137.432674861647));
#239763=CARTESIAN_POINT('Ctrl Pts',(-116.621181462946,6.79771732743703,
132.486434712303));
#239764=CARTESIAN_POINT('Ctrl Pts',(-116.899629086759,5.08950883367243,
125.994450643782));
#239765=CARTESIAN_POINT('Ctrl Pts',(-117.178076710572,-1.2957096419083,
123.922538864004));
#239766=CARTESIAN_POINT('Ctrl Pts',(-117.456524334385,-6.49023425551004,
128.174685080065));
#239767=CARTESIAN_POINT('Ctrl Pts',(-117.734971958198,-5.7205506538686,
134.843374648297));
#239768=CARTESIAN_POINT('Ctrl Pts',(-118.013419582011,0.306039534242538,
137.800407639092));
#239769=CARTESIAN_POINT('Ctrl Pts',(-118.291867205823,6.05139434124684,
134.328415193001));
#239770=CARTESIAN_POINT('Ctrl Pts',(-118.570314829636,6.23581337569426,
127.617988751722));
#239771=CARTESIAN_POINT('Ctrl Pts',(-118.848762453449,0.689824554297045,
123.835682392233));
#239772=CARTESIAN_POINT('Ctrl Pts',(-119.127210077262,-5.49007933269568,
126.457250882969));
#239773=CARTESIAN_POINT('Ctrl Pts',(-119.405657701075,-6.62486851822702,
133.073600851681));
#239774=CARTESIAN_POINT('Ctrl Pts',(-119.684105324888,-1.67172717832737,
137.60462990379));
#239775=CARTESIAN_POINT('Ctrl Pts',(-119.962552948701,4.81764977004229,
135.886543693482));
#239776=CARTESIAN_POINT('Ctrl Pts',(-120.241000572514,6.87984193501854,
129.498179514853));
#239777=CARTESIAN_POINT('Ctrl Pts',(-120.519448196327,2.61979546067638,
124.310131959122));
#239778=CARTESIAN_POINT('Ctrl Pts',(-120.79789582014,-4.04771505790416,
125.089963279793));
#239779=CARTESIAN_POINT('Ctrl Pts',(-121.076343443952,-6.9955731801444,
131.121046590047));
#239780=CARTESIAN_POINT('Ctrl Pts',(-121.354791067765,-3.51484130258126,
136.86111096256));
#239781=CARTESIAN_POINT('Ctrl Pts',(-121.633238691578,3.19585802251066,
137.035317656727));
#239782=CARTESIAN_POINT('Ctrl Pts',(-121.911686315391,6.96971995125911,
131.483579231079));
#239783=CARTESIAN_POINT('Ctrl Pts',(-122.190133939204,4.3387497345494,125.307672081285));
#239784=CARTESIAN_POINT('Ctrl Pts',(-122.468581563017,-2.2793195285039,
124.182953168171));
#239785=CARTESIAN_POINT('Ctrl Pts',(-122.74702918683,-6.80280549581075,
129.142984227312));
#239786=CARTESIAN_POINT('Ctrl Pts',(-123.025476810643,-5.07484554799192,
135.629739026348));
#239787=CARTESIAN_POINT('Ctrl Pts',(-123.303924434456,1.31664953844379,
137.682206800553));
#239788=CARTESIAN_POINT('Ctrl Pts',(-123.582372058268,6.49820802095541,
133.414269934058));
#239789=CARTESIAN_POINT('Ctrl Pts',(-123.860819682081,5.7082307873194,126.747953906865));
#239790=CARTESIAN_POINT('Ctrl Pts',(-124.139267305894,-0.327331677286216,
123.809277480321));
#239791=CARTESIAN_POINT('Ctrl Pts',(-124.417714929707,-6.06209232150722,
127.298740728095));
#239792=CARTESIAN_POINT('Ctrl Pts',(-124.69616255352,-6.22608627193705,
134.009697395242));
#239793=CARTESIAN_POINT('Ctrl Pts',(-124.974610177333,-0.668611099680587,
137.77510615311));
#239794=CARTESIAN_POINT('Ctrl Pts',(-125.253057801146,5.50328500971429,
135.134740303665));
#239795=CARTESIAN_POINT('Ctrl Pts',(-125.531505424959,6.61793104560076,
128.514967073503));
#239796=CARTESIAN_POINT('Ctrl Pts',(-125.809953048772,1.6510217544855,123.999034667242));
#239797=CARTESIAN_POINT('Ctrl Pts',(-126.088400672584,-4.8330958721059,
125.736864350674));
#239798=CARTESIAN_POINT('Ctrl Pts',(-126.366848296398,-6.87583450209069,
132.131475542423));
#239799=CARTESIAN_POINT('Ctrl Pts',(-126.64529592021,-2.60001712784396,
137.306532951397));
#239800=CARTESIAN_POINT('Ctrl Pts',(-126.923743544023,4.06508896899354,
136.506411634357));
#239801=CARTESIAN_POINT('Ctrl Pts',(-127.202191167836,6.99457689396224,
130.466383993564));
#239802=CARTESIAN_POINT('Ctrl Pts',(-127.480638791649,3.49639035745773,
124.736940359153));
#239803=CARTESIAN_POINT('Ctrl Pts',(-127.759086415462,-3.21480810938582,
124.583159532264));
#239804=CARTESIAN_POINT('Ctrl Pts',(-128.037534039275,-6.97175497581086,
130.146358580199));
#239805=CARTESIAN_POINT('Ctrl Pts',(-128.315981663087,-4.32199960863106,
136.314229355287));
#239806=CARTESIAN_POINT('Ctrl Pts',(-128.594429286901,2.29946225746178,
137.418799932461));
#239807=CARTESIAN_POINT('Ctrl Pts',(-128.872876910713,6.80783064392392,
132.44502391257));
#239808=CARTESIAN_POINT('Ctrl Pts',(-129.151324534526,5.06013524963555,
125.963558475429));
#239809=CARTESIAN_POINT('Ctrl Pts',(-129.429772158339,-1.33757723771771,
123.930553720578));
#239810=CARTESIAN_POINT('Ctrl Pts',(-129.708219782152,-6.50612158788957,
128.214241699924));
#239811=CARTESIAN_POINT('Ctrl Pts',(-129.986667405965,-5.69585804050008,
134.878122430239));
#239812=CARTESIAN_POINT('Ctrl Pts',(-130.265115029778,0.348620787973942,
137.798415069035));
#239813=CARTESIAN_POINT('Ctrl Pts',(-130.543562653591,6.07273414337257,
134.291513345486));
#239814=CARTESIAN_POINT('Ctrl Pts',(-130.822010277403,6.21630149056731,
127.58008862186));
#239815=CARTESIAN_POINT('Ctrl Pts',(-131.100457901217,0.647391451141708,
123.831612347843));
#239816=CARTESIAN_POINT('Ctrl Pts',(-131.378905525029,-5.5164397050528,
126.490751096011));
#239817=CARTESIAN_POINT('Ctrl Pts',(-131.657353148842,-6.61093226536518,
133.113886262947));
#239818=CARTESIAN_POINT('Ctrl Pts',(-131.935800772655,-1.63030103580305,
137.614680188378));
#239819=CARTESIAN_POINT('Ctrl Pts',(-132.214248396468,4.848497201029,135.857123130838));
#239820=CARTESIAN_POINT('Ctrl Pts',(-132.492696020281,6.87176337237162,
129.456324164773));
#239821=CARTESIAN_POINT('Ctrl Pts',(-132.771143644094,2.58021470880796,
124.294304843582));
#239822=CARTESIAN_POINT('Ctrl Pts',(-133.049591267907,-4.08242522165371,
125.114708744776));
#239823=CARTESIAN_POINT('Ctrl Pts',(-133.32803889172,-6.99351581097555,
131.163624762118));
#239824=CARTESIAN_POINT('Ctrl Pts',(-133.606486515532,-3.47790702225152,
136.882394581644));
#239825=CARTESIAN_POINT('Ctrl Pts',(-133.884934139345,3.23372841471757,
137.015748116649));
#239826=CARTESIAN_POINT('Ctrl Pts',(-134.163381763158,6.97372541497715,
131.441139983145));
#239827=CARTESIAN_POINT('Ctrl Pts',(-134.441829386971,4.30520944429882,
125.281362721075));
#239828=CARTESIAN_POINT('Ctrl Pts',(-134.720277010784,-2.31958368451587,
124.196950712432));
#239829=CARTESIAN_POINT('Ctrl Pts',(-134.998724634597,-6.81279272522359,
129.184425616688));
#239830=CARTESIAN_POINT('Ctrl Pts',(-135.27717225841,-5.04537807487797,
135.660541648527));
#239831=CARTESIAN_POINT('Ctrl Pts',(-135.555619882223,1.35849254585843,
137.674064550544));
#239832=CARTESIAN_POINT('Ctrl Pts',(-135.834067506036,6.51397488300169,
133.374665141848));
#239833=CARTESIAN_POINT('Ctrl Pts',(-136.112515129848,5.68343252803032,
126.713281441693));
#239834=CARTESIAN_POINT('Ctrl Pts',(-136.390962753662,-0.369906669086523,
123.811399643837));
#239835=CARTESIAN_POINT('Ctrl Pts',(-136.669410377474,-6.08331970825794,
127.335707355701));
#239836=CARTESIAN_POINT('Ctrl Pts',(-136.947858001288,-6.20645912223011,
134.047537962086));
#239837=CARTESIAN_POINT('Ctrl Pts',(-137.2263056251,-0.626165805256695,
137.779047026878));
#239838=CARTESIAN_POINT('Ctrl Pts',(-137.504753248913,5.52954329684707,
135.101160013885));
#239839=CARTESIAN_POINT('Ctrl Pts',(-137.783200872726,6.60387224235649,
128.474724265995));
#239840=CARTESIAN_POINT('Ctrl Pts',(-138.061648496539,1.60956521423443,
123.989110516135));
#239841=CARTESIAN_POINT('Ctrl Pts',(-138.340096120352,-4.86385361413656,
125.766378666012));
#239842=CARTESIAN_POINT('Ctrl Pts',(-138.618543744165,-6.86762858357524,
132.173306110266));
#239843=CARTESIAN_POINT('Ctrl Pts',(-138.896991367977,-2.56038838701599,
137.322239523433));
#239844=CARTESIAN_POINT('Ctrl Pts',(-139.17543899179,4.09972365528409,136.481560638194));
#239845=CARTESIAN_POINT('Ctrl Pts',(-139.453886615603,6.99238994101352,
130.423812280637));
#239846=CARTESIAN_POINT('Ctrl Pts',(-139.732334239416,3.45939146819007,
124.715769253897));
#239847=CARTESIAN_POINT('Ctrl Pts',(-140.010781863229,-3.25261876323132,
124.602844246145));
#239848=CARTESIAN_POINT('Ctrl Pts',(-140.289229487042,-6.97563125050334,
130.188809822811));
#239849=CARTESIAN_POINT('Ctrl Pts',(-140.567677110855,-4.28837939709471,
136.340436508528));
#239850=CARTESIAN_POINT('Ctrl Pts',(-140.846124734668,2.33968362326381,
137.404679902793));
#239851=CARTESIAN_POINT('Ctrl Pts',(-141.124572358481,6.81769169374202,
132.403552317457));
#239852=CARTESIAN_POINT('Ctrl Pts',(-141.403019982293,5.03057416042698,
125.932845684778));
#239853=CARTESIAN_POINT('Ctrl Pts',(-141.681467606106,-1.37939526911043,
123.938823288595));
#239854=CARTESIAN_POINT('Ctrl Pts',(-141.959915229919,-6.52176783354029,
128.253894297592));
#239855=CARTESIAN_POINT('Ctrl Pts',(-142.238362853732,-5.67095436501806,
134.912719257437));
#239856=CARTESIAN_POINT('Ctrl Pts',(-142.516810477545,0.39118912343359,
137.796163331718));
#239857=CARTESIAN_POINT('Ctrl Pts',(-142.795258101358,6.09384891810056,
134.254482280245));
#239858=CARTESIAN_POINT('Ctrl Pts',(-143.073705725171,6.19655925810344,
127.542307968582));
#239859=CARTESIAN_POINT('Ctrl Pts',(-143.352153348984,0.604934358657401,
123.827800681205));
#239860=CARTESIAN_POINT('Ctrl Pts',(-143.630600972796,-5.54259566370794,
126.524411151443));
#239861=CARTESIAN_POINT('Ctrl Pts',(-143.90904859661,-6.59675104197701,
133.154086093891));
#239862=CARTESIAN_POINT('Ctrl Pts',(-144.187496220422,-1.58881448187379,
137.624478114069));
#239863=CARTESIAN_POINT('Ctrl Pts',(-144.465943844235,4.87916496916901,
135.827515336221));
#239864=CARTESIAN_POINT('Ctrl Pts',(-144.744391468048,6.86343017400547,
129.41451876668));
#239865=CARTESIAN_POINT('Ctrl Pts',(-145.022839091861,2.54053834613545,
124.278718960552));
#239866=CARTESIAN_POINT('Ctrl Pts',(-145.301286715674,-4.11698410963516,
125.139665041902));
#239867=CARTESIAN_POINT('Ctrl Pts',(-145.579734339487,-6.99119929450595,
131.206189621523));
#239868=CARTESIAN_POINT('Ctrl Pts',(-145.8581819633,-3.44084386679896,136.903452976945));
#239869=CARTESIAN_POINT('Ctrl Pts',(-146.136629587113,3.27147897992919,
136.995948411323));
#239870=CARTESIAN_POINT('Ctrl Pts',(-146.415077210925,6.97747246473481,
131.398677139117));
#239871=CARTESIAN_POINT('Ctrl Pts',(-146.693524834738,4.27150962292939,
125.255258017582));
#239872=CARTESIAN_POINT('Ctrl Pts',(-146.971972458551,-2.35976188750221,
124.211193096699));
#239873=CARTESIAN_POINT('Ctrl Pts',(-147.250420082364,-6.82252750409623,
129.225927033352));
#239874=CARTESIAN_POINT('Ctrl Pts',(-147.528867706177,-5.01572364342383,
135.69116432313));
#239875=CARTESIAN_POINT('Ctrl Pts',(-147.80731532999,1.40028521383297,137.665667741127));
#239876=CARTESIAN_POINT('Ctrl Pts',(-148.085762953803,6.52950036731291,
133.334965106058));
#239877=CARTESIAN_POINT('Ctrl Pts',(-148.364210577616,5.65842366705879,
126.678760572968));
#239878=CARTESIAN_POINT('Ctrl Pts',(-148.642658201429,-0.412467953858535,
123.813780934094));
#239879=CARTESIAN_POINT('Ctrl Pts',(-148.921105825242,-6.10432167535963,
127.372802515528));
#239880=CARTESIAN_POINT('Ctrl Pts',(-149.199553449054,-6.18660198989778,
134.085258351801));
#239881=CARTESIAN_POINT('Ctrl Pts',(-149.478001072867,-0.583697308029368,
137.782729451077));
#239882=CARTESIAN_POINT('Ctrl Pts',(-149.75644869668,5.55559668471987,135.067420504625));
#239883=CARTESIAN_POINT('Ctrl Pts',(-150.034896320493,6.58956873019717,
128.434567784019));
#239884=CARTESIAN_POINT('Ctrl Pts',(-150.313343944306,1.56804903095274,
123.979438906626));
#239885=CARTESIAN_POINT('Ctrl Pts',(-150.591791568119,-4.89443112428377,
125.796079665625));
#239886=CARTESIAN_POINT('Ctrl Pts',(-150.870239191931,-6.85916818255639,
132.21508595133));
#239887=CARTESIAN_POINT('Ctrl Pts',(-151.148686815745,-2.52066477005453,
137.33770457307));
#239888=CARTESIAN_POINT('Ctrl Pts',(-151.427134439557,4.13420642480782,
136.456499271296));
#239889=CARTESIAN_POINT('Ctrl Pts',(-151.705582063371,6.98994388248347,
130.381254669068));
#239890=CARTESIAN_POINT('Ctrl Pts',(-151.984029687183,3.42226438989971,
124.694823763634));
#239891=CARTESIAN_POINT('Ctrl Pts',(-152.262477310996,-3.29030889009209,
124.622758759495));
#239892=CARTESIAN_POINT('Ctrl Pts',(-152.540924934809,-6.97924904061452,
130.231283874884));
#239893=CARTESIAN_POINT('Ctrl Pts',(-152.819372558622,-4.25460027808296,
136.366438520441));
#239894=CARTESIAN_POINT('Ctrl Pts',(-153.097820182435,2.37981829122829,
137.390315295868));
#239895=CARTESIAN_POINT('Ctrl Pts',(-153.376267806248,6.82730011148789,
132.362021463707));
#239896=CARTESIAN_POINT('Ctrl Pts',(-153.654715430061,5.00082666144207,
125.902313409905));
#239897=CARTESIAN_POINT('Ctrl Pts',(-153.933163053873,-1.42116218650446,
123.947347261623));
#239898=CARTESIAN_POINT('Ctrl Pts',(-154.211610677687,-6.53717241268631,
128.293641403726));
#239899=CARTESIAN_POINT('Ctrl Pts',(-154.490058301499,-5.64584055023574,
134.947163847896));
#239900=CARTESIAN_POINT('Ctrl Pts',(-154.768505925312,0.433742963236675,
137.79365251058));
#239901=CARTESIAN_POINT('Ctrl Pts',(-155.046953549125,6.11473788301669,
134.217323369476));
#239902=CARTESIAN_POINT('Ctrl Pts',(-155.325401172938,6.17658740985663,
127.504648191865));
#239903=CARTESIAN_POINT('Ctrl Pts',(-155.603848796751,0.562454850108638,
123.824247533559));
#239904=CARTESIAN_POINT('Ctrl Pts',(-155.882296420564,-5.5685462394425,
126.558229801974));
#239905=CARTESIAN_POINT('Ctrl Pts',(-156.160744044376,-6.5823253735531,
133.194198854895));
#239906=CARTESIAN_POINT('Ctrl Pts',(-156.43919166819,-1.54726905384013,
137.634023317798));
#239907=CARTESIAN_POINT('Ctrl Pts',(-156.717639292002,4.90965193805665,
135.79772140676));
#239908=CARTESIAN_POINT('Ctrl Pts',(-156.996086915816,6.8548426487106,129.372764869687));
#239909=CARTESIAN_POINT('Ctrl Pts',(-157.274534539628,2.50076784287941,
124.263374887574));
#239910=CARTESIAN_POINT('Ctrl Pts',(-157.552982163441,-4.15139044125659,
125.164831246407));
#239911=CARTESIAN_POINT('Ctrl Pts',(-157.831429787254,-6.98862371657603,
131.248739591007));
#239912=CARTESIAN_POINT('Ctrl Pts',(-158.109877411067,-3.40365320961064,
136.924285368134));
#239913=CARTESIAN_POINT('Ctrl Pts',(-158.38832503488,3.30910831928323,136.975919274434));
#239914=CARTESIAN_POINT('Ctrl Pts',(-158.666772658693,6.98096096168483,
131.356192272474));
#239915=CARTESIAN_POINT('Ctrl Pts',(-158.945220282506,4.23765151920024,
125.229358938127));
#239916=CARTESIAN_POINT('Ctrl Pts',(-159.223667906319,-2.39985264864321,
124.225679793212));
#239917=CARTESIAN_POINT('Ctrl Pts',(-159.502115530131,-6.8320094717036,
129.267486939452));
#239918=CARTESIAN_POINT('Ctrl Pts',(-159.780563153944,-4.98588335248574,
135.721605915426));
#239919=CARTESIAN_POINT('Ctrl Pts',(-160.059010777757,1.44202599372318,
137.657016683454));
#239920=CARTESIAN_POINT('Ctrl Pts',(-160.33745840157,6.54478389858708,133.295171297791));
#239921=CARTESIAN_POINT('Ctrl Pts',(-160.615906025383,5.63320513111742,
126.644392579866));
#239922=CARTESIAN_POINT('Ctrl Pts',(-160.894353649196,-0.455013954479453,
123.816421262852));
#239923=CARTESIAN_POINT('Ctrl Pts',(-161.172801273009,-6.12509744457689,
127.410024833003));
#239924=CARTESIAN_POINT('Ctrl Pts',(-161.451248896821,-6.16651561075379,
134.122857166646));
#239925=CARTESIAN_POINT('Ctrl Pts',(-161.729696520635,-0.541207181682879,
137.786153289251));
#239926=CARTESIAN_POINT('Ctrl Pts',(-162.008144144447,5.58144420791359,
135.033523026113));
#239927=CARTESIAN_POINT('Ctrl Pts',(-162.286591768261,6.57502103914602,
128.394499115588));
#239928=CARTESIAN_POINT('Ctrl Pts',(-162.565039392073,1.52647474303778,
123.970020197102));
#239929=CARTESIAN_POINT('Ctrl Pts',(-162.843487015886,-4.92482726948487,
125.825966248931));
#239930=CARTESIAN_POINT('Ctrl Pts',(-163.121934639699,-6.85045361253876,
132.256813517449));
#239931=CARTESIAN_POINT('Ctrl Pts',(-163.400382263512,-2.48084774893327,
137.352927527244));
#239932=CARTESIAN_POINT('Ctrl Pts',(-163.678829887325,4.16853599979124,
136.431228462323));
#239933=CARTESIAN_POINT('Ctrl Pts',(-163.957277511138,6.98723880901292,
130.338712735846));
#239934=CARTESIAN_POINT('Ctrl Pts',(-164.23572513495,3.3850104983435,124.674104664506));
#239935=CARTESIAN_POINT('Ctrl Pts',(-164.514172758764,-3.32787709334726,
124.642902334375));
#239936=CARTESIAN_POINT('Ctrl Pts',(-164.792620382576,-6.98260821208591,
130.273779162525));
#239937=CARTESIAN_POINT('Ctrl Pts',(-165.07106800639,-4.22066350329308,
136.392234427513));
#239938=CARTESIAN_POINT('Ctrl Pts',(-165.349515630202,2.4198647741513,137.37570664397));
#239939=CARTESIAN_POINT('Ctrl Pts',(-165.627963254015,6.83665554111671,
132.320432890263));
#239940=CARTESIAN_POINT('Ctrl Pts',(-165.906410877828,4.97089385498702,
125.871962782194));
#239941=CARTESIAN_POINT('Ctrl Pts',(-166.184858501641,-1.46287644221077,
123.956125323802));
#239942=CARTESIAN_POINT('Ctrl Pts',(-166.463306125454,-6.55233475450377,
128.333481545486));
#239943=CARTESIAN_POINT('Ctrl Pts',(-166.741753749267,-5.62051752675643,
134.981454925258));
#239944=CARTESIAN_POINT('Ctrl Pts',(-167.020201373079,0.476280730534997,
137.790882698662));
#239945=CARTESIAN_POINT('Ctrl Pts',(-167.298648996893,6.13540026407138,
134.180037990117));
#239946=CARTESIAN_POINT('Ctrl Pts',(-167.577096620705,6.15638668589229,
127.467110687205));
#239947=CARTESIAN_POINT('Ctrl Pts',(-167.855544244518,0.519954499587912,
123.820953036571));
#239948=CARTESIAN_POINT('Ctrl Pts',(-168.133991868331,-5.5942904706483,
126.592205794446));
#239949=CARTESIAN_POINT('Ctrl Pts',(-168.412439492144,-6.56765579464175,
133.234223059563));
#239950=CARTESIAN_POINT('Ctrl Pts',(-168.690887115956,-1.50566629118217,
137.643315445865));
#239951=CARTESIAN_POINT('Ctrl Pts',(-168.96933473977,4.93995697798634,135.767742446477));
#239952=CARTESIAN_POINT('Ctrl Pts',(-169.247782363582,6.84600111470013,
129.331064021001));
#239953=CARTESIAN_POINT('Ctrl Pts',(-169.526229987396,2.46090467275213,
124.248273193229));
#239954=CARTESIAN_POINT('Ctrl Pts',(-169.804677611208,-4.18564294157836,
125.190206425745));
#239955=CARTESIAN_POINT('Ctrl Pts',(-170.083125235021,-6.98578917262369,
131.291273093865));
#239956=CARTESIAN_POINT('Ctrl Pts',(-170.361572858834,-3.36633642880185,
136.944890983262));
#239957=CARTESIAN_POINT('Ctrl Pts',(-170.640020482647,3.34661503841248,
136.955661448171));
#239958=CARTESIAN_POINT('Ctrl Pts',(-170.91846810646,6.98419077655865,131.313686957504));
#239959=CARTESIAN_POINT('Ctrl Pts',(-171.196915730273,4.20363638773547,
125.203666442409));
#239960=CARTESIAN_POINT('Ctrl Pts',(-171.475363354086,-2.43985448236259,
124.240410265162));
#239961=CARTESIAN_POINT('Ctrl Pts',(-171.753810977898,-6.84123827668714,
129.309103794972));
#239962=CARTESIAN_POINT('Ctrl Pts',(-172.032258601712,-4.9558583078063,
135.751865297389));
#239963=CARTESIAN_POINT('Ctrl Pts',(-172.310706225524,1.48371333881067,
137.648111698089));
#239964=CARTESIAN_POINT('Ctrl Pts',(-172.589153849337,6.55982491048677,
133.255285191615));
#239965=CARTESIAN_POINT('Ctrl Pts',(-172.86760147315,5.60777785468832,126.610178735912));
#239966=CARTESIAN_POINT('Ctrl Pts',(-173.146049096963,-0.497543094390354,
123.819320532272));
#239967=CARTESIAN_POINT('Ctrl Pts',(-173.424496720776,-6.14564624605571,
127.447372928838));
#239968=CARTESIAN_POINT('Ctrl Pts',(-173.702944344589,-6.14620072910595,
134.160333013378));
#239969=CARTESIAN_POINT('Ctrl Pts',(-173.981391968402,-0.498697000705985,
137.789318414533));
#239970=CARTESIAN_POINT('Ctrl Pts',(-174.259839592215,5.60708490864046,
134.999468834432));
#239971=CARTESIAN_POINT('Ctrl Pts',(-174.538287216028,6.56022970827155,
128.354519745462));
#239972=CARTESIAN_POINT('Ctrl Pts',(-174.81673483984,1.48484389103961,123.960854736574));
#239973=CARTESIAN_POINT('Ctrl Pts',(-175.095182463654,-4.95504092340126,
125.85603730847));
#239974=CARTESIAN_POINT('Ctrl Pts',(-175.373630087466,-6.8414851964426,
132.298487262391));
#239975=CARTESIAN_POINT('Ctrl Pts',(-175.652077711279,-2.44093879908611,
137.367907821863));
#239976=CARTESIAN_POINT('Ctrl Pts',(-175.930525335092,4.20271110814107,
136.405749147692));
#239977=CARTESIAN_POINT('Ctrl Pts',(-176.208972958905,6.98427482083815,
130.296188057377));
#239978=CARTESIAN_POINT('Ctrl Pts',(-176.487420582718,3.3476311739788,124.653612724266));
#239979=CARTESIAN_POINT('Ctrl Pts',(-176.765868206531,-3.36532198089259,
124.663274224357));
#239980=CARTESIAN_POINT('Ctrl Pts',(-177.044315830343,-6.98570864044213,
130.316294111058));
#239981=CARTESIAN_POINT('Ctrl Pts',(-177.322763454156,-4.18657033026512,
136.417823273865));
#239982=CARTESIAN_POINT('Ctrl Pts',(-177.601211077969,2.4598215880947,137.360854488428));
#239983=CARTESIAN_POINT('Ctrl Pts',(-177.879658701782,6.84575763596098,
132.278788138201));
#239984=CARTESIAN_POINT('Ctrl Pts',(-178.158106325595,4.94077685023126,
125.841794926299));
#239985=CARTESIAN_POINT('Ctrl Pts',(-178.436553949408,-1.50453649049278,
123.965157149858));
#239986=CARTESIAN_POINT('Ctrl Pts',(-178.715001573221,-6.56725429714808,
128.373413246577));
#239987=CARTESIAN_POINT('Ctrl Pts',(-178.993449197033,-5.59498623293233,
135.015591218853));
#239988=CARTESIAN_POINT('Ctrl Pts',(-179.271896820847,0.518800849074927,
137.787853998597));
#239989=CARTESIAN_POINT('Ctrl Pts',(-179.550344444659,6.15583529561319,
134.142627523792));
#239990=CARTESIAN_POINT('Ctrl Pts',(-179.828792068472,6.13595783475539,
127.429696845569));
#239991=CARTESIAN_POINT('Ctrl Pts',(-180.107239692285,0.477434881962636,
123.81791731232));
#239992=CARTESIAN_POINT('Ctrl Pts',(-180.385687316098,-5.61982740336347,
126.626337869861));
#239993=CARTESIAN_POINT('Ctrl Pts',(-180.664134939911,-6.55274284882976,
133.274157224785));
#239994=CARTESIAN_POINT('Ctrl Pts',(-180.942582563724,-1.4640077355066,
137.652354153945));
#239995=CARTESIAN_POINT('Ctrl Pts',(-181.221030187537,4.97007896599344,
135.737579566256));
#239996=CARTESIAN_POINT('Ctrl Pts',(-181.499477811349,6.83690589960112,
129.289417765863));
#239997=CARTESIAN_POINT('Ctrl Pts',(-181.777925435163,2.42095031289641,
124.233414437113));
#239998=CARTESIAN_POINT('Ctrl Pts',(-182.056373058975,-4.21974034136189,
125.215789639631));
#239999=CARTESIAN_POINT('Ctrl Pts',(-182.334820682789,-6.98269576768506,
131.333788554001));
#240000=CARTESIAN_POINT('Ctrl Pts',(-182.613268306601,-3.32889490715784,
136.965269058779));
#240001=CARTESIAN_POINT('Ctrl Pts',(-182.891715930414,3.38399774748988,
136.935175683191));
#240002=CARTESIAN_POINT('Ctrl Pts',(-183.170163554227,6.98716178967534,
131.27116276926));
#240003=CARTESIAN_POINT('Ctrl Pts',(-183.44861117804,4.16946548897866,125.178181482475));
#240004=CARTESIAN_POINT('Ctrl Pts',(-183.727058801853,-2.47976590637605,
124.255383966707));
#240005=CARTESIAN_POINT('Ctrl Pts',(-184.005506425666,-6.85021357707087,
129.350776057783));
#240006=CARTESIAN_POINT('Ctrl Pts',(-184.283954049479,-4.92564962197493,
135.781941347746));
#240007=CARTESIAN_POINT('Ctrl Pts',(-184.562401673291,1.52534570435398,
137.63895311501));
#240008=CARTESIAN_POINT('Ctrl Pts',(-184.840849297105,6.5746228456623,133.215308265529));
#240009=CARTESIAN_POINT('Ctrl Pts',(-185.119296920917,5.58214277998856,
126.576120308909));
#240010=CARTESIAN_POINT('Ctrl Pts',(-185.39774454473,-0.540053797659538,
123.822478634922));
#240011=CARTESIAN_POINT('Ctrl Pts',(-185.676192168543,-6.16596731835295,
127.484845419088));
#240012=CARTESIAN_POINT('Ctrl Pts',(-185.954639792356,-6.12565809773001,
134.197684503321));
#240013=CARTESIAN_POINT('Ctrl Pts',(-186.233087416169,-0.456168340327589,
137.792224709632));
#240014=CARTESIAN_POINT('Ctrl Pts',(-186.511535039982,5.63251783677319,
134.965259191474));
#240015=CARTESIAN_POINT('Ctrl Pts',(-186.789982663795,6.54519528567348,
128.314631155089));
#240016=CARTESIAN_POINT('Ctrl Pts',(-187.068430287608,1.44315801760525,
123.951942864674));
#240017=CARTESIAN_POINT('Ctrl Pts',(-187.346877911421,-4.98507096645316,
125.886291729948));
#240018=CARTESIAN_POINT('Ctrl Pts',(-187.625325535233,-6.83226326659722,
132.340105641921));
#240019=CARTESIAN_POINT('Ctrl Pts',(-187.903773159046,-2.40093939935397,
137.382644901827));
#240020=CARTESIAN_POINT('Ctrl Pts',(-188.182220782859,4.23673048348491,
136.380062271549));
#240021=CARTESIAN_POINT('Ctrl Pts',(-188.460668406672,6.98105202779173,
130.25368220943));
#240022=CARTESIAN_POINT('Ctrl Pts',(-188.739116030485,3.31012780190951,
124.633348702251));
#240023=CARTESIAN_POINT('Ctrl Pts',(-189.017563654298,-3.40264216519462,
124.683873674555));
#240024=CARTESIAN_POINT('Ctrl Pts',(-189.296011278111,-6.98855021079573,
130.358827145076));
#240025=CARTESIAN_POINT('Ctrl Pts',(-189.574458901924,-4.15232202233378,
136.443204111294));
#240026=CARTESIAN_POINT('Ctrl Pts',(-189.852906525736,2.49968725244504,
137.345759379595));
#240027=CARTESIAN_POINT('Ctrl Pts',(-190.13135414955,6.85460605873784,132.237088750687));
#240028=CARTESIAN_POINT('Ctrl Pts',(-190.409801773362,4.91047676317321,
125.8118109601));
#240029=CARTESIAN_POINT('Ctrl Pts',(-190.688249397175,-1.5461407876216,
123.974442405114));
#240030=CARTESIAN_POINT('Ctrl Pts',(-190.966697020988,-6.58193048776853,
128.413435027317));
#240031=CARTESIAN_POINT('Ctrl Pts',(-191.245144644801,-5.56924761483672,
135.049571463749));
#240032=CARTESIAN_POINT('Ctrl Pts',(-191.523592268614,0.561301743259386,
137.784566522618));
#240033=CARTESIAN_POINT('Ctrl Pts',(-191.802039892427,6.17604222041412,
134.105093356759));
#240034=CARTESIAN_POINT('Ctrl Pts',(-192.08048751624,6.11530161344434,127.39240805334));
#240035=CARTESIAN_POINT('Ctrl Pts',(-192.358935140053,0.43489757281158,
123.815140473294));
#240036=CARTESIAN_POINT('Ctrl Pts',(-192.637382763865,-5.64515609130746,
126.660624763449));
#240037=CARTESIAN_POINT('Ctrl Pts',(-192.915830387678,-6.53758708872167,
133.313999870785));
#240038=CARTESIAN_POINT('Ctrl Pts',(-193.194278011491,-1.42229493048546,
137.661139107108));
#240039=CARTESIAN_POINT('Ctrl Pts',(-193.472725635304,5.00001678589681,
135.707233883791));
#240040=CARTESIAN_POINT('Ctrl Pts',(-193.751173259117,6.82755734043935,
129.247827647489));
#240041=CARTESIAN_POINT('Ctrl Pts',(-194.02962088293,2.38090624383734,124.218799169824));
#240042=CARTESIAN_POINT('Ctrl Pts',(-194.308068506743,-4.25368137711504,
125.241579940071));
#240043=CARTESIAN_POINT('Ctrl Pts',(-194.586516130556,-6.97934361638637,
131.376284395991));
#240044=CARTESIAN_POINT('Ctrl Pts',(-194.864963754369,-3.29133003208973,
136.985418839569));
#240045=CARTESIAN_POINT('Ctrl Pts',(-195.143411378181,3.42125506128717,
136.914462738605));
#240046=CARTESIAN_POINT('Ctrl Pts',(-195.421859001994,6.98987389094189,
131.22862128349));
#240047=CARTESIAN_POINT('Ctrl Pts',(-195.700306625807,4.13514008914463,
125.152905002676));
#240048=CARTESIAN_POINT('Ctrl Pts',(-195.97875424962,-2.51958544175274,
124.270600342989));
#240049=CARTESIAN_POINT('Ctrl Pts',(-196.257201873433,-6.85893504027095,
129.392502183704));
#240050=CARTESIAN_POINT('Ctrl Pts',(-196.535649497246,-4.89525841438522,
135.811832952018));
#240051=CARTESIAN_POINT('Ctrl Pts',(-196.814097121059,1.56692154765205,
137.629541273595));
#240052=CARTESIAN_POINT('Ctrl Pts',(-197.092544744872,6.58917715577019,
133.175242000891));
#240053=CARTESIAN_POINT('Ctrl Pts',(-197.370992368684,5.55630085693524,
126.542218560906));
#240054=CARTESIAN_POINT('Ctrl Pts',(-197.649439992498,-0.582544489036021,
123.825895453776));
#240055=CARTESIAN_POINT('Ctrl Pts',(-197.92788761631,-6.18605990846357,
127.522440915193));
#240056=CARTESIAN_POINT('Ctrl Pts',(-198.206335240123,-6.10488847784037,
134.234910252398));
#240057=CARTESIAN_POINT('Ctrl Pts',(-198.484782863936,-0.413622776464342,
137.79487206686));
#240058=CARTESIAN_POINT('Ctrl Pts',(-198.763230487749,5.657742049887,134.930895364888));
#240059=CARTESIAN_POINT('Ctrl Pts',(-199.041678111562,6.52991832845634,
128.274834822558));
#240060=CARTESIAN_POINT('Ctrl Pts',(-199.320125735375,1.40141866741961,
123.943284911633));
#240061=CARTESIAN_POINT('Ctrl Pts',(-199.598573359188,-5.01491628586802,
125.916728392279));
#240062=CARTESIAN_POINT('Ctrl Pts',(-199.877020983,-6.82278816472322,132.381667113854));
#240063=CARTESIAN_POINT('Ctrl Pts',(-200.155468606814,-2.36085103192995,
137.397138221046));
#240064=CARTESIAN_POINT('Ctrl Pts',(-200.433916230626,4.27059286522247,
136.354168785731));
#240065=CARTESIAN_POINT('Ctrl Pts',(-200.712363854439,6.97757054929515,
130.211196767073));
#240066=CARTESIAN_POINT('Ctrl Pts',(-200.990811478252,3.27250177183757,
124.613313349352));
#240067=CARTESIAN_POINT('Ctrl Pts',(-201.269259102065,-3.43983626333961,
124.704699921646));
#240068=CARTESIAN_POINT('Ctrl Pts',(-201.547706725878,-6.9911328178512,
130.401376688499));
#240069=CARTESIAN_POINT('Ctrl Pts',(-201.826154349691,-4.1179198485831,
136.468375999304));
#240070=CARTESIAN_POINT('Ctrl Pts',(-202.104601973504,2.53946028996452,
137.330421876826));
#240071=CARTESIAN_POINT('Ctrl Pts',(-202.383049597317,6.86320048156709,
132.195336272904));
#240072=CARTESIAN_POINT('Ctrl Pts',(-202.66149722113,4.87999471659204,125.782011994664));
#240073=CARTESIAN_POINT('Ctrl Pts',(-202.939944844942,-1.5876877919352,
123.983980745501));
#240074=CARTESIAN_POINT('Ctrl Pts',(-203.218392468755,-6.59636278253501,
128.453545404684));
#240075=CARTESIAN_POINT('Ctrl Pts',(-203.496840092568,-5.54330262622176,
135.083394400798));
#240076=CARTESIAN_POINT('Ctrl Pts',(-203.775287716381,0.603781838200554,
137.781020392543));
#240077=CARTESIAN_POINT('Ctrl Pts',(-204.053735340194,6.19602028969954,
134.067436879861));
#240078=CARTESIAN_POINT('Ctrl Pts',(-204.332182964007,6.09441878738321,
127.355245692268));
#240079=CARTESIAN_POINT('Ctrl Pts',(-204.61063058782,0.392344148371673,
123.812622622391));
#240080=CARTESIAN_POINT('Ctrl Pts',(-204.889078211633,-5.67027559591653,
126.69506520469));
#240081=CARTESIAN_POINT('Ctrl Pts',(-205.167525835445,-6.5221890759199,
133.353749521179));
#240082=CARTESIAN_POINT('Ctrl Pts',(-205.445973459259,-1.38052942180316,
137.66966997982));
#240083=CARTESIAN_POINT('Ctrl Pts',(-205.724421083071,5.02976932833932,
135.676706523556));
#240084=CARTESIAN_POINT('Ctrl Pts',(-206.002868706884,6.8179557836299,129.206295207017));
#240085=CARTESIAN_POINT('Ctrl Pts',(-206.281316330697,2.340773949421,124.204427932937));
#240086=CARTESIAN_POINT('Ctrl Pts',(-206.55976395451,-4.28746479114066,
125.267576371395));
#240087=CARTESIAN_POINT('Ctrl Pts',(-206.838211578323,-6.97573284294384,
131.418759045136));
#240088=CARTESIAN_POINT('Ctrl Pts',(-207.116659202136,-3.253643195576,137.005339578972));
#240089=CARTESIAN_POINT('Ctrl Pts',(-207.395106825949,3.4583855992191,136.893523381939));
#240090=CARTESIAN_POINT('Ctrl Pts',(-207.673554449762,6.99232697986142,
131.186064076586));
#240091=CARTESIAN_POINT('Ctrl Pts',(-207.952002073574,4.10066146017411,
125.127837939644));
#240092=CARTESIAN_POINT('Ctrl Pts',(-208.230449697387,-2.55931161296347,
124.286058830161));
#240093=CARTESIAN_POINT('Ctrl Pts',(-208.5088973212,-6.86740234311116,129.434280626559));
#240094=CARTESIAN_POINT('Ctrl Pts',(-208.787344945013,-4.86468581119477,
135.841539002563));
#240095=CARTESIAN_POINT('Ctrl Pts',(-209.065792568826,1.60843932809579,
137.619876522599));
#240096=CARTESIAN_POINT('Ctrl Pts',(-209.344240192639,6.60348730149562,
133.135087882371));
#240097=CARTESIAN_POINT('Ctrl Pts',(-209.622687816452,5.53025304311036,
126.508474748144));
#240098=CARTESIAN_POINT('Ctrl Pts',(-209.901135440264,-0.625013594012848,
123.829570862223));
#240099=CARTESIAN_POINT('Ctrl Pts',(-210.179583064078,-6.20592327184948,
127.56015802404));
#240100=CARTESIAN_POINT('Ctrl Pts',(-210.45803068789,-6.08389263906328,
134.272008881199));
#240101=CARTESIAN_POINT('Ctrl Pts',(-210.736478311703,-0.371061885656257,
137.797260388114));
#240102=CARTESIAN_POINT('Ctrl Pts',(-211.014925935516,5.68275661328764,
134.896378628042));
#240103=CARTESIAN_POINT('Ctrl Pts',(-211.293373559329,6.51439940271492,
128.235132222534));
#240104=CARTESIAN_POINT('Ctrl Pts',(-211.571821183142,1.35962738715011,
123.934881198276));
#240105=CARTESIAN_POINT('Ctrl Pts',(-211.850268806955,-5.04457577571481,
125.947346167619));
#240106=CARTESIAN_POINT('Ctrl Pts',(-212.128716430768,-6.81306024192543,
132.423170138115));
#240107=CARTESIAN_POINT('Ctrl Pts',(-212.40716405458,-2.32067518230222,
137.411387242468));
#240108=CARTESIAN_POINT('Ctrl Pts',(-212.685611678394,4.30429699857105,
136.32806964973));
#240109=CARTESIAN_POINT('Ctrl Pts',(-212.964059302206,6.97383051435588,
130.168733304621));
#240110=CARTESIAN_POINT('Ctrl Pts',(-213.24250692602,3.23475447800865,124.593507407987));
#240111=CARTESIAN_POINT('Ctrl Pts',(-213.520954549832,-3.47690289708716,
124.725752193909));
#240112=CARTESIAN_POINT('Ctrl Pts',(-213.799402173646,-6.99345636590915,
130.443941164641));
#240113=CARTESIAN_POINT('Ctrl Pts',(-214.077849797458,-4.08336508379785,
136.49333800514));
#240114=CARTESIAN_POINT('Ctrl Pts',(-214.356297421271,2.57913922684953,
137.314842548456));
#240115=CARTESIAN_POINT('Ctrl Pts',(-214.634745045084,6.87154058597789,
132.153532252007));
#240116=CARTESIAN_POINT('Ctrl Pts',(-214.913192668897,4.84933184001288,
125.752399134204));
#240117=CARTESIAN_POINT('Ctrl Pts',(-215.19164029271,-1.62917596389355,
123.993771817573));
#240118=CARTESIAN_POINT('Ctrl Pts',(-215.470087916522,-6.61055064665203,
128.493742892374));
#240119=CARTESIAN_POINT('Ctrl Pts',(-215.748535540335,-5.51715222849034,
135.117058776675));
#240120=CARTESIAN_POINT('Ctrl Pts',(-216.026983164148,0.646239559784443,
137.777215739773));
#240121=CARTESIAN_POINT('Ctrl Pts',(-216.305430787961,6.21576876317433,
134.029659488472));
#240122=CARTESIAN_POINT('Ctrl Pts',(-216.583878411774,6.0733101303926,127.318211139417));
#240123=CARTESIAN_POINT('Ctrl Pts',(-216.862326035587,0.349776185474419,
123.810363852911));
#240124=CARTESIAN_POINT('Ctrl Pts',(-217.1407736594,-5.69518498637811,126.729657917385));
#240125=CARTESIAN_POINT('Ctrl Pts',(-217.419221283213,-6.50654938100331,
133.393404703032));
#240126=CARTESIAN_POINT('Ctrl Pts',(-217.697668907026,-1.33871275709491,
137.67794645597));
#240127=CARTESIAN_POINT('Ctrl Pts',(-217.976116530838,5.05933549082977,
135.64599861675));
#240128=CARTESIAN_POINT('Ctrl Pts',(-218.254564154652,6.80810158496121,
129.164821983446));
#240129=CARTESIAN_POINT('Ctrl Pts',(-218.533011778464,2.30055491676597,
124.190301258982));
#240130=CARTESIAN_POINT('Ctrl Pts',(-218.811459402277,-4.32108933158155,
125.293777970294));
#240131=CARTESIAN_POINT('Ctrl Pts',(-219.08990702609,-6.97186358115499,
131.461210927519));
#240132=CARTESIAN_POINT('Ctrl Pts',(-219.368354649903,-3.21583579411804,
137.02503053882));
#240133=CARTESIAN_POINT('Ctrl Pts',(-219.646802273716,3.49538798540175,
136.872358389107));
#240134=CARTESIAN_POINT('Ctrl Pts',(-219.925249897529,6.99452096553273,
131.143492725519));
#240135=CARTESIAN_POINT('Ctrl Pts',(-220.203697521342,4.06603087968498,
125.102981222246));
#240136=CARTESIAN_POINT('Ctrl Pts',(-220.482145145155,-2.59894294794204,
124.301758855404));
#240137=CARTESIAN_POINT('Ctrl Pts',(-220.760592768967,-6.87561517183164,
129.476109838232));
#240138=CARTESIAN_POINT('Ctrl Pts',(-221.03904039278,-4.83393294528274,
135.87105839861));
#240139=CARTESIAN_POINT('Ctrl Pts',(-221.317488016593,1.64989750722823,
137.609959220154));
#240140=CARTESIAN_POINT('Ctrl Pts',(-221.595935640406,6.61755275257056,
133.094847397895));
#240141=CARTESIAN_POINT('Ctrl Pts',(-221.874383264219,5.5040003037252,126.474890121013));
#240142=CARTESIAN_POINT('Ctrl Pts',(-222.152830888031,-0.667459538880483,
123.83350472407));
#240143=CARTESIAN_POINT('Ctrl Pts',(-222.431278511845,-6.22555667246622,
127.597995348007));
#240144=CARTESIAN_POINT('Ctrl Pts',(-222.709726135657,-6.06267135940695,
134.308979015016));
#240145=CARTESIAN_POINT('Ctrl Pts',(-222.988173759471,-0.328487245014279,
137.799389584896));
#240146=CARTESIAN_POINT('Ctrl Pts',(-223.266621383283,5.70756060005303,
134.861710259961));
#240147=CARTESIAN_POINT('Ctrl Pts',(-223.545069007096,6.49863908350723,
128.195524826214));
#240148=CARTESIAN_POINT('Ctrl Pts',(-223.823516630909,1.31778572538753,
123.926732036005));
#240149=CARTESIAN_POINT('Ctrl Pts',(-224.101964254722,-5.07404833695195,
125.978143921416));
#240150=CARTESIAN_POINT('Ctrl Pts',(-224.380411878535,-6.80307985867417,
132.464613176793));
#240151=CARTESIAN_POINT('Ctrl Pts',(-224.658859502348,-2.28041333920269,
137.425391438088));
#240152=CARTESIAN_POINT('Ctrl Pts',(-224.937307126161,4.33784163461131,
136.30176583066));
#240153=CARTESIAN_POINT('Ctrl Pts',(-225.215754749974,6.96983206156226,
130.126293395573));
#240154=CARTESIAN_POINT('Ctrl Pts',(-225.494202373786,3.19688731916334,
124.573931612073));
#240155=CARTESIAN_POINT('Ctrl Pts',(-225.7726499976,-3.51384069291894,124.747029711241));
#240156=CARTESIAN_POINT('Ctrl Pts',(-226.051097621412,-6.9955207688696,
130.486518996257));
#240157=CARTESIAN_POINT('Ctrl Pts',(-226.329545245225,-4.04865900841799,
136.518089203828));
#240158=CARTESIAN_POINT('Ctrl Pts',(-226.607992869038,2.61872259278156,
137.299021971784));
#240159=CARTESIAN_POINT('Ctrl Pts',(-226.886440492851,6.87962606292594,
132.111678237058));
#240160=CARTESIAN_POINT('Ctrl Pts',(-227.164888116664,4.81848926965818,
125.722973476035));
#240161=CARTESIAN_POINT('Ctrl Pts',(-227.443335740477,-1.67060376613766,
124.003815258517));
#240162=CARTESIAN_POINT('Ctrl Pts',(-227.72178336429,-6.62449355438458,
128.534026000853));
#240163=CARTESIAN_POINT('Ctrl Pts',(-228.000230988102,-5.49079739065326,
135.150563343936));
#240164=CARTESIAN_POINT('Ctrl Pts',(-228.278678611916,0.688673334723007,
137.773152705292));
#240165=CARTESIAN_POINT('Ctrl Pts',(-228.557126235728,6.23528690905198,
133.991762582447));
#240166=CARTESIAN_POINT('Ctrl Pts',(-228.835573859542,6.05197642466173,
127.281305767118));
#240167=CARTESIAN_POINT('Ctrl Pts',(-229.114021483354,0.307195261492642,
123.808364248553));
#240168=CARTESIAN_POINT('Ctrl Pts',(-229.392469107167,-5.7198833396657,
126.764401619687));
#240169=CARTESIAN_POINT('Ctrl Pts',(-229.670916730979,-6.49066858350677,
133.432963946903));
#240170=CARTESIAN_POINT('Ctrl Pts',(-229.949364354793,-1.29684648589306,
137.685968228869));
#240171=CARTESIAN_POINT('Ctrl Pts',(-230.227811978605,5.0887141777831,135.615111301269));
#240172=CARTESIAN_POINT('Ctrl Pts',(-230.506259602419,6.79799510958498,
129.123409513582));
#240173=CARTESIAN_POINT('Ctrl Pts',(-230.784707226231,2.26025063620168,
124.176419671429));
#240174=CARTESIAN_POINT('Ctrl Pts',(-231.063154850045,-4.35455375246839,
125.32018376586));
#240175=CARTESIAN_POINT('Ctrl Pts',(-231.341602473857,-6.96773597439774,
131.503638470075));
#240176=CARTESIAN_POINT('Ctrl Pts',(-231.62005009767,-3.17790922868121,
137.044490989456));
#240177=CARTESIAN_POINT('Ctrl Pts',(-231.898497721483,3.53226084869627,
136.850968544386));
#240178=CARTESIAN_POINT('Ctrl Pts',(-232.176945345296,6.99645576665798,
131.100908807788));
#240179=CARTESIAN_POINT('Ctrl Pts',(-232.455392969109,4.03124963092651,
125.078335771559));
#240180=CARTESIAN_POINT('Ctrl Pts',(-232.733840592922,-2.63847797813309,
124.317699836946));
#240181=CARTESIAN_POINT('Ctrl Pts',(-233.012288216734,-6.88357322210384,
129.517988268725));
#240182=CARTESIAN_POINT('Ctrl Pts',(-233.290735840548,-4.80300095620762,
135.900390046307));
#240183=CARTESIAN_POINT('Ctrl Pts',(-233.56918346436,1.6912945488023,137.599789733751));
#240184=CARTESIAN_POINT('Ctrl Pts',(-233.847631088173,6.63137298779474,
133.05452203859));
#240185=CARTESIAN_POINT('Ctrl Pts',(-234.126078711986,5.47754361158473,
126.441465924004));
#240186=CARTESIAN_POINT('Ctrl Pts',(-234.404526335799,-0.709880750790079,
123.837696893545));
#240187=CARTESIAN_POINT('Ctrl Pts',(-234.682973959612,-6.24495938279112,
127.635951485018));
#240188=CARTESIAN_POINT('Ctrl Pts',(-234.961421583425,-6.04122542523402,
134.345819283911));
#240189=CARTESIAN_POINT('Ctrl Pts',(-235.239869207238,-0.285900432155891,
137.801259578306));
#240190=CARTESIAN_POINT('Ctrl Pts',(-235.518316831051,5.73215309106056,
134.826891545298));
#240191=CARTESIAN_POINT('Ctrl Pts',(-235.796764454864,6.48263795483918,
128.156014101264));
#240192=CARTESIAN_POINT('Ctrl Pts',(-236.075212078676,1.27589523259052,
123.918837726791));
#240193=CARTESIAN_POINT('Ctrl Pts',(-236.353659702489,-5.10333287746112,
126.009120512446));
#240194=CARTESIAN_POINT('Ctrl Pts',(-236.632107326302,-6.79284738479763,
132.505994694203));
#240195=CARTESIAN_POINT('Ctrl Pts',(-236.910554950115,-2.24006699454776,
137.439150288976));
#240196=CARTESIAN_POINT('Ctrl Pts',(-237.189002573928,4.3712255303347,136.275258303218));
#240197=CARTESIAN_POINT('Ctrl Pts',(-237.467450197741,6.96557533907847,
130.083878612554));
#240198=CARTESIAN_POINT('Ctrl Pts',(-237.745897821554,3.15890169848239,
124.554586686994));
#240199=CARTESIAN_POINT('Ctrl Pts',(-238.024345445366,-3.55064828209192,
124.768531685198));
#240200=CARTESIAN_POINT('Ctrl Pts',(-238.30279306918,-6.99732595023538,
130.529108605612));
#240201=CARTESIAN_POINT('Ctrl Pts',(-238.581240692992,-4.01380290848946,
136.542628678202));
#240202=CARTESIAN_POINT('Ctrl Pts',(-238.859688316805,2.65820892098533,
137.282960733047));
#240203=CARTESIAN_POINT('Ctrl Pts',(-239.138135940618,6.88745661279959,
132.069775778975));
#240204=CARTESIAN_POINT('Ctrl Pts',(-239.416583564431,4.78746814841248,
125.693736110535));
#240205=CARTESIAN_POINT('Ctrl Pts',(-239.695031188244,-1.71196966354462,
124.014110696169));
#240206=CARTESIAN_POINT('Ctrl Pts',(-239.973478812057,-6.63819098907155,
128.574393237416));
#240207=CARTESIAN_POINT('Ctrl Pts',(-240.25192643587,-5.46423908930053,
135.183906861057));
#240208=CARTESIAN_POINT('Ctrl Pts',(-240.530374059683,0.731081590618679,
137.768831439659));
#240209=CARTESIAN_POINT('Ctrl Pts',(-240.808821683496,6.25457400407998,
133.95374756607));
#240210=CARTESIAN_POINT('Ctrl Pts',(-241.087269307308,6.03041846071876,
127.244530942912));
#240211=CARTESIAN_POINT('Ctrl Pts',(-241.365716931122,0.264602954276818,
123.806623883412));
#240212=CARTESIAN_POINT('Ctrl Pts',(-241.644164554934,-5.74436974057257,
126.799295024156));
#240213=CARTESIAN_POINT('Ctrl Pts',(-241.922612178747,-6.47454727189872,
133.472425786911));
#240214=CARTESIAN_POINT('Ctrl Pts',(-242.20105980256,-1.25493215956847,
137.693735001267));
#240215=CARTESIAN_POINT('Ctrl Pts',(-242.479507426373,5.11790430056101,
135.584045721651));
#240216=CARTESIAN_POINT('Ctrl Pts',(-242.757955050186,6.78763673199965,
129.082059331979));
#240217=CARTESIAN_POINT('Ctrl Pts',(-243.036402673998,2.21986260121965,
124.162783684665));
#240218=CARTESIAN_POINT('Ctrl Pts',(-243.314850297812,-4.38785681376436,
125.346792779616));
#240219=CARTESIAN_POINT('Ctrl Pts',(-243.593297921624,-6.96335017562108,
131.54604010063));
#240220=CARTESIAN_POINT('Ctrl Pts',(-243.871745545438,-3.13986490465013,
137.063720209766));
#240221=CARTESIAN_POINT('Ctrl Pts',(-244.15019316925,3.56900282276695,136.829354640385));
#240222=CARTESIAN_POINT('Ctrl Pts',(-244.428640793064,6.99813131154132,
131.058313901354));
#240223=CARTESIAN_POINT('Ctrl Pts',(-244.707088416876,3.99631900273028,
125.053902500829));
#240224=CARTESIAN_POINT('Ctrl Pts',(-244.985536040689,-2.67791523855318,
124.333881184089));
#240225=CARTESIAN_POINT('Ctrl Pts',(-245.263983664501,-6.89127619903846,
129.559914366219));
#240226=CARTESIAN_POINT('Ctrl Pts',(-245.542431288315,-4.7718909901659,
135.929532858758));
#240227=CARTESIAN_POINT('Ctrl Pts',(-245.820878912128,1.73262891883438,
137.589368440225));
#240228=CARTESIAN_POINT('Ctrl Pts',(-246.09932653594,6.6449474950541,133.014113298726));
#240229=CARTESIAN_POINT('Ctrl Pts',(-246.377774159753,5.45088394705135,
126.408203395661));
#240230=CARTESIAN_POINT('Ctrl Pts',(-246.656221783566,-0.752275657806765,
123.842147215306));
#240231=CARTESIAN_POINT('Ctrl Pts',(-246.934669407379,-6.26413068384941,
127.674025028594));
#240232=CARTESIAN_POINT('Ctrl Pts',(-247.213117031192,-6.01955563123113,
134.382528322752));
#240233=CARTESIAN_POINT('Ctrl Pts',(-247.491564655005,-0.243303025152602,
137.802870299053));
#240234=CARTESIAN_POINT('Ctrl Pts',(-247.770012278818,5.75653317502817,
134.791923774272));
#240235=CARTESIAN_POINT('Ctrl Pts',(-248.048459902631,6.46639660963695,
128.116601511768));
#240236=CARTESIAN_POINT('Ctrl Pts',(-248.326907526444,1.23395746102625,
123.91119856316));
#240237=CARTESIAN_POINT('Ctrl Pts',(-248.605355150257,-5.13242831209467,
126.040274792862));
#240238=CARTESIAN_POINT('Ctrl Pts',(-248.883802774069,-6.78236319946242,
132.547313156937));
#240239=CARTESIAN_POINT('Ctrl Pts',(-249.162250397883,-2.19963764338714,
137.452663285294));
#240240=CARTESIAN_POINT('Ctrl Pts',(-249.440698021695,4.40444744868852,
136.24854804965));
#240241=CARTESIAN_POINT('Ctrl Pts',(-249.719145645508,6.96106050463867,
130.041490527264));
#240242=CARTESIAN_POINT('Ctrl Pts',(-249.997593269321,3.12079902353814,
124.535473349588));
#240243=CARTESIAN_POINT('Ctrl Pts',(-250.276040893134,-3.58732430068758,
124.790257319018));
#240244=CARTESIAN_POINT('Ctrl Pts',(-250.554488516946,-6.99887184311352,
130.571708414529));
#240245=CARTESIAN_POINT('Ctrl Pts',(-250.83293614076,-3.97879807562073,
136.566955518948));
#240246=CARTESIAN_POINT('Ctrl Pts',(-251.111383764572,2.69759674828547,
137.26665942739));
#240247=CARTESIAN_POINT('Ctrl Pts',(-251.389831388386,6.89503194542569,
132.027826430486));
#240248=CARTESIAN_POINT('Ctrl Pts',(-251.668279012198,4.75626962579305,
125.66468812107));
#240249=CARTESIAN_POINT('Ctrl Pts',(-251.946726636011,-1.75327212332407,
124.024657749096));
#240250=CARTESIAN_POINT('Ctrl Pts',(-252.225174259824,-6.65164244307981,
128.614843106116));
#240251=CARTESIAN_POINT('Ctrl Pts',(-252.503621883637,-5.43747830869239,
135.217088092717));
#240252=CARTESIAN_POINT('Ctrl Pts',(-252.78206950745,0.773462756270139,
137.764252102553));
#240253=CARTESIAN_POINT('Ctrl Pts',(-253.060517131263,6.2736293330892,133.91561584884));
#240254=CARTESIAN_POINT('Ctrl Pts',(-253.338964755075,6.00863703830687,
127.207888027921));
#240255=CARTESIAN_POINT('Ctrl Pts',(-253.617412378889,0.222000840393564,
123.805142824969));
#240256=CARTESIAN_POINT('Ctrl Pts',(-253.895860002702,-5.76864327852066,
126.83433683216));
#240257=CARTESIAN_POINT('Ctrl Pts',(-254.174307626514,-6.45818604965135,
133.511788771436));
#240258=CARTESIAN_POINT('Ctrl Pts',(-254.452755250327,-1.21297131977014,
137.701246465247));
#240259=CARTESIAN_POINT('Ctrl Pts',(-254.73120287414,5.14690475579816,135.55280306703));
#240260=CARTESIAN_POINT('Ctrl Pts',(-255.009650497953,6.7770268770417,129.040772899161));
#240261=CARTESIAN_POINT('Ctrl Pts',(-255.288098121766,2.17939223099114,
124.149393939406));
#240262=CARTESIAN_POINT('Ctrl Pts',(-255.566545745579,-4.42099713522674,
125.37360376984));
#240263=CARTESIAN_POINT('Ctrl Pts',(-255.844993369392,-6.95870662337211,
131.588414730824));
#240264=CARTESIAN_POINT('Ctrl Pts',(-256.123440993205,-3.10170371057109,
137.082716575498));
#240265=CARTESIAN_POINT('Ctrl Pts',(-256.401888617018,3.60561156199617,
136.807519199501));
#240266=CARTESIAN_POINT('Ctrl Pts',(-256.68033624083,6.99954939633056,131.01570633407));
#240267=CARTESIAN_POINT('Ctrl Pts',(-256.958783864643,3.96123678073902,
125.029688453078));
#240268=CARTESIAN_POINT('Ctrl Pts',(-257.237231488456,-2.71724664265218,
124.350290708114));
#240269=CARTESIAN_POINT('Ctrl Pts',(-257.515679112269,-6.89873632689917,
129.601908459729));
#240270=CARTESIAN_POINT('Ctrl Pts',(-257.794126736082,-4.74058057908887,
135.958444437253));
#240271=CARTESIAN_POINT('Ctrl Pts',(-258.072574359895,1.77385448465437,
137.578773744179));
#240272=CARTESIAN_POINT('Ctrl Pts',(-258.351021983707,6.6583599873155,132.973475360041));
#240273=CARTESIAN_POINT('Ctrl Pts',(-258.629469607521,5.42386327951784,
126.375381938049));
#240274=CARTESIAN_POINT('Ctrl Pts',(-258.907917231333,-0.794342416617398,
123.846330221273));
#240275=CARTESIAN_POINT('Ctrl Pts',(-259.186364855146,-6.28363694765996,
127.713206958712));
#240276=CARTESIAN_POINT('Ctrl Pts',(-259.464812478959,-5.99659113747434,
134.41722675292));
#240277=CARTESIAN_POINT('Ctrl Pts',(-259.743260102772,-0.202727240537578,
137.807801967267));
#240278=CARTESIAN_POINT('Ctrl Pts',(-260.021707726585,5.7845923739281,134.749768174183));
#240279=CARTESIAN_POINT('Ctrl Pts',(-260.253747413096,6.33253704604016,
129.202365411857));
#240280=CARTESIAN_POINT('Ctrl Pts',(-260.439389088604,3.82430165355141,
125.973250269562));
#240281=CARTESIAN_POINT('Ctrl Pts',(-260.532214889509,1.97943258085903,
125.138073123498));
#240282=CARTESIAN_POINT('Ctrl Pts',(-260.578632753112,1.00712299976162,
124.970230583726));
#240283=CARTESIAN_POINT('',(177.476367722506,5.62666147572432,130.804360632945));
#240284=CARTESIAN_POINT('Ctrl Pts',(177.727351910922,4.07805626267757,128.049722934653));
#240285=CARTESIAN_POINT('Ctrl Pts',(177.71910609987,4.13364155314972,128.094597587437));
#240286=CARTESIAN_POINT('Ctrl Pts',(177.710836728767,4.1882073110253,128.140733789961));
#240287=CARTESIAN_POINT('Ctrl Pts',(177.668436485582,4.46292964568284,128.384086882844));
#240288=CARTESIAN_POINT('Ctrl Pts',(177.634553719226,4.66558123475735,128.601241704498));
#240289=CARTESIAN_POINT('Ctrl Pts',(177.567013746104,5.05830116010295,129.120170708466));
#240290=CARTESIAN_POINT('Ctrl Pts',(177.534914197562,5.23713864285283,129.429348263662));
#240291=CARTESIAN_POINT('Ctrl Pts',(177.491184739739,5.49518559902329,130.065605691881));
#240292=CARTESIAN_POINT('Ctrl Pts',(177.478557559001,5.57905246121522,130.386047316322));
#240293=CARTESIAN_POINT('Ctrl Pts',(177.476455077554,5.62086138792093,130.74479140865));
#240294=CARTESIAN_POINT('Ctrl Pts',(177.476367722476,5.62395081735113,130.774568592934));
#240295=CARTESIAN_POINT('Ctrl Pts',(177.476367722506,5.62666147433654,130.804360633071));
#240296=CARTESIAN_POINT('Ctrl Pts',(207.343245771341,2.3877455813801,126.510892848288));
#240297=CARTESIAN_POINT('Ctrl Pts',(207.275858229453,2.15528266814333,126.281350675543));
#240298=CARTESIAN_POINT('Ctrl Pts',(207.205844547368,1.89354568495696,126.064552767189));
#240299=CARTESIAN_POINT('Ctrl Pts',(207.10286979807,1.39124105048774,125.761845041447));
#240300=CARTESIAN_POINT('Ctrl Pts',(207.06364877788,1.14897513173755,125.652900568378));
#240301=CARTESIAN_POINT('Ctrl Pts',(207.039544129699,0.852522970188626,
125.586612482375));
#240302=CARTESIAN_POINT('Ctrl Pts',(207.036751493533,0.812407362098567,
125.578958169151));
#240303=CARTESIAN_POINT('Ctrl Pts',(207.034346644558,0.770380885625219,
125.572377570558));
#240304=CARTESIAN_POINT('Ctrl Pts',(207.034253959284,0.76874693830571,125.572123968997));
#240305=CARTESIAN_POINT('Ctrl Pts',(207.034033708417,0.76482971591445,125.571521376621));
#240306=CARTESIAN_POINT('Ctrl Pts',(207.03390689775,0.762546089248627,125.571174470768));
#240307=CARTESIAN_POINT('Ctrl Pts',(207.033710514163,0.758964574572171,
125.570637298871));
#240308=CARTESIAN_POINT('Ctrl Pts',(207.033639889101,0.757667190070412,
125.570444129042));
#240309=CARTESIAN_POINT('Ctrl Pts',(207.033544370583,0.755899632091822,
125.570182888153));
#240310=CARTESIAN_POINT('Ctrl Pts',(207.033519040958,0.755429661562308,
125.570113613793));
#240311=CARTESIAN_POINT('Ctrl Pts',(207.033487449577,0.75484194224604,125.570027216002));
#240312=CARTESIAN_POINT('Ctrl Pts',(207.033481126023,0.754724221366939,
125.570009922105));
#240313=CARTESIAN_POINT('Ctrl Pts',(207.033468679808,0.75449236414991,125.569975883918));
#240314=CARTESIAN_POINT('Ctrl Pts',(207.033462556857,0.754378227124989,
125.569959138824));
#240315=CARTESIAN_POINT('Ctrl Pts',(207.033453376976,0.7542069949192,125.569934033751));
#240316=CARTESIAN_POINT('Ctrl Pts',(207.033450317046,0.754149899488901,
125.569925665499));
#240317=CARTESIAN_POINT('Ctrl Pts',(207.033444862271,0.754048085319076,
125.5699107479));
#240318=CARTESIAN_POINT('Ctrl Pts',(207.033442467482,0.754003374824332,
125.569904198698));
#240319=CARTESIAN_POINT('Ctrl Pts',(207.033437443175,0.75390954752979,125.569890458394));
#240320=CARTESIAN_POINT('Ctrl Pts',(207.033434813833,0.753860431646158,
125.569883267775));
#240321=CARTESIAN_POINT('Ctrl Pts',(207.033427919641,0.753731612570639,
125.569864413858));
#240322=CARTESIAN_POINT('Ctrl Pts',(207.033423655866,0.753651906963209,
125.569852753528));
#240323=CARTESIAN_POINT('Ctrl Pts',(207.03340516309,0.753306051493517,125.569802180728));
#240324=CARTESIAN_POINT('Ctrl Pts',(207.033390953313,0.753039892352538,
125.569763321276));
#240325=CARTESIAN_POINT('Ctrl Pts',(207.032637262426,0.738901169539525,
125.567702230136));
#240326=CARTESIAN_POINT('Ctrl Pts',(207.031955337296,0.72500443032654,125.565838715569));
#240327=CARTESIAN_POINT('Ctrl Pts',(207.02839943031,0.645577309011463,125.556126262888));
#240328=CARTESIAN_POINT('Ctrl Pts',(207.026791222654,0.58006201298121,125.55175022771));
#240329=CARTESIAN_POINT('Ctrl Pts',(207.026066210465,0.390615670661435,
125.549775550373));
#240330=CARTESIAN_POINT('Ctrl Pts',(207.030357517256,0.268505495823795,
125.561416336111));
#240331=CARTESIAN_POINT('Ctrl Pts',(207.051180759308,-0.0272120970339418,
125.618546972655));
#240332=CARTESIAN_POINT('Ctrl Pts',(207.072035822298,-0.195505216489052,
125.676082796202));
#240333=CARTESIAN_POINT('Ctrl Pts',(207.11742615221,-0.475952586113691,
125.805214506685));
#240334=CARTESIAN_POINT('Ctrl Pts',(207.139776849114,-0.591942288014956,
125.869844509151));
#240335=CARTESIAN_POINT('Ctrl Pts',(207.16361981536,-0.702841334627603,
125.940658199356));
#240336=CARTESIAN_POINT('Ctrl Pts',(207.300060471638,3.90699806772733,135.242283170685));
#240337=CARTESIAN_POINT('Ctrl Pts',(207.34413274425,3.94262575384843,135.097475191392));
#240338=CARTESIAN_POINT('Ctrl Pts',(207.386092965017,3.97836208698807,134.951861709998));
#240339=CARTESIAN_POINT('Ctrl Pts',(207.469685208882,4.05173223617054,134.644592220037));
#240340=CARTESIAN_POINT('Ctrl Pts',(207.510886564299,4.08921616848532,134.482726191452));
#240341=CARTESIAN_POINT('Ctrl Pts',(207.592391673631,4.16413723955857,134.138864482574));
#240342=CARTESIAN_POINT('Ctrl Pts',(207.632065558946,4.20108743265175,133.956753701393));
#240343=CARTESIAN_POINT('Ctrl Pts',(207.710182522622,4.27216743944126,133.563382656296));
#240344=CARTESIAN_POINT('Ctrl Pts',(207.747210242616,4.30461553044184,133.35420995967));
#240345=CARTESIAN_POINT('Ctrl Pts',(207.780393500533,4.3310565938262,133.140241056514));
#240346=CARTESIAN_POINT('Ctrl Pts',(178.535810555027,-1.96534307107584,
125.221017543274));
#240347=CARTESIAN_POINT('Ctrl Pts',(178.572363368561,-1.60399563351745,
125.128167470391));
#240348=CARTESIAN_POINT('Ctrl Pts',(178.600500782542,-1.23860474272998,
125.059173954896));
#240349=CARTESIAN_POINT('Ctrl Pts',(178.621003548882,-0.856428478077489,
125.009278016813));
#240350=CARTESIAN_POINT('Ctrl Pts',(178.621801810245,-0.841279080621699,
125.007336534832));
#240351=CARTESIAN_POINT('Ctrl Pts',(178.623990647172,-0.798973658475563,
125.002015992207));
#240352=CARTESIAN_POINT('Ctrl Pts',(178.625349900214,-0.771805929769255,
124.998715493147));
#240353=CARTESIAN_POINT('Ctrl Pts',(178.62668571351,-0.744165676501276,
124.995474921175));
#240354=CARTESIAN_POINT('Ctrl Pts',(178.626707795983,-0.743708481662123,
124.995421351801));
#240355=CARTESIAN_POINT('Ctrl Pts',(178.626816871274,-0.741448850750257,
124.995156752781));
#240356=CARTESIAN_POINT('Ctrl Pts',(178.626903676827,-0.739646350809624,
124.994946190002));
#240357=CARTESIAN_POINT('Ctrl Pts',(178.627010610293,-0.737420683462579,
124.9946868197));
#240358=CARTESIAN_POINT('Ctrl Pts',(178.627030927358,-0.736997579512831,
124.994637540787));
#240359=CARTESIAN_POINT('Ctrl Pts',(178.62706240287,-0.736341738602775,
124.99456119827));
#240360=CARTESIAN_POINT('Ctrl Pts',(178.627073568876,-0.736109006983649,
124.99453411582));
#240361=CARTESIAN_POINT('Ctrl Pts',(178.627094018329,-0.735682652195354,
124.994484517351));
#240362=CARTESIAN_POINT('Ctrl Pts',(178.627103302812,-0.735489029217585,
124.994461998755));
#240363=CARTESIAN_POINT('Ctrl Pts',(178.627123488216,-0.735067966852662,
124.994413041381));
#240364=CARTESIAN_POINT('Ctrl Pts',(178.627134388279,-0.734840526798812,
124.994386604746));
#240365=CARTESIAN_POINT('Ctrl Pts',(178.627164443798,-0.734213203786545,
124.994313709709));
#240366=CARTESIAN_POINT('Ctrl Pts',(178.627183592622,-0.733813317949453,
124.994267267836));
#240367=CARTESIAN_POINT('Ctrl Pts',(178.62728583349,-0.73167710034013,124.994019305302));
#240368=CARTESIAN_POINT('Ctrl Pts',(178.627368749657,-0.729940710022163,
124.993818222811));
#240369=CARTESIAN_POINT('Ctrl Pts',(178.629059143694,-0.69446056615761,
124.989719045218));
#240370=CARTESIAN_POINT('Ctrl Pts',(178.630596698252,-0.660693007946553,
124.985995081663));
#240371=CARTESIAN_POINT('Ctrl Pts',(178.634998934465,-0.559328070586893,
124.975343706825));
#240372=CARTESIAN_POINT('Ctrl Pts',(178.637653366489,-0.491663502550943,
124.968936267428));
#240373=CARTESIAN_POINT('Ctrl Pts',(178.652290692225,-0.0741053585462007,
124.933657265026));
#240374=CARTESIAN_POINT('Ctrl Pts',(178.65706528323,0.278036573125624,124.922313922981));
#240375=CARTESIAN_POINT('Ctrl Pts',(178.654556968681,0.629286258110217,
124.928317377817));
#240376=CARTESIAN_POINT('Ctrl Pts',(177.476367722506,5.62666147433657,130.804360633071));
#240377=CARTESIAN_POINT('Ctrl Pts',(177.476367722745,5.64800886896215,131.038983619647));
#240378=CARTESIAN_POINT('Ctrl Pts',(177.481815845156,5.64587111696085,131.2745273672));
#240379=CARTESIAN_POINT('Ctrl Pts',(177.493340279704,5.61850113655357,131.523613241248));
#240380=CARTESIAN_POINT('Ctrl Pts',(177.494046319909,5.61678087678775,131.538405721014));
#240381=CARTESIAN_POINT('Ctrl Pts',(177.494830441239,5.6148248201693,131.554346920936));
#240382=CARTESIAN_POINT('Ctrl Pts',(177.494887671502,5.61468180143515,131.555507707183));
#240383=CARTESIAN_POINT('Ctrl Pts',(177.494958749217,5.61450386495011,131.556946013306));
#240384=CARTESIAN_POINT('Ctrl Pts',(177.494972474835,5.61446948972427,131.557223606544));
#240385=CARTESIAN_POINT('Ctrl Pts',(177.494993809106,5.61441603657773,131.557654841551));
#240386=CARTESIAN_POINT('Ctrl Pts',(177.495001412615,5.61439698152929,131.557808486065));
#240387=CARTESIAN_POINT('Ctrl Pts',(177.495015372434,5.61436198892514,131.558090486421));
#240388=CARTESIAN_POINT('Ctrl Pts',(177.495021728047,5.6143460544523,131.558218842378));
#240389=CARTESIAN_POINT('Ctrl Pts',(177.49503551666,5.61431147766019,131.558497241617));
#240390=CARTESIAN_POINT('Ctrl Pts',(177.495042950192,5.61429283288377,131.558647283569));
#240391=CARTESIAN_POINT('Ctrl Pts',(177.495063575169,5.6142410896851,131.559063463467));
#240392=CARTESIAN_POINT('Ctrl Pts',(177.49507677126,5.61420797059531,131.559329598846));
#240393=CARTESIAN_POINT('Ctrl Pts',(177.495147761058,5.614029731868,131.560760544247));
#240394=CARTESIAN_POINT('Ctrl Pts',(177.495205678106,5.61388406288704,131.561925280089));
#240395=CARTESIAN_POINT('Ctrl Pts',(177.498353203655,5.60595394007177,131.625077226177));
#240396=CARTESIAN_POINT('Ctrl Pts',(177.501809975298,5.59653185305586,131.686815725141));
#240397=CARTESIAN_POINT('Ctrl Pts',(177.517258408342,5.55180098308332,131.935795836193));
#240398=CARTESIAN_POINT('Ctrl Pts',(177.53216773447,5.50319392797717,132.119815974191));
#240399=CARTESIAN_POINT('Ctrl Pts',(177.579958465937,5.33412594249757,132.604732031663));
#240400=CARTESIAN_POINT('Ctrl Pts',(177.61742104521,5.18961629328228,132.891229558403));
#240401=CARTESIAN_POINT('Ctrl Pts',(177.722598493876,4.74529882642138,133.563053730255));
#240402=CARTESIAN_POINT('Ctrl Pts',(177.794691730185,4.41119386074116,133.919144338343));
#240403=CARTESIAN_POINT('Ctrl Pts',(177.927395241577,3.71809800550664,134.49513348593));
#240404=CARTESIAN_POINT('Ctrl Pts',(177.989174049252,3.36304316837917,134.730227794869));
#240405=CARTESIAN_POINT('Ctrl Pts',(178.082682503228,2.74398222802927,135.062813747627));
#240406=CARTESIAN_POINT('Ctrl Pts',(178.117862998488,2.48723912541729,135.181048337578));
#240407=CARTESIAN_POINT('Ctrl Pts',(178.197858320915,1.82144645103899,135.441236023159));
#240408=CARTESIAN_POINT('Ctrl Pts',(178.238066467768,1.40117430183672,135.563242037453));
#240409=CARTESIAN_POINT('Ctrl Pts',(178.266323014416,0.960634556419806,
135.647607167646));
#240410=CARTESIAN_POINT('Ctrl Pts',(178.267150551097,0.947540843553741,
135.650075767119));
#240411=CARTESIAN_POINT('Ctrl Pts',(178.268982584149,0.918113096294057,
135.655536346135));
#240412=CARTESIAN_POINT('Ctrl Pts',(178.26998060066,0.901773160982638,135.658507888363));
#240413=CARTESIAN_POINT('Ctrl Pts',(178.271818928666,0.871078974814065,
135.663976038944));
#240414=CARTESIAN_POINT('Ctrl Pts',(178.27266304642,0.856736664322277,135.666484646891));
#240415=CARTESIAN_POINT('Ctrl Pts',(178.273548891525,0.841415948934087,
135.669115076619));
#240416=CARTESIAN_POINT('Ctrl Pts',(178.273604905292,0.840446016661627,
135.669281394459));
#240417=CARTESIAN_POINT('Ctrl Pts',(178.273680705371,0.83913187483764,135.66950644962));
#240418=CARTESIAN_POINT('Ctrl Pts',(178.27370054899,0.838787699115299,135.669565365371));
#240419=CARTESIAN_POINT('Ctrl Pts',(178.273733193885,0.838221249282319,
135.669662286179));
#240420=CARTESIAN_POINT('Ctrl Pts',(178.273745999974,0.837998977982071,
135.66970030622));
#240421=CARTESIAN_POINT('Ctrl Pts',(178.273770748392,0.837569307966119,
135.669773780926));
#240422=CARTESIAN_POINT('Ctrl Pts',(178.273782691233,0.837361908358778,
135.669809237174));
#240423=CARTESIAN_POINT('Ctrl Pts',(178.273810458122,0.8368795828714,135.669891671306));
#240424=CARTESIAN_POINT('Ctrl Pts',(178.273826279791,0.836604657560614,
135.669938641801));
#240425=CARTESIAN_POINT('Ctrl Pts',(178.273876010189,0.835740219580388,
135.670086276272));
#240426=CARTESIAN_POINT('Ctrl Pts',(178.273909899986,0.835150695482057,
135.670186881322));
#240427=CARTESIAN_POINT('Ctrl Pts',(178.274371088221,0.827122245215414,
135.671555914787));
#240428=CARTESIAN_POINT('Ctrl Pts',(178.274794555457,0.819681066691097,
135.672812421509));
#240429=CARTESIAN_POINT('Ctrl Pts',(178.28084223278,0.712402304277549,135.69074942723));
#240430=CARTESIAN_POINT('Ctrl Pts',(178.285775955922,0.612166885418918,
135.705288668747));
#240431=CARTESIAN_POINT('Ctrl Pts',(178.299419217276,0.288637961509831,
135.745352837328));
#240432=CARTESIAN_POINT('Ctrl Pts',(178.305399847096,0.0641175829676573,
135.762692232661));
#240433=CARTESIAN_POINT('Ctrl Pts',(178.311924012651,-0.490333735750563,
135.781624064638));
#240434=CARTESIAN_POINT('Ctrl Pts',(178.308617172973,-0.821441843563681,
135.772121437776));
#240435=CARTESIAN_POINT('Ctrl Pts',(178.285319321399,-1.5965832586439,135.704101279333));
#240436=CARTESIAN_POINT('Ctrl Pts',(178.259606239746,-2.04175646283672,
135.628895105993));
#240437=CARTESIAN_POINT('Ctrl Pts',(178.197253864959,-2.79960490124737,
135.437212662791));
#240438=CARTESIAN_POINT('Ctrl Pts',(178.164853130157,-3.11943053718718,
135.335366999488));
#240439=CARTESIAN_POINT('Ctrl Pts',(178.08645413946,-3.78099261367155,135.075940074041));
#240440=CARTESIAN_POINT('Ctrl Pts',(178.038838181365,-4.12315427920155,
134.911670696906));
#240441=CARTESIAN_POINT('Ctrl Pts',(177.9874951389,-4.44976524376849,134.718437431287));
#240442=CARTESIAN_POINT('Origin',(192.718407221598,12.,130.804360617566));
#240443=CARTESIAN_POINT('',(177.476367722507,-12.,130.804360617566));
#240444=CARTESIAN_POINT('Origin',(192.718407221598,-12.,130.804360617566));
#240445=CARTESIAN_POINT('',(177.476367722506,12.,130.804360617566));
#240446=CARTESIAN_POINT('',(177.476367722507,12.,130.804360617566));
#240447=CARTESIAN_POINT('',(177.476367722506,12.,130.804360617566));
#240448=CARTESIAN_POINT('Origin',(192.718407221598,12.,130.804360617566));
#240449=CARTESIAN_POINT('Origin',(192.718407221598,-12.,130.804360617566));
#240450=CARTESIAN_POINT('Origin',(192.718407221598,12.,130.804360617566));
#279249=UNCERTAINTY_MEASURE_WITH_UNIT(LENGTH_MEASURE(0.01),#279267,
'DISTANCE_ACCURACY_VALUE',
'Maximum model space distance between geometric entities at asserted c
onnectivities');
#279255=UNCERTAINTY_MEASURE_WITH_UNIT(LENGTH_MEASURE(0.01),#279267,
'DISTANCE_ACCURACY_VALUE',
'Maximum model space distance between geometric entities at asserted c
onnectivities');
#279260=(
GEOMETRIC_REPRESENTATION_CONTEXT(3)
GLOBAL_UNCERTAINTY_ASSIGNED_CONTEXT((#279249))
GLOBAL_UNIT_ASSIGNED_CONTEXT((#279267,#279269,#279270))
REPRESENTATION_CONTEXT('','3D')
);
#279266=(
GEOMETRIC_REPRESENTATION_CONTEXT(3)
GLOBAL_UNCERTAINTY_ASSIGNED_CONTEXT((#279255))
GLOBAL_UNIT_ASSIGNED_CONTEXT((#279267,#279269,#279270))
REPRESENTATION_CONTEXT('','3D')
);
#279267=(
LENGTH_UNIT()
NAMED_UNIT(*)
SI_UNIT(.MILLI.,.METRE.)
);
#279269=(
NAMED_UNIT(*)
PLANE_ANGLE_UNIT()
SI_UNIT($,.RADIAN.)
);
#279270=(
NAMED_UNIT(*)
SI_UNIT($,.STERADIAN.)
SOLID_ANGLE_UNIT()
);
#279275=SHAPE_DEFINITION_REPRESENTATION(#279285,#279304);
#279285=PRODUCT_DEFINITION_SHAPE('',$,#279315);
#279304=SHAPE_REPRESENTATION('',(#15446),#279260);
#279310=PRODUCT_DEFINITION_CONTEXT('part definition',#279342,'design');
#279315=PRODUCT_DEFINITION('Shaft_01','Shaft_01',#279325,#279310);
#279325=PRODUCT_DEFINITION_FORMATION('',$,#279348);
#279342=APPLICATION_CONTEXT(
'Core Data for Automotive Mechanical Design Process');
#279343=PRODUCT_CONTEXT('part definition',#279342,'mechanical');
#279348=PRODUCT('Shaft_01','Shaft_01',$,(#279343));
#279355=PRESENTATION_STYLE_ASSIGNMENT((#279357));
#279357=SURFACE_STYLE_USAGE(.BOTH.,#279359);
#279359=SURFACE_SIDE_STYLE('',(#279361));
#279361=SURFACE_STYLE_FILL_AREA(#279363);
#279363=FILL_AREA_STYLE('Opaque(160,160,160)',(#279365));
#279365=FILL_AREA_STYLE_COLOUR('Opaque(160,160,160)',#279367);
#279367=COLOUR_RGB('Opaque(160,160,160)', 0.66274510, 0.83137255, 0.94901961);
ENDSEC;
END-ISO-10303-21;
